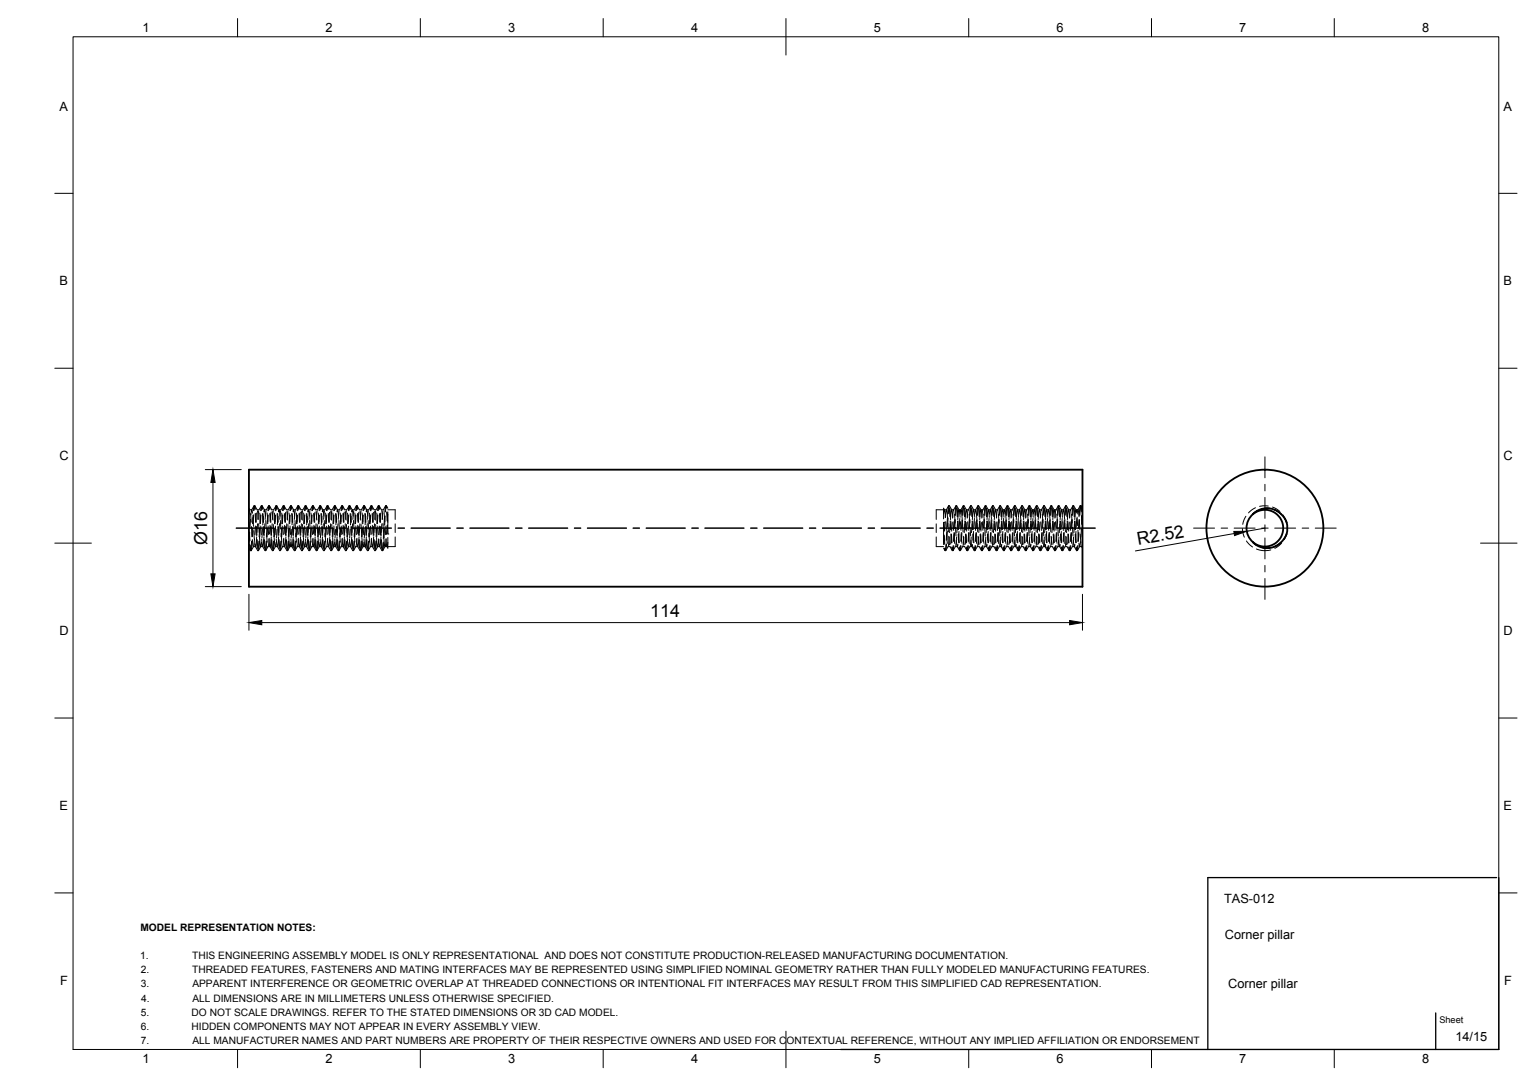
ISO-10303-21;
HEADER;
/* Generated by software containing ST-Developer
 * from STEP Tools, Inc. (www.steptools.com) 
 */

FILE_DESCRIPTION(
/* description */ (
'Independent welded steel electronics enclosure with removable sealed 
lid, internal mounting tray and two threaded cable entries. 300 x 220 
mm body. No ingress or electrical safety rating assigned.'),
/* implementation_level */ '2;1');

FILE_NAME(
/* name */ 'Corner pillar.step',
/* time_stamp */ '2026-11-14T09:13:27-08:00',
/* author */ (''),
/* organization */ (''),
/* preprocessor_version */ 'ST-DEVELOPER v20.2',
/* originating_system */ 'Autodesk Translation Framework v15.17.0.0',
/* authorisation */ '');

FILE_SCHEMA (('AUTOMOTIVE_DESIGN { 1 0 10303 214 3 1 1 }'));
ENDSEC;

DATA;
#10=MECHANICAL_DESIGN_GEOMETRIC_PRESENTATION_REPRESENTATION('',(#970),#94412);
#154=B_SPLINE_SURFACE_WITH_KNOTS('',3,3,((#38427,#38428,#38429,#38430,#38431,
#38432,#38433,#38434,#38435,#38436,#38437,#38438,#38439,#38440,#38441,#38442,
#38443,#38444,#38445,#38446,#38447,#38448,#38449,#38450,#38451,#38452,#38453,
#38454,#38455,#38456,#38457,#38458,#38459,#38460,#38461,#38462,#38463,#38464,
#38465,#38466,#38467,#38468,#38469,#38470,#38471,#38472,#38473,#38474,#38475,
#38476,#38477,#38478,#38479,#38480,#38481,#38482,#38483,#38484,#38485,#38486,
#38487,#38488,#38489,#38490,#38491,#38492,#38493,#38494,#38495,#38496,#38497,
#38498,#38499,#38500,#38501,#38502,#38503,#38504,#38505,#38506,#38507,#38508,
#38509,#38510,#38511,#38512,#38513,#38514,#38515,#38516,#38517,#38518,#38519,
#38520,#38521,#38522,#38523,#38524,#38525,#38526,#38527,#38528,#38529,#38530,
#38531,#38532,#38533,#38534,#38535,#38536,#38537,#38538,#38539,#38540,#38541,
#38542,#38543,#38544,#38545,#38546,#38547,#38548,#38549,#38550,#38551),
(#38552,#38553,#38554,#38555,#38556,#38557,#38558,#38559,#38560,#38561,
#38562,#38563,#38564,#38565,#38566,#38567,#38568,#38569,#38570,#38571,#38572,
#38573,#38574,#38575,#38576,#38577,#38578,#38579,#38580,#38581,#38582,#38583,
#38584,#38585,#38586,#38587,#38588,#38589,#38590,#38591,#38592,#38593,#38594,
#38595,#38596,#38597,#38598,#38599,#38600,#38601,#38602,#38603,#38604,#38605,
#38606,#38607,#38608,#38609,#38610,#38611,#38612,#38613,#38614,#38615,#38616,
#38617,#38618,#38619,#38620,#38621,#38622,#38623,#38624,#38625,#38626,#38627,
#38628,#38629,#38630,#38631,#38632,#38633,#38634,#38635,#38636,#38637,#38638,
#38639,#38640,#38641,#38642,#38643,#38644,#38645,#38646,#38647,#38648,#38649,
#38650,#38651,#38652,#38653,#38654,#38655,#38656,#38657,#38658,#38659,#38660,
#38661,#38662,#38663,#38664,#38665,#38666,#38667,#38668,#38669,#38670,#38671,
#38672,#38673,#38674,#38675,#38676),(#38677,#38678,#38679,#38680,#38681,
#38682,#38683,#38684,#38685,#38686,#38687,#38688,#38689,#38690,#38691,#38692,
#38693,#38694,#38695,#38696,#38697,#38698,#38699,#38700,#38701,#38702,#38703,
#38704,#38705,#38706,#38707,#38708,#38709,#38710,#38711,#38712,#38713,#38714,
#38715,#38716,#38717,#38718,#38719,#38720,#38721,#38722,#38723,#38724,#38725,
#38726,#38727,#38728,#38729,#38730,#38731,#38732,#38733,#38734,#38735,#38736,
#38737,#38738,#38739,#38740,#38741,#38742,#38743,#38744,#38745,#38746,#38747,
#38748,#38749,#38750,#38751,#38752,#38753,#38754,#38755,#38756,#38757,#38758,
#38759,#38760,#38761,#38762,#38763,#38764,#38765,#38766,#38767,#38768,#38769,
#38770,#38771,#38772,#38773,#38774,#38775,#38776,#38777,#38778,#38779,#38780,
#38781,#38782,#38783,#38784,#38785,#38786,#38787,#38788,#38789,#38790,#38791,
#38792,#38793,#38794,#38795,#38796,#38797,#38798,#38799,#38800,#38801),
(#38802,#38803,#38804,#38805,#38806,#38807,#38808,#38809,#38810,#38811,
#38812,#38813,#38814,#38815,#38816,#38817,#38818,#38819,#38820,#38821,#38822,
#38823,#38824,#38825,#38826,#38827,#38828,#38829,#38830,#38831,#38832,#38833,
#38834,#38835,#38836,#38837,#38838,#38839,#38840,#38841,#38842,#38843,#38844,
#38845,#38846,#38847,#38848,#38849,#38850,#38851,#38852,#38853,#38854,#38855,
#38856,#38857,#38858,#38859,#38860,#38861,#38862,#38863,#38864,#38865,#38866,
#38867,#38868,#38869,#38870,#38871,#38872,#38873,#38874,#38875,#38876,#38877,
#38878,#38879,#38880,#38881,#38882,#38883,#38884,#38885,#38886,#38887,#38888,
#38889,#38890,#38891,#38892,#38893,#38894,#38895,#38896,#38897,#38898,#38899,
#38900,#38901,#38902,#38903,#38904,#38905,#38906,#38907,#38908,#38909,#38910,
#38911,#38912,#38913,#38914,#38915,#38916,#38917,#38918,#38919,#38920,#38921,
#38922,#38923,#38924,#38925,#38926)),.UNSPECIFIED.,.F.,.F.,.F.,(4,4),(4,
1,1,1,1,1,1,1,1,1,1,1,1,1,1,1,1,1,1,1,1,1,1,1,1,1,1,1,1,1,1,1,1,1,1,1,1,
1,1,1,1,1,1,1,1,1,1,1,1,1,1,1,1,1,1,1,1,1,1,1,1,1,1,1,1,1,1,1,1,1,1,1,1,
1,1,1,1,1,1,1,1,1,1,1,1,1,1,1,1,1,1,1,1,1,1,1,1,1,1,1,1,1,1,1,1,1,1,1,1,
1,1,1,1,1,1,1,1,1,1,1,1,1,4),(-0.000512721802289974,0.0646569623865103),
(11.8584761405054,12.8540500568113,13.849111251315,14.8441724458186,15.8392336403222,
16.8342948348258,17.8293560293294,18.824417223833,19.8194784183366,20.8145396128402,
21.8096008073438,22.8046620018475,23.7997231963511,24.7947843908547,25.7898455853583,
26.7849067798619,27.7799679743655,28.7750291688691,29.7700903633727,30.7651515578764,
31.76021275238,32.7552739468836,33.7503351413872,34.7453963358908,35.7404575303944,
36.735518724898,37.7305799194016,38.7256411139052,39.7207023084089,40.7157635029125,
41.7108246974161,42.7058858919197,43.7009470864233,44.6960082809269,45.6910694754305,
46.6861306699341,47.6811918644377,48.6762530589414,49.671314253445,50.6663754479486,
51.6614366424522,52.6564978369558,53.6515590314594,54.646620225963,55.6416814204666,
56.6367426149702,57.6318038094739,58.6268650039775,59.6219261984811,60.6169873929847,
61.6120485874883,62.6071097819919,63.6021709764955,64.5972321709991,65.5922933655027,
66.5873545600064,67.58241575451,68.5774769490136,69.5725381435172,70.5675993380208,
71.5626605325244,72.557721727028,73.5527829215316,74.5478441160353,75.5429053105389,
76.5379665050425,77.5330276995461,78.5280888940497,79.5231500885533,80.5182112830569,
81.5132724775605,82.5083336720641,83.5033948665678,84.4984560610714,85.493517255575,
86.4885784500786,87.4836396445822,88.4787008390858,89.4737620335894,90.468823228093,
91.4638844225966,92.4589456171003,93.4540068116039,94.4490680061075,95.4441292006111,
96.4391903951147,97.4342515896183,98.4293127841219,99.4243739786255,100.419435173129,
101.414496367633,102.409557562136,103.40461875664,104.399679951144,105.394741145647,
106.389802340151,107.384863534654,108.379924729158,109.374985923662,110.370047118165,
111.365108312669,112.360169507172,113.355230701676,114.35029189618,115.345353090683,
116.340414285187,117.335475479691,118.330536674194,119.325597868698,120.320659063201,
121.315720257705,122.310781452209,123.305842646712,124.300903841216,125.295965035719,
126.291026230223,127.286087424727,128.28114861923,129.276209813734,130.271271008237,
131.266332202741,132.261393397245,133.256910204201),.UNSPECIFIED.);
#155=B_SPLINE_SURFACE_WITH_KNOTS('',3,3,((#39015,#39016,#39017,#39018,#39019,
#39020,#39021,#39022,#39023,#39024,#39025,#39026,#39027,#39028,#39029,#39030,
#39031,#39032,#39033,#39034,#39035,#39036,#39037,#39038,#39039,#39040,#39041,
#39042,#39043,#39044,#39045,#39046,#39047,#39048,#39049,#39050,#39051,#39052,
#39053,#39054,#39055,#39056,#39057,#39058,#39059,#39060,#39061,#39062,#39063,
#39064,#39065,#39066,#39067,#39068,#39069,#39070,#39071,#39072,#39073,#39074,
#39075,#39076,#39077,#39078,#39079,#39080,#39081,#39082,#39083,#39084,#39085,
#39086,#39087,#39088,#39089,#39090,#39091,#39092,#39093,#39094,#39095,#39096,
#39097,#39098,#39099,#39100,#39101,#39102,#39103,#39104,#39105,#39106,#39107,
#39108,#39109,#39110,#39111,#39112,#39113,#39114,#39115,#39116,#39117,#39118,
#39119,#39120,#39121,#39122,#39123,#39124,#39125,#39126,#39127,#39128,#39129,
#39130,#39131,#39132,#39133,#39134,#39135,#39136,#39137,#39138,#39139),
(#39140,#39141,#39142,#39143,#39144,#39145,#39146,#39147,#39148,#39149,
#39150,#39151,#39152,#39153,#39154,#39155,#39156,#39157,#39158,#39159,#39160,
#39161,#39162,#39163,#39164,#39165,#39166,#39167,#39168,#39169,#39170,#39171,
#39172,#39173,#39174,#39175,#39176,#39177,#39178,#39179,#39180,#39181,#39182,
#39183,#39184,#39185,#39186,#39187,#39188,#39189,#39190,#39191,#39192,#39193,
#39194,#39195,#39196,#39197,#39198,#39199,#39200,#39201,#39202,#39203,#39204,
#39205,#39206,#39207,#39208,#39209,#39210,#39211,#39212,#39213,#39214,#39215,
#39216,#39217,#39218,#39219,#39220,#39221,#39222,#39223,#39224,#39225,#39226,
#39227,#39228,#39229,#39230,#39231,#39232,#39233,#39234,#39235,#39236,#39237,
#39238,#39239,#39240,#39241,#39242,#39243,#39244,#39245,#39246,#39247,#39248,
#39249,#39250,#39251,#39252,#39253,#39254,#39255,#39256,#39257,#39258,#39259,
#39260,#39261,#39262,#39263,#39264),(#39265,#39266,#39267,#39268,#39269,
#39270,#39271,#39272,#39273,#39274,#39275,#39276,#39277,#39278,#39279,#39280,
#39281,#39282,#39283,#39284,#39285,#39286,#39287,#39288,#39289,#39290,#39291,
#39292,#39293,#39294,#39295,#39296,#39297,#39298,#39299,#39300,#39301,#39302,
#39303,#39304,#39305,#39306,#39307,#39308,#39309,#39310,#39311,#39312,#39313,
#39314,#39315,#39316,#39317,#39318,#39319,#39320,#39321,#39322,#39323,#39324,
#39325,#39326,#39327,#39328,#39329,#39330,#39331,#39332,#39333,#39334,#39335,
#39336,#39337,#39338,#39339,#39340,#39341,#39342,#39343,#39344,#39345,#39346,
#39347,#39348,#39349,#39350,#39351,#39352,#39353,#39354,#39355,#39356,#39357,
#39358,#39359,#39360,#39361,#39362,#39363,#39364,#39365,#39366,#39367,#39368,
#39369,#39370,#39371,#39372,#39373,#39374,#39375,#39376,#39377,#39378,#39379,
#39380,#39381,#39382,#39383,#39384,#39385,#39386,#39387,#39388,#39389),
(#39390,#39391,#39392,#39393,#39394,#39395,#39396,#39397,#39398,#39399,
#39400,#39401,#39402,#39403,#39404,#39405,#39406,#39407,#39408,#39409,#39410,
#39411,#39412,#39413,#39414,#39415,#39416,#39417,#39418,#39419,#39420,#39421,
#39422,#39423,#39424,#39425,#39426,#39427,#39428,#39429,#39430,#39431,#39432,
#39433,#39434,#39435,#39436,#39437,#39438,#39439,#39440,#39441,#39442,#39443,
#39444,#39445,#39446,#39447,#39448,#39449,#39450,#39451,#39452,#39453,#39454,
#39455,#39456,#39457,#39458,#39459,#39460,#39461,#39462,#39463,#39464,#39465,
#39466,#39467,#39468,#39469,#39470,#39471,#39472,#39473,#39474,#39475,#39476,
#39477,#39478,#39479,#39480,#39481,#39482,#39483,#39484,#39485,#39486,#39487,
#39488,#39489,#39490,#39491,#39492,#39493,#39494,#39495,#39496,#39497,#39498,
#39499,#39500,#39501,#39502,#39503,#39504,#39505,#39506,#39507,#39508,#39509,
#39510,#39511,#39512,#39513,#39514)),.UNSPECIFIED.,.F.,.F.,.F.,(4,4),(4,
1,1,1,1,1,1,1,1,1,1,1,1,1,1,1,1,1,1,1,1,1,1,1,1,1,1,1,1,1,1,1,1,1,1,1,1,
1,1,1,1,1,1,1,1,1,1,1,1,1,1,1,1,1,1,1,1,1,1,1,1,1,1,1,1,1,1,1,1,1,1,1,1,
1,1,1,1,1,1,1,1,1,1,1,1,1,1,1,1,1,1,1,1,1,1,1,1,1,1,1,1,1,1,1,1,1,1,1,1,
1,1,1,1,1,1,1,1,1,1,1,1,1,4),(-0.000455618124563469,0.0646112265793122),
(14.3984001269718,15.3934613214754,16.388522515979,17.3835837104826,18.3786449049862,
19.3737060994898,20.3687672939934,21.3638284884971,22.3588896830007,23.3539508775043,
24.3490120720079,25.3440732665115,26.3391344610151,27.3341956555187,28.3292568500223,
29.3243180445259,30.3193792390296,31.3144404335332,32.3095016280368,33.3045628225404,
34.299624017044,35.2946852115476,36.2897464060512,37.2848076005548,38.2798687950584,
39.2749299895621,40.2699911840657,41.2650523785693,42.2601135730729,43.2551747675765,
44.2502359620801,45.2452971565837,46.2403583510873,47.235419545591,48.2304807400946,
49.2255419345982,50.2206031291018,51.2156643236054,52.210725518109,53.2057867126126,
54.2008479071162,55.1959091016198,56.1909702961235,57.1860314906271,58.1810926851307,
59.1761538796343,60.1712150741379,61.1662762686415,62.1613374631451,63.1563986576487,
64.1514598521523,65.1465210466559,66.1415822411596,67.1366434356632,68.1317046301668,
69.1267658246704,70.121827019174,71.1168882136776,72.1119494081812,73.1070106026849,
74.1020717971885,75.0971329916921,76.0921941861957,77.0872553806993,78.0823165752029,
79.0773777697065,80.0724389642101,81.0675001587137,82.0625613532173,83.057622547721,
84.0526837422246,85.0477449367282,86.0428061312318,87.0378673257354,88.032928520239,
89.0279897147426,90.0230509092463,91.0181121037498,92.0131732982535,93.0082344927571,
94.0032956872607,94.9983568817643,95.9934180762679,96.9884792707715,97.9835404652751,
98.9786016597787,99.9736628542824,100.968724048786,101.96378524329,102.958846437793,
103.953907632297,104.9489688268,105.944030021304,106.939091215808,107.934152410311,
108.929213604815,109.924274799318,110.919335993822,111.914397188326,112.909458382829,
113.904519577333,114.899580771837,115.89464196634,116.889703160844,117.884764355347,
118.879825549851,119.874886744355,120.869947938858,121.865009133362,122.860070327865,
123.855131522369,124.850192716873,125.845253911376,126.84031510588,127.835376300383,
128.830437494887,129.825498689391,130.820559883894,131.815621078398,132.810682272902,
133.805743467405,134.800804661909,135.795865856412),.UNSPECIFIED.);
#156=B_SPLINE_SURFACE_WITH_KNOTS('',3,3,((#39790,#39791,#39792,#39793,#39794,
#39795,#39796,#39797,#39798,#39799,#39800,#39801,#39802,#39803,#39804,#39805,
#39806,#39807,#39808,#39809,#39810,#39811,#39812,#39813,#39814,#39815,#39816,
#39817,#39818,#39819,#39820,#39821,#39822,#39823,#39824,#39825,#39826,#39827,
#39828,#39829,#39830,#39831,#39832,#39833,#39834,#39835,#39836,#39837,#39838,
#39839,#39840,#39841,#39842,#39843,#39844,#39845,#39846,#39847,#39848,#39849,
#39850,#39851,#39852,#39853,#39854,#39855,#39856,#39857,#39858,#39859,#39860,
#39861,#39862,#39863,#39864,#39865,#39866,#39867,#39868,#39869,#39870,#39871,
#39872,#39873,#39874,#39875,#39876,#39877,#39878,#39879,#39880,#39881,#39882,
#39883,#39884,#39885,#39886,#39887,#39888,#39889,#39890,#39891,#39892,#39893,
#39894,#39895,#39896,#39897,#39898,#39899,#39900,#39901,#39902,#39903,#39904,
#39905,#39906,#39907,#39908,#39909,#39910,#39911,#39912,#39913,#39914),
(#39915,#39916,#39917,#39918,#39919,#39920,#39921,#39922,#39923,#39924,
#39925,#39926,#39927,#39928,#39929,#39930,#39931,#39932,#39933,#39934,#39935,
#39936,#39937,#39938,#39939,#39940,#39941,#39942,#39943,#39944,#39945,#39946,
#39947,#39948,#39949,#39950,#39951,#39952,#39953,#39954,#39955,#39956,#39957,
#39958,#39959,#39960,#39961,#39962,#39963,#39964,#39965,#39966,#39967,#39968,
#39969,#39970,#39971,#39972,#39973,#39974,#39975,#39976,#39977,#39978,#39979,
#39980,#39981,#39982,#39983,#39984,#39985,#39986,#39987,#39988,#39989,#39990,
#39991,#39992,#39993,#39994,#39995,#39996,#39997,#39998,#39999,#40000,#40001,
#40002,#40003,#40004,#40005,#40006,#40007,#40008,#40009,#40010,#40011,#40012,
#40013,#40014,#40015,#40016,#40017,#40018,#40019,#40020,#40021,#40022,#40023,
#40024,#40025,#40026,#40027,#40028,#40029,#40030,#40031,#40032,#40033,#40034,
#40035,#40036,#40037,#40038,#40039),(#40040,#40041,#40042,#40043,#40044,
#40045,#40046,#40047,#40048,#40049,#40050,#40051,#40052,#40053,#40054,#40055,
#40056,#40057,#40058,#40059,#40060,#40061,#40062,#40063,#40064,#40065,#40066,
#40067,#40068,#40069,#40070,#40071,#40072,#40073,#40074,#40075,#40076,#40077,
#40078,#40079,#40080,#40081,#40082,#40083,#40084,#40085,#40086,#40087,#40088,
#40089,#40090,#40091,#40092,#40093,#40094,#40095,#40096,#40097,#40098,#40099,
#40100,#40101,#40102,#40103,#40104,#40105,#40106,#40107,#40108,#40109,#40110,
#40111,#40112,#40113,#40114,#40115,#40116,#40117,#40118,#40119,#40120,#40121,
#40122,#40123,#40124,#40125,#40126,#40127,#40128,#40129,#40130,#40131,#40132,
#40133,#40134,#40135,#40136,#40137,#40138,#40139,#40140,#40141,#40142,#40143,
#40144,#40145,#40146,#40147,#40148,#40149,#40150,#40151,#40152,#40153,#40154,
#40155,#40156,#40157,#40158,#40159,#40160,#40161,#40162,#40163,#40164),
(#40165,#40166,#40167,#40168,#40169,#40170,#40171,#40172,#40173,#40174,
#40175,#40176,#40177,#40178,#40179,#40180,#40181,#40182,#40183,#40184,#40185,
#40186,#40187,#40188,#40189,#40190,#40191,#40192,#40193,#40194,#40195,#40196,
#40197,#40198,#40199,#40200,#40201,#40202,#40203,#40204,#40205,#40206,#40207,
#40208,#40209,#40210,#40211,#40212,#40213,#40214,#40215,#40216,#40217,#40218,
#40219,#40220,#40221,#40222,#40223,#40224,#40225,#40226,#40227,#40228,#40229,
#40230,#40231,#40232,#40233,#40234,#40235,#40236,#40237,#40238,#40239,#40240,
#40241,#40242,#40243,#40244,#40245,#40246,#40247,#40248,#40249,#40250,#40251,
#40252,#40253,#40254,#40255,#40256,#40257,#40258,#40259,#40260,#40261,#40262,
#40263,#40264,#40265,#40266,#40267,#40268,#40269,#40270,#40271,#40272,#40273,
#40274,#40275,#40276,#40277,#40278,#40279,#40280,#40281,#40282,#40283,#40284,
#40285,#40286,#40287,#40288,#40289)),.UNSPECIFIED.,.F.,.F.,.F.,(4,4),(4,
1,1,1,1,1,1,1,1,1,1,1,1,1,1,1,1,1,1,1,1,1,1,1,1,1,1,1,1,1,1,1,1,1,1,1,1,
1,1,1,1,1,1,1,1,1,1,1,1,1,1,1,1,1,1,1,1,1,1,1,1,1,1,1,1,1,1,1,1,1,1,1,1,
1,1,1,1,1,1,1,1,1,1,1,1,1,1,1,1,1,1,1,1,1,1,1,1,1,1,1,1,1,1,1,1,1,1,1,1,
1,1,1,1,1,1,1,1,1,1,1,1,1,4),(-0.000520200608884411,0.0646393933935523),
(11.8584686616988,12.8540500568113,13.8491112513149,14.8441724458185,15.8392336403222,
16.8342948348258,17.8293560293294,18.824417223833,19.8194784183366,20.8145396128402,
21.8096008073438,22.8046620018474,23.799723196351,24.7947843908547,25.7898455853583,
26.7849067798619,27.7799679743655,28.7750291688691,29.7700903633727,30.7651515578763,
31.7602127523799,32.7552739468835,33.7503351413872,34.7453963358908,35.7404575303944,
36.735518724898,37.7305799194016,38.7256411139052,39.7207023084088,40.7157635029124,
41.7108246974161,42.7058858919197,43.7009470864233,44.6960082809269,45.6910694754305,
46.6861306699341,47.6811918644377,48.6762530589413,49.6713142534449,50.6663754479486,
51.6614366424522,52.6564978369558,53.6515590314594,54.646620225963,55.6416814204666,
56.6367426149702,57.6318038094738,58.6268650039775,59.6219261984811,60.6169873929847,
61.6120485874883,62.6071097819919,63.6021709764955,64.5972321709991,65.5922933655027,
66.5873545600063,67.58241575451,68.5774769490136,69.5725381435172,70.5675993380208,
71.5626605325244,72.557721727028,73.5527829215316,74.5478441160352,75.5429053105389,
76.5379665050425,77.5330276995461,78.5280888940497,79.5231500885533,80.5182112830569,
81.5132724775605,82.5083336720641,83.5033948665677,84.4984560610714,85.493517255575,
86.4885784500786,87.4836396445822,88.4787008390858,89.4737620335894,90.468823228093,
91.4638844225966,92.4589456171003,93.4540068116039,94.4490680061075,95.4441292006111,
96.4391903951147,97.4342515896183,98.4293127841219,99.4243739786255,100.419435173129,
101.414496367633,102.409557562136,103.40461875664,104.399679951144,105.394741145647,
106.389802340151,107.384863534654,108.379924729158,109.374985923662,110.370047118165,
111.365108312669,112.360169507172,113.355230701676,114.35029189618,115.345353090683,
116.340414285187,117.335475479691,118.330536674194,119.325597868698,120.320659063201,
121.315720257705,122.310781452209,123.305842646712,124.300903841216,125.295965035719,
126.291026230223,127.286087424727,128.28114861923,129.276209813734,130.271271008237,
131.266332202741,132.261393397245,133.256454591748),.UNSPECIFIED.);
#157=B_SPLINE_SURFACE_WITH_KNOTS('',3,3,((#40378,#40379,#40380,#40381,#40382,
#40383,#40384,#40385,#40386,#40387,#40388,#40389,#40390,#40391,#40392,#40393,
#40394,#40395,#40396,#40397,#40398,#40399,#40400,#40401,#40402,#40403,#40404,
#40405,#40406,#40407,#40408,#40409,#40410,#40411,#40412,#40413,#40414,#40415,
#40416,#40417,#40418,#40419,#40420,#40421,#40422,#40423,#40424,#40425,#40426,
#40427,#40428,#40429,#40430,#40431,#40432,#40433,#40434,#40435,#40436,#40437,
#40438,#40439,#40440,#40441,#40442,#40443,#40444,#40445,#40446,#40447,#40448,
#40449,#40450,#40451,#40452,#40453,#40454,#40455,#40456,#40457,#40458,#40459,
#40460,#40461,#40462,#40463,#40464,#40465,#40466,#40467,#40468,#40469,#40470,
#40471,#40472,#40473,#40474,#40475,#40476,#40477,#40478,#40479,#40480,#40481,
#40482,#40483,#40484,#40485,#40486,#40487,#40488,#40489,#40490,#40491,#40492,
#40493,#40494,#40495,#40496,#40497,#40498,#40499,#40500,#40501,#40502),
(#40503,#40504,#40505,#40506,#40507,#40508,#40509,#40510,#40511,#40512,
#40513,#40514,#40515,#40516,#40517,#40518,#40519,#40520,#40521,#40522,#40523,
#40524,#40525,#40526,#40527,#40528,#40529,#40530,#40531,#40532,#40533,#40534,
#40535,#40536,#40537,#40538,#40539,#40540,#40541,#40542,#40543,#40544,#40545,
#40546,#40547,#40548,#40549,#40550,#40551,#40552,#40553,#40554,#40555,#40556,
#40557,#40558,#40559,#40560,#40561,#40562,#40563,#40564,#40565,#40566,#40567,
#40568,#40569,#40570,#40571,#40572,#40573,#40574,#40575,#40576,#40577,#40578,
#40579,#40580,#40581,#40582,#40583,#40584,#40585,#40586,#40587,#40588,#40589,
#40590,#40591,#40592,#40593,#40594,#40595,#40596,#40597,#40598,#40599,#40600,
#40601,#40602,#40603,#40604,#40605,#40606,#40607,#40608,#40609,#40610,#40611,
#40612,#40613,#40614,#40615,#40616,#40617,#40618,#40619,#40620,#40621,#40622,
#40623,#40624,#40625,#40626,#40627),(#40628,#40629,#40630,#40631,#40632,
#40633,#40634,#40635,#40636,#40637,#40638,#40639,#40640,#40641,#40642,#40643,
#40644,#40645,#40646,#40647,#40648,#40649,#40650,#40651,#40652,#40653,#40654,
#40655,#40656,#40657,#40658,#40659,#40660,#40661,#40662,#40663,#40664,#40665,
#40666,#40667,#40668,#40669,#40670,#40671,#40672,#40673,#40674,#40675,#40676,
#40677,#40678,#40679,#40680,#40681,#40682,#40683,#40684,#40685,#40686,#40687,
#40688,#40689,#40690,#40691,#40692,#40693,#40694,#40695,#40696,#40697,#40698,
#40699,#40700,#40701,#40702,#40703,#40704,#40705,#40706,#40707,#40708,#40709,
#40710,#40711,#40712,#40713,#40714,#40715,#40716,#40717,#40718,#40719,#40720,
#40721,#40722,#40723,#40724,#40725,#40726,#40727,#40728,#40729,#40730,#40731,
#40732,#40733,#40734,#40735,#40736,#40737,#40738,#40739,#40740,#40741,#40742,
#40743,#40744,#40745,#40746,#40747,#40748,#40749,#40750,#40751,#40752),
(#40753,#40754,#40755,#40756,#40757,#40758,#40759,#40760,#40761,#40762,
#40763,#40764,#40765,#40766,#40767,#40768,#40769,#40770,#40771,#40772,#40773,
#40774,#40775,#40776,#40777,#40778,#40779,#40780,#40781,#40782,#40783,#40784,
#40785,#40786,#40787,#40788,#40789,#40790,#40791,#40792,#40793,#40794,#40795,
#40796,#40797,#40798,#40799,#40800,#40801,#40802,#40803,#40804,#40805,#40806,
#40807,#40808,#40809,#40810,#40811,#40812,#40813,#40814,#40815,#40816,#40817,
#40818,#40819,#40820,#40821,#40822,#40823,#40824,#40825,#40826,#40827,#40828,
#40829,#40830,#40831,#40832,#40833,#40834,#40835,#40836,#40837,#40838,#40839,
#40840,#40841,#40842,#40843,#40844,#40845,#40846,#40847,#40848,#40849,#40850,
#40851,#40852,#40853,#40854,#40855,#40856,#40857,#40858,#40859,#40860,#40861,
#40862,#40863,#40864,#40865,#40866,#40867,#40868,#40869,#40870,#40871,#40872,
#40873,#40874,#40875,#40876,#40877)),.UNSPECIFIED.,.F.,.F.,.F.,(4,4),(4,
1,1,1,1,1,1,1,1,1,1,1,1,1,1,1,1,1,1,1,1,1,1,1,1,1,1,1,1,1,1,1,1,1,1,1,1,
1,1,1,1,1,1,1,1,1,1,1,1,1,1,1,1,1,1,1,1,1,1,1,1,1,1,1,1,1,1,1,1,1,1,1,1,
1,1,1,1,1,1,1,1,1,1,1,1,1,1,1,1,1,1,1,1,1,1,1,1,1,1,1,1,1,1,1,1,1,1,1,1,
1,1,1,1,1,1,1,1,1,1,1,1,1,4),(-0.000457317293645526,0.064610822672929),
(14.3984001269718,15.3934613214754,16.388522515979,17.3835837104827,18.3786449049863,
19.3737060994899,20.3687672939935,21.3638284884971,22.3588896830007,23.3539508775043,
24.3490120720079,25.3440732665115,26.3391344610152,27.3341956555188,28.3292568500224,
29.324318044526,30.3193792390296,31.3144404335332,32.3095016280368,33.3045628225404,
34.299624017044,35.2946852115477,36.2897464060513,37.2848076005549,38.2798687950585,
39.2749299895621,40.2699911840657,41.2650523785693,42.2601135730729,43.2551747675765,
44.2502359620802,45.2452971565838,46.2403583510874,47.235419545591,48.2304807400946,
49.2255419345982,50.2206031291018,51.2156643236054,52.2107255181091,53.2057867126127,
54.2008479071163,55.1959091016199,56.1909702961235,57.1860314906271,58.1810926851307,
59.1761538796343,60.1712150741379,61.1662762686416,62.1613374631452,63.1563986576488,
64.1514598521524,65.146521046656,66.1415822411596,67.1366434356632,68.1317046301668,
69.1267658246704,70.121827019174,71.1168882136777,72.1119494081813,73.1070106026849,
74.1020717971885,75.0971329916921,76.0921941861957,77.0872553806993,78.082316575203,
79.0773777697065,80.0724389642102,81.0675001587138,82.0625613532174,83.057622547721,
84.0526837422246,85.0477449367282,86.0428061312318,87.0378673257354,88.0329285202391,
89.0279897147427,90.0230509092463,91.0181121037499,92.0131732982535,93.0082344927571,
94.0032956872607,94.9983568817644,95.9934180762679,96.9884792707716,97.9835404652752,
98.9786016597788,99.9736628542824,100.968724048786,101.96378524329,102.958846437793,
103.953907632297,104.9489688268,105.944030021304,106.939091215808,107.934152410311,
108.929213604815,109.924274799319,110.919335993822,111.914397188326,112.909458382829,
113.904519577333,114.899580771837,115.89464196634,116.889703160844,117.884764355347,
118.879825549851,119.874886744355,120.869947938858,121.865009133362,122.860070327865,
123.855131522369,124.850192716873,125.845253911376,126.84031510588,127.835376300384,
128.830437494887,129.825498689391,130.820559883894,131.815621078398,132.810682272902,
133.805743467405,134.800804661909,135.795865856412),.UNSPECIFIED.);
#170=B_SPLINE_CURVE_WITH_KNOTS('',3,(#10608,#10609,#10610,#10611,#10612,
#10613,#10614,#10615,#10616,#10617,#10618,#10619,#10620,#10621,#10622,#10623,
#10624,#10625,#10626,#10627,#10628,#10629,#10630,#10631,#10632,#10633,#10634,
#10635,#10636,#10637,#10638,#10639,#10640,#10641,#10642,#10643,#10644,#10645,
#10646,#10647,#10648,#10649,#10650,#10651,#10652,#10653,#10654,#10655,#10656,
#10657,#10658,#10659,#10660,#10661,#10662,#10663,#10664,#10665,#10666,#10667,
#10668,#10669,#10670,#10671,#10672,#10673,#10674,#10675,#10676,#10677,#10678,
#10679,#10680,#10681,#10682,#10683),.UNSPECIFIED.,.F.,.F.,(4,3,3,3,3,3,
3,3,3,3,3,3,3,3,3,3,3,3,3,3,3,3,3,3,3,4),(131.030639485952,131.124862922685,
131.219235943061,131.266332202741,131.359553276607,131.452645853409,131.54563967122,
131.638570862278,131.731470852847,131.82436633402,131.917283987168,132.01031659896,
132.103410766158,132.196676516921,132.261393397245,132.358253800053,132.454968934237,
132.555154641426,132.651629546133,132.748037988853,132.844400764937,132.940738621606,
133.037097136043,133.133466654998,133.229897556966,133.256454591748),
 .UNSPECIFIED.);
#171=B_SPLINE_CURVE_WITH_KNOTS('',3,(#10686,#10687,#10688,#10689,#10690,
#10691,#10692,#10693,#10694,#10695,#10696,#10697,#10698,#10699,#10700,#10701,
#10702,#10703,#10704,#10705,#10706,#10707,#10708,#10709,#10710,#10711,#10712,
#10713,#10714,#10715,#10716,#10717,#10718,#10719,#10720,#10721,#10722,#10723,
#10724,#10725,#10726,#10727,#10728,#10729,#10730,#10731,#10732,#10733,#10734,
#10735,#10736,#10737,#10738,#10739,#10740,#10741,#10742,#10743,#10744,#10745,
#10746,#10747,#10748,#10749,#10750,#10751,#10752,#10753,#10754,#10755,#10756,
#10757,#10758,#10759,#10760,#10761,#10762,#10763,#10764,#10765,#10766,#10767,
#10768,#10769,#10770,#10771,#10772,#10773,#10774,#10775,#10776,#10777,#10778,
#10779),.UNSPECIFIED.,.F.,.F.,(4,3,3,3,3,3,3,3,3,3,3,3,3,3,3,3,3,3,3,3,
3,3,3,3,3,3,3,3,3,3,3,4),(131.031745185056,131.129729671724,131.223528237148,
131.317300342785,131.41107178814,131.504868364938,131.598771830413,131.692738307433,
131.78685139804,131.815621078398,131.910038792203,132.004328170091,132.098517526913,
132.192637791453,132.286722645945,132.380797529135,132.474887864195,132.569075924233,
132.663317785296,132.757707314553,132.810682272902,132.904609653633,132.998411531174,
133.095962894,133.189603092652,133.283213322859,133.376819590518,133.470447891049,
133.564178560621,133.657969940107,133.751903898015,133.778822433787),
 .UNSPECIFIED.);
#172=B_SPLINE_CURVE_WITH_KNOTS('',3,(#10785,#10786,#10787,#10788,#10789,
#10790,#10791,#10792,#10793,#10794,#10795,#10796,#10797,#10798,#10799,#10800,
#10801,#10802,#10803,#10804,#10805,#10806,#10807,#10808,#10809,#10810,#10811,
#10812,#10813,#10814,#10815,#10816,#10817,#10818,#10819,#10820,#10821,#10822,
#10823,#10824,#10825,#10826,#10827,#10828,#10829,#10830,#10831,#10832,#10833,
#10834,#10835,#10836,#10837,#10838,#10839,#10840,#10841,#10842,#10843,#10844,
#10845,#10846,#10847,#10848,#10849,#10850,#10851,#10852,#10853,#10854,#10855,
#10856,#10857,#10858,#10859,#10860,#10861,#10862,#10863,#10864,#10865,#10866,
#10867,#10868,#10869,#10870,#10871,#10872,#10873,#10874,#10875,#10876,#10877,
#10878,#10879,#10880,#10881,#10882,#10883,#10884,#10885,#10886,#10887,#10888,
#10889,#10890,#10891,#10892,#10893,#10894,#10895,#10896,#10897,#10898,#10899,
#10900,#10901,#10902,#10903,#10904,#10905,#10906,#10907,#10908,#10909,#10910,
#10911,#10912,#10913,#10914,#10915,#10916,#10917,#10918,#10919,#10920),
 .UNSPECIFIED.,.F.,.F.,(4,3,3,3,3,3,3,3,3,3,3,3,3,3,3,3,3,3,3,3,3,3,3,3,
3,3,3,3,3,3,3,3,3,3,3,3,3,3,3,3,3,3,3,3,3,4),(124.748128028511,124.842034576069,
124.935951918733,125.0299669327,125.124031831941,125.218255583323,125.295965035719,
125.390184105335,125.484275308534,125.578267220964,125.672191936185,125.766082489566,
125.859964553955,125.953863787903,126.047864515545,126.141920902379,126.236129692714,
126.291026230223,126.385285904234,126.479417652453,126.573449997981,126.667414816189,
126.761345254291,126.855266938143,126.949205479067,127.043244801221,127.137339437753,
127.231585558755,127.286087424727,127.380353085992,127.474491224045,127.568530347491,
127.662502487566,127.756440580176,127.850370239497,127.944317065442,128.038365089124,
128.132468674872,128.226724042984,128.28114861923,128.378996644742,128.476673059547,
128.574146032619,128.671497438999,128.768713686957,128.805298797182),
 .UNSPECIFIED.);
#173=B_SPLINE_CURVE_WITH_KNOTS('',3,(#10921,#10922,#10923,#10924,#10925,
#10926,#10927,#10928,#10929,#10930,#10931,#10932,#10933,#10934,#10935,#10936,
#10937,#10938,#10939,#10940,#10941,#10942,#10943,#10944,#10945,#10946,#10947,
#10948,#10949,#10950,#10951,#10952,#10953,#10954,#10955,#10956,#10957,#10958,
#10959,#10960,#10961,#10962,#10963,#10964,#10965,#10966,#10967,#10968,#10969,
#10970,#10971,#10972,#10973,#10974,#10975,#10976,#10977,#10978,#10979,#10980,
#10981,#10982,#10983,#10984,#10985,#10986,#10987,#10988,#10989,#10990,#10991,
#10992,#10993),.UNSPECIFIED.,.F.,.F.,(4,3,3,3,3,3,3,3,3,3,3,3,3,3,3,3,3,
3,3,3,3,3,3,3,4),(128.805298797455,128.904575923864,129.004169174393,129.103925506044,
129.203971261245,129.276209813734,129.370627582079,129.464917013993,129.559106424263,
129.653226741186,129.747311647382,129.84138658154,129.935476966773,130.029665075484,
130.123906984442,130.218296559918,130.271271008237,130.366192067951,130.460422790932,
130.554564192512,130.648641837038,130.744141249266,130.838189532557,130.934414509254,
131.030639485952),.UNSPECIFIED.);
#174=B_SPLINE_CURVE_WITH_KNOTS('',3,(#10995,#10996,#10997,#10998,#10999,
#11000,#11001,#11002,#11003,#11004,#11005,#11006,#11007,#11008,#11009,#11010,
#11011,#11012,#11013,#11014,#11015,#11016,#11017,#11018,#11019,#11020,#11021,
#11022,#11023,#11024,#11025,#11026,#11027,#11028,#11029,#11030,#11031,#11032,
#11033,#11034,#11035,#11036,#11037,#11038,#11039,#11040,#11041,#11042,#11043,
#11044,#11045,#11046,#11047,#11048,#11049,#11050,#11051,#11052,#11053,#11054,
#11055,#11056,#11057,#11058,#11059,#11060,#11061,#11062,#11063,#11064,#11065,
#11066,#11067,#11068,#11069,#11070,#11071,#11072,#11073),.UNSPECIFIED.,
 .F.,.F.,(4,3,3,3,3,3,3,3,3,3,3,3,3,3,3,3,3,3,3,3,3,3,3,3,3,3,4),(128.805298797182,
128.830437494887,128.924697154801,129.018828889054,129.112861220763,129.206826025422,
129.300756450148,129.394678120809,129.488616648745,129.582655958293,129.676750582416,
129.770996691439,129.825498689391,129.919764295011,130.01390237706,130.107941444223,
130.201913527833,130.295851563885,130.389781166627,130.483727936041,130.577775903607,
130.671879433392,130.766134746334,130.820559883894,130.914675364851,131.0086511327,
131.031745185056),.UNSPECIFIED.);
#175=B_SPLINE_CURVE_WITH_KNOTS('',3,(#11074,#11075,#11076,#11077,#11078,
#11079,#11080,#11081),.UNSPECIFIED.,.F.,.F.,(4,1,1,1,1,4),(124.74739205894,
124.850192716873,125.845253911376,126.84031510588,127.835376300383,128.805295331209),
 .UNSPECIFIED.);
#176=B_SPLINE_CURVE_WITH_KNOTS('',3,(#11087,#11088,#11089,#11090,#11091,
#11092,#11093,#11094,#11095,#11096,#11097,#11098,#11099,#11100,#11101,#11102,
#11103,#11104,#11105,#11106,#11107,#11108,#11109,#11110,#11111,#11112,#11113,
#11114,#11115,#11116,#11117,#11118,#11119,#11120,#11121,#11122,#11123,#11124,
#11125,#11126,#11127,#11128,#11129,#11130,#11131,#11132,#11133,#11134,#11135,
#11136,#11137,#11138,#11139,#11140,#11141,#11142,#11143,#11144,#11145,#11146,
#11147,#11148,#11149,#11150,#11151,#11152,#11153,#11154,#11155,#11156,#11157,
#11158,#11159,#11160,#11161,#11162,#11163,#11164,#11165,#11166,#11167,#11168,
#11169,#11170,#11171,#11172,#11173,#11174,#11175,#11176,#11177,#11178,#11179,
#11180,#11181,#11182,#11183,#11184,#11185,#11186,#11187,#11188,#11189,#11190,
#11191,#11192,#11193,#11194,#11195,#11196,#11197,#11198,#11199,#11200,#11201,
#11202,#11203,#11204,#11205,#11206,#11207,#11208,#11209,#11210,#11211,#11212,
#11213,#11214,#11215,#11216,#11217,#11218,#11219),.UNSPECIFIED.,.F.,.F.,
(4,3,3,3,3,3,3,3,3,3,3,3,3,3,3,3,3,3,3,3,3,3,3,3,3,3,3,3,3,3,3,3,3,3,3,
3,3,3,3,3,3,3,3,3,4),(118.465309189798,118.559373810011,118.655151817347,
118.749077565128,118.842980638927,118.936886679199,119.034064476574,119.128108308656,
119.226853088677,119.325597868698,119.419836017092,119.513946331371,119.607957361602,
119.701901126583,119.795810680877,119.889711674647,119.983629743695,120.077649048852,
120.171723895481,120.26595077801,120.320659063201,120.414897817102,120.509008734383,
120.603020364354,120.696964721818,120.790874863903,120.884776440091,120.978695085495,
121.072714954328,121.166790358315,121.261017782786,121.315720257705,121.409959739289,
121.504071392924,121.598083766821,121.69202887633,121.78593977519,121.879842111928,
121.973761520711,122.067782152519,122.16185832038,122.256086502537,122.310781452209,
122.4414864556,122.522113490002),.UNSPECIFIED.);
#177=B_SPLINE_CURVE_WITH_KNOTS('',3,(#11220,#11221,#11222,#11223,#11224,
#11225,#11226,#11227,#11228,#11229,#11230,#11231,#11232,#11233,#11234,#11235,
#11236,#11237,#11238,#11239,#11240,#11241,#11242,#11243,#11244,#11245,#11246,
#11247,#11248,#11249,#11250,#11251,#11252,#11253,#11254,#11255,#11256,#11257,
#11258,#11259,#11260,#11261,#11262,#11263,#11264,#11265,#11266,#11267,#11268,
#11269,#11270,#11271,#11272,#11273,#11274,#11275,#11276,#11277,#11278,#11279,
#11280,#11281,#11282,#11283,#11284,#11285,#11286,#11287,#11288,#11289,#11290,
#11291,#11292,#11293,#11294,#11295),.UNSPECIFIED.,.F.,.F.,(4,3,3,3,3,3,
3,3,3,3,3,3,3,3,3,3,3,3,3,3,3,3,3,3,3,4),(122.522113490206,122.614859586664,
122.707525591219,122.800150201744,122.892760399084,122.985383144327,123.078100878442,
123.170872581003,123.263789214971,123.305842646712,123.400083492223,123.494196487762,
123.588210180099,123.682156568083,123.776068720305,123.869972283944,123.96389289179,
124.057914673282,124.151991964677,124.246221218337,124.300903841216,124.395154214485,
124.489253372224,124.583264788189,124.677212213272,124.748128028511),
 .UNSPECIFIED.);
#178=B_SPLINE_CURVE_WITH_KNOTS('',3,(#11297,#11298,#11299,#11300,#11301,
#11302),.UNSPECIFIED.,.F.,.F.,(4,1,1,4),(122.522113490002,122.860070327865,
123.855131522369,124.74739205894),.UNSPECIFIED.);
#179=B_SPLINE_CURVE_WITH_KNOTS('',3,(#11303,#11304,#11305,#11306,#11307,
#11308,#11309,#11310),.UNSPECIFIED.,.F.,.F.,(4,1,1,1,1,4),(118.464366347269,
118.879825549851,119.874886744355,120.869947938858,121.865009133362,122.522113490002),
 .UNSPECIFIED.);
#180=B_SPLINE_CURVE_WITH_KNOTS('',3,(#11316,#11317,#11318,#11319,#11320,
#11321,#11322,#11323,#11324,#11325,#11326,#11327,#11328,#11329,#11330,#11331,
#11332,#11333,#11334,#11335,#11336,#11337,#11338,#11339,#11340,#11341,#11342,
#11343,#11344,#11345,#11346,#11347,#11348,#11349,#11350,#11351,#11352,#11353,
#11354,#11355,#11356,#11357,#11358,#11359,#11360,#11361,#11362,#11363,#11364,
#11365,#11366,#11367,#11368,#11369,#11370,#11371,#11372,#11373,#11374,#11375,
#11376,#11377,#11378,#11379,#11380,#11381,#11382,#11383,#11384,#11385,#11386,
#11387,#11388,#11389,#11390,#11391,#11392,#11393,#11394,#11395,#11396,#11397,
#11398,#11399,#11400,#11401,#11402,#11403,#11404,#11405,#11406,#11407,#11408,
#11409,#11410,#11411,#11412,#11413,#11414,#11415,#11416,#11417,#11418,#11419,
#11420,#11421,#11422,#11423,#11424,#11425,#11426,#11427,#11428,#11429,#11430,
#11431,#11432,#11433,#11434,#11435,#11436,#11437,#11438,#11439,#11440,#11441,
#11442,#11443,#11444,#11445,#11446,#11447,#11448,#11449,#11450,#11451),
 .UNSPECIFIED.,.F.,.F.,(4,3,3,3,3,3,3,3,3,3,3,3,3,3,3,3,3,3,3,3,3,3,3,3,
3,3,3,3,3,3,3,3,3,3,3,3,3,3,3,3,3,3,3,3,3,4),(112.181027744827,112.275243743586,
112.360169507172,112.454408044935,112.548518748739,112.642530168135,112.736474320159,
112.830384260048,112.924285637504,113.018204087869,113.112223768433,113.20629898769,
113.3005262348,113.355230701676,113.449469228602,113.543579921563,113.637591330125,
113.731535471375,113.825445400529,113.919346767303,114.013265207052,114.107284877163,
114.201360086044,114.295587323002,114.35029189618,114.444530429606,114.538641128994,
114.632652543903,114.726596691355,114.820506626619,114.914407999406,115.008326445062,
115.102346120886,115.196421335378,115.290648577732,115.345353090683,115.438408490029,
115.531337087903,115.624161186544,115.716928481106,115.809665873421,115.90240022995,
115.995209800998,116.088059601802,116.181043570387,116.238928182603),
 .UNSPECIFIED.);
#181=B_SPLINE_CURVE_WITH_KNOTS('',3,(#11452,#11453,#11454,#11455,#11456,
#11457,#11458,#11459,#11460,#11461,#11462,#11463,#11464,#11465,#11466,#11467,
#11468,#11469,#11470,#11471,#11472,#11473,#11474,#11475,#11476,#11477,#11478,
#11479,#11480,#11481,#11482,#11483,#11484,#11485,#11486,#11487,#11488,#11489,
#11490,#11491,#11492,#11493,#11494,#11495,#11496,#11497,#11498,#11499,#11500,
#11501,#11502,#11503,#11504,#11505,#11506,#11507,#11508,#11509,#11510,#11511,
#11512,#11513,#11514,#11515,#11516,#11517,#11518,#11519,#11520,#11521,#11522,
#11523,#11524,#11525,#11526,#11527),.UNSPECIFIED.,.F.,.F.,(4,3,3,3,3,3,
3,3,3,3,3,3,3,3,3,3,3,3,3,3,3,3,3,3,3,4),(116.238928182822,116.340414285187,
116.434652766824,116.528763414508,116.622774777863,116.716718874193,116.810628758621,
116.904530080917,116.998448476488,117.092468103145,117.186543268915,117.280770463729,
117.335475479691,117.429714028249,117.523824742414,117.617836171729,117.711780332983,
117.805690281671,117.899591667489,117.993510125772,118.087529813532,118.18160503959,
118.275832292814,118.330536674194,118.424770353341,118.465309189798),
 .UNSPECIFIED.);
#182=B_SPLINE_CURVE_WITH_KNOTS('',3,(#11529,#11530,#11531,#11532,#11533,
#11534),.UNSPECIFIED.,.F.,.F.,(4,1,1,4),(116.238928182822,116.889703160844,
117.884764355347,118.464366347269),.UNSPECIFIED.);
#183=B_SPLINE_CURVE_WITH_KNOTS('',3,(#11535,#11536,#11537,#11538,#11539,
#11540,#11541,#11542),.UNSPECIFIED.,.F.,.F.,(4,1,1,1,1,4),(112.182488223733,
112.909458382829,113.904519577333,114.899580771837,115.89464196634,116.238928182822),
 .UNSPECIFIED.);
#184=B_SPLINE_CURVE_WITH_KNOTS('',3,(#11548,#11549,#11550,#11551,#11552,
#11553,#11554,#11555,#11556,#11557,#11558,#11559,#11560,#11561,#11562,#11563,
#11564,#11565,#11566,#11567,#11568,#11569,#11570,#11571,#11572,#11573,#11574,
#11575,#11576,#11577,#11578,#11579,#11580,#11581,#11582,#11583,#11584,#11585,
#11586,#11587,#11588,#11589,#11590,#11591,#11592,#11593,#11594,#11595,#11596,
#11597,#11598,#11599,#11600,#11601,#11602,#11603,#11604,#11605,#11606,#11607,
#11608,#11609,#11610,#11611,#11612,#11613,#11614,#11615,#11616,#11617,#11618,
#11619,#11620,#11621,#11622,#11623,#11624,#11625,#11626,#11627,#11628,#11629,
#11630,#11631,#11632,#11633,#11634,#11635,#11636,#11637,#11638,#11639,#11640,
#11641,#11642,#11643,#11644,#11645,#11646,#11647,#11648,#11649,#11650,#11651,
#11652,#11653,#11654,#11655,#11656,#11657,#11658,#11659,#11660,#11661,#11662,
#11663,#11664,#11665,#11666,#11667,#11668,#11669,#11670,#11671,#11672,#11673,
#11674,#11675,#11676,#11677,#11678,#11679,#11680,#11681,#11682,#11683),
 .UNSPECIFIED.,.F.,.F.,(4,3,3,3,3,3,3,3,3,3,3,3,3,3,3,3,3,3,3,3,3,3,3,3,
3,3,3,3,3,3,3,3,3,3,3,3,3,3,3,3,3,3,3,3,3,4),(105.898399443487,105.992303958498,
106.08623467724,106.180271478522,106.274372028075,106.368615159332,106.389802340151,
106.484040874008,106.578151573893,106.672162989362,106.766107137465,106.860017073436,
106.953918446983,107.047836893455,107.141856570169,107.235931785597,107.330159028946,
107.384863534654,107.479102068317,107.573212768008,107.667224183284,107.761168331195,
107.855078266976,107.948979640334,108.042898086619,108.136917763148,108.230992978392,
108.325220221563,108.379924729158,108.474163262819,108.568273962506,108.662285377776,
108.756229525679,108.850139461449,108.944040834797,109.037959281067,109.131978957582,
109.226054172809,109.320281415961,109.374985923662,109.471046274508,109.566961713017,
109.664157003673,109.759830056109,109.857786465876,109.955742875643),
 .UNSPECIFIED.);
#185=B_SPLINE_CURVE_WITH_KNOTS('',3,(#11684,#11685,#11686,#11687,#11688,
#11689,#11690,#11691,#11692,#11693,#11694,#11695,#11696,#11697,#11698,#11699,
#11700,#11701,#11702,#11703,#11704,#11705,#11706,#11707,#11708,#11709,#11710,
#11711,#11712,#11713,#11714,#11715,#11716,#11717,#11718,#11719,#11720,#11721,
#11722,#11723,#11724,#11725,#11726,#11727,#11728,#11729,#11730,#11731,#11732,
#11733,#11734,#11735,#11736,#11737,#11738,#11739,#11740,#11741,#11742,#11743,
#11744,#11745,#11746,#11747,#11748,#11749,#11750,#11751,#11752,#11753,#11754,
#11755,#11756),.UNSPECIFIED.,.F.,.F.,(4,3,3,3,3,3,3,3,3,3,3,3,3,3,3,3,3,
3,3,3,3,3,3,3,4),(109.955742875829,110.059318936413,110.162337101908,110.266192110037,
110.370047118165,110.464285651067,110.558396349998,110.652407764516,110.746351911677,
110.840261846711,110.934163219329,111.028081664878,111.122101340687,111.216176555218,
111.310403797692,111.365108312669,111.459358827616,111.55345200354,111.647455302587,
111.741394476697,111.835295216048,111.929214837184,112.023142266139,112.117153308002,
112.181027744827),.UNSPECIFIED.);
#186=B_SPLINE_CURVE_WITH_KNOTS('',3,(#11758,#11759,#11760,#11761,#11762,
#11763),.UNSPECIFIED.,.F.,.F.,(4,1,1,4),(109.955742875643,110.919335993822,
111.914397188326,112.182488223733),.UNSPECIFIED.);
#187=B_SPLINE_CURVE_WITH_KNOTS('',3,(#11764,#11765,#11766,#11767,#11768,
#11769,#11770,#11771,#11772),.UNSPECIFIED.,.F.,.F.,(4,1,1,1,1,1,4),(105.898136542595,
105.944030021304,106.939091215808,107.934152410311,108.929213604815,109.924274799318,
109.955742875643),.UNSPECIFIED.);
#188=B_SPLINE_CURVE_WITH_KNOTS('',3,(#11778,#11779,#11780,#11781,#11782,
#11783,#11784,#11785,#11786,#11787,#11788,#11789,#11790,#11791,#11792,#11793,
#11794,#11795,#11796,#11797,#11798,#11799,#11800,#11801,#11802,#11803,#11804,
#11805,#11806,#11807,#11808,#11809,#11810,#11811,#11812,#11813,#11814,#11815,
#11816,#11817,#11818,#11819,#11820,#11821,#11822,#11823,#11824,#11825,#11826,
#11827,#11828,#11829,#11830,#11831,#11832,#11833,#11834,#11835,#11836,#11837,
#11838,#11839,#11840,#11841,#11842,#11843,#11844,#11845,#11846,#11847,#11848,
#11849,#11850,#11851,#11852,#11853,#11854,#11855,#11856,#11857,#11858,#11859,
#11860,#11861,#11862,#11863,#11864,#11865,#11866,#11867,#11868,#11869,#11870,
#11871,#11872,#11873,#11874,#11875,#11876,#11877,#11878,#11879,#11880,#11881,
#11882,#11883,#11884,#11885,#11886,#11887,#11888,#11889,#11890,#11891,#11892,
#11893,#11894,#11895,#11896,#11897,#11898,#11899,#11900,#11901,#11902,#11903,
#11904,#11905,#11906,#11907,#11908,#11909,#11910,#11911,#11912,#11913),
 .UNSPECIFIED.,.F.,.F.,(4,3,3,3,3,3,3,3,3,3,3,3,3,3,3,3,3,3,3,3,3,3,3,3,
3,3,3,3,3,3,3,3,3,3,3,3,3,3,3,3,3,3,3,3,3,4),(99.6158155142023,99.7098241487408,
99.8037667638163,99.8976760105222,99.9915775377616,100.085496980766,100.179518115865,
100.273595547336,100.36782410646,100.419435173129,100.513673706899,100.607784406696,
100.701795822077,100.795739970093,100.889649905977,100.983551279438,101.077469725824,
101.171489402453,101.265564617795,101.359791861062,101.414496367633,101.5087349014,
101.602845601194,101.696857016572,101.790801164585,101.884711100466,101.978612473925,
102.072530920308,102.166550596934,102.260625812274,102.354853055537,102.409557562136,
102.5037960959,102.597906795691,102.691918211066,102.785862359076,102.879772294954,
102.97367366841,103.067592114789,103.161611791412,103.255687006749,103.34991425001,
103.40461875664,103.524030082473,103.64134504394,103.672557568263),
 .UNSPECIFIED.);
#189=B_SPLINE_CURVE_WITH_KNOTS('',3,(#11914,#11915,#11916,#11917,#11918,
#11919,#11920,#11921,#11922,#11923,#11924,#11925,#11926,#11927,#11928,#11929,
#11930,#11931,#11932,#11933,#11934,#11935,#11936,#11937,#11938,#11939,#11940,
#11941,#11942,#11943,#11944,#11945,#11946,#11947,#11948,#11949,#11950,#11951,
#11952,#11953,#11954,#11955,#11956,#11957,#11958,#11959,#11960,#11961,#11962,
#11963,#11964,#11965,#11966,#11967,#11968,#11969,#11970,#11971,#11972,#11973,
#11974,#11975,#11976,#11977,#11978,#11979,#11980,#11981,#11982,#11983,#11984,
#11985,#11986,#11987,#11988,#11989),.UNSPECIFIED.,.F.,.F.,(4,3,3,3,3,3,
3,3,3,3,3,3,3,3,3,3,3,3,3,3,3,3,3,3,3,4),(103.672557568463,103.765628528253,
103.858652863662,103.951657206799,104.04466816524,104.137772858376,104.230925480976,
104.324235541602,104.399679951144,104.4939184849,104.588029184684,104.682040600052,
104.775984748054,104.869894683925,104.963796057374,105.057714503746,105.151734180363,
105.245809395693,105.340036638947,105.394741145647,105.488978918377,105.583093547084,
105.677096798483,105.771035902528,105.864939461167,105.898399443487),
 .UNSPECIFIED.);
#190=B_SPLINE_CURVE_WITH_KNOTS('',3,(#11991,#11992,#11993,#11994,#11995,
#11996),.UNSPECIFIED.,.F.,.F.,(4,1,1,4),(103.672557568463,103.953907632297,
104.9489688268,105.898136542595),.UNSPECIFIED.);
#191=B_SPLINE_CURVE_WITH_KNOTS('',3,(#11997,#11998,#11999,#12000,#12001,
#12002,#12003,#12004),.UNSPECIFIED.,.F.,.F.,(4,1,1,1,1,4),(99.6145705654374,
99.9736628542824,100.968724048786,101.96378524329,102.958846437793,103.672557568463),
 .UNSPECIFIED.);
#192=B_SPLINE_CURVE_WITH_KNOTS('',3,(#12010,#12011,#12012,#12013,#12014,
#12015,#12016,#12017,#12018,#12019,#12020,#12021,#12022,#12023,#12024,#12025,
#12026,#12027,#12028,#12029,#12030,#12031,#12032,#12033,#12034,#12035,#12036,
#12037,#12038,#12039,#12040,#12041,#12042,#12043,#12044,#12045,#12046,#12047,
#12048,#12049,#12050,#12051,#12052,#12053,#12054,#12055,#12056,#12057,#12058,
#12059,#12060,#12061,#12062,#12063,#12064,#12065,#12066,#12067,#12068,#12069,
#12070,#12071,#12072,#12073,#12074,#12075,#12076,#12077,#12078,#12079,#12080,
#12081,#12082,#12083,#12084,#12085,#12086,#12087,#12088,#12089,#12090,#12091,
#12092,#12093,#12094,#12095,#12096,#12097,#12098,#12099,#12100,#12101,#12102,
#12103,#12104,#12105,#12106,#12107,#12108,#12109,#12110,#12111,#12112,#12113,
#12114,#12115,#12116,#12117,#12118,#12119,#12120,#12121,#12122,#12123,#12124,
#12125,#12126,#12127,#12128,#12129,#12130,#12131,#12132,#12133,#12134,#12135,
#12136,#12137,#12138,#12139,#12140,#12141,#12142,#12143,#12144,#12145,#12146,
#12147,#12148),.UNSPECIFIED.,.F.,.F.,(4,3,3,3,3,3,3,3,3,3,3,3,3,3,3,3,3,
3,3,3,3,3,3,3,3,3,3,3,3,3,3,3,3,3,3,3,3,3,3,3,3,3,3,3,3,3,4),(93.3315517313818,
93.4257912333858,93.4540068116039,93.548245345372,93.6423560451674,93.7363674605468,
93.8303116085609,93.9242215444431,94.0181229179026,94.1120413642863,94.2060610409137,
94.3001362562545,94.394363499519,94.4490680061075,94.5433065398756,94.6374172396711,
94.7314286550505,94.8253728030646,94.9192827389468,95.0131841124064,95.1071025587901,
95.2011222354176,95.2951974507585,95.389424694023,95.4441292006111,95.5383677343792,
95.6324784341746,95.7264898495538,95.820433997568,95.9143439334501,96.0082453069096,
96.1021637532933,96.1961834299208,96.2902586452616,96.3844858885261,96.4391903951147,
96.5327727036347,96.6262277012863,96.7216207712496,96.8149119236731,96.9081721054003,
97.0014277028664,97.0984138423979,97.1917929587829,97.2852342917175,97.3788110498964,
97.3893722609925),.UNSPECIFIED.);
#193=B_SPLINE_CURVE_WITH_KNOTS('',3,(#12149,#12150,#12151,#12152,#12153,
#12154,#12155,#12156,#12157,#12158,#12159,#12160,#12161,#12162,#12163,#12164,
#12165,#12166,#12167,#12168,#12169,#12170,#12171,#12172,#12173,#12174,#12175,
#12176,#12177,#12178,#12179,#12180,#12181,#12182,#12183,#12184,#12185,#12186,
#12187,#12188,#12189,#12190,#12191,#12192,#12193,#12194,#12195,#12196,#12197,
#12198,#12199,#12200,#12201,#12202,#12203,#12204,#12205,#12206,#12207,#12208,
#12209,#12210,#12211,#12212,#12213,#12214,#12215,#12216,#12217,#12218,#12219,
#12220,#12221,#12222,#12223,#12224),.UNSPECIFIED.,.F.,.F.,(4,3,3,3,3,3,
3,3,3,3,3,3,3,3,3,3,3,3,3,3,3,3,3,3,3,4),(97.3893722612835,97.4342515896183,
97.5284901233866,97.6226008231821,97.7166122385618,97.8105563865762,97.9044663224586,
97.9983676959184,98.0922861423024,98.18630581893,98.280381034271,98.3746082775358,
98.4293127841219,98.5235513178899,98.6176620176852,98.7116734330645,98.8056175810786,
98.8995275169606,98.99342889042,99.0873473368037,99.181367013431,99.2754422287717,
99.3696694720362,99.4243739786255,99.5200947464139,99.6158155142023),
 .UNSPECIFIED.);
#194=B_SPLINE_CURVE_WITH_KNOTS('',3,(#12226,#12227,#12228,#12229,#12230,
#12231),.UNSPECIFIED.,.F.,.F.,(4,1,1,4),(97.3893722612835,97.9835404652751,
98.9786016597787,99.6145705654374),.UNSPECIFIED.);
#195=B_SPLINE_CURVE_WITH_KNOTS('',3,(#12232,#12233,#12234,#12235,#12236,
#12237,#12238,#12239),.UNSPECIFIED.,.F.,.F.,(4,1,1,1,1,4),(93.3328220857922,
94.0032956872607,94.9983568817643,95.9934180762679,96.9884792707715,97.3893722612835),
 .UNSPECIFIED.);
#196=B_SPLINE_CURVE_WITH_KNOTS('',3,(#12245,#12246,#12247,#12248,#12249,
#12250,#12251,#12252,#12253,#12254,#12255,#12256,#12257,#12258,#12259,#12260,
#12261,#12262,#12263,#12264,#12265,#12266,#12267,#12268,#12269,#12270,#12271,
#12272,#12273,#12274,#12275,#12276,#12277,#12278,#12279,#12280,#12281,#12282,
#12283,#12284,#12285,#12286,#12287,#12288,#12289,#12290,#12291,#12292,#12293,
#12294,#12295,#12296,#12297,#12298,#12299,#12300,#12301,#12302,#12303,#12304,
#12305,#12306,#12307,#12308,#12309,#12310,#12311,#12312,#12313,#12314,#12315,
#12316,#12317,#12318,#12319,#12320,#12321,#12322,#12323,#12324,#12325,#12326,
#12327,#12328,#12329,#12330,#12331,#12332,#12333,#12334,#12335,#12336,#12337,
#12338,#12339,#12340,#12341,#12342,#12343,#12344,#12345,#12346,#12347,#12348,
#12349,#12350,#12351,#12352,#12353,#12354,#12355,#12356,#12357,#12358,#12359,
#12360,#12361,#12362,#12363,#12364,#12365,#12366,#12367,#12368,#12369,#12370,
#12371,#12372,#12373,#12374,#12375,#12376,#12377,#12378,#12379,#12380),
 .UNSPECIFIED.,.F.,.F.,(4,3,3,3,3,3,3,3,3,3,3,3,3,3,3,3,3,3,3,3,3,3,3,3,
3,3,3,3,3,3,3,3,3,3,3,3,3,3,3,3,3,3,3,3,3,4),(87.0486737068653,87.1425908968732,
87.2366087113943,87.3306810779644,87.424906653528,87.4836396445822,87.5778781783503,
87.6719888781456,87.7660002935252,87.8599444415393,87.9538543774215,88.0477557508808,
88.1416741972643,88.2356938738917,88.3297690892326,88.4239963324971,88.4787008390858,
88.5729393728539,88.6670500726492,88.7610614880287,88.8550056360428,88.9489155719249,
89.0428169453844,89.1367353917684,89.2307550683958,89.3248302837367,89.4190575270012,
89.4737620335894,89.5680005673576,89.6621112671529,89.7561226825329,89.8500668305469,
89.9439767664291,90.0378781398886,90.1317965862726,90.2258162628999,90.3198914782409,
90.4141187215054,90.468823228093,90.5634949768986,90.6580371372986,90.7524748824258,
90.8468296227406,90.9411345169126,91.0354333352937,91.106186954104),
 .UNSPECIFIED.);
#197=B_SPLINE_CURVE_WITH_KNOTS('',3,(#12381,#12382,#12383,#12384,#12385,
#12386,#12387,#12388,#12389,#12390,#12391,#12392,#12393,#12394,#12395,#12396,
#12397,#12398,#12399,#12400,#12401,#12402,#12403,#12404,#12405,#12406,#12407,
#12408,#12409,#12410,#12411,#12412,#12413,#12414,#12415,#12416,#12417,#12418,
#12419,#12420,#12421,#12422,#12423,#12424,#12425,#12426,#12427,#12428,#12429,
#12430,#12431,#12432,#12433,#12434,#12435,#12436,#12437,#12438,#12439,#12440,
#12441,#12442,#12443,#12444,#12445,#12446,#12447,#12448,#12449,#12450,#12451,
#12452,#12453,#12454,#12455,#12456),.UNSPECIFIED.,.F.,.F.,(4,3,3,3,3,3,
3,3,3,3,3,3,3,3,3,3,3,3,3,3,3,3,3,3,3,4),(91.1061869543323,91.213064427723,
91.3204667481002,91.4284945161649,91.4638844225966,91.5581229563647,91.65223365616,
91.7462450715394,91.8401892195535,91.9340991554356,92.0280005288953,92.121918975279,
92.2159386519064,92.3100138672473,92.4042411105118,92.4589456171003,92.5531921674731,
92.6504871129617,92.7444873978673,92.8384257693604,92.9323279140037,93.0262194804531,
93.1201637235949,93.2141400856374,93.3082154234006,93.3315517313818),
 .UNSPECIFIED.);
#198=B_SPLINE_CURVE_WITH_KNOTS('',3,(#12458,#12459,#12460,#12461,#12462,
#12463),.UNSPECIFIED.,.F.,.F.,(4,1,1,4),(91.106186954104,92.0131732982535,
93.0082344927571,93.3328220857922),.UNSPECIFIED.);
#199=B_SPLINE_CURVE_WITH_KNOTS('',3,(#12464,#12465,#12466,#12467,#12468,
#12469,#12470,#12471),.UNSPECIFIED.,.F.,.F.,(4,1,1,1,1,4),(87.0489316649163,
88.032928520239,89.0279897147426,90.0230509092463,91.0181121037498,91.106186954104),
 .UNSPECIFIED.);
#200=B_SPLINE_CURVE_WITH_KNOTS('',3,(#12477,#12478,#12479,#12480,#12481,
#12482,#12483,#12484,#12485,#12486,#12487,#12488,#12489,#12490,#12491,#12492,
#12493,#12494,#12495,#12496,#12497,#12498,#12499,#12500,#12501,#12502,#12503,
#12504,#12505,#12506,#12507,#12508,#12509,#12510,#12511,#12512,#12513,#12514,
#12515,#12516,#12517,#12518,#12519,#12520,#12521,#12522,#12523,#12524,#12525,
#12526,#12527,#12528,#12529,#12530,#12531,#12532,#12533,#12534,#12535,#12536,
#12537,#12538,#12539,#12540,#12541,#12542,#12543,#12544,#12545,#12546,#12547,
#12548,#12549,#12550,#12551,#12552,#12553,#12554,#12555,#12556,#12557,#12558,
#12559,#12560,#12561,#12562,#12563,#12564,#12565,#12566,#12567,#12568,#12569,
#12570,#12571,#12572,#12573,#12574,#12575,#12576,#12577,#12578,#12579,#12580,
#12581,#12582,#12583,#12584,#12585,#12586,#12587,#12588,#12589,#12590,#12591,
#12592,#12593,#12594,#12595,#12596,#12597,#12598,#12599,#12600,#12601,#12602,
#12603,#12604,#12605,#12606,#12607,#12608,#12609),.UNSPECIFIED.,.F.,.F.,
(4,3,3,3,3,3,3,3,3,3,3,3,3,3,3,3,3,3,3,3,3,3,3,3,3,3,3,3,3,3,3,3,3,3,3,
3,3,3,3,3,3,3,3,3,4),(80.7662489266783,80.8602119699798,80.9541314258835,
81.0480329545828,81.1419421942353,81.2359473431976,81.3299996171077,81.4242143061157,
81.5132724775605,81.6075110113286,81.7016217111242,81.7956331265037,81.8895772745178,
81.9834872103999,82.0773885838594,82.1713070302434,82.2653267068708,82.3594019222119,
82.4536291654764,82.5083336720641,82.6025722058322,82.6966829056277,82.7906943210076,
82.8846384690218,82.9785484049039,83.0724497783636,83.1663682247472,83.2603879013746,
83.3544631167155,83.44869035998,83.5033948665678,83.5976334003359,83.6917441001315,
83.7857555155109,83.879699663525,83.9736095994071,84.0675109728665,84.1614294192497,
84.2554490958772,84.3495243112182,84.4437515544827,84.4984560610714,84.6098153997727,
84.7200586670623,84.8230016467187),.UNSPECIFIED.);
#201=B_SPLINE_CURVE_WITH_KNOTS('',3,(#12610,#12611,#12612,#12613,#12614,
#12615,#12616,#12617,#12618,#12619,#12620,#12621,#12622,#12623,#12624,#12625,
#12626,#12627,#12628,#12629,#12630,#12631,#12632,#12633,#12634,#12635,#12636,
#12637,#12638,#12639,#12640,#12641,#12642,#12643,#12644,#12645,#12646,#12647,
#12648,#12649,#12650,#12651,#12652,#12653,#12654,#12655,#12656,#12657,#12658,
#12659,#12660,#12661,#12662,#12663,#12664,#12665,#12666,#12667,#12668,#12669,
#12670,#12671,#12672,#12673,#12674,#12675,#12676,#12677,#12678,#12679,#12680,
#12681,#12682,#12683,#12684,#12685),.UNSPECIFIED.,.F.,.F.,(4,3,3,3,3,3,
3,3,3,3,3,3,3,3,3,3,3,3,3,3,3,3,3,3,3,4),(84.8230016469244,84.9167396222475,
85.0104582715235,85.1041833778222,85.2015168472604,85.2953896866708,85.3893326790534,
85.4834206132757,85.493517255575,85.5877557893431,85.6818664891383,85.7758779045175,
85.8698220525316,85.9637319884137,86.0576333618732,86.1515518082569,86.2455714848842,
86.3396467002252,86.4338739434898,86.4885784500786,86.5828095671125,86.6769188826881,
86.7709219388292,86.864861379201,86.9587807538247,87.0486737068653),
 .UNSPECIFIED.);
#202=B_SPLINE_CURVE_WITH_KNOTS('',3,(#12687,#12688,#12689,#12690,#12691,
#12692,#12693),.UNSPECIFIED.,.F.,.F.,(4,1,1,1,4),(84.8230016469244,85.0477449367282,
86.0428061312318,87.0378673257354,87.0489316649163),.UNSPECIFIED.);
#203=B_SPLINE_CURVE_WITH_KNOTS('',3,(#12694,#12695,#12696,#12697,#12698,
#12699,#12700,#12701),.UNSPECIFIED.,.F.,.F.,(4,1,1,1,1,4),(80.7648480623333,
81.0675001587137,82.0625613532173,83.057622547721,84.0526837422246,84.8230016469244),
 .UNSPECIFIED.);
#204=B_SPLINE_CURVE_WITH_KNOTS('',3,(#12707,#12708,#12709,#12710,#12711,
#12712,#12713,#12714,#12715),.UNSPECIFIED.,.F.,.F.,(4,1,1,1,1,1,4),(74.4820968515054,
74.5478441160353,75.5429053105389,76.5379665050425,77.5330276995461,78.5280888940497,
78.5398163397448),.UNSPECIFIED.);
#205=B_SPLINE_CURVE_WITH_KNOTS('',3,(#12716,#12717,#12718,#12719,#12720,
#12721,#12722,#12723,#12724,#12725,#12726,#12727,#12728,#12729,#12730,#12731,
#12732,#12733,#12734,#12735,#12736,#12737,#12738,#12739,#12740,#12741,#12742,
#12743,#12744,#12745,#12746,#12747,#12748,#12749,#12750,#12751,#12752,#12753,
#12754,#12755,#12756,#12757,#12758,#12759,#12760,#12761,#12762,#12763,#12764,
#12765,#12766,#12767,#12768,#12769,#12770,#12771,#12772,#12773,#12774,#12775,
#12776,#12777,#12778,#12779,#12780,#12781,#12782,#12783,#12784,#12785,#12786,
#12787,#12788,#12789,#12790,#12791),.UNSPECIFIED.,.F.,.F.,(4,3,3,3,3,3,
3,3,3,3,3,3,3,3,3,3,3,3,3,3,3,3,3,3,3,4),(78.5398163397448,78.6338611328131,
78.7277784183953,78.8215970084241,78.9153494264419,79.0090686503385,79.1027805638895,
79.1965110375713,79.290343065833,79.3842324145137,79.4782706042544,79.5231500885533,
79.6173886223214,79.7114993221167,79.8055107374961,79.8994548855102,79.9933648213923,
80.087266194852,80.1811846412356,80.275204317863,80.3692795332038,80.4635067764684,
80.5182112830569,80.6124499986686,80.7065483033557,80.7662489266783),
 .UNSPECIFIED.);
#206=B_SPLINE_CURVE_WITH_KNOTS('',3,(#12793,#12794,#12795,#12796,#12797,
#12798),.UNSPECIFIED.,.F.,.F.,(4,1,1,4),(78.5398163397448,79.0773777697065,
80.0724389642101,80.7648480623333),.UNSPECIFIED.);
#207=B_SPLINE_CURVE_WITH_KNOTS('',3,(#12799,#12800,#12801,#12802,#12803,
#12804,#12805,#12806),.UNSPECIFIED.,.F.,.F.,(4,1,1,1,1,4),(74.483068094227,
75.0971329916921,76.0921941861957,77.0872553806993,78.0823165752029,78.5398163397448),
 .UNSPECIFIED.);
#208=B_SPLINE_CURVE_WITH_KNOTS('',3,(#12812,#12813,#12814,#12815,#12816,
#12817,#12818,#12819),.UNSPECIFIED.,.F.,.F.,(4,1,1,1,1,4),(68.1987206882195,
68.5774769490136,69.5725381435172,70.5675993380208,71.5626605325244,72.2566310325652),
 .UNSPECIFIED.);
#209=B_SPLINE_CURVE_WITH_KNOTS('',3,(#12820,#12821,#12822,#12823,#12824,
#12825),.UNSPECIFIED.,.F.,.F.,(4,1,1,4),(72.2566310325652,72.557721727028,
73.5527829215316,74.4820968515054),.UNSPECIFIED.);
#210=B_SPLINE_CURVE_WITH_KNOTS('',3,(#12827,#12828,#12829,#12830,#12831,
#12832),.UNSPECIFIED.,.F.,.F.,(4,1,1,4),(72.2566310325652,73.1070106026849,
74.1020717971885,74.483068094227),.UNSPECIFIED.);
#211=B_SPLINE_CURVE_WITH_KNOTS('',3,(#12833,#12834,#12835,#12836,#12837,
#12838,#12839,#12840),.UNSPECIFIED.,.F.,.F.,(4,1,1,1,1,4),(68.1997135830677,
69.1267658246704,70.121827019174,71.1168882136776,72.1119494081812,72.2566310325652),
 .UNSPECIFIED.);
#212=B_SPLINE_CURVE_WITH_KNOTS('',3,(#12846,#12847,#12848,#12849,#12850,
#12851,#12852,#12853),.UNSPECIFIED.,.F.,.F.,(4,1,1,1,1,4),(61.9169450544327,
62.6071097819919,63.6021709764955,64.5972321709991,65.5922933655027,65.9734457253856),
 .UNSPECIFIED.);
#213=B_SPLINE_CURVE_WITH_KNOTS('',3,(#12854,#12855,#12856,#12857,#12858,
#12859),.UNSPECIFIED.,.F.,.F.,(4,1,1,4),(65.9734457253856,66.5873545600064,
67.58241575451,68.1987206882195),.UNSPECIFIED.);
#214=B_SPLINE_CURVE_WITH_KNOTS('',3,(#12861,#12862,#12863,#12864,#12865,
#12866,#12867),.UNSPECIFIED.,.F.,.F.,(4,1,1,1,4),(65.9734457253856,66.1415822411596,
67.1366434356632,68.1317046301668,68.1997135830677),.UNSPECIFIED.);
#215=B_SPLINE_CURVE_WITH_KNOTS('',3,(#12868,#12869,#12870,#12871,#12872,
#12873,#12874,#12875,#12876,#12877,#12878,#12879,#12880,#12881,#12882,#12883,
#12884,#12885,#12886,#12887,#12888,#12889,#12890,#12891,#12892,#12893,#12894,
#12895,#12896,#12897,#12898,#12899,#12900,#12901,#12902,#12903,#12904,#12905,
#12906,#12907,#12908,#12909,#12910,#12911,#12912,#12913,#12914,#12915,#12916,
#12917,#12918,#12919,#12920,#12921,#12922,#12923,#12924,#12925,#12926,#12927,
#12928,#12929,#12930,#12931,#12932,#12933,#12934,#12935,#12936,#12937,#12938,
#12939,#12940,#12941,#12942,#12943,#12944,#12945,#12946,#12947,#12948,#12949,
#12950,#12951,#12952,#12953,#12954,#12955,#12956,#12957,#12958,#12959,#12960,
#12961,#12962,#12963,#12964,#12965,#12966,#12967,#12968,#12969,#12970,#12971,
#12972,#12973,#12974,#12975,#12976,#12977,#12978,#12979,#12980,#12981,#12982,
#12983,#12984,#12985,#12986,#12987,#12988,#12989,#12990,#12991,#12992,#12993,
#12994,#12995,#12996,#12997,#12998,#12999,#13000,#13001,#13002,#13003),
 .UNSPECIFIED.,.F.,.F.,(4,3,3,3,3,3,3,3,3,3,3,3,3,3,3,3,3,3,3,3,3,3,3,3,
3,3,3,3,3,3,3,3,3,3,3,3,3,3,3,3,3,3,3,3,3,4),(61.9155474649507,62.0096207055437,
62.1038467898607,62.1613374631451,62.2555759969132,62.3496866967087,62.443698112088,
62.5376422601021,62.6315521959843,62.7254535694438,62.8193720158276,62.913391692455,
63.0074669077958,63.1016941510604,63.1563986576487,63.2506371914168,63.3447478912122,
63.4387593065916,63.5327034546057,63.6266133904879,63.7205147639474,63.8144332103311,
63.9084528869585,64.0025281022993,64.0967553455639,64.1514598521523,64.2456983859204,
64.3398090857158,64.4338205010951,64.5277646491093,64.6216745849914,64.715575958451,
64.8094944048347,64.903514081462,64.9975892968029,65.0918165400675,65.1465210466559,
65.2393639284444,65.3320574568455,65.4246665115195,65.5172182347161,65.6097397018219,
65.7023016612752,65.7948804375009,65.887574788458,65.9734457253856),
 .UNSPECIFIED.);
#216=B_SPLINE_CURVE_WITH_KNOTS('',3,(#13009,#13010,#13011,#13012,#13013,
#13014,#13015,#13016,#13017),.UNSPECIFIED.,.F.,.F.,(4,1,1,1,1,1,4),(55.63288052974,
55.6416814204666,56.6367426149702,57.6318038094739,58.6268650039775,59.6219261984811,
59.690260418206),.UNSPECIFIED.);
#217=B_SPLINE_CURVE_WITH_KNOTS('',3,(#13018,#13019,#13020,#13021,#13022,
#13023),.UNSPECIFIED.,.F.,.F.,(4,1,1,4),(59.690260418206,60.6169873929847,
61.6120485874883,61.9169450544327),.UNSPECIFIED.);
#218=B_SPLINE_CURVE_WITH_KNOTS('',3,(#13025,#13026,#13027,#13028,#13029,
#13030,#13031,#13032,#13033,#13034,#13035,#13036,#13037,#13038,#13039,#13040,
#13041,#13042,#13043,#13044,#13045,#13046,#13047,#13048,#13049,#13050,#13051,
#13052,#13053,#13054,#13055,#13056,#13057,#13058,#13059,#13060,#13061,#13062,
#13063,#13064,#13065,#13066,#13067,#13068,#13069,#13070,#13071,#13072,#13073,
#13074,#13075,#13076,#13077,#13078,#13079,#13080,#13081,#13082,#13083,#13084,
#13085,#13086,#13087,#13088,#13089,#13090,#13091,#13092,#13093,#13094,#13095,
#13096,#13097),.UNSPECIFIED.,.F.,.F.,(4,3,3,3,3,3,3,3,3,3,3,3,3,3,3,3,3,
3,3,3,3,3,3,3,4),(59.69026041838,59.7892918179424,59.8886169604212,59.9880911992762,
60.0878449487758,60.1712150741379,60.265453607906,60.3595643077015,60.453575723081,
60.5475198710951,60.6414298069773,60.7353311804368,60.8292496268206,60.9232693034479,
61.0173445187888,61.1115717620534,61.1662762686415,61.2604897277826,61.3545858806246,
61.4485905700231,61.5425295525125,61.636449941463,61.7303545167224,61.8243186129422,
61.9155474649507),.UNSPECIFIED.);
#219=B_SPLINE_CURVE_WITH_KNOTS('',3,(#13098,#13099,#13100,#13101,#13102,
#13103,#13104,#13105,#13106,#13107,#13108,#13109,#13110,#13111,#13112,#13113,
#13114,#13115,#13116,#13117,#13118,#13119,#13120,#13121,#13122,#13123,#13124,
#13125,#13126,#13127,#13128,#13129,#13130,#13131,#13132,#13133,#13134,#13135,
#13136,#13137,#13138,#13139,#13140,#13141,#13142,#13143,#13144,#13145,#13146,
#13147,#13148,#13149,#13150,#13151,#13152,#13153,#13154,#13155,#13156,#13157,
#13158,#13159,#13160,#13161,#13162,#13163,#13164,#13165,#13166,#13167,#13168,
#13169,#13170,#13171,#13172,#13173,#13174,#13175,#13176,#13177,#13178,#13179,
#13180,#13181,#13182,#13183,#13184,#13185,#13186,#13187,#13188,#13189,#13190,
#13191,#13192,#13193,#13194,#13195,#13196,#13197,#13198,#13199,#13200,#13201,
#13202,#13203,#13204,#13205,#13206,#13207,#13208,#13209,#13210,#13211,#13212,
#13213,#13214,#13215,#13216,#13217,#13218,#13219,#13220,#13221,#13222,#13223,
#13224,#13225,#13226,#13227,#13228,#13229,#13230,#13231,#13232,#13233),
 .UNSPECIFIED.,.F.,.F.,(4,3,3,3,3,3,3,3,3,3,3,3,3,3,3,3,3,3,3,3,3,3,3,3,
3,3,3,3,3,3,3,3,3,3,3,3,3,3,3,3,3,3,3,3,3,4),(55.6331177742522,55.7270192353002,
55.8209287590395,55.9149343983334,56.0089874786209,56.1032025709014,56.1909702961235,
56.2852088298917,56.3793195296874,56.4733309450668,56.5672750930809,56.661185028963,
56.7550864024225,56.8490048488062,56.9430245254336,57.0370997407745,57.1313269840391,
57.1860314906271,57.2802700243952,57.3743807241905,57.4683921395699,57.562336287584,
57.656246223466,57.7501475969256,57.8440660433095,57.9380857199369,58.0321609352777,
58.1263881785422,58.1810926851307,58.2753312188987,58.3694419186941,58.463453334074,
58.557397482088,58.6513074179702,58.7452087914297,58.8391272378137,58.933146914441,
59.0272221297817,59.1214493730463,59.1761538796343,59.274502750808,59.3726743921946,
59.4706312790708,59.568458264237,59.6661366206854,59.690260418206),
 .UNSPECIFIED.);
#220=B_SPLINE_CURVE_WITH_KNOTS('',3,(#13239,#13240,#13241,#13242,#13243,
#13244,#13245,#13246),.UNSPECIFIED.,.F.,.F.,(4,1,1,1,1,4),(49.3489697493475,
49.671314253445,50.6663754479486,51.6614366424522,52.6564978369558,53.4070751110264),
 .UNSPECIFIED.);
#221=B_SPLINE_CURVE_WITH_KNOTS('',3,(#13247,#13248,#13249,#13250,#13251,
#13252),.UNSPECIFIED.,.F.,.F.,(4,1,1,4),(53.4070751110264,53.6515590314594,
54.646620225963,55.63288052974),.UNSPECIFIED.);
#222=B_SPLINE_CURVE_WITH_KNOTS('',3,(#13254,#13255,#13256,#13257,#13258,
#13259,#13260,#13261,#13262,#13263,#13264,#13265,#13266,#13267,#13268,#13269,
#13270,#13271,#13272,#13273,#13274,#13275,#13276,#13277,#13278,#13279,#13280,
#13281,#13282,#13283,#13284,#13285,#13286,#13287,#13288,#13289,#13290,#13291,
#13292,#13293,#13294,#13295,#13296,#13297,#13298,#13299,#13300,#13301,#13302,
#13303,#13304,#13305,#13306,#13307,#13308,#13309,#13310,#13311,#13312,#13313,
#13314,#13315,#13316,#13317,#13318,#13319,#13320,#13321,#13322,#13323,#13324,
#13325,#13326,#13327,#13328,#13329),.UNSPECIFIED.,.F.,.F.,(4,3,3,3,3,3,
3,3,3,3,3,3,3,3,3,3,3,3,3,3,3,3,3,3,3,4),(53.4070751113289,53.4997993899176,
53.5924384457477,53.685032722364,53.777609233099,53.8701949680628,53.9628735164002,
54.0556031024292,54.1484802212983,54.2008479071162,54.2950864408842,54.3891971406796,
54.483208556059,54.5771527040731,54.6710626399553,54.7649640134149,54.8588824597985,
54.9529021364258,55.0469773517667,55.1412045950313,55.1959091016198,55.2901555279544,
55.3842501725594,55.4782569490822,55.5721977073362,55.6331177742522),
 .UNSPECIFIED.);
#223=B_SPLINE_CURVE_WITH_KNOTS('',3,(#13330,#13331,#13332,#13333,#13334,
#13335,#13336,#13337,#13338,#13339,#13340,#13341,#13342,#13343,#13344,#13345,
#13346,#13347,#13348,#13349,#13350,#13351,#13352,#13353,#13354,#13355,#13356,
#13357,#13358,#13359,#13360,#13361,#13362,#13363,#13364,#13365,#13366,#13367,
#13368,#13369,#13370,#13371,#13372,#13373,#13374,#13375,#13376,#13377,#13378,
#13379,#13380,#13381,#13382,#13383,#13384,#13385,#13386,#13387,#13388,#13389,
#13390,#13391,#13392,#13393,#13394,#13395,#13396,#13397,#13398,#13399,#13400,
#13401,#13402,#13403,#13404,#13405,#13406,#13407,#13408,#13409,#13410,#13411,
#13412,#13413,#13414,#13415,#13416,#13417,#13418,#13419,#13420,#13421,#13422,
#13423,#13424,#13425,#13426,#13427,#13428,#13429,#13430,#13431,#13432,#13433,
#13434,#13435,#13436,#13437,#13438,#13439,#13440,#13441,#13442,#13443,#13444,
#13445,#13446,#13447,#13448,#13449,#13450,#13451,#13452,#13453,#13454,#13455,
#13456,#13457,#13458,#13459,#13460,#13461,#13462,#13463,#13464,#13465),
 .UNSPECIFIED.,.F.,.F.,(4,3,3,3,3,3,3,3,3,3,3,3,3,3,3,3,3,3,3,3,3,3,3,3,
3,3,3,3,3,3,3,3,3,3,3,3,3,3,3,3,3,3,3,3,3,4),(49.3502511000592,49.4443265486276,
49.5413611211869,49.6352901440451,49.7291940914598,49.8230986056186,49.9170293218311,
50.0110661197233,50.1051666643787,50.1994097924107,50.2206031291018,50.3148416628698,
50.4089523626651,50.5029637780443,50.5969079260583,50.6908178619404,50.7847192353998,
50.8786376817835,50.9726573584107,51.0667325737515,51.1609598170159,51.2156643236054,
51.3099028573735,51.4040135571689,51.4980249725482,51.5919691205624,51.6858790564445,
51.779780429904,51.8736988762878,51.9677185529151,52.061793768256,52.1560210115205,
52.210725518109,52.3049640518771,52.3990747516726,52.493086167052,52.5870303150662,
52.6809402509483,52.7748416244079,52.8687600707917,52.9627797474192,53.05685496276,
53.1510822060246,53.2057867126126,53.3395856335401,53.4070751110264),
 .UNSPECIFIED.);
#224=B_SPLINE_CURVE_WITH_KNOTS('',3,(#13471,#13472,#13473,#13474,#13475,
#13476,#13477,#13478),.UNSPECIFIED.,.F.,.F.,(4,1,1,1,1,4),(43.0672191665734,
43.7009470864233,44.6960082809269,45.6910694754305,46.6861306699341,47.1238898038468),
 .UNSPECIFIED.);
#225=B_SPLINE_CURVE_WITH_KNOTS('',3,(#13479,#13480,#13481,#13482,#13483,
#13484),.UNSPECIFIED.,.F.,.F.,(4,1,1,4),(47.1238898038468,47.6811918644377,
48.6762530589414,49.3489697493475),.UNSPECIFIED.);
#226=B_SPLINE_CURVE_WITH_KNOTS('',3,(#13486,#13487,#13488,#13489,#13490,
#13491,#13492,#13493,#13494,#13495,#13496,#13497,#13498,#13499,#13500,#13501,
#13502,#13503,#13504,#13505,#13506,#13507,#13508,#13509,#13510,#13511,#13512,
#13513,#13514,#13515,#13516,#13517,#13518,#13519,#13520,#13521,#13522,#13523,
#13524,#13525,#13526,#13527,#13528,#13529,#13530,#13531,#13532,#13533,#13534,
#13535,#13536,#13537,#13538,#13539,#13540,#13541,#13542,#13543,#13544,#13545,
#13546,#13547,#13548,#13549,#13550,#13551,#13552,#13553,#13554,#13555,#13556,
#13557,#13558,#13559,#13560,#13561),.UNSPECIFIED.,.F.,.F.,(4,3,3,3,3,3,
3,3,3,3,3,3,3,3,3,3,3,3,3,3,3,3,3,3,3,4),(47.1238898038468,47.235419545591,
47.3296580793584,47.4237687791533,47.5177801945321,47.6117243425455,47.7056342784269,
47.7995356518858,47.8934540982688,47.9874737748954,48.0815489902356,48.1757762334995,
48.2304807400946,48.3247192738626,48.418829973658,48.5128413890372,48.6067855370512,
48.7006954729333,48.7945968463928,48.8885152927764,48.9825349694037,49.0766101847445,
49.1708374280089,49.2255419345982,49.3197803055326,49.3502511000592),
 .UNSPECIFIED.);
#227=B_SPLINE_CURVE_WITH_KNOTS('',3,(#13562,#13563,#13564,#13565,#13566,
#13567,#13568,#13569,#13570,#13571,#13572,#13573,#13574,#13575,#13576,#13577,
#13578,#13579,#13580,#13581,#13582,#13583,#13584,#13585,#13586,#13587,#13588,
#13589,#13590,#13591,#13592,#13593,#13594,#13595,#13596,#13597,#13598,#13599,
#13600,#13601,#13602,#13603,#13604,#13605,#13606,#13607,#13608,#13609,#13610,
#13611,#13612,#13613,#13614,#13615,#13616,#13617,#13618,#13619,#13620,#13621,
#13622,#13623,#13624,#13625,#13626,#13627,#13628,#13629,#13630,#13631,#13632,
#13633,#13634,#13635,#13636,#13637,#13638,#13639,#13640,#13641,#13642,#13643,
#13644,#13645,#13646,#13647,#13648,#13649,#13650,#13651,#13652,#13653,#13654,
#13655,#13656,#13657,#13658,#13659,#13660,#13661,#13662,#13663,#13664,#13665,
#13666,#13667,#13668,#13669,#13670,#13671,#13672,#13673,#13674,#13675,#13676,
#13677,#13678,#13679,#13680,#13681,#13682,#13683,#13684,#13685,#13686,#13687,
#13688,#13689,#13690,#13691,#13692,#13693,#13694,#13695,#13696,#13697),
 .UNSPECIFIED.,.F.,.F.,(4,3,3,3,3,3,3,3,3,3,3,3,3,3,3,3,3,3,3,3,3,3,3,3,
3,3,3,3,3,3,3,3,3,3,3,3,3,3,3,3,3,3,3,3,3,4),(43.0659835124591,43.1605791400178,
43.2551747675765,43.3494133013565,43.4435240011641,43.5375354165557,43.6314795645823,
43.725389500477,43.8192908739492,43.9132093203457,44.0072289969859,44.1013042123396,
44.1955314556169,44.2502359620801,44.3444744958442,44.4385851956356,44.5325966110109,
44.6265407590209,44.720450694899,44.8143520683544,44.908270514734,45.0022901913573,
45.0963654066941,45.1905926499546,45.2452971565837,45.3395356903508,45.4336463901451,
45.5276578055234,45.6216019535364,45.7155118894175,45.8094132628759,45.9033317092585,
45.9973513858848,46.0914266012245,46.1856538444878,46.2403583510873,46.333353832454,
46.4262225404454,46.5189866105434,46.6116939361539,46.7043714684796,46.7970461230593,
46.8897940511829,46.9825825279247,47.0754997300084,47.1238898036263),
 .UNSPECIFIED.);
#228=B_SPLINE_CURVE_WITH_KNOTS('',3,(#13703,#13704,#13705,#13706,#13707,
#13708,#13709,#13710),.UNSPECIFIED.,.F.,.F.,(4,1,1,1,1,4),(36.7836747455901,
37.7305799194016,38.7256411139052,39.7207023084089,40.7157635029125,40.8407044966672),
 .UNSPECIFIED.);
#229=B_SPLINE_CURVE_WITH_KNOTS('',3,(#13711,#13712,#13713,#13714,#13715,
#13716),.UNSPECIFIED.,.F.,.F.,(4,1,1,4),(40.8407044966672,41.7108246974161,
42.7058858919197,43.0672191665734),.UNSPECIFIED.);
#230=B_SPLINE_CURVE_WITH_KNOTS('',3,(#13718,#13719,#13720,#13721,#13722,
#13723,#13724,#13725,#13726,#13727,#13728,#13729,#13730,#13731,#13732,#13733,
#13734,#13735,#13736,#13737,#13738,#13739,#13740,#13741,#13742,#13743,#13744,
#13745,#13746,#13747,#13748,#13749,#13750,#13751,#13752,#13753,#13754,#13755,
#13756,#13757,#13758,#13759,#13760,#13761,#13762,#13763,#13764,#13765,#13766,
#13767,#13768,#13769,#13770,#13771,#13772,#13773,#13774,#13775,#13776,#13777,
#13778,#13779,#13780,#13781,#13782,#13783,#13784,#13785,#13786,#13787,#13788,
#13789,#13790),.UNSPECIFIED.,.F.,.F.,(4,3,3,3,3,3,3,3,3,3,3,3,3,3,3,3,3,
3,3,3,3,3,3,3,4),(40.8407044968377,40.9467914672706,41.0491746663428,41.1571135224561,
41.2650523785693,41.3592909123152,41.4534016120883,41.5474130274451,41.6413571754367,
41.7352671112963,41.8291684847333,41.9230869310945,42.0171066076995,42.111181823018,
42.2054090662605,42.2601135730729,42.3543648080943,42.4484583692329,42.5424618160507,
42.6364009011465,42.7303013150761,42.8242184397312,42.9181432776328,43.0121464883181,
43.0659835124591),.UNSPECIFIED.);
#231=B_SPLINE_CURVE_WITH_KNOTS('',3,(#13791,#13792,#13793,#13794,#13795,
#13796,#13797,#13798,#13799,#13800,#13801,#13802,#13803,#13804,#13805,#13806,
#13807,#13808,#13809,#13810,#13811,#13812,#13813,#13814,#13815,#13816,#13817,
#13818,#13819,#13820,#13821,#13822,#13823,#13824,#13825,#13826,#13827,#13828,
#13829,#13830,#13831,#13832,#13833,#13834,#13835,#13836,#13837,#13838,#13839,
#13840,#13841,#13842,#13843,#13844,#13845,#13846,#13847,#13848,#13849,#13850,
#13851,#13852,#13853,#13854,#13855,#13856,#13857,#13858,#13859,#13860,#13861,
#13862,#13863,#13864,#13865,#13866,#13867,#13868,#13869,#13870,#13871,#13872,
#13873,#13874,#13875,#13876,#13877,#13878,#13879,#13880,#13881,#13882,#13883,
#13884,#13885,#13886,#13887,#13888,#13889,#13890,#13891,#13892,#13893,#13894,
#13895,#13896,#13897,#13898,#13899,#13900,#13901,#13902,#13903,#13904,#13905,
#13906,#13907,#13908,#13909,#13910,#13911,#13912,#13913,#13914,#13915,#13916,
#13917,#13918,#13919,#13920,#13921,#13922,#13923,#13924,#13925,#13926),
 .UNSPECIFIED.,.F.,.F.,(4,3,3,3,3,3,3,3,3,3,3,3,3,3,3,3,3,3,3,3,3,3,3,3,
3,3,3,3,3,3,3,3,3,3,3,3,3,3,3,3,3,3,3,3,3,4),(36.7833917266701,36.8772949592417,
36.971221661623,37.0652530285966,37.1593456853982,37.2535836813732,37.2848076005548,
37.3790461348947,37.4731568352694,37.5671682512346,37.6611123998426,37.755022336323,
37.8489237103847,37.9428421573735,38.036861834607,38.1309370505553,38.2251642944236,
38.2798687950584,38.3741073287149,38.4682180283984,38.5622294436654,38.6561735915675,
38.750083527338,38.843984900686,38.9379033469586,39.0319230234764,39.1259982387085,
39.2202254818661,39.2749299895621,39.3691685232372,39.4632792229378,39.5572906382204,
39.6512347861354,39.7451447219173,39.8390460952754,39.932964541557,40.0269842180808,
40.1210594333172,40.2152866764772,40.2699911840657,40.3663474040655,40.4625550535571,
40.5586031869615,40.6545575386078,40.7504306626063,40.8407044966672),
 .UNSPECIFIED.);
#232=B_SPLINE_CURVE_WITH_KNOTS('',3,(#13932,#13933,#13934,#13935,#13936,
#13937,#13938,#13939),.UNSPECIFIED.,.F.,.F.,(4,1,1,1,1,4),(30.4993075292779,
30.7651515578764,31.76021275238,32.7552739468836,33.7503351413872,34.5575191894876),
 .UNSPECIFIED.);
#233=B_SPLINE_CURVE_WITH_KNOTS('',3,(#13940,#13941,#13942,#13943,#13944,
#13945,#13946),.UNSPECIFIED.,.F.,.F.,(4,1,1,1,4),(34.5575191894876,34.7453963358908,
35.7404575303944,36.735518724898,36.7836747455901),.UNSPECIFIED.);
#234=B_SPLINE_CURVE_WITH_KNOTS('',3,(#13948,#13949,#13950,#13951,#13952,
#13953,#13954,#13955,#13956,#13957,#13958,#13959,#13960,#13961,#13962,#13963,
#13964,#13965,#13966,#13967,#13968,#13969,#13970,#13971,#13972,#13973,#13974,
#13975,#13976,#13977,#13978,#13979,#13980,#13981,#13982,#13983,#13984,#13985,
#13986,#13987,#13988,#13989,#13990,#13991,#13992,#13993,#13994,#13995,#13996,
#13997,#13998,#13999,#14000,#14001,#14002,#14003,#14004,#14005,#14006,#14007,
#14008,#14009,#14010,#14011,#14012,#14013,#14014,#14015,#14016,#14017,#14018,
#14019,#14020,#14021,#14022,#14023),.UNSPECIFIED.,.F.,.F.,(4,3,3,3,3,3,
3,3,3,3,3,3,3,3,3,3,3,3,3,3,3,3,3,3,3,4),(34.5575191894876,34.650507384765,
34.7434447378057,34.8363579762665,34.9292737992236,35.0222802874223,35.1153312645007,
35.208542165953,35.2946852115476,35.3889237448561,35.4830344441946,35.5770458591202,
35.6709900066873,35.7648999421268,35.8588013151486,35.9527197611,36.0467394373063,
36.1408146522315,36.2350418950937,36.2897464060512,36.3839854254529,36.4781010625499,
36.572104614555,36.6660439246588,36.7599457437182,36.7833917266701),
 .UNSPECIFIED.);
#235=B_SPLINE_CURVE_WITH_KNOTS('',3,(#14024,#14025,#14026,#14027,#14028,
#14029,#14030,#14031,#14032,#14033,#14034,#14035,#14036,#14037,#14038,#14039,
#14040,#14041,#14042,#14043,#14044,#14045,#14046,#14047,#14048,#14049,#14050,
#14051,#14052,#14053,#14054,#14055,#14056,#14057,#14058,#14059,#14060,#14061,
#14062,#14063,#14064,#14065,#14066,#14067,#14068,#14069,#14070,#14071,#14072,
#14073,#14074,#14075,#14076,#14077,#14078,#14079,#14080,#14081,#14082,#14083,
#14084,#14085,#14086,#14087,#14088,#14089,#14090,#14091,#14092,#14093,#14094,
#14095,#14096,#14097,#14098,#14099,#14100,#14101,#14102,#14103,#14104,#14105,
#14106,#14107,#14108,#14109,#14110,#14111,#14112,#14113,#14114,#14115,#14116,
#14117,#14118,#14119,#14120,#14121,#14122,#14123,#14124,#14125,#14126,#14127,
#14128,#14129,#14130,#14131,#14132,#14133,#14134,#14135,#14136,#14137,#14138,
#14139,#14140,#14141,#14142,#14143,#14144,#14145,#14146,#14147,#14148,#14149,
#14150,#14151,#14152,#14153,#14154,#14155,#14156,#14157,#14158,#14159),
 .UNSPECIFIED.,.F.,.F.,(4,3,3,3,3,3,3,3,3,3,3,3,3,3,3,3,3,3,3,3,3,3,3,3,
3,3,3,3,3,3,3,3,3,3,3,3,3,3,3,3,3,3,3,3,3,4),(30.5007718328711,30.5947895666449,
30.6887372141556,30.7826487508107,30.8765498282776,30.9704660823069,31.0644825169794,
31.1585527858859,31.2527771290475,31.3144404335332,31.408678991978,31.5027897167387,
31.5968011573355,31.6907453308385,31.7846552923679,31.8785566916019,31.9724751638558,
32.0664948663422,32.1605701075741,32.2547973765244,32.3095016280368,32.4037401608989,
32.4978508598401,32.591862274418,32.6858064217136,32.7797163569288,32.8736177297741,
32.9675361755972,33.0615558517501,33.1556310666643,33.2498583095829,33.3045628225404,
33.3988013500615,33.4929120435014,33.5869234524259,33.6808675938635,33.7747775230965,
33.868678889842,33.9625973294547,34.0566169992651,34.1506922077529,34.2449194441747,
34.299624017044,34.4208944647328,34.5397648462028,34.5575191891919),
 .UNSPECIFIED.);
#236=B_SPLINE_CURVE_WITH_KNOTS('',3,(#14165,#14166,#14167,#14168,#14169,
#14170,#14171,#14172),.UNSPECIFIED.,.F.,.F.,(4,1,1,1,1,4),(24.2174208605652,
24.7947843908547,25.7898455853583,26.7849067798619,27.7799679743655,28.274333882308),
 .UNSPECIFIED.);
#237=B_SPLINE_CURVE_WITH_KNOTS('',3,(#14173,#14174,#14175,#14176,#14177,
#14178),.UNSPECIFIED.,.F.,.F.,(4,1,1,4),(28.274333882308,28.7750291688691,
29.7700903633727,30.4993075292779),.UNSPECIFIED.);
#238=B_SPLINE_CURVE_WITH_KNOTS('',3,(#14180,#14181,#14182,#14183,#14184,
#14185,#14186,#14187,#14188,#14189,#14190,#14191,#14192,#14193,#14194,#14195,
#14196,#14197,#14198,#14199,#14200,#14201,#14202,#14203,#14204,#14205,#14206,
#14207,#14208,#14209,#14210,#14211,#14212,#14213,#14214,#14215,#14216,#14217,
#14218,#14219,#14220,#14221,#14222,#14223,#14224,#14225,#14226,#14227,#14228,
#14229,#14230,#14231,#14232,#14233,#14234,#14235,#14236,#14237,#14238,#14239,
#14240,#14241,#14242,#14243,#14244,#14245,#14246,#14247,#14248,#14249,#14250,
#14251,#14252,#14253,#14254,#14255),.UNSPECIFIED.,.F.,.F.,(4,3,3,3,3,3,
3,3,3,3,3,3,3,3,3,3,3,3,3,3,3,3,3,3,3,4),(28.274333882308,28.3292568500223,
28.4234955385194,28.5176063946983,28.6116179678894,28.7055622751876,28.7994723712053,
28.8933739054553,28.9872925130887,29.0813123506841,29.1753877270723,29.2696151299171,
29.3243180445259,29.4185565881387,29.5126672983678,29.6066787247526,29.7006228845845,
29.7945328327832,29.8884342190449,29.9823526787031,30.0763723692509,30.1704475988978,
30.2646748569405,30.3193792390296,30.4135944693525,30.5007718328711),
 .UNSPECIFIED.);
#239=B_SPLINE_CURVE_WITH_KNOTS('',3,(#14256,#14257,#14258,#14259,#14260,
#14261,#14262,#14263,#14264,#14265,#14266,#14267,#14268,#14269,#14270,#14271,
#14272,#14273,#14274,#14275,#14276,#14277,#14278,#14279,#14280,#14281,#14282,
#14283,#14284,#14285,#14286,#14287,#14288,#14289,#14290,#14291,#14292,#14293,
#14294,#14295,#14296,#14297,#14298,#14299,#14300,#14301,#14302,#14303,#14304,
#14305,#14306,#14307,#14308,#14309,#14310,#14311,#14312,#14313,#14314,#14315,
#14316,#14317,#14318,#14319,#14320,#14321,#14322,#14323,#14324,#14325,#14326,
#14327,#14328,#14329,#14330,#14331,#14332,#14333,#14334,#14335,#14336,#14337,
#14338,#14339,#14340,#14341,#14342,#14343,#14344,#14345,#14346,#14347,#14348,
#14349,#14350,#14351,#14352,#14353,#14354,#14355,#14356,#14357,#14358,#14359,
#14360,#14361,#14362,#14363,#14364,#14365,#14366,#14367,#14368,#14369,#14370,
#14371,#14372,#14373,#14374,#14375,#14376,#14377,#14378,#14379,#14380,#14381,
#14382,#14383,#14384,#14385,#14386,#14387,#14388,#14389,#14390,#14391),
 .UNSPECIFIED.,.F.,.F.,(4,3,3,3,3,3,3,3,3,3,3,3,3,3,3,3,3,3,3,3,3,3,3,3,
3,3,3,3,3,3,3,3,3,3,3,3,3,3,3,3,3,3,3,3,3,4),(24.2164936820193,24.3107305689308,
24.3490120720079,24.4432480127433,24.53735608089,24.6313648298541,24.7253062705863,
24.8192134748993,24.9131120958114,25.0070277719615,25.1010446681085,25.1951170930602,
25.2893415577707,25.3440732665115,25.4383127320977,25.5324243724796,25.6264367358588,
25.720381838964,25.8142927339653,25.908195069392,26.0021144794129,26.0961351163385,
26.1902112915144,26.2844394843798,26.3391344610151,26.4333731743329,26.5274840592679,
26.6214956650936,26.7154400107166,26.8093501485702,26.903251728129,26.9971703845084,
27.0911902758432,27.185265708871,27.2794931724116,27.3341956555187,27.4276602318839,
27.5209976121009,27.6151646458553,27.7083392261065,27.8014829430723,27.8946222986052,
27.9895501944879,28.0828111807321,28.1785725314341,28.2743338821362),
 .UNSPECIFIED.);
#240=B_SPLINE_CURVE_WITH_KNOTS('',3,(#14397,#14398,#14399,#14400,#14401,
#14402,#14403,#14404,#14405,#14406,#14407,#14408,#14409,#14410,#14411,#14412,
#14413,#14414,#14415,#14416,#14417,#14418,#14419,#14420,#14421,#14422,#14423,
#14424,#14425,#14426,#14427,#14428,#14429,#14430,#14431,#14432,#14433,#14434,
#14435,#14436,#14437,#14438,#14439,#14440,#14441,#14442,#14443,#14444,#14445,
#14446,#14447,#14448,#14449,#14450,#14451,#14452,#14453,#14454,#14455,#14456,
#14457,#14458,#14459,#14460,#14461,#14462,#14463,#14464,#14465,#14466,#14467,
#14468,#14469,#14470,#14471,#14472),.UNSPECIFIED.,.F.,.F.,(4,3,3,3,3,3,
3,3,3,3,3,3,3,3,3,3,3,3,3,3,3,3,3,3,3,4),(15.7079632679489,15.8007859309492,
15.8935795723414,15.9863709089602,16.0791866498076,16.1721111225518,16.2650994944724,
16.3582389121077,16.388522515979,16.4829033285741,16.5771564891806,16.6713103389117,
16.7653962546427,16.8594474840588,16.9534894914163,17.0475477260245,17.141705019005,
17.2359168213297,17.3302776617067,17.3835837104826,17.4779774291156,17.5722520765761,
17.6664233060793,17.7605330002792,17.854621932,17.9336209525117),
 .UNSPECIFIED.);
#241=B_SPLINE_CURVE_WITH_KNOTS('',3,(#14474,#14475,#14476,#14477,#14478),
 .UNSPECIFIED.,.F.,.F.,(4,1,4),(14.3984001269718,15.3934613214754,15.7079548348344),
 .UNSPECIFIED.);
#242=B_SPLINE_CURVE_WITH_KNOTS('',3,(#14482,#14483,#14484,#14485,#14486,
#14487,#14488,#14489,#14490,#14491,#14492,#14493,#14494,#14495,#14496,#14497,
#14498,#14499,#14500,#14501,#14502,#14503,#14504,#14505,#14506,#14507,#14508,
#14509,#14510,#14511,#14512,#14513,#14514,#14515,#14516,#14517,#14518,#14519,
#14520,#14521,#14522,#14523,#14524,#14525,#14526,#14527,#14528,#14529,#14530,
#14531,#14532,#14533,#14534,#14535,#14536,#14537,#14538,#14539,#14540,#14541,
#14542,#14543,#14544,#14545),.UNSPECIFIED.,.F.,.F.,(4,3,3,3,3,3,3,3,3,3,
3,3,3,3,3,3,3,3,3,3,3,4),(13.8759338288966,13.9698681094706,14.063675502176,
14.1612376201314,14.2548798577636,14.3484908494825,14.4420966018558,14.5357231098688,
14.6294501266586,14.7232367530041,14.8171644342521,14.8441724458186,14.9372022831589,
15.0335474062577,15.1263493200002,15.2190977781909,15.3118197005127,15.4045419742366,
15.4973366037527,15.590174778641,15.6831317332385,15.7079632679489),
 .UNSPECIFIED.);
#243=B_SPLINE_CURVE_WITH_KNOTS('',3,(#14546,#14547,#14548,#14549,#14550,
#14551,#14552),.UNSPECIFIED.,.F.,.F.,(4,1,1,1,4),(15.7079632679489,15.8392336403222,
16.8342948348258,17.8293560293294,17.9344061060102),.UNSPECIFIED.);
#244=B_SPLINE_CURVE_WITH_KNOTS('',3,(#14558,#14559,#14560,#14561,#14562,
#14563,#14564,#14565,#14566,#14567,#14568,#14569),.UNSPECIFIED.,.F.,.F.,
(4,2,2,2,2,4),(-0.0891720069757108,-0.0494869050463887,-0.0101787320937009,
-0.00433426661833915,-0.00195064461630957,0.),.UNSPECIFIED.);
#245=B_SPLINE_CURVE_WITH_KNOTS('',3,(#14577,#14578,#14579,#14580,#14581,
#14582,#14583,#14584,#14585,#14586,#14587,#14588,#14589,#14590,#14591,#14592,
#14593,#14594,#14595,#14596,#14597,#14598,#14599,#14600,#14601,#14602,#14603,
#14604,#14605,#14606,#14607,#14608,#14609,#14610,#14611,#14612,#14613,#14614,
#14615,#14616,#14617,#14618,#14619,#14620,#14621,#14622,#14623,#14624,#14625,
#14626,#14627,#14628,#14629,#14630,#14631,#14632,#14633,#14634,#14635,#14636,
#14637,#14638,#14639,#14640,#14641,#14642,#14643),.UNSPECIFIED.,.F.,.F.,
(4,3,3,3,3,3,3,3,3,3,3,3,3,3,3,3,3,3,3,3,3,3,4),(-119.380510462334,-119.281771177695,
-119.183171276094,-119.084683219952,-118.98625595986,-118.88785925611,-118.789462906781,
-118.690971819416,-118.592433148612,-118.493725456286,-118.41228214593,
-118.313053489152,-118.213961788152,-118.114369183561,-118.015446937852,
-117.916554860053,-117.817663412407,-117.717552797162,-117.618516407178,
-117.517868679302,-117.417220951426,-117.311998815212,-117.299669606592),
 .UNSPECIFIED.);
#246=B_SPLINE_CURVE_WITH_KNOTS('',3,(#14649,#14650,#14651,#14652,#14653,
#14654,#14655,#14656,#14657,#14658,#14659,#14660,#14661,#14662,#14663,#14664,
#14665,#14666,#14667,#14668,#14669,#14670,#14671,#14672,#14673,#14674,#14675,
#14676,#14677,#14678,#14679,#14680,#14681,#14682,#14683,#14684,#14685,#14686,
#14687,#14688,#14689,#14690,#14691,#14692,#14693,#14694,#14695,#14696,#14697,
#14698,#14699,#14700,#14701,#14702,#14703,#14704,#14705,#14706,#14707,#14708,
#14709,#14710,#14711,#14712,#14713,#14714,#14715,#14716,#14717,#14718,#14719,
#14720,#14721,#14722,#14723,#14724,#14725,#14726,#14727,#14728,#14729,#14730,
#14731,#14732,#14733,#14734,#14735,#14736,#14737,#14738,#14739,#14740,#14741,
#14742,#14743,#14744,#14745,#14746,#14747,#14748,#14749,#14750,#14751,#14752,
#14753,#14754,#14755,#14756,#14757,#14758,#14759,#14760,#14761,#14762,#14763,
#14764,#14765,#14766,#14767,#14768,#14769,#14770,#14771,#14772,#14773,#14774,
#14775,#14776,#14777,#14778,#14779,#14780,#14781,#14782,#14783,#14784,#14785,
#14786,#14787,#14788,#14789,#14790,#14791,#14792,#14793,#14794,#14795,#14796,
#14797,#14798,#14799,#14800,#14801,#14802,#14803,#14804,#14805,#14806,#14807,
#14808,#14809,#14810,#14811,#14812,#14813,#14814,#14815,#14816,#14817,#14818,
#14819,#14820,#14821,#14822,#14823,#14824,#14825,#14826,#14827,#14828,#14829,
#14830,#14831,#14832),.UNSPECIFIED.,.F.,.F.,(4,3,3,3,3,3,3,3,3,3,3,3,3,
3,3,3,3,3,3,3,3,3,3,3,3,3,3,3,3,3,3,3,3,3,3,3,3,3,3,3,3,3,3,3,3,3,3,3,3,
3,3,3,3,3,3,3,3,3,3,3,3,4),(114.761330096248,114.860080090372,114.958806946108,
115.057540414678,115.156375577384,115.255263663134,115.354321468029,115.427098562419,
115.526186136662,115.625133609413,115.724761877852,115.823533291856,115.922272394729,
116.021008931117,116.121296637569,116.220174922379,116.321167339651,116.422159756923,
116.521079048506,116.619857573038,116.719527995337,116.818130058757,116.916700027885,
117.015267869772,117.115756140185,117.214468515351,117.315844733388,117.417220951426,
117.516468414644,117.615574873252,117.715163282337,117.814090335468,117.91298347636,
118.011872245612,118.111974720691,118.210999270349,118.311640708139,118.41228214593,
118.51148086908,118.610541479571,118.710141712178,118.809030190265,118.907887549976,
119.006743360195,119.106893355254,119.205892130244,119.306617735339,119.407343340433,
119.505333524646,119.60318256861,119.703085314401,119.800762950198,119.89841208206,
119.996063705263,120.097648912682,120.195465284113,120.293361575936,120.391426373293,
120.402404534937,120.534601350672,120.663480247902,120.690073491388),
 .UNSPECIFIED.);
#247=B_SPLINE_CURVE_WITH_KNOTS('',3,(#14833,#14834,#14835,#14836,#14837,
#14838,#14839,#14840,#14841,#14842,#14843,#14844,#14845,#14846,#14847,#14848,
#14849,#14850,#14851,#14852),.UNSPECIFIED.,.F.,.F.,(4,2,2,2,2,2,2,2,2,4),
(-0.178823947996459,-0.142362827283928,-0.126740729259348,-0.12110726670276,
-0.117062474690017,-0.113022490578283,-0.109070108678785,-0.103377303050124,
-0.0894510093045505,-0.0891720069757108),.UNSPECIFIED.);
#248=B_SPLINE_CURVE_WITH_KNOTS('',3,(#14854,#14855,#14856,#14857,#14858,
#14859,#14860,#14861,#14862,#14863,#14864,#14865,#14866),.UNSPECIFIED.,
 .F.,.F.,(4,3,3,3,4),(-117.299669606592,-117.194805922057,-117.090145972068,
-116.985755035457,-116.946309935109),.UNSPECIFIED.);
#249=B_SPLINE_CURVE_WITH_KNOTS('',3,(#14867,#14868,#14869,#14870,#14871,
#14872,#14873,#14874,#14875,#14876,#14877,#14878,#14879,#14880,#14881,#14882,
#14883,#14884,#14885,#14886,#14887,#14888,#14889,#14890,#14891,#14892,#14893,
#14894,#14895,#14896,#14897,#14898,#14899,#14900,#14901,#14902,#14903,#14904,
#14905,#14906,#14907,#14908,#14909,#14910,#14911,#14912,#14913,#14914,#14915,
#14916,#14917,#14918,#14919,#14920,#14921,#14922,#14923,#14924,#14925,#14926,
#14927,#14928,#14929,#14930,#14931,#14932,#14933,#14934,#14935,#14936,#14937,
#14938,#14939,#14940,#14941,#14942,#14943,#14944,#14945,#14946,#14947,#14948,
#14949,#14950,#14951,#14952,#14953,#14954,#14955,#14956,#14957,#14958,#14959,
#14960,#14961,#14962,#14963,#14964,#14965,#14966,#14967,#14968,#14969,#14970,
#14971,#14972,#14973,#14974,#14975,#14976,#14977,#14978,#14979,#14980,#14981,
#14982,#14983,#14984,#14985,#14986,#14987,#14988,#14989,#14990,#14991,#14992,
#14993,#14994,#14995,#14996,#14997,#14998,#14999,#15000,#15001,#15002,#15003,
#15004,#15005,#15006,#15007,#15008,#15009,#15010,#15011,#15012,#15013,#15014,
#15015,#15016,#15017,#15018,#15019,#15020,#15021,#15022,#15023,#15024,#15025,
#15026,#15027,#15028,#15029,#15030,#15031,#15032,#15033,#15034,#15035,#15036,
#15037,#15038,#15039,#15040,#15041,#15042,#15043,#15044,#15045,#15046,#15047,
#15048,#15049,#15050,#15051,#15052,#15053,#15054,#15055,#15056,#15057,#15058,
#15059,#15060,#15061,#15062,#15063,#15064,#15065,#15066),.UNSPECIFIED.,
 .F.,.F.,(4,2,2,2,2,2,2,2,2,2,2,2,2,2,2,2,2,2,2,2,2,2,2,2,2,2,2,2,2,2,2,
2,2,2,2,2,2,2,2,2,2,2,2,2,2,2,2,2,2,2,2,2,2,2,2,2,2,2,2,2,2,2,2,2,2,2,2,
2,2,2,2,2,2,2,2,2,2,2,2,2,2,2,2,2,2,2,2,2,2,2,2,2,2,2,2,2,2,2,2,4),(-3.17306480281887,
-3.17031484000139,-3.16702949099971,-3.16357845900456,-3.15898974631456,
-3.14908917358974,-3.13871904583365,-3.09338330631132,-3.0497559080526,
-3.04427467983949,-3.04173163639629,-3.03977609528626,-3.03749715605209,
-3.03349583520392,-3.01607623423926,-2.97206449120236,-2.92764725149413,
-2.92031574423137,-2.91629008485033,-2.91286552807971,-2.90879756401509,
-2.9015209743123,-2.85317700352524,-2.81612752193056,-2.80290955054846,
-2.79449102094127,-2.79145426303676,-2.78940447377351,-2.78756203924621,
-2.78502055221003,-2.77854920780034,-2.73999230460291,-2.69688096552749,
-2.67476879138662,-2.66859810618169,-2.66476788008122,-2.6612413129484,
-2.6566883864451,-2.64673342784875,-2.59498225700094,-2.56534414342733,
-2.55179741996168,-2.54323388281634,-2.54018590528232,-2.53814045860138,
-2.53630787075916,-2.53330764179099,-2.52568548954152,-2.47396426601489,
-2.42723505989897,-2.41889428352826,-2.41460669782412,-2.41112133712132,
-2.4070986672778,-2.40021003083625,-2.37040805697371,-2.31979073887641,
-2.30251506025713,-2.29567342382265,-2.29054405344137,-2.28805763546822,
-2.28628746235987,-2.28403114102655,-2.28012678810709,-2.26409276851681,
-2.19920558313719,-2.18168302415323,-2.16947559351126,-2.16448973953458,
-2.16090520542717,-2.15763752132235,-2.15324369428735,-2.14465257285608,
-2.08549010643853,-2.04487905252895,-2.03946046521272,-2.0369158830879,
-2.03495208127562,-2.03265822773036,-2.02858893341875,-2.01006858852172,
-1.95649051486607,-1.9223662483841,-1.91540697721669,-1.91140662811411,
-1.90791571821389,-1.90358913525673,-1.89690266429737,-1.84827039965294,
-1.81100662114177,-1.79781730636118,-1.78941752718114,-1.78639195533164,
-1.78435109299796,-1.78251336957195,-1.77998086993912,-1.77354403440157,
-1.73236136865648,-1.69256242796197,-1.67593543967424),.UNSPECIFIED.);
#250=B_SPLINE_CURVE_WITH_KNOTS('',3,(#15072,#15073,#15074,#15075,#15076,
#15077,#15078,#15079,#15080,#15081,#15082,#15083,#15084,#15085,#15086,#15087,
#15088,#15089,#15090,#15091,#15092,#15093,#15094,#15095,#15096,#15097,#15098,
#15099,#15100,#15101,#15102,#15103,#15104,#15105,#15106,#15107,#15108,#15109,
#15110,#15111,#15112,#15113,#15114,#15115,#15116,#15117,#15118,#15119,#15120,
#15121,#15122,#15123,#15124,#15125,#15126,#15127,#15128,#15129,#15130,#15131,
#15132,#15133,#15134,#15135,#15136,#15137,#15138,#15139,#15140,#15141,#15142,
#15143,#15144,#15145,#15146,#15147,#15148,#15149,#15150,#15151,#15152,#15153,
#15154,#15155,#15156,#15157,#15158,#15159,#15160,#15161,#15162,#15163,#15164,
#15165,#15166,#15167,#15168,#15169,#15170,#15171,#15172,#15173,#15174,#15175,
#15176,#15177,#15178,#15179,#15180,#15181,#15182,#15183,#15184,#15185,#15186,
#15187,#15188,#15189,#15190,#15191,#15192,#15193,#15194,#15195,#15196,#15197,
#15198,#15199,#15200,#15201,#15202,#15203,#15204,#15205,#15206,#15207,#15208,
#15209,#15210,#15211,#15212,#15213,#15214,#15215,#15216,#15217,#15218,#15219,
#15220,#15221,#15222,#15223,#15224,#15225,#15226,#15227,#15228,#15229,#15230,
#15231,#15232,#15233,#15234,#15235,#15236,#15237,#15238,#15239,#15240,#15241,
#15242,#15243,#15244,#15245,#15246,#15247,#15248,#15249,#15250,#15251,#15252),
 .UNSPECIFIED.,.F.,.F.,(4,3,3,3,3,3,3,3,3,3,3,3,3,3,3,3,3,3,3,3,3,3,3,3,
3,3,3,3,3,3,3,3,3,3,3,3,3,3,3,3,3,3,3,3,3,3,3,3,3,3,3,3,3,3,3,3,3,3,3,3,
4),(108.477780689588,108.5768149494,108.675714162024,108.774507135944,108.873242407719,
108.971949794152,109.070659077164,109.169467502809,109.268324650162,109.367357262576,
109.456731395397,109.555791506682,109.654711181245,109.754346357327,109.853089367671,
109.951799904424,110.050507752022,110.150828961492,110.249678553296,110.350735571598,
110.451792589901,110.550848797479,110.649764558671,110.749400711888,110.848139813769,
110.946846452491,111.045550417668,111.145876259352,111.244722046462,111.345787915433,
111.446853784404,111.545915329689,111.644836413925,111.744471234548,111.84321558588,
111.941927435112,112.040636565101,112.140956168553,112.239806956383,112.340860967646,
112.441914978908,112.540979666107,112.639903958053,112.739537984973,112.838285679204,
112.937000914266,113.035713468157,113.136029144471,113.234883413822,113.335929793617,
113.436976173412,113.535600535162,113.634084744862,113.732456535692,113.830767187538,
113.929047085794,114.027326577713,114.125701961597,114.224125092387,114.322720068555,
114.406898669989),.UNSPECIFIED.);
#251=B_SPLINE_CURVE_WITH_KNOTS('',3,(#15253,#15254,#15255,#15256,#15257,
#15258,#15259,#15260,#15261,#15262,#15263,#15264,#15265,#15266,#15267,#15268),
 .UNSPECIFIED.,.F.,.F.,(4,3,3,3,3,4),(114.40689867021,114.432037367915,
114.531100262932,114.630039899472,114.728867567748,114.761330096248),
 .UNSPECIFIED.);
#252=B_SPLINE_CURVE_WITH_KNOTS('',3,(#15269,#15270,#15271,#15272,#15273,
#15274,#15275,#15276,#15277,#15278,#15279,#15280,#15281,#15282,#15283,#15284,
#15285,#15286,#15287,#15288,#15289,#15290,#15291,#15292,#15293,#15294,#15295,
#15296,#15297,#15298,#15299,#15300,#15301,#15302,#15303,#15304,#15305,#15306,
#15307,#15308,#15309,#15310,#15311,#15312,#15313,#15314,#15315,#15316,#15317,
#15318,#15319,#15320,#15321,#15322,#15323,#15324,#15325,#15326,#15327,#15328,
#15329,#15330,#15331,#15332,#15333,#15334,#15335,#15336,#15337,#15338,#15339,
#15340,#15341,#15342,#15343,#15344,#15345,#15346,#15347,#15348,#15349,#15350,
#15351,#15352,#15353,#15354,#15355,#15356,#15357,#15358,#15359,#15360,#15361,
#15362,#15363,#15364,#15365,#15366,#15367,#15368,#15369,#15370,#15371,#15372,
#15373,#15374,#15375,#15376,#15377,#15378,#15379,#15380,#15381,#15382,#15383,
#15384,#15385,#15386,#15387,#15388,#15389,#15390,#15391,#15392,#15393,#15394,
#15395,#15396,#15397,#15398,#15399,#15400,#15401,#15402,#15403,#15404,#15405,
#15406,#15407,#15408,#15409,#15410,#15411,#15412,#15413,#15414,#15415,#15416,
#15417,#15418,#15419,#15420,#15421,#15422,#15423,#15424,#15425,#15426,#15427,
#15428,#15429,#15430,#15431,#15432,#15433,#15434,#15435,#15436,#15437,#15438,
#15439,#15440,#15441,#15442,#15443,#15444,#15445,#15446,#15447,#15448,#15449,
#15450,#15451,#15452,#15453,#15454,#15455,#15456,#15457,#15458,#15459,#15460,
#15461,#15462,#15463,#15464,#15465,#15466,#15467,#15468,#15469,#15470,#15471,
#15472,#15473,#15474,#15475,#15476,#15477,#15478,#15479,#15480,#15481,#15482,
#15483,#15484,#15485,#15486,#15487,#15488,#15489,#15490,#15491,#15492,#15493,
#15494,#15495,#15496,#15497,#15498,#15499,#15500,#15501,#15502,#15503,#15504,
#15505,#15506,#15507,#15508,#15509,#15510,#15511,#15512,#15513,#15514,#15515,
#15516,#15517,#15518,#15519,#15520,#15521,#15522,#15523,#15524,#15525,#15526,
#15527,#15528,#15529,#15530,#15531,#15532,#15533,#15534),.UNSPECIFIED.,
 .F.,.F.,(4,2,2,2,2,2,2,2,2,2,2,2,2,2,2,2,2,2,2,2,2,2,2,2,2,2,2,2,2,2,2,
2,2,2,2,2,2,2,2,2,2,2,2,2,2,2,2,2,2,2,2,2,2,2,2,2,2,2,2,2,2,2,2,2,2,2,2,
2,2,2,2,2,2,2,2,2,2,2,2,2,2,2,2,2,2,2,2,2,2,2,2,2,2,2,2,2,2,2,2,2,2,2,2,
2,2,2,2,2,2,2,2,2,2,2,2,2,2,2,2,2,2,2,2,2,2,2,2,2,2,2,2,2,4),(-1.67593543967424,
-1.66977071673315,-1.66354338195487,-1.65970269687102,-1.6561828918038,
-1.65166153531714,-1.64186898951177,-1.58634824894007,-1.54408962606901,
-1.53768435112349,-1.53515704690784,-1.53332059773318,-1.53127792378963,
-1.52824448468582,-1.51978946372215,-1.5064782730895,-1.46932156034882,
-1.42074022860206,-1.4140535538658,-1.40972678469582,-1.40623565313944,
-1.40223496659467,-1.39527486134847,-1.36113297586233,-1.33008289262082,
-1.311897933727,-1.28951619754529,-1.28561070249212,-1.28314763875336,-1.28119020106764,
-1.27883569814171,-1.274365456639,-1.24122551170778,-1.18894101047551,-1.16756528212953,
-1.16123706487441,-1.15737414235223,-1.15385999665028,-1.14930622145439,
-1.13960488170706,-1.10006900335747,-1.05784774183277,-1.03808274275315,
-1.03394194019783,-1.03163233178748,-1.02986816179068,-1.02745127240965,
-1.02267768203832,-0.980115772537609,-0.921927856483065,-0.912301497716021,
-0.907810551833117,-0.904294918827611,-0.900438921298833,-0.894141611983562,
-0.870516464371559,-0.828011912858863,-0.810533582686724,-0.803829989198249,
-0.786620077210319,-0.782634748517623,-0.780360453081858,-0.778592386597329,
-0.776130388602689,-0.771131501835579,-0.730658552018725,-0.670477574292303,
-0.661027362715015,-0.656520968644825,-0.653013057915604,-0.649126210953403,
-0.642687022142984,-0.617248156183727,-0.587319819794684,-0.538998674496578,
-0.532837592146501,-0.530351753654805,-0.528344334310793,-0.526245201980107,
-0.522947702781798,-0.512354900195278,-0.493979030775597,-0.437748537043523,
-0.414389473105762,-0.407868567874907,-0.403964070590822,-0.400460178951072,
-0.395986550410335,-0.386707768108472,-0.350631073872998,-0.322597152601837,
-0.285219816526485,-0.281097498216689,-0.278570049382816,-0.27660911752628,
-0.276597237604701,-0.276585878671202,-0.276575017380847,-0.276562679594506,
-0.276550465228692,-0.276538372722027,-0.276526400552761,-0.276514547213202,
-0.276502811223774,-0.276491191118132,-0.27647968545302,-0.276468292803317,
-0.276457011765121,-0.276445840955162,-0.276434779009765,-0.276423824572702,
-0.276412976324931,-0.276402232954849,-0.276391593166715,-0.276381055688099,
-0.276370619265946,-0.276360282659443,-0.276350044652056,-0.276339904043702,
-0.276329859643788,-0.276319910288696,-0.276310054812429,-0.273939459509603,
-0.269266499659848,-0.263130102235049,-0.200228930266931,-0.164576114030874,
-0.157409452806997,-0.153322721388574,-0.149872398915665,-0.145672531750551,
-0.137766863027111,-0.0898945060156978),.UNSPECIFIED.);
#253=B_SPLINE_CURVE_WITH_KNOTS('',3,(#15540,#15541,#15542,#15543,#15544,
#15545,#15546,#15547,#15548,#15549,#15550,#15551,#15552,#15553,#15554,#15555,
#15556,#15557,#15558,#15559,#15560,#15561,#15562,#15563,#15564,#15565,#15566,
#15567,#15568,#15569,#15570,#15571,#15572,#15573,#15574,#15575,#15576,#15577,
#15578,#15579,#15580,#15581,#15582,#15583,#15584,#15585,#15586,#15587,#15588,
#15589,#15590,#15591,#15592,#15593,#15594,#15595,#15596,#15597,#15598,#15599,
#15600,#15601,#15602,#15603,#15604,#15605,#15606,#15607,#15608,#15609,#15610,
#15611,#15612,#15613,#15614,#15615,#15616,#15617,#15618,#15619,#15620,#15621,
#15622,#15623,#15624,#15625,#15626,#15627,#15628,#15629,#15630,#15631,#15632,
#15633,#15634,#15635,#15636,#15637,#15638,#15639,#15640,#15641,#15642,#15643,
#15644,#15645,#15646,#15647,#15648,#15649,#15650,#15651,#15652,#15653,#15654,
#15655,#15656,#15657,#15658,#15659,#15660,#15661,#15662,#15663,#15664,#15665,
#15666,#15667,#15668,#15669,#15670,#15671,#15672,#15673,#15674,#15675,#15676,
#15677,#15678,#15679,#15680,#15681,#15682,#15683,#15684,#15685,#15686,#15687,
#15688,#15689,#15690,#15691,#15692,#15693,#15694,#15695,#15696,#15697,#15698,
#15699,#15700,#15701,#15702,#15703,#15704,#15705,#15706,#15707,#15708,#15709,
#15710,#15711,#15712,#15713,#15714,#15715,#15716,#15717,#15718,#15719,#15720),
 .UNSPECIFIED.,.F.,.F.,(4,3,3,3,3,3,3,3,3,3,3,3,3,3,3,3,3,3,3,3,3,3,3,3,
3,3,3,3,3,3,3,3,3,3,3,3,3,3,3,3,3,3,3,3,3,3,3,3,3,3,3,3,3,3,3,3,3,3,3,3,
4),(102.194035073172,102.293066856479,102.392288804316,102.491303033872,
102.590362151105,102.689280824941,102.788916250371,102.88765825113,102.986367777226,
103.085074614465,103.185397017943,103.28424561045,103.385304919413,103.486364228376,
103.585423372849,103.68434207411,103.783977492706,103.88271952114,103.981429074944,
104.080135939883,104.180458310632,104.279306930543,104.380366176711,104.481425422879,
104.580484485822,104.679403105462,104.779038544452,104.877780491632,104.976489964496,
105.075196748918,105.175519216035,105.274367757282,105.375427187332,105.476486617383,
105.575545750516,105.67446443986,105.774099861363,105.872841876573,105.971551416695,
106.070258267518,106.17058065361,106.26942925849,106.370488535188,106.471547811886,
106.570607096495,106.669525938662,106.769161322128,106.867903492302,106.966613187844,
107.06532019433,107.165642397345,107.264491156885,107.365550081638,107.46660900639,
107.565720969537,107.664694591166,107.763559737028,107.862348777346,107.96109209191,
108.059845284113,108.12371336303),.UNSPECIFIED.);
#254=B_SPLINE_CURVE_WITH_KNOTS('',3,(#15721,#15722,#15723,#15724,#15725,
#15726,#15727,#15728,#15729,#15730,#15731,#15732,#15733),.UNSPECIFIED.,
 .F.,.F.,(4,3,3,3,4),(108.123713363395,108.237935126024,108.353261782782,
108.461670200894,108.477780689588),.UNSPECIFIED.);
#255=B_SPLINE_CURVE_WITH_KNOTS('',3,(#15735,#15736,#15737,#15738,#15739,
#15740,#15741,#15742,#15743,#15744,#15745,#15746,#15747,#15748,#15749,#15750,
#15751,#15752,#15753,#15754,#15755,#15756,#15757,#15758),.UNSPECIFIED.,
 .F.,.F.,(4,2,2,2,2,2,2,2,2,2,2,4),(-0.0898945060156978,-0.0877788736441257,
-0.0584159942359854,-0.0420681203200915,-0.0318936166568689,-0.0285276046855637,
-0.0264136235710413,-0.0245613831015139,-0.02256053581784,-0.0198266182957172,
-0.0129848053672012,-0.00073538908808835),.UNSPECIFIED.);
#256=B_SPLINE_CURVE_WITH_KNOTS('',3,(#15759,#15760,#15761,#15762,#15763,
#15764,#15765,#15766,#15767,#15768,#15769,#15770,#15771,#15772,#15773,#15774,
#15775,#15776,#15777,#15778,#15779,#15780,#15781,#15782,#15783,#15784,#15785,
#15786,#15787,#15788,#15789,#15790,#15791,#15792,#15793,#15794,#15795,#15796,
#15797,#15798,#15799,#15800,#15801,#15802,#15803,#15804,#15805,#15806,#15807,
#15808,#15809,#15810,#15811,#15812,#15813,#15814,#15815,#15816,#15817,#15818,
#15819,#15820,#15821,#15822,#15823,#15824,#15825,#15826,#15827,#15828,#15829,
#15830,#15831,#15832,#15833,#15834,#15835,#15836,#15837,#15838,#15839,#15840,
#15841,#15842,#15843,#15844,#15845,#15846,#15847,#15848,#15849,#15850,#15851,
#15852,#15853,#15854,#15855,#15856,#15857,#15858,#15859,#15860,#15861,#15862,
#15863,#15864,#15865,#15866,#15867,#15868,#15869,#15870,#15871,#15872,#15873,
#15874,#15875,#15876,#15877,#15878,#15879,#15880,#15881,#15882,#15883,#15884,
#15885,#15886,#15887,#15888,#15889,#15890,#15891,#15892,#15893,#15894,#15895,
#15896,#15897,#15898,#15899,#15900,#15901,#15902,#15903,#15904,#15905,#15906,
#15907,#15908,#15909,#15910,#15911,#15912,#15913,#15914,#15915,#15916,#15917,
#15918,#15919,#15920,#15921,#15922,#15923,#15924,#15925,#15926,#15927,#15928,
#15929,#15930,#15931,#15932,#15933,#15934,#15935,#15936,#15937,#15938,#15939,
#15940,#15941,#15942,#15943,#15944,#15945,#15946,#15947,#15948,#15949,#15950,
#15951,#15952,#15953,#15954),.UNSPECIFIED.,.F.,.F.,(4,2,2,2,2,2,2,2,2,2,
2,2,2,2,2,2,2,2,2,2,2,2,2,2,2,2,2,2,2,2,2,2,2,2,2,2,2,2,2,2,2,2,2,2,2,2,
2,2,2,2,2,2,2,2,2,2,2,2,2,2,2,2,2,2,2,2,2,2,2,2,2,2,2,2,2,2,2,2,2,2,2,2,
2,2,2,2,2,2,2,2,2,2,2,2,2,2,2,4),(-3.17299869679545,-3.11930868620718,-3.08516340173328,
-3.0782033673962,-3.07420299319222,-3.07071230450638,-3.06638630930797,
-3.05970133226788,-3.01057690666402,-2.97143166652684,-2.95971840779162,
-2.95446075643838,-2.95144690533868,-2.94885196127524,-2.94691465319532,
-2.94475488930145,-2.94118378964679,-2.92926687777781,-2.8733577666771,
-2.83772729522022,-2.82850472930221,-2.82404147000846,-2.82053831344959,
-2.8166269896721,-2.8100763476369,-2.78639181069776,-2.7362217952012,-2.70523489407633,
-2.69984428601455,-2.69730626778358,-2.69534415057137,-2.69304812126027,
-2.68896725915922,-2.67026600134761,-2.61687386102311,-2.58276964344561,
-2.57581212225449,-2.57181256763865,-2.56832222822974,-2.56399619202329,
-2.55731024136613,-2.51013164139134,-2.47613848394035,-2.45215196593302,
-2.44794263153176,-2.44564353797843,-2.44368189528988,-2.44114847131218,
-2.43700648764584,-2.40258751709594,-2.33574739643697,-2.32625748155609,
-2.32174374069557,-2.31823510386827,-2.31435253101593,-2.3079323237752,
-2.28557987932447,-2.22837541068936,-2.20112534521756,-2.19680174369964,
-2.19447838274541,-2.1925193399347,-2.19001909025172,-2.18598847928527,
-2.16008795613757,-2.11364937095877,-2.08032853919854,-2.07340879037839,
-2.06941753445167,-2.06592654366318,-2.06158943649462,-2.05486657409817,
-2.00789996740124,-1.97417154799861,-1.95772113977322,-1.95109781991293,
-1.94609540520812,-1.94363284327397,-1.94186483412151,-1.93959127415406,
-1.93560872631805,-1.91843957669912,-1.87431182369492,-1.8314436777169,
-1.82321565830487,-1.81894926166893,-1.81546293016809,-1.81141865724694,
-1.80444174463076,-1.77305818201536,-1.72333265178782,-1.69868871668601,
-1.69445431188591,-1.69214996679527,-1.69018910419601,-1.68766348217317,
-1.68354749361738,-1.67617331063835),.UNSPECIFIED.);
#257=B_SPLINE_CURVE_WITH_KNOTS('',3,(#15960,#15961,#15962,#15963,#15964,
#15965,#15966,#15967,#15968,#15969,#15970,#15971,#15972,#15973,#15974,#15975,
#15976,#15977,#15978,#15979,#15980,#15981,#15982,#15983,#15984,#15985,#15986,
#15987,#15988,#15989,#15990,#15991,#15992,#15993,#15994,#15995,#15996,#15997,
#15998,#15999,#16000,#16001,#16002,#16003,#16004,#16005,#16006,#16007,#16008,
#16009,#16010,#16011,#16012,#16013,#16014,#16015,#16016,#16017,#16018,#16019,
#16020,#16021,#16022,#16023,#16024,#16025,#16026,#16027,#16028,#16029,#16030,
#16031,#16032,#16033,#16034,#16035,#16036,#16037,#16038,#16039,#16040,#16041,
#16042,#16043,#16044,#16045,#16046,#16047,#16048,#16049,#16050,#16051,#16052,
#16053,#16054,#16055,#16056,#16057,#16058,#16059,#16060,#16061,#16062,#16063,
#16064,#16065,#16066,#16067,#16068,#16069,#16070,#16071,#16072,#16073,#16074,
#16075,#16076,#16077,#16078,#16079,#16080,#16081,#16082,#16083,#16084,#16085,
#16086,#16087,#16088,#16089,#16090,#16091,#16092,#16093,#16094,#16095,#16096,
#16097,#16098,#16099,#16100,#16101,#16102,#16103,#16104,#16105,#16106,#16107,
#16108,#16109,#16110,#16111,#16112,#16113,#16114,#16115,#16116,#16117,#16118,
#16119,#16120,#16121,#16122,#16123,#16124,#16125,#16126,#16127,#16128,#16129,
#16130,#16131,#16132,#16133,#16134,#16135,#16136,#16137,#16138,#16139,#16140),
 .UNSPECIFIED.,.F.,.F.,(4,3,3,3,3,3,3,3,3,3,3,3,3,3,3,3,3,3,3,3,3,3,3,3,
3,3,3,3,3,3,3,3,3,3,3,3,3,3,3,3,3,3,3,3,3,3,3,3,3,3,3,3,3,3,3,3,3,3,3,3,
4),(95.9117879380488,96.0100034795647,96.1082084022929,96.2113902684322,
96.3097261601217,96.4081294765302,96.5066850939811,96.5209358668503,96.6199949843232,
96.7189136584695,96.81854908383,96.9172910850647,97.0160006116976,97.1147074495317,
97.2150298524872,97.3138784457295,97.4149377535417,97.5159970613539,97.6150561795708,
97.7139748544642,97.8136102796383,97.9123522816226,98.0110618090045,98.1097686475857,
98.2100910496536,98.3089396436311,98.4099989497443,98.5110582558575,98.6101173725349,
98.7090360458894,98.8086714714483,98.9074134719061,99.006122997769,99.1048298348414,
99.2051522387213,99.3040008312296,99.4050601407953,99.5061194503611,99.6051785675261,
99.7040972413552,99.8037326667939,99.9024746676917,100.001184193981,100.099891031466,
100.200213434816,100.299062027698,100.400121336281,100.501180644865,100.600239766633,
100.69915844509,100.798793869374,100.897535874927,100.99624540587,101.094952248002,
101.195274645844,101.294123243309,101.395182541339,101.496241839368,101.611067070977,
101.725797563226,101.840528055476),.UNSPECIFIED.);
#258=B_SPLINE_CURVE_WITH_KNOTS('',3,(#16141,#16142,#16143,#16144,#16145,
#16146,#16147,#16148,#16149,#16150,#16151,#16152,#16153),.UNSPECIFIED.,
 .F.,.F.,(4,3,3,3,4),(101.84052805585,101.939398954914,102.038252712471,
102.13715687785,102.194035073172),.UNSPECIFIED.);
#259=B_SPLINE_CURVE_WITH_KNOTS('',3,(#16154,#16155,#16156,#16157,#16158,
#16159,#16160,#16161,#16162,#16163,#16164,#16165,#16166,#16167,#16168,#16169,
#16170,#16171,#16172,#16173,#16174,#16175,#16176,#16177,#16178,#16179,#16180,
#16181,#16182,#16183,#16184,#16185,#16186,#16187,#16188,#16189,#16190,#16191,
#16192,#16193,#16194,#16195,#16196,#16197,#16198,#16199,#16200,#16201,#16202,
#16203,#16204,#16205,#16206,#16207,#16208,#16209,#16210,#16211,#16212,#16213,
#16214,#16215,#16216,#16217,#16218,#16219,#16220,#16221,#16222,#16223,#16224,
#16225,#16226,#16227,#16228,#16229,#16230,#16231,#16232,#16233,#16234,#16235,
#16236,#16237,#16238,#16239,#16240,#16241,#16242,#16243,#16244,#16245,#16246,
#16247,#16248,#16249,#16250,#16251,#16252,#16253,#16254,#16255,#16256,#16257,
#16258,#16259,#16260,#16261,#16262,#16263,#16264,#16265,#16266,#16267,#16268,
#16269,#16270,#16271,#16272,#16273,#16274,#16275,#16276,#16277,#16278,#16279,
#16280,#16281,#16282,#16283,#16284,#16285,#16286,#16287,#16288,#16289,#16290,
#16291,#16292,#16293,#16294,#16295,#16296,#16297,#16298,#16299,#16300,#16301,
#16302,#16303,#16304,#16305,#16306,#16307,#16308,#16309,#16310,#16311,#16312,
#16313,#16314,#16315,#16316,#16317,#16318,#16319,#16320,#16321,#16322,#16323,
#16324,#16325,#16326,#16327,#16328,#16329,#16330,#16331,#16332,#16333,#16334,
#16335,#16336,#16337,#16338,#16339,#16340,#16341,#16342,#16343,#16344,#16345,
#16346,#16347,#16348,#16349,#16350,#16351,#16352,#16353,#16354,#16355),
 .UNSPECIFIED.,.F.,.F.,(4,2,2,2,2,2,2,2,2,2,2,2,2,2,2,2,2,2,2,2,2,2,2,2,
2,2,2,2,2,2,2,2,2,2,2,2,2,2,2,2,2,2,2,2,2,2,2,2,2,2,2,2,2,2,2,2,2,2,2,2,
2,2,2,2,2,2,2,2,2,2,2,2,2,2,2,2,2,2,2,2,2,2,2,2,2,2,2,2,2,2,2,2,2,2,2,2,
2,2,2,2,4),(-1.67617331063835,-1.65240527865461,-1.58687592034162,-1.57442556265288,
-1.56926424535368,-1.56601000523216,-1.56241757877178,-1.55737807047799,
-1.54481344327795,-1.4793696505965,-1.44802118236873,-1.44390266605422,
-1.44137630223774,-1.43941540291114,-1.43711166835483,-1.43287998920887,
-1.40831238849089,-1.37469787011544,-1.3277573326033,-1.32105082638772,
-1.31671879965861,-1.31322833391444,-1.3092337844796,-1.30229826622656,
-1.26864079726897,-1.21935167748512,-1.19652066960891,-1.19259819116766,
-1.19013042844333,-1.18817331943532,-1.18582407860207,-1.181377308325,-1.14936068376642,
-1.14561538752557,-1.08666483299086,-1.07265258302901,-1.06724130086439,
-1.06394192907254,-1.06038726053178,-1.05555970995575,-1.04430782832272,
-1.00383906640406,-0.955902843636391,-0.943964555576926,-0.940391730966087,
-0.938231909977202,-0.936235182236847,-0.933439536542829,-0.926578127566507,
-0.916560121925209,-0.884645511785449,-0.829239768756867,-0.819441950638088,
-0.814920026342847,-0.811400557812437,-0.807561016390277,-0.801337251876116,
-0.778577818170857,-0.738872834052586,-0.697644244322333,-0.691211055000536,
-0.688679419105671,-0.68684210805264,-0.684801515971349,-0.681775846915014,
-0.673372644654906,-0.660172853642147,-0.622915133599126,-0.57429251824916,
-0.567608153363514,-0.563282978348824,-0.559793201584947,-0.555794147350037,
-0.54883710564091,-0.51471845981321,-0.461086219597697,-0.442677525577018,
-0.438616544874642,-0.436325255813899,-0.434362943197346,-0.431819124933974,
-0.426396509729469,-0.381917409217466,-0.327018231694746,-0.317305841914941,
-0.31273167827336,-0.309204618487064,-0.305389709784263,-0.29963636586302,
-0.280325453086069,-0.246025036075861,-0.194715530598949,-0.18918085810934,
-0.186259915204884,-0.1842603314317,-0.182150006312332,-0.178800731731504,
-0.167954900504291,-0.136827243060613,-0.104566733046293,-0.0902712750032826),
 .UNSPECIFIED.);
#260=B_SPLINE_CURVE_WITH_KNOTS('',3,(#16361,#16362,#16363,#16364,#16365,
#16366,#16367,#16368,#16369,#16370,#16371,#16372,#16373,#16374,#16375,#16376,
#16377,#16378,#16379,#16380,#16381,#16382,#16383,#16384,#16385,#16386,#16387,
#16388,#16389,#16390,#16391,#16392,#16393,#16394,#16395,#16396,#16397,#16398,
#16399,#16400,#16401,#16402,#16403,#16404,#16405,#16406,#16407,#16408,#16409,
#16410,#16411,#16412,#16413,#16414,#16415,#16416,#16417,#16418,#16419,#16420,
#16421,#16422,#16423,#16424,#16425,#16426,#16427,#16428,#16429,#16430,#16431,
#16432,#16433,#16434,#16435,#16436,#16437,#16438,#16439,#16440,#16441,#16442,
#16443,#16444,#16445,#16446,#16447,#16448,#16449,#16450,#16451,#16452,#16453,
#16454,#16455,#16456,#16457,#16458,#16459,#16460,#16461,#16462,#16463,#16464,
#16465,#16466,#16467,#16468,#16469,#16470,#16471,#16472,#16473,#16474,#16475,
#16476,#16477,#16478,#16479,#16480,#16481,#16482,#16483,#16484,#16485,#16486,
#16487,#16488,#16489,#16490,#16491,#16492,#16493,#16494,#16495,#16496,#16497,
#16498,#16499,#16500,#16501,#16502,#16503,#16504,#16505,#16506,#16507,#16508,
#16509,#16510,#16511,#16512,#16513,#16514,#16515,#16516,#16517,#16518,#16519,
#16520,#16521,#16522,#16523,#16524,#16525,#16526,#16527,#16528,#16529,#16530,
#16531,#16532,#16533,#16534,#16535,#16536,#16537,#16538,#16539,#16540,#16541,
#16542,#16543,#16544),.UNSPECIFIED.,.F.,.F.,(4,3,3,3,3,3,3,3,3,3,3,3,3,
3,3,3,3,3,3,3,3,3,3,3,3,3,3,3,3,3,3,3,3,3,3,3,3,3,3,3,3,3,3,3,3,3,3,3,3,
3,3,3,3,3,3,3,3,3,3,3,3,4),(89.6284844345084,89.7274368855644,89.8303283623474,
89.929082090238,90.02779646593,90.1265012818364,90.2252263120905,90.3240613148707,
90.4229615017662,90.5220189447325,90.5505686998286,90.6496278174091,90.7485464916642,
90.8481819169977,90.9469239183443,91.04563344509,91.1443402830374,91.2446626858612,
91.3435112792174,91.4445705867748,91.5456298943323,91.6446890119303,91.7436076862031,
91.8432431115322,91.9419851128963,92.0406946396595,92.1394014776244,92.2397238804273,
92.3385724738006,92.4396317813182,92.5406910888358,92.6397502064081,92.7386688806553,
92.8383043059908,92.9370463073297,93.0357558340677,93.1344626720077,93.2347850748407,
93.3336336681899,93.4346929757647,93.5357522833395,93.6348114009011,93.7337300751373,
93.8333655004755,93.9321075018028,94.030817028529,94.129523866457,94.2298462693035,
94.3286948626404,94.4297541702417,94.5308134778431,94.6298725955208,94.7287912698735,
94.8284266951827,94.9271686966265,95.0258782234692,95.1245850615132,95.2249074642216,
95.3237560576724,95.4248153650096,95.5258746723467,95.5573427486709),
 .UNSPECIFIED.);
#261=B_SPLINE_CURVE_WITH_KNOTS('',3,(#16545,#16546,#16547,#16548,#16549,
#16550,#16551,#16552,#16553,#16554,#16555,#16556,#16557),.UNSPECIFIED.,
 .F.,.F.,(4,3,3,3,4),(95.5573427489394,95.6558631085308,95.7542623752097,
95.8525566826487,95.9117879380488),.UNSPECIFIED.);
#262=B_SPLINE_CURVE_WITH_KNOTS('',3,(#16559,#16560,#16561,#16562,#16563,
#16564,#16565,#16566,#16567,#16568,#16569,#16570,#16571,#16572,#16573,#16574,
#16575,#16576),.UNSPECIFIED.,.F.,.F.,(4,2,2,2,2,2,2,2,4),(-0.0902712750032826,
-0.0715222222732456,-0.0644702729272379,-0.0604092697845244,-0.0569242638253706,
-0.0535880866901934,-0.0494330478813112,-0.0431186936204873,-0.000735300760668054),
 .UNSPECIFIED.);
#263=B_SPLINE_CURVE_WITH_KNOTS('',3,(#16577,#16578,#16579,#16580,#16581,
#16582,#16583,#16584,#16585,#16586,#16587,#16588,#16589,#16590,#16591,#16592,
#16593,#16594,#16595,#16596,#16597,#16598,#16599,#16600,#16601,#16602,#16603,
#16604,#16605,#16606,#16607,#16608,#16609,#16610,#16611,#16612,#16613,#16614,
#16615,#16616,#16617,#16618,#16619,#16620,#16621,#16622,#16623,#16624,#16625,
#16626,#16627,#16628,#16629,#16630,#16631,#16632,#16633,#16634,#16635,#16636,
#16637,#16638,#16639,#16640,#16641,#16642,#16643,#16644,#16645,#16646,#16647,
#16648,#16649,#16650,#16651,#16652,#16653,#16654,#16655,#16656,#16657,#16658,
#16659,#16660,#16661,#16662,#16663,#16664,#16665,#16666,#16667,#16668,#16669,
#16670,#16671,#16672,#16673,#16674,#16675,#16676,#16677,#16678,#16679,#16680,
#16681,#16682,#16683,#16684,#16685,#16686,#16687,#16688,#16689,#16690,#16691,
#16692,#16693,#16694,#16695,#16696,#16697,#16698,#16699,#16700,#16701,#16702,
#16703,#16704,#16705,#16706,#16707,#16708,#16709,#16710,#16711,#16712,#16713,
#16714,#16715,#16716,#16717,#16718,#16719,#16720,#16721,#16722,#16723,#16724,
#16725,#16726,#16727,#16728,#16729,#16730,#16731,#16732,#16733,#16734,#16735,
#16736,#16737,#16738,#16739,#16740,#16741,#16742,#16743,#16744,#16745,#16746,
#16747,#16748,#16749,#16750,#16751,#16752,#16753,#16754,#16755,#16756,#16757,
#16758,#16759,#16760,#16761,#16762,#16763,#16764,#16765,#16766,#16767,#16768,
#16769,#16770,#16771,#16772),.UNSPECIFIED.,.F.,.F.,(4,2,2,2,2,2,2,2,2,2,
2,2,2,2,2,2,2,2,2,2,2,2,2,2,2,2,2,2,2,2,2,2,2,2,2,2,2,2,2,2,2,2,2,2,2,2,
2,2,2,2,2,2,2,2,2,2,2,2,2,2,2,2,2,2,2,2,2,2,2,2,2,2,2,2,2,2,2,2,2,2,2,2,
2,2,2,2,2,2,2,2,2,2,2,2,2,2,2,4),(-3.17301486575304,-3.1206283445989,-3.11407337427932,
-3.11056394982659,-3.10753018932838,-3.10548730126036,-3.10365040474306,
-3.10112245888732,-3.0947153741012,-3.05241203064243,-3.01284825003375,
-2.99079619169157,-2.98488514110301,-2.98099007817135,-2.97748268291822,
-2.97298798518856,-2.96360368478635,-2.90144618614788,-2.86327364670942,
-2.85800863157681,-2.85549422419458,-2.85353353619308,-2.85121937078231,
-2.84705977303144,-2.82696252670283,-2.7602873464793,-2.74632465560078,
-2.7360404617071,-2.73137994349378,-2.7278506959479,-2.724036688092,-2.71793424587706,
-2.69861344667929,-2.63812877933858,-2.61935040144618,-2.61212096353624,
-2.60676698599902,-2.60423563489,-2.60227373439065,-2.59997218175929,-2.59586810912478,
-2.57677422610921,-2.51485685331853,-2.48879305540503,-2.48230695477302,
-2.47840940274739,-2.47490297859551,-2.47041398216779,-2.46105822842412,
-2.39996331632049,-2.3609309519789,-2.35551534083815,-2.35297233482591,
-2.35100949683694,-2.34871627676867,-2.34464880324007,-2.3261520343103,
-2.27254313667151,-2.23841063472823,-2.23145093024342,-2.22745050336487,
-2.22395962693813,-2.21963321554159,-2.21294724305685,-2.16432918558983,
-2.12707837980584,-2.11388481409811,-2.10548300889584,-2.10245696381255,
-2.10041584346821,-2.0985778517584,-2.09604499381951,-2.0896072678779,-2.04840130561755,
-2.00862123847753,-1.98583514559368,-1.97960772459686,-1.97576665709208,
-1.97224627618495,-1.96772385759357,-1.95792764197776,-1.90247498967226,
-1.88839175429163,-1.85846943078831,-1.85307884475064,-1.850540663228,-1.8485783394236,
-1.84628197463637,-1.84220029875838,-1.82349073063694,-1.77009891745668,
-1.73599163242005,-1.72903337740783,-1.7250333892754,-1.72154266468868,
-1.71721614218406,-1.7105294228205,-1.67610690530384),.UNSPECIFIED.);
#264=B_SPLINE_CURVE_WITH_KNOTS('',3,(#16778,#16779,#16780,#16781,#16782,
#16783,#16784,#16785,#16786,#16787,#16788,#16789,#16790,#16791,#16792,#16793,
#16794,#16795,#16796,#16797,#16798,#16799,#16800,#16801,#16802,#16803,#16804,
#16805,#16806,#16807,#16808,#16809,#16810,#16811,#16812,#16813,#16814,#16815,
#16816,#16817,#16818,#16819,#16820,#16821,#16822,#16823,#16824,#16825,#16826,
#16827,#16828,#16829,#16830,#16831,#16832,#16833,#16834,#16835,#16836,#16837,
#16838,#16839,#16840,#16841,#16842,#16843,#16844,#16845,#16846,#16847,#16848,
#16849,#16850,#16851,#16852,#16853,#16854,#16855,#16856,#16857,#16858,#16859,
#16860,#16861,#16862,#16863,#16864,#16865,#16866,#16867,#16868,#16869,#16870,
#16871,#16872,#16873,#16874,#16875,#16876,#16877,#16878,#16879,#16880,#16881,
#16882,#16883,#16884,#16885,#16886,#16887,#16888,#16889,#16890,#16891,#16892,
#16893,#16894,#16895,#16896,#16897,#16898,#16899,#16900,#16901,#16902,#16903,
#16904,#16905,#16906,#16907,#16908,#16909,#16910,#16911,#16912,#16913,#16914,
#16915,#16916,#16917,#16918,#16919,#16920,#16921,#16922,#16923,#16924,#16925,
#16926,#16927,#16928,#16929,#16930,#16931,#16932,#16933,#16934,#16935,#16936,
#16937,#16938,#16939,#16940,#16941,#16942,#16943,#16944,#16945,#16946,#16947,
#16948,#16949,#16950,#16951,#16952,#16953,#16954,#16955,#16956,#16957,#16958,
#16959,#16960,#16961),.UNSPECIFIED.,.F.,.F.,(4,3,3,3,3,3,3,3,3,3,3,3,3,
3,3,3,3,3,3,3,3,3,3,3,3,3,3,3,3,3,3,3,3,3,3,3,3,3,3,3,3,3,3,3,3,3,3,3,3,
3,3,3,3,3,3,3,3,3,3,3,3,4),(83.3443379263979,83.4447395826579,83.5453289227515,
83.5851403383034,83.684199455888,83.7831181301475,83.8827535554799,83.9814955568308,
84.0802050835807,84.1789119215326,84.2792343243512,84.3780829177116,84.4791422252593,
84.580201532807,84.6792606503917,84.7781793246507,84.8778147499832,84.9765567513339,
85.0752662780837,85.1739731160353,85.2742955188541,85.3731441122144,85.4742034197625,
85.5752627273106,85.6743218448955,85.7732405191552,85.8728759444876,85.9716179458387,
86.0703274725889,86.1690343105409,86.2693567133593,86.3682053067201,86.4692646142671,
86.5703239218142,86.6693830393988,86.7683017136583,86.8679371389907,86.9666791403415,
87.0653886670914,87.1640955050432,87.2644179078619,87.3632665012222,87.46432580877,
87.5653851163178,87.6644442339017,87.7633629081602,87.8629983334929,87.9617403348428,
88.060449861592,88.159156699543,88.2594791023626,88.3583276957222,88.4593870032718,
88.5604463108214,88.6586782050391,88.7567801508798,88.8547831364389,88.9527180356713,
89.0506354266417,89.1485438993684,89.2465050935619,89.2741574414913),
 .UNSPECIFIED.);
#265=B_SPLINE_CURVE_WITH_KNOTS('',3,(#16962,#16963,#16964,#16965,#16966,
#16967,#16968,#16969,#16970,#16971,#16972,#16973,#16974),.UNSPECIFIED.,
 .F.,.F.,(4,3,3,3,4),(89.2741574417129,89.3952590898568,89.5183032212418,
89.555507505325,89.6284844345084),.UNSPECIFIED.);
#266=B_SPLINE_CURVE_WITH_KNOTS('',3,(#16975,#16976,#16977,#16978,#16979,
#16980,#16981,#16982,#16983,#16984,#16985,#16986,#16987,#16988,#16989,#16990,
#16991,#16992,#16993,#16994,#16995,#16996,#16997,#16998,#16999,#17000,#17001,
#17002,#17003,#17004,#17005,#17006,#17007,#17008,#17009,#17010,#17011,#17012,
#17013,#17014,#17015,#17016,#17017,#17018,#17019,#17020,#17021,#17022,#17023,
#17024,#17025,#17026,#17027,#17028,#17029,#17030,#17031,#17032,#17033,#17034,
#17035,#17036,#17037,#17038,#17039,#17040,#17041,#17042,#17043,#17044,#17045,
#17046,#17047,#17048,#17049,#17050,#17051,#17052,#17053,#17054,#17055,#17056,
#17057,#17058,#17059,#17060,#17061,#17062,#17063,#17064,#17065,#17066,#17067,
#17068,#17069,#17070,#17071,#17072,#17073,#17074,#17075,#17076,#17077,#17078,
#17079,#17080,#17081,#17082,#17083,#17084,#17085,#17086,#17087,#17088,#17089,
#17090,#17091,#17092,#17093,#17094,#17095,#17096,#17097,#17098,#17099,#17100,
#17101,#17102,#17103,#17104,#17105,#17106,#17107,#17108,#17109,#17110,#17111,
#17112,#17113,#17114,#17115,#17116,#17117,#17118,#17119,#17120,#17121,#17122,
#17123,#17124,#17125,#17126,#17127,#17128,#17129,#17130,#17131,#17132,#17133,
#17134,#17135,#17136,#17137,#17138,#17139,#17140,#17141,#17142,#17143,#17144,
#17145,#17146,#17147,#17148,#17149,#17150,#17151,#17152,#17153,#17154,#17155,
#17156,#17157,#17158,#17159,#17160,#17161,#17162,#17163,#17164,#17165,#17166,
#17167,#17168,#17169,#17170,#17171,#17172,#17173,#17174,#17175,#17176,#17177,
#17178,#17179,#17180,#17181,#17182,#17183,#17184,#17185,#17186,#17187,#17188,
#17189,#17190,#17191,#17192,#17193,#17194,#17195,#17196,#17197,#17198,#17199,
#17200,#17201,#17202,#17203,#17204),.UNSPECIFIED.,.F.,.F.,(4,2,2,2,2,2,
2,2,2,2,2,2,2,2,2,2,2,2,2,2,2,2,2,2,2,2,2,2,2,2,2,2,2,2,2,2,2,2,2,2,2,2,
2,2,2,2,2,2,2,2,2,2,2,2,2,2,2,2,2,2,2,2,2,2,2,2,2,2,2,2,2,2,2,2,2,2,2,2,
2,2,2,2,2,2,2,2,2,2,2,2,2,2,2,2,2,2,2,2,2,2,2,2,2,2,2,2,2,2,2,2,2,2,2,2,
4),(-1.67610690530384,-1.6616369887965,-1.62333502436374,-1.61096724728315,
-1.60294978026278,-1.59997780896286,-1.59794773242811,-1.5960994502116,
-1.59352637505502,-1.58683233751666,-1.5768486480398,-1.54513187295802,
-1.48942278688358,-1.47963748100296,-1.47511721859763,-1.47159733351867,
-1.46775561050102,-1.461524424053,-1.43868987089723,-1.39875742273635,-1.3578246093106,
-1.35138663769448,-1.34885387598515,-1.34701600803389,-1.34497511122133,
-1.34194952498888,-1.33355000241599,-1.3203593926047,-1.28308031174571,
-1.23444010741391,-1.22775420407525,-1.22342804097365,-1.21993747175966,
-1.21593751468033,-1.2089789159288,-1.1748529936249,-1.12121280191642,-1.10279567750514,
-1.0987335162647,-1.09644164856244,-1.09447889831456,-1.09193458805955,
-1.08651119289879,-1.04129543346864,-0.987136726983808,-0.978257759967374,
-0.973793857064194,-0.970510122579206,-0.966942804391354,-0.962044746684032,
-0.950371840794784,-0.912877498172957,-0.869045980907529,-0.851501911813965,
-0.847494624944847,-0.845215276346162,-0.843269559894183,-0.840717627740071,
-0.835253506745143,-0.796548696827613,-0.735116849406508,-0.725795186697969,
-0.721313136481602,-0.717808029656794,-0.713907718925966,-0.707406984130386,
-0.681125986141361,-0.617641911449229,-0.600240180318242,-0.59624212837838,
-0.593964878170609,-0.592018837985877,-0.589463724190013,-0.583982715851276,
-0.543041178005608,-0.484272344219113,-0.474814472468086,-0.470289464739249,
-0.466769131731241,-0.462930195873847,-0.456710891376531,-0.434010493816948,
-0.394493357917899,-0.352996728369668,-0.346559228090515,-0.344026660515154,
-0.342188936429314,-0.34014820298669,-0.337122865100116,-0.32872407166341,
-0.315534646011128,-0.259359438239033,-0.22887831113395,-0.221951293100366,
-0.217918225180366,-0.214436322317702,-0.214354968226818,-0.214282117819541,
-0.214216647499058,-0.214157620443795,-0.214104249088067,-0.21405586634476,
-0.214011903269021,-0.213971871545232,-0.213935349618804,-0.21385359452961,
-0.209447266042847,-0.200158986039909,-0.187794132821037,-0.155762060016917,
-0.105580955608446,-0.0963519117470314,-0.0931109279364058,-0.0912314720885978,
-0.0899840747648518),.UNSPECIFIED.);
#267=B_SPLINE_CURVE_WITH_KNOTS('',3,(#17210,#17211,#17212,#17213,#17214,
#17215,#17216,#17217,#17218,#17219,#17220,#17221,#17222,#17223,#17224,#17225,
#17226,#17227,#17228,#17229,#17230,#17231,#17232,#17233,#17234,#17235,#17236,
#17237,#17238,#17239,#17240,#17241,#17242,#17243,#17244,#17245,#17246,#17247,
#17248,#17249,#17250,#17251,#17252,#17253,#17254,#17255,#17256,#17257,#17258,
#17259,#17260,#17261,#17262,#17263,#17264,#17265,#17266,#17267,#17268,#17269,
#17270,#17271,#17272,#17273,#17274,#17275,#17276,#17277,#17278,#17279,#17280,
#17281,#17282,#17283,#17284,#17285,#17286,#17287,#17288,#17289,#17290,#17291,
#17292,#17293,#17294,#17295,#17296,#17297,#17298,#17299,#17300,#17301,#17302,
#17303,#17304,#17305,#17306,#17307,#17308,#17309,#17310,#17311,#17312,#17313,
#17314,#17315,#17316,#17317,#17318,#17319,#17320,#17321,#17322,#17323,#17324,
#17325,#17326,#17327,#17328,#17329,#17330,#17331,#17332,#17333,#17334,#17335,
#17336,#17337,#17338,#17339,#17340,#17341,#17342,#17343,#17344,#17345,#17346,
#17347,#17348,#17349,#17350,#17351,#17352,#17353,#17354,#17355,#17356,#17357,
#17358,#17359,#17360,#17361,#17362,#17363,#17364,#17365,#17366,#17367,#17368,
#17369,#17370,#17371,#17372,#17373,#17374,#17375,#17376,#17377,#17378,#17379,
#17380,#17381,#17382,#17383,#17384,#17385,#17386,#17387,#17388,#17389,#17390),
 .UNSPECIFIED.,.F.,.F.,(4,3,3,3,3,3,3,3,3,3,3,3,3,3,3,3,3,3,3,3,3,3,3,3,
3,3,3,3,3,3,3,3,3,3,3,3,3,3,3,3,3,3,3,3,3,3,3,3,3,3,3,3,3,3,3,3,3,3,3,3,
4),(77.0622289400388,77.1598104900222,77.2573935220109,77.3550721489496,
77.4528016237076,77.5506953978965,77.6147731712817,77.7138322888664,77.8127509631259,
77.9123863884583,78.0111283898092,78.1098379165591,78.2085447545109,78.3088671573295,
78.4077157506899,78.5087750582376,78.6098343657853,78.7088934833699,78.8078121576294,
78.9074475829619,79.0061895843128,79.1048991110627,79.2036059490145,79.3039283518331,
79.4027769451936,79.5038362527413,79.6048955602889,79.7039546778735,79.802873352133,
79.9025087774654,80.0012507788162,80.0999603055661,80.1986671435179,80.2989895463366,
80.397838139697,80.4988974472448,80.5999567547925,80.6990158723771,80.7979345466367,
80.8975699719691,80.99631197332,81.0950215000699,81.1937283380216,81.2940507408402,
81.3928993342007,81.4939586417484,81.5950179492961,81.6940770668806,81.7929957411399,
81.8926311664724,81.9913731678233,82.0900826945732,82.1887895325249,82.2891119353436,
82.3879605287041,82.4890198362519,82.5900791437997,82.699827112012,82.8092455102988,
82.9180995588103,82.990972133969),.UNSPECIFIED.);
#268=B_SPLINE_CURVE_WITH_KNOTS('',3,(#17391,#17392,#17393,#17394,#17395,
#17396,#17397,#17398,#17399,#17400,#17401,#17402,#17403),.UNSPECIFIED.,
 .F.,.F.,(4,3,3,3,4),(82.9909721343117,83.0910899879919,83.1912299242207,
83.2914717628289,83.3443379263979),.UNSPECIFIED.);
#269=B_SPLINE_CURVE_WITH_KNOTS('',3,(#17405,#17406,#17407,#17408,#17409,
#17410,#17411,#17412,#17413,#17414,#17415,#17416),.UNSPECIFIED.,.F.,.F.,
(4,2,2,2,2,4),(-0.0899840747648518,-0.0892272765238516,-0.086389960181531,
-0.0792681453191874,-0.0687374840803309,-0.000736241093440834),
 .UNSPECIFIED.);
#270=B_SPLINE_CURVE_WITH_KNOTS('',3,(#17417,#17418,#17419,#17420,#17421,
#17422,#17423,#17424,#17425,#17426,#17427,#17428,#17429,#17430,#17431,#17432,
#17433,#17434,#17435,#17436,#17437,#17438,#17439,#17440,#17441,#17442,#17443,
#17444,#17445,#17446,#17447,#17448,#17449,#17450,#17451,#17452,#17453,#17454,
#17455,#17456,#17457,#17458,#17459,#17460,#17461,#17462,#17463,#17464,#17465,
#17466,#17467,#17468,#17469,#17470,#17471,#17472,#17473,#17474,#17475,#17476,
#17477,#17478,#17479,#17480,#17481,#17482,#17483,#17484,#17485,#17486,#17487,
#17488,#17489,#17490,#17491,#17492,#17493,#17494,#17495,#17496,#17497,#17498,
#17499,#17500,#17501,#17502,#17503,#17504,#17505,#17506,#17507,#17508,#17509,
#17510,#17511,#17512,#17513,#17514,#17515,#17516,#17517,#17518,#17519,#17520,
#17521,#17522,#17523,#17524,#17525,#17526,#17527,#17528,#17529,#17530,#17531,
#17532,#17533,#17534,#17535,#17536,#17537,#17538,#17539,#17540,#17541,#17542,
#17543,#17544,#17545,#17546,#17547,#17548,#17549,#17550,#17551,#17552,#17553,
#17554,#17555,#17556,#17557,#17558,#17559,#17560,#17561,#17562,#17563,#17564,
#17565,#17566,#17567,#17568,#17569,#17570,#17571,#17572,#17573,#17574,#17575,
#17576,#17577,#17578,#17579,#17580,#17581,#17582,#17583,#17584,#17585,#17586,
#17587,#17588,#17589,#17590,#17591,#17592,#17593,#17594,#17595,#17596,#17597,
#17598,#17599,#17600,#17601,#17602,#17603,#17604,#17605,#17606,#17607,#17608,
#17609,#17610,#17611,#17612,#17613,#17614,#17615,#17616,#17617,#17618,#17619,
#17620,#17621,#17622,#17623,#17624,#17625,#17626,#17627,#17628,#17629,#17630,
#17631,#17632,#17633,#17634,#17635,#17636,#17637,#17638,#17639,#17640,#17641,
#17642,#17643,#17644,#17645,#17646,#17647,#17648,#17649,#17650,#17651,#17652,
#17653,#17654,#17655,#17656),.UNSPECIFIED.,.F.,.F.,(4,2,2,2,2,2,2,2,2,2,
2,2,2,2,2,2,2,2,2,2,2,2,2,2,2,2,2,2,2,2,2,2,2,2,2,2,2,2,2,2,2,2,2,2,2,2,
2,2,2,2,2,2,2,2,2,2,2,2,2,2,2,2,2,2,2,2,2,2,2,2,2,2,2,2,2,2,2,2,2,2,2,2,
2,2,2,2,2,2,2,2,2,2,2,2,2,2,2,2,2,2,2,2,2,2,2,2,2,2,2,2,2,2,2,2,2,2,2,2,
2,4),(-3.17255739968768,-3.1576069634066,-3.14810732836851,-3.1434954008955,
-3.14001384955691,-3.1366931493451,-3.13341536905306,-3.12897456274974,
-3.11789721165226,-3.09383691093029,-3.05431535560038,-3.02234715151782,
-3.01585248463183,-3.0131172296154,-3.0111303830683,-3.00894508086758,-3.00525735952246,
-2.99217804282792,-2.93735433907239,-2.91155966332515,-2.90077694145438,
-2.89242416032427,-2.888175408801,-2.88813682609947,-2.88809592484398,-2.88805255764975,
-2.88800656701802,-2.88795778460018,-2.88790603041391,-2.88785111200833,
-2.8877928235698,-2.88773094498928,-2.88766524088317,-2.88759545956919,
-2.88752133201663,-2.88744257077892,-2.8873916312179,-2.88732376443447,
-2.88383385795497,-2.87950808817963,-2.87282203001381,-2.82425470811119,
-2.78707875500556,-2.77382862793589,-2.76540157604663,-2.76237260180553,
-2.76033129012896,-2.75849452277717,-2.75596512238182,-2.7495456510586,
-2.70805249457556,-2.66848411540881,-2.65343162211825,-2.64254216049128,
-2.63777630490657,-2.63423179872332,-2.6304619102664,-2.62455886316772,
-2.60692581809593,-2.54452914118,-2.52565285485955,-2.51839967740849,-2.51303255352772,
-2.51049922246228,-2.50853776331244,-2.50623903802823,-2.50214536434144,
-2.48321505155067,-2.41545795016458,-2.40141088354109,-2.39108020280365,
-2.38641256868019,-2.38288347968782,-2.37954029889709,-2.37389537766366,
-2.35826974519288,-2.29366213650761,-2.27455594012858,-2.26368070816965,
-2.26035230955456,-2.25824652364475,-2.25624393067389,-2.25377574107253,
-2.24771576250172,-2.19730867504513,-2.15167721387559,-2.14035302513635,
-2.13551344101775,-2.13195685753111,-2.12866062188454,-2.12326571199652,
-2.10935786499212,-2.05034045231045,-2.01466594914582,-2.01015434745451,
-2.00779164049775,-2.00583529778113,-2.00338352628568,-1.99951373709683,
-1.97798602112789,-1.92961929266239,-1.90580901282673,-1.89557754644634,
-1.88750095468426,-1.88326570157758,-1.88011904533669,-1.87617276256836,
-1.86945916271794,-1.84363199615531,-1.78972878497356,-1.77173815772437,
-1.7647101512041,-1.75947235049566,-1.75696389032812,-1.7551908631053,-1.75294907964165,
-1.74910487000024,-1.73376493847121,-1.68831539067684,-1.67587718660285),
 .UNSPECIFIED.);
#271=B_SPLINE_CURVE_WITH_KNOTS('',3,(#17662,#17663,#17664,#17665,#17666,
#17667,#17668,#17669,#17670,#17671,#17672,#17673,#17674,#17675,#17676,#17677,
#17678,#17679,#17680,#17681,#17682,#17683,#17684,#17685,#17686,#17687,#17688,
#17689,#17690,#17691,#17692,#17693,#17694,#17695,#17696,#17697,#17698,#17699,
#17700,#17701,#17702,#17703,#17704,#17705,#17706,#17707,#17708,#17709,#17710,
#17711,#17712,#17713,#17714,#17715,#17716,#17717,#17718,#17719,#17720,#17721,
#17722,#17723,#17724,#17725,#17726,#17727,#17728,#17729,#17730,#17731,#17732,
#17733,#17734,#17735,#17736,#17737,#17738,#17739,#17740,#17741,#17742,#17743,
#17744,#17745,#17746,#17747,#17748,#17749,#17750,#17751,#17752,#17753,#17754,
#17755,#17756,#17757,#17758,#17759,#17760,#17761,#17762,#17763,#17764,#17765,
#17766,#17767,#17768,#17769,#17770,#17771,#17772,#17773,#17774,#17775,#17776,
#17777,#17778,#17779,#17780,#17781,#17782,#17783,#17784,#17785,#17786,#17787,
#17788,#17789,#17790,#17791,#17792,#17793,#17794,#17795,#17796,#17797,#17798,
#17799,#17800,#17801,#17802,#17803,#17804,#17805,#17806,#17807,#17808,#17809,
#17810,#17811,#17812,#17813,#17814,#17815,#17816,#17817,#17818,#17819,#17820,
#17821,#17822,#17823,#17824,#17825,#17826,#17827,#17828,#17829,#17830,#17831,
#17832,#17833,#17834,#17835,#17836,#17837,#17838,#17839,#17840,#17841,#17842),
 .UNSPECIFIED.,.F.,.F.,(4,3,3,3,3,3,3,3,3,3,3,3,3,3,3,3,3,3,3,3,3,3,3,3,
3,3,3,3,3,3,3,3,3,3,3,3,3,3,3,3,3,3,3,3,3,3,3,3,3,3,3,3,3,3,3,3,3,3,3,3,
4),(70.7790859150367,70.8779677866101,70.976750148986,71.0754792147284,
71.1741847940566,71.272896666296,71.3717103894916,71.4705767843822,71.5696140703515,
71.64440600426,71.7434651218447,71.8423837961042,71.9420192214366,72.0407612227875,
72.1394707495375,72.2381775874893,72.3384999903079,72.4373485836684,72.5384078912161,
72.6394671987637,72.7385263163483,72.8374449906077,72.9370804159401,73.0358224172909,
73.1345319440408,73.2332387819926,73.3335611848112,73.4324097781717,73.5334690857194,
73.6345283932672,73.7335875108519,73.8325061851113,73.9321416104438,74.0308836117947,
74.1295931385446,74.2282999764964,74.328622379315,74.4274709726755,74.5285302802232,
74.6295895877709,74.7286487053556,74.827567379615,74.9272028049475,75.0259448062983,
75.1246543330483,75.223361171,75.3236835738186,75.4225321671791,75.5235914747268,
75.6246507822745,75.7237098998592,75.8226285741186,75.9222639994511,76.0210060008019,
76.1197155275518,76.2184223655036,76.3187447683222,76.4175933616826,76.5186526692304,
76.6197119767781,76.7077868271321),.UNSPECIFIED.);
#272=B_SPLINE_CURVE_WITH_KNOTS('',3,(#17843,#17844,#17845,#17846,#17847,
#17848,#17849,#17850,#17851,#17852,#17853,#17854,#17855),.UNSPECIFIED.,
 .F.,.F.,(4,3,3,3,4),(76.7077868273919,76.80563266964,76.9033659598873,
77.0010095015004,77.0622289400388),.UNSPECIFIED.);
#273=B_SPLINE_CURVE_WITH_KNOTS('',3,(#17856,#17857,#17858,#17859,#17860,
#17861,#17862,#17863,#17864,#17865,#17866,#17867,#17868,#17869,#17870,#17871,
#17872,#17873,#17874,#17875,#17876,#17877,#17878,#17879,#17880,#17881,#17882,
#17883,#17884,#17885,#17886,#17887,#17888,#17889,#17890,#17891,#17892,#17893,
#17894,#17895,#17896,#17897,#17898,#17899,#17900,#17901,#17902,#17903,#17904,
#17905,#17906,#17907,#17908,#17909,#17910,#17911,#17912,#17913,#17914,#17915,
#17916,#17917,#17918,#17919,#17920,#17921,#17922,#17923,#17924,#17925,#17926,
#17927,#17928,#17929,#17930,#17931,#17932,#17933,#17934,#17935,#17936,#17937,
#17938,#17939,#17940,#17941,#17942,#17943,#17944,#17945,#17946,#17947,#17948,
#17949,#17950,#17951,#17952,#17953,#17954,#17955,#17956,#17957,#17958,#17959,
#17960,#17961,#17962,#17963,#17964,#17965,#17966,#17967,#17968,#17969,#17970,
#17971,#17972,#17973,#17974,#17975,#17976,#17977,#17978,#17979,#17980,#17981,
#17982,#17983,#17984,#17985,#17986,#17987,#17988,#17989,#17990,#17991,#17992,
#17993,#17994,#17995,#17996,#17997,#17998,#17999,#18000,#18001,#18002,#18003,
#18004,#18005,#18006,#18007,#18008,#18009,#18010,#18011,#18012,#18013,#18014,
#18015,#18016,#18017,#18018,#18019,#18020,#18021,#18022,#18023,#18024,#18025,
#18026,#18027,#18028,#18029,#18030,#18031,#18032,#18033,#18034,#18035,#18036,
#18037,#18038,#18039,#18040,#18041,#18042,#18043,#18044,#18045,#18046,#18047,
#18048,#18049,#18050,#18051,#18052,#18053,#18054,#18055,#18056,#18057,#18058,
#18059,#18060,#18061,#18062,#18063,#18064,#18065,#18066,#18067,#18068,#18069,
#18070,#18071,#18072,#18073,#18074,#18075,#18076,#18077,#18078,#18079,#18080,
#18081,#18082,#18083,#18084,#18085,#18086,#18087,#18088,#18089,#18090,#18091,
#18092,#18093,#18094,#18095,#18096,#18097,#18098,#18099,#18100,#18101,#18102,
#18103,#18104,#18105,#18106,#18107,#18108,#18109,#18110,#18111,#18112,#18113,
#18114,#18115,#18116,#18117,#18118,#18119),.UNSPECIFIED.,.F.,.F.,(4,2,2,
2,2,2,2,2,2,2,2,2,2,2,2,2,2,2,2,2,2,2,2,2,2,2,2,2,2,2,2,2,2,2,2,2,2,2,2,
2,2,2,2,2,2,2,2,2,2,2,2,2,2,2,2,2,2,2,2,2,2,2,2,2,2,2,2,2,2,2,2,2,2,2,2,
2,2,2,2,2,2,2,2,2,2,2,2,2,2,2,2,2,2,2,2,2,2,2,2,2,2,2,2,2,2,2,2,2,2,2,2,
2,2,2,2,2,2,2,2,2,2,2,2,2,2,2,2,2,2,2,2,4),(-1.67587718660285,-1.64470114731754,
-1.63647046963179,-1.63220378597921,-1.62871775902039,-1.62467444600192,
-1.6177007090087,-1.58636809487528,-1.55382222748207,-1.51560561651707,
-1.50915676664446,-1.50662260068978,-1.50478470099826,-1.50274495878806,
-1.4997231097777,-1.49134699995697,-1.47820598339102,-1.44088827611686,
-1.39223653872546,-1.38555236722436,-1.38122735493086,-1.37773773384927,
-1.37373888475572,-1.36678226923295,-1.33266754457923,-1.27905923984327,
-1.26062970521329,-1.25656758957397,-1.25427610557754,-1.25231392102026,
-1.24977065231729,-1.24435057700418,-1.20064947555576,-1.14488351546687,
-1.1351050407246,-1.13058685891227,-1.1270681467531,-1.12322725200407,-1.11699639170761,
-1.09415043676683,-1.05417258885683,-1.01333443966294,-1.0068962700886,
-1.00436392221548,-1.00252652364608,-1.00048635198209,-0.997462188138732,
-0.989068854014529,-0.975890169613667,-0.938614078903735,-0.889984451129513,
-0.883300572107022,-0.878975723789251,-0.875486218612126,-0.871487484358028,
-0.864531022016475,-0.830415817385973,-0.776794804848949,-0.758380451001099,
-0.754319355211467,-0.752028147121937,-0.75006600050795,-0.747522523119937,
-0.742101083048869,-0.697144193570694,-0.64273914651985,-0.633021504888423,
-0.628446534665607,-0.624919573066694,-0.621105483888715,-0.614997317620162,
-0.593529695061223,-0.523171917700296,-0.506923580403083,-0.50300514422664,
-0.500746351216423,-0.498976348647329,-0.496493494002344,-0.491387295857933,
-0.484585700126944,-0.467463706225077,-0.416972038713945,-0.386891587004229,
-0.379985316746016,-0.375957271575916,-0.372470138009076,-0.368183977833826,
-0.359857332809512,-0.308097725810674,-0.259426865680415,-0.253290154277052,
-0.250589983140797,-0.248631522338408,-0.248546394839057,-0.248480095286316,
-0.248434302691515,-0.248401216776203,-0.248356785540407,-0.248314849649355,
-0.248275051527834,-0.24823709904409,-0.248200750116737,-0.248165801610515,
-0.24813208113155,-0.248099440884787,-0.248067752982383,-0.2480369058037,
-0.248006801144657,-0.247977351956688,-0.247948480520079,-0.247920116975015,
-0.247892198115205,-0.247864666392897,-0.247837469092272,-0.247810557626377,
-0.247783886950667,-0.247757415076964,-0.247731102636315,-0.247704912507719,
-0.247678809502094,-0.247652760086345,-0.245124567611522,-0.239610186869502,
-0.194140884841972,-0.140430070911066,-0.131537338139361,-0.127070658394206,
-0.123786806840283,-0.120221209184394,-0.115328872331299,-0.103686018322656,
-0.0900938466068125),.UNSPECIFIED.);
#274=B_SPLINE_CURVE_WITH_KNOTS('',3,(#18125,#18126,#18127,#18128,#18129,
#18130,#18131,#18132,#18133,#18134,#18135,#18136,#18137,#18138,#18139,#18140,
#18141,#18142,#18143,#18144,#18145,#18146,#18147,#18148,#18149,#18150,#18151,
#18152,#18153,#18154,#18155,#18156,#18157,#18158,#18159,#18160,#18161,#18162,
#18163,#18164,#18165,#18166,#18167,#18168,#18169,#18170,#18171,#18172,#18173,
#18174,#18175,#18176,#18177,#18178,#18179,#18180,#18181,#18182,#18183,#18184,
#18185,#18186,#18187,#18188,#18189,#18190,#18191,#18192,#18193,#18194,#18195,
#18196,#18197,#18198,#18199,#18200,#18201,#18202,#18203,#18204,#18205,#18206,
#18207,#18208,#18209,#18210,#18211,#18212,#18213,#18214,#18215,#18216,#18217,
#18218,#18219,#18220,#18221,#18222,#18223,#18224,#18225,#18226,#18227,#18228,
#18229,#18230,#18231,#18232,#18233,#18234,#18235,#18236,#18237,#18238,#18239,
#18240,#18241,#18242,#18243,#18244,#18245,#18246,#18247,#18248,#18249,#18250,
#18251,#18252,#18253,#18254,#18255,#18256,#18257,#18258,#18259,#18260,#18261,
#18262,#18263,#18264,#18265,#18266,#18267,#18268,#18269,#18270,#18271,#18272,
#18273,#18274,#18275,#18276,#18277,#18278,#18279,#18280,#18281,#18282,#18283,
#18284,#18285,#18286,#18287,#18288,#18289,#18290,#18291,#18292,#18293,#18294,
#18295,#18296,#18297,#18298,#18299,#18300,#18301,#18302,#18303,#18304,#18305),
 .UNSPECIFIED.,.F.,.F.,(4,3,3,3,3,3,3,3,3,3,3,3,3,3,3,3,3,3,3,3,3,3,3,3,
3,3,3,3,3,3,3,3,3,3,3,3,3,3,3,3,3,3,3,3,3,3,3,3,3,3,3,3,3,3,3,3,3,3,3,3,
4),(64.494741390819,64.5971431881403,64.6789776427348,64.7780367603194,
64.8769554345788,64.9765908599113,65.0753328612621,65.1740423880121,65.2727492259639,
65.3730716287825,65.471920222143,65.5729795296907,65.6740388372384,65.7730979548231,
65.8720166290825,65.9716520544149,66.0703940557658,66.1691035825159,66.2678104204676,
66.3681328232862,66.4669814166466,66.5680407241943,66.669100031742,66.7681591493267,
66.8670778235862,66.9667132489186,67.0654552502695,67.1641647770195,67.2628716149714,
67.36319401779,67.4620426111503,67.563101918698,67.6641612262456,67.7632203438303,
67.8621390180899,67.9617744434223,68.0605164447731,68.1592259715231,68.257932809475,
68.3582552122935,68.457103805654,68.5581631132016,68.6592224207492,68.7582815383338,
68.8572002125931,68.9568356379256,69.0555776392764,69.1542871660265,69.252994003978,
69.3533164067967,69.4521650001572,69.553224307705,69.6542836152528,69.7520048359883,
69.8496009043765,69.9471033152915,70.0445434457333,70.1419872142467,70.239427096225,
70.3369604616554,70.4246015196188),.UNSPECIFIED.);
#275=B_SPLINE_CURVE_WITH_KNOTS('',3,(#18306,#18307,#18308,#18309,#18310,
#18311,#18312,#18313,#18314,#18315,#18316,#18317,#18318),.UNSPECIFIED.,
 .F.,.F.,(4,3,3,3,4),(70.4246015199525,70.558216925384,70.6493448097564,
70.7484011637564,70.7790859150367),.UNSPECIFIED.);
#276=B_SPLINE_CURVE_WITH_KNOTS('',3,(#18320,#18321,#18322,#18323,#18324,
#18325,#18326,#18327,#18328,#18329,#18330,#18331),.UNSPECIFIED.,.F.,.F.,
(4,2,2,2,2,4),(-0.0900938466068125,-0.0674452343315531,-0.0150635790955834,
-0.00474487467251724,-0.00202527891974473,-0.000735711368292737),
 .UNSPECIFIED.);
#277=B_SPLINE_CURVE_WITH_KNOTS('',3,(#18332,#18333,#18334,#18335,#18336,
#18337,#18338,#18339,#18340,#18341,#18342,#18343,#18344,#18345,#18346,#18347,
#18348,#18349,#18350,#18351,#18352,#18353,#18354,#18355,#18356,#18357,#18358,
#18359,#18360,#18361,#18362,#18363,#18364,#18365,#18366,#18367,#18368,#18369,
#18370,#18371,#18372,#18373,#18374,#18375,#18376,#18377,#18378,#18379,#18380,
#18381,#18382,#18383,#18384,#18385,#18386,#18387,#18388,#18389,#18390,#18391,
#18392,#18393,#18394,#18395,#18396,#18397,#18398,#18399,#18400,#18401,#18402,
#18403,#18404,#18405,#18406,#18407,#18408,#18409,#18410,#18411,#18412,#18413,
#18414,#18415,#18416,#18417,#18418,#18419,#18420,#18421,#18422,#18423,#18424,
#18425,#18426,#18427,#18428,#18429,#18430,#18431,#18432,#18433,#18434,#18435,
#18436,#18437,#18438,#18439,#18440,#18441,#18442,#18443,#18444,#18445,#18446,
#18447,#18448,#18449,#18450,#18451,#18452,#18453,#18454,#18455,#18456,#18457,
#18458,#18459,#18460,#18461,#18462,#18463,#18464,#18465,#18466,#18467,#18468,
#18469,#18470,#18471,#18472,#18473,#18474,#18475,#18476,#18477,#18478,#18479,
#18480,#18481,#18482,#18483,#18484,#18485,#18486,#18487,#18488,#18489,#18490,
#18491,#18492,#18493,#18494,#18495,#18496,#18497,#18498,#18499,#18500,#18501,
#18502,#18503,#18504,#18505,#18506,#18507,#18508,#18509,#18510,#18511,#18512,
#18513,#18514,#18515,#18516,#18517,#18518,#18519,#18520,#18521,#18522,#18523,
#18524,#18525,#18526,#18527,#18528,#18529),.UNSPECIFIED.,.F.,.F.,(4,2,2,
2,2,2,2,2,2,2,2,2,2,2,2,2,2,2,2,2,2,2,2,2,2,2,2,2,2,2,2,2,2,2,2,2,2,2,2,
2,2,2,2,2,2,2,2,2,2,2,2,2,2,2,2,2,2,2,2,2,2,2,2,2,2,2,2,2,2,2,2,2,2,2,2,
2,2,2,2,2,2,2,2,2,2,2,2,2,2,2,2,2,2,2,2,2,2,2,4),(-3.17281145082706,-3.17188027035177,
-3.17011455900862,-3.16814177566368,-3.16536628592734,-3.15874480285747,
-3.15220734656136,-3.10107551468508,-3.06396462670712,-3.05229874038881,
-3.04740198696655,-3.04383505388989,-3.04055129370548,-3.03608676995585,
-3.02720478086407,-2.97321112537944,-2.9403159161049,-2.92508434746351,
-2.9223517896374,-2.91989294767224,-2.91796885123375,-2.91567095303065,
-2.91165945767271,-2.89355018091552,-2.82498478813721,-2.8108738051289,
-2.80050696065795,-2.79583260004176,-2.7923022345682,-2.78849601899172,
-2.78242566322933,-2.76338309446505,-2.69540674641322,-2.68133621198321,
-2.67253820728772,-2.66945904008345,-2.66740713480705,-2.66557876538935,
-2.66308337399262,-2.65686647058534,-2.60936117063643,-2.57254067602311,
-2.55910703345573,-2.54912373534732,-2.54451843205932,-2.54099786332001,
-2.53716081099802,-2.53094935906433,-2.5106642423816,-2.45128072817204,
-2.43258150088448,-2.42186218796596,-2.41855062813285,-2.41644837588608,
-2.41444303680745,-2.41196504279072,-2.40584956329628,-2.35672826458412,
-2.30473691496518,-2.29676401322865,-2.29254987678195,-2.28940496931344,
-2.28544258395633,-2.27865582592454,-2.2517194580498,-2.19877863104351,
-2.18097230430283,-2.17399163084602,-2.16878106314646,-2.16627774498469,
-2.16450522136393,-2.16225978498189,-2.15840015819994,-2.1429358618492,
-2.0975776506416,-2.05401530361326,-2.04578419546068,-2.04151720767012,
-2.03803089221701,-2.03398719957246,-2.02701269506793,-1.99567387081475,
-1.94591795336698,-1.92125799155268,-1.91702303195283,-1.91471858844261,
-1.91275776866927,-1.91023236524179,-1.90611705058611,-1.87501721898451,
-1.82536639610872,-1.79974373585842,-1.79329110579242,-1.78940152535256,
-1.78589457133846,-1.78139417962398,-1.7719744872921,-1.71154169179078,
-1.67612525783103),.UNSPECIFIED.);
#278=B_SPLINE_CURVE_WITH_KNOTS('',3,(#18535,#18536,#18537,#18538,#18539,
#18540,#18541,#18542,#18543,#18544,#18545,#18546,#18547,#18548,#18549,#18550,
#18551,#18552,#18553,#18554,#18555,#18556,#18557,#18558,#18559,#18560,#18561,
#18562,#18563,#18564,#18565,#18566,#18567,#18568,#18569,#18570,#18571,#18572,
#18573,#18574,#18575,#18576,#18577,#18578,#18579,#18580,#18581,#18582,#18583,
#18584,#18585,#18586,#18587,#18588,#18589,#18590,#18591,#18592,#18593,#18594,
#18595,#18596,#18597,#18598,#18599,#18600,#18601,#18602,#18603,#18604,#18605,
#18606,#18607,#18608,#18609,#18610,#18611,#18612,#18613,#18614,#18615,#18616,
#18617,#18618,#18619,#18620,#18621,#18622,#18623,#18624,#18625,#18626,#18627,
#18628,#18629,#18630,#18631,#18632,#18633,#18634,#18635,#18636,#18637,#18638,
#18639,#18640,#18641,#18642,#18643,#18644,#18645,#18646,#18647,#18648,#18649,
#18650,#18651,#18652,#18653,#18654,#18655,#18656,#18657,#18658,#18659,#18660,
#18661,#18662,#18663,#18664,#18665,#18666,#18667,#18668,#18669,#18670,#18671,
#18672,#18673,#18674,#18675,#18676,#18677,#18678,#18679,#18680,#18681,#18682,
#18683,#18684,#18685,#18686,#18687,#18688,#18689,#18690,#18691,#18692,#18693,
#18694,#18695,#18696,#18697,#18698,#18699,#18700,#18701,#18702,#18703,#18704,
#18705,#18706,#18707,#18708,#18709,#18710,#18711,#18712,#18713,#18714,#18715),
 .UNSPECIFIED.,.F.,.F.,(4,3,3,3,3,3,3,3,3,3,3,3,3,3,3,3,3,3,3,3,3,3,3,3,
3,3,3,3,3,3,3,3,3,3,3,3,3,3,3,3,3,3,3,3,3,3,3,3,3,3,3,3,3,3,3,3,3,3,3,3,
4),(58.2125415401659,58.3098255944961,58.4095218148003,58.506928276048,
58.6077693758806,58.7086104757131,58.8076695932977,58.9065882675571,59.0062236928895,
59.1049656942404,59.2036752209903,59.302382058942,59.4027044617607,59.5015530551212,
59.602612362669,59.7036716702167,59.8027307878014,59.901649462061,60.0012848873934,
60.1000268887443,60.1987364154943,60.297443253446,60.3977656562646,60.4966142496251,
60.5976735571727,60.6987328647203,60.7977919823049,60.8967106565642,60.9963460818967,
61.0950880832477,61.1937976099976,61.2925044479492,61.3928268507679,61.4916754441283,
61.5927347516761,61.6937940592239,61.7928531768085,61.891771851068,61.9914072764005,
62.0901492777514,62.1888588045013,62.287565642453,62.3878880452717,62.4867366386322,
62.5877959461799,62.6888552537275,62.787914371312,62.886833045571,62.9864684709035,
63.0852104722542,63.1839199990042,63.2826268369558,63.3829492397746,63.4817978331351,
63.5828571406831,63.6839164482311,63.790091202586,63.8959105065078,64.0015055025796,
64.1067929756919,64.1414162124289),.UNSPECIFIED.);
#279=B_SPLINE_CURVE_WITH_KNOTS('',3,(#18716,#18717,#18718,#18719,#18720,
#18721,#18722,#18723,#18724,#18725,#18726,#18727,#18728),.UNSPECIFIED.,
 .F.,.F.,(4,3,3,3,4),(64.1414162127729,64.2432632342092,64.3451869563365,
64.4472800563271,64.494741390819),.UNSPECIFIED.);
#280=B_SPLINE_CURVE_WITH_KNOTS('',3,(#18729,#18730,#18731,#18732,#18733,
#18734,#18735,#18736,#18737,#18738,#18739,#18740,#18741,#18742,#18743,#18744,
#18745,#18746,#18747,#18748,#18749,#18750,#18751,#18752,#18753,#18754,#18755,
#18756,#18757,#18758,#18759,#18760,#18761,#18762,#18763,#18764,#18765,#18766,
#18767,#18768,#18769,#18770,#18771,#18772,#18773,#18774,#18775,#18776,#18777,
#18778,#18779,#18780,#18781,#18782,#18783,#18784,#18785,#18786,#18787,#18788,
#18789,#18790,#18791,#18792,#18793,#18794,#18795,#18796,#18797,#18798,#18799,
#18800,#18801,#18802,#18803,#18804,#18805,#18806,#18807,#18808,#18809,#18810,
#18811,#18812,#18813,#18814,#18815,#18816,#18817,#18818,#18819,#18820,#18821,
#18822,#18823,#18824,#18825,#18826,#18827,#18828,#18829,#18830,#18831,#18832,
#18833,#18834,#18835,#18836,#18837,#18838,#18839,#18840,#18841,#18842,#18843,
#18844,#18845,#18846,#18847,#18848,#18849,#18850,#18851,#18852,#18853,#18854,
#18855,#18856,#18857,#18858,#18859,#18860,#18861,#18862,#18863,#18864,#18865,
#18866,#18867,#18868,#18869,#18870,#18871,#18872,#18873,#18874,#18875,#18876,
#18877,#18878,#18879,#18880,#18881,#18882,#18883,#18884,#18885,#18886,#18887,
#18888,#18889,#18890,#18891,#18892,#18893,#18894,#18895,#18896,#18897,#18898,
#18899,#18900,#18901,#18902,#18903,#18904,#18905,#18906,#18907,#18908,#18909,
#18910,#18911,#18912,#18913,#18914,#18915,#18916,#18917,#18918,#18919,#18920,
#18921,#18922,#18923,#18924,#18925,#18926,#18927,#18928,#18929,#18930,#18931,
#18932,#18933,#18934,#18935,#18936,#18937,#18938,#18939,#18940,#18941,#18942,
#18943,#18944,#18945,#18946,#18947,#18948,#18949,#18950,#18951,#18952,#18953,
#18954,#18955,#18956,#18957,#18958,#18959,#18960,#18961,#18962),
 .UNSPECIFIED.,.F.,.F.,(4,2,2,2,2,2,2,2,2,2,2,2,2,2,2,2,2,2,2,2,2,2,2,2,
2,2,2,2,2,2,2,2,2,2,2,2,2,2,2,2,2,2,2,2,2,2,2,2,2,2,2,2,2,2,2,2,2,2,2,2,
2,2,2,2,2,2,2,2,2,2,2,2,2,2,2,2,2,2,2,2,2,2,2,2,2,2,2,2,2,2,2,2,2,2,2,2,
2,2,2,2,2,2,2,2,2,2,2,2,2,2,2,2,2,2,2,2,4),(-1.67612525783103,-1.67174155907941,
-1.66648156089626,-1.66396868833182,-1.66200878639615,-1.65969506490472,
-1.65553511836417,-1.63540930721214,-1.62791510237671,-1.58699491302144,
-1.55012914773024,-1.54355213901721,-1.53925941060774,-1.53577151944839,
-1.53174770444095,-1.52467686017826,-1.4879475655404,-1.43011326387354,
-1.41778899611528,-1.41417614708776,-1.41200731945494,-1.41001406766565,
-1.4072399095018,-1.40051159009237,-1.39075243572799,-1.36026795863329,
-1.30278664947792,-1.29310955289729,-1.28860944621497,-1.28509274360082,
-1.28124178547242,-1.27496683694818,-1.25160834000514,-1.20998964578862,
-1.17140470168752,-1.16494154608508,-1.16240479488504,-1.1605660603719,
-1.15852664402118,-1.15550740738203,-1.14715219810917,-1.13405737329597,
-1.09653663451939,-1.04799751253387,-1.04131266115002,-1.03698710189031,
-1.03349697003164,-1.02949745947286,-1.02253949583949,-0.988412944134841,
-0.934735496039016,-0.916364898014789,-0.91230593754306,-0.910014964838313,
-0.908052377271597,-0.905507492527266,-0.900080067987926,-0.892720579479789,
-0.873418276659511,-0.808250294851859,-0.793223255264992,-0.787662671944456,
-0.784335242298483,-0.780797485085342,-0.776074978341524,-0.765435754157361,
-0.750838630810988,-0.708071731289013,-0.669041224697704,-0.662597791203747,
-0.660064384195309,-0.658226564648076,-0.65618634450042,-0.653162822247264,
-0.644775864418675,-0.631611716705835,-0.594313695712995,-0.545669150698194,
-0.538984390849457,-0.534658983050692,-0.531169033245429,-0.527169796921197,
-0.520212480438021,-0.486093596738575,-0.432471748943184,-0.41404901850279,
-0.409987038857585,-0.407695456099797,-0.405733070753092,-0.403189390685247,
-0.397767899600971,-0.353325302359996,-0.298385286632885,-0.288670657109038,
-0.284095927751782,-0.280568643134865,-0.280263529789934,-0.280127193369226,
-0.280024732261122,-0.279947873131842,-0.279890296579403,-0.27981037236961,
-0.279735201254423,-0.275740057189021,-0.27146445934223,-0.264857510107381,
-0.252288982215485,-0.219383292098332,-0.165732596392655,-0.15990316160231,
-0.157505808860149,-0.155521027524159,-0.153383949837367,-0.149913837214301,
-0.137656752234916,-0.114724389595725,-0.0901916154543634),
 .UNSPECIFIED.);
#281=B_SPLINE_CURVE_WITH_KNOTS('',3,(#18968,#18969,#18970,#18971,#18972,
#18973,#18974,#18975,#18976,#18977,#18978,#18979,#18980,#18981,#18982,#18983,
#18984,#18985,#18986,#18987,#18988,#18989,#18990,#18991,#18992,#18993,#18994,
#18995,#18996,#18997,#18998,#18999,#19000,#19001,#19002,#19003,#19004,#19005,
#19006,#19007,#19008,#19009,#19010,#19011,#19012,#19013,#19014,#19015,#19016,
#19017,#19018,#19019,#19020,#19021,#19022,#19023,#19024,#19025,#19026,#19027,
#19028,#19029,#19030,#19031,#19032,#19033,#19034,#19035,#19036,#19037,#19038,
#19039,#19040,#19041,#19042,#19043,#19044,#19045,#19046,#19047,#19048,#19049,
#19050,#19051,#19052,#19053,#19054,#19055,#19056,#19057,#19058,#19059,#19060,
#19061,#19062,#19063,#19064,#19065,#19066,#19067,#19068,#19069,#19070,#19071,
#19072,#19073,#19074,#19075,#19076,#19077,#19078,#19079,#19080,#19081,#19082,
#19083,#19084,#19085,#19086,#19087,#19088,#19089,#19090,#19091,#19092,#19093,
#19094,#19095,#19096,#19097,#19098,#19099,#19100,#19101,#19102,#19103,#19104,
#19105,#19106,#19107,#19108,#19109,#19110,#19111,#19112,#19113,#19114,#19115,
#19116,#19117,#19118,#19119,#19120,#19121,#19122,#19123,#19124,#19125,#19126,
#19127,#19128,#19129,#19130,#19131,#19132,#19133,#19134,#19135,#19136,#19137,
#19138,#19139,#19140,#19141,#19142,#19143,#19144,#19145,#19146,#19147,#19148),
 .UNSPECIFIED.,.F.,.F.,(4,3,3,3,3,3,3,3,3,3,3,3,3,3,3,3,3,3,3,3,3,3,3,3,
3,3,3,3,3,3,3,3,3,3,3,3,3,3,3,3,3,3,3,3,3,3,3,3,3,3,3,3,3,3,3,3,3,3,3,3,
4),(51.9295993767367,52.030679868231,52.1294268781299,52.2281383612316,
52.3268441060956,52.4296939067445,52.5285380981942,52.6274520266398,52.7265185872557,
52.7382433086914,52.8373024262761,52.9362211005355,53.0358565258679,53.1345985272188,
53.2333080539687,53.3320148919204,53.4323372947391,53.5311858880996,53.6322451956473,
53.733304503195,53.8323636207796,53.9312822950391,54.0309177203715,54.1296597217224,
54.2283692484723,54.327076086424,54.4273984892427,54.5262470826031,54.6273063901509,
54.7283656976986,54.8274248152833,54.9263434895427,55.0259789148752,55.1247209162261,
55.223430442976,55.3221372809278,55.4224596837464,55.5213082771069,55.6223675846546,
55.7234268922023,55.822486009787,55.9214046840465,56.0210401093789,56.1197821107298,
56.2184916374798,56.3171984754316,56.4175208782501,56.5163694716106,56.6174287791582,
56.7184880867059,56.8175472042906,56.9164658785501,57.0161013038825,57.1148433052334,
57.2135528319833,57.3122596699351,57.4125820727537,57.5114306661142,57.6124899736618,
57.7135492812095,57.8582309055933),.UNSPECIFIED.);
#282=B_SPLINE_CURVE_WITH_KNOTS('',3,(#19149,#19150,#19151,#19152,#19153,
#19154,#19155,#19156,#19157,#19158,#19159,#19160,#19161),.UNSPECIFIED.,
 .F.,.F.,(4,3,3,3,4),(57.8582309058197,57.9557212700061,58.0531125158964,
58.1504356450135,58.2125415401659),.UNSPECIFIED.);
#283=B_SPLINE_CURVE_WITH_KNOTS('',3,(#19163,#19164,#19165,#19166,#19167,
#19168,#19169,#19170,#19171,#19172,#19173,#19174,#19175,#19176,#19177,#19178,
#19179,#19180,#19181,#19182),.UNSPECIFIED.,.F.,.F.,(4,2,2,2,2,2,2,2,2,4),
(-0.0901916154543634,-0.0674014413990488,-0.0431045913887549,-0.0359174086979867,
-0.031825889082996,-0.0286630733899206,-0.0253644269643822,-0.0213655915020832,
-0.0130902425129321,-0.000734942023342333),.UNSPECIFIED.);
#284=B_SPLINE_CURVE_WITH_KNOTS('',3,(#19183,#19184,#19185,#19186,#19187,
#19188,#19189,#19190,#19191,#19192,#19193,#19194,#19195,#19196,#19197,#19198,
#19199,#19200,#19201,#19202,#19203,#19204,#19205,#19206,#19207,#19208,#19209,
#19210,#19211,#19212,#19213,#19214,#19215,#19216,#19217,#19218,#19219,#19220,
#19221,#19222,#19223,#19224,#19225,#19226,#19227,#19228,#19229,#19230,#19231,
#19232,#19233,#19234,#19235,#19236,#19237,#19238,#19239,#19240,#19241,#19242,
#19243,#19244,#19245,#19246,#19247,#19248,#19249,#19250,#19251,#19252,#19253,
#19254,#19255,#19256,#19257,#19258,#19259,#19260,#19261,#19262,#19263,#19264,
#19265,#19266,#19267,#19268,#19269,#19270,#19271,#19272,#19273,#19274,#19275,
#19276,#19277,#19278,#19279,#19280,#19281,#19282,#19283,#19284,#19285,#19286,
#19287,#19288,#19289,#19290,#19291,#19292,#19293,#19294,#19295,#19296,#19297,
#19298,#19299,#19300,#19301,#19302,#19303,#19304,#19305,#19306,#19307,#19308,
#19309,#19310,#19311,#19312,#19313,#19314,#19315,#19316,#19317,#19318,#19319,
#19320,#19321,#19322,#19323,#19324,#19325,#19326,#19327,#19328,#19329,#19330,
#19331,#19332,#19333,#19334,#19335,#19336,#19337,#19338,#19339,#19340,#19341,
#19342,#19343,#19344,#19345,#19346,#19347,#19348,#19349,#19350,#19351,#19352,
#19353,#19354,#19355,#19356,#19357,#19358,#19359,#19360,#19361,#19362,#19363,
#19364,#19365,#19366,#19367,#19368,#19369,#19370,#19371,#19372,#19373,#19374,
#19375,#19376,#19377,#19378,#19379,#19380,#19381,#19382,#19383,#19384,#19385,
#19386,#19387,#19388),.UNSPECIFIED.,.F.,.F.,(4,2,2,2,2,2,2,2,2,2,2,2,2,
2,2,2,2,2,2,2,2,2,2,2,2,2,2,2,2,2,2,2,2,2,2,2,2,2,2,2,2,2,2,2,2,2,2,2,2,
2,2,2,2,2,2,2,2,2,2,2,2,2,2,2,2,2,2,2,2,2,2,2,2,2,2,2,2,2,2,2,2,2,2,2,2,
2,2,2,2,2,2,2,2,2,2,2,2,2,2,2,2,2,4),(-3.17197906884703,-3.10233466004078,
-3.089202820326,-3.08083016006895,-3.0778087659958,-3.07576908159546,-3.07393104859413,
-3.07139643924237,-3.06494515748726,-3.0250064008028,-2.98434155349365,
-2.969062282852,-2.96149583078054,-2.95522557350808,-2.95145121181416,-2.94795203707633,
-2.94351945030074,-2.93445282117953,-2.87091017572828,-2.83390571702822,
-2.82849433722826,-2.82595265796583,-2.8239905392314,-2.82169780433466,
-2.81763037603098,-2.79911749706469,-2.74554947518647,-2.71143124425603,
-2.70447406319494,-2.70047504552521,-2.69698537465109,-2.69266042605793,
-2.68597665402958,-2.63734724162226,-2.60005378034847,-2.58691715724735,
-2.5785423167163,-2.57552063662163,-2.5734809049158,-2.57164294363849,-2.56910857842963,
-2.56265869954775,-2.52377639203534,-2.48087102576355,-2.45881671916317,
-2.45265493229194,-2.44882903076144,-2.44530566693922,-2.4407557949069,
-2.43080303020682,-2.37959668304745,-2.34968991379883,-2.33608719051898,
-2.32749975612256,-2.32444905958529,-2.32240334456791,-2.32057057596628,
-2.3180567157288,-2.31172952406076,-2.26675882142933,-2.22823420224264,
-2.21444975133346,-2.20426730008706,-2.19962628629593,-2.19610111206187,
-2.19228113815883,-2.18614633315895,-2.16651063085258,-2.10641258449006,
-2.0876653494613,-2.07692801989668,-2.07361479158612,-2.07151237925171,
-2.06950765985588,-2.06703124301668,-2.06092364659599,-2.01164170773385,
-1.98226238920811,-1.95708012101653,-1.95066083152453,-1.94677874952197,
-1.94327051996894,-1.93875725086566,-1.92926807521707,-1.86956606516565,
-1.84058779339195,-1.83111315372105,-1.82453252462884,-1.8217830304196,
-1.81979405219135,-1.81761531280894,-1.81395671970291,-1.8011863593112,
-1.78980566277747,-1.77194431229076,-1.72787970199721,-1.70550815978039,
-1.69931810463794,-1.69548595781237,-1.69196437054264,-1.68742732020908,
-1.67754594539564,-1.67566955000462),.UNSPECIFIED.);
#285=B_SPLINE_CURVE_WITH_KNOTS('',3,(#19394,#19395,#19396,#19397,#19398,
#19399,#19400,#19401,#19402,#19403,#19404,#19405,#19406,#19407,#19408,#19409,
#19410,#19411,#19412,#19413,#19414,#19415,#19416,#19417,#19418,#19419,#19420,
#19421,#19422,#19423,#19424,#19425,#19426,#19427,#19428,#19429,#19430,#19431,
#19432,#19433,#19434,#19435,#19436,#19437,#19438,#19439,#19440,#19441,#19442,
#19443,#19444,#19445,#19446,#19447,#19448,#19449,#19450,#19451,#19452,#19453,
#19454,#19455,#19456,#19457,#19458,#19459,#19460,#19461,#19462,#19463,#19464,
#19465,#19466,#19467,#19468,#19469,#19470,#19471,#19472,#19473,#19474,#19475,
#19476,#19477,#19478,#19479,#19480,#19481,#19482,#19483,#19484,#19485,#19486,
#19487,#19488,#19489,#19490,#19491,#19492,#19493,#19494,#19495,#19496,#19497,
#19498,#19499,#19500,#19501,#19502,#19503,#19504,#19505,#19506,#19507,#19508,
#19509,#19510,#19511,#19512,#19513,#19514,#19515,#19516,#19517,#19518,#19519,
#19520,#19521,#19522,#19523,#19524,#19525,#19526,#19527,#19528,#19529,#19530,
#19531,#19532,#19533,#19534,#19535,#19536,#19537,#19538,#19539,#19540,#19541,
#19542,#19543,#19544,#19545,#19546,#19547,#19548,#19549,#19550,#19551,#19552,
#19553,#19554,#19555,#19556,#19557,#19558,#19559,#19560,#19561,#19562,#19563,
#19564,#19565,#19566,#19567,#19568,#19569,#19570,#19571,#19572,#19573,#19574,
#19575,#19576,#19577),.UNSPECIFIED.,.F.,.F.,(4,3,3,3,3,3,3,3,3,3,3,3,3,
3,3,3,3,3,3,3,3,3,3,3,3,3,3,3,3,3,3,3,3,3,3,3,3,3,3,3,3,3,3,3,3,3,3,3,3,
3,3,3,3,3,3,3,3,3,3,3,3,4),(45.6452617210371,45.7501727111588,45.7728149471661,
45.8718740647507,45.9707927390101,46.0704281643426,46.1691701656934,46.2678796924433,
46.3665865303951,46.4669089332138,46.5657575265742,46.666816834122,46.7678761416697,
46.8669352592544,46.9658539335139,47.0654893588463,47.1642313601972,47.2629408869472,
47.361647724899,47.4619701277176,47.5608187210781,47.6618780286258,47.7629373361734,
47.8619964537581,47.9609151280175,48.0605505533499,48.1592925547008,48.2580020814507,
48.3567089194025,48.4570313222211,48.5558799155816,48.6569392231293,48.757998530677,
48.8570576482616,48.955976322521,49.0556117478535,49.1543537492043,49.2530632759542,
49.351770113906,49.4520925167247,49.5509411100851,49.6520004176329,49.7530597251806,
49.8521188427653,49.9510375170247,50.0506729423571,50.149414943708,50.2481244704579,
50.3468313084097,50.4471537112284,50.5460023045888,50.6470616121365,50.7481209196842,
50.8457129935021,50.9431428324126,51.0404816382021,51.1377609277277,51.2350121400979,
51.3323110164863,51.4296360130142,51.5270774501447,51.5750455980568),
 .UNSPECIFIED.);
#286=B_SPLINE_CURVE_WITH_KNOTS('',3,(#19578,#19579,#19580,#19581,#19582,
#19583,#19584,#19585,#19586,#19587,#19588,#19589,#19590),.UNSPECIFIED.,
 .F.,.F.,(4,3,3,3,4),(51.5750455984137,51.7300295918744,51.7431821141878,
51.842215157546,51.9295993767367),.UNSPECIFIED.);
#287=B_SPLINE_CURVE_WITH_KNOTS('',3,(#19591,#19592,#19593,#19594,#19595,
#19596,#19597,#19598,#19599,#19600,#19601,#19602,#19603,#19604,#19605,#19606,
#19607,#19608,#19609,#19610,#19611,#19612,#19613,#19614,#19615,#19616,#19617,
#19618,#19619,#19620,#19621,#19622,#19623,#19624,#19625,#19626,#19627,#19628,
#19629,#19630,#19631,#19632,#19633,#19634,#19635,#19636,#19637,#19638,#19639,
#19640,#19641,#19642,#19643,#19644,#19645,#19646,#19647,#19648,#19649,#19650,
#19651,#19652,#19653,#19654,#19655,#19656,#19657,#19658,#19659,#19660,#19661,
#19662,#19663,#19664,#19665,#19666,#19667,#19668,#19669,#19670,#19671,#19672,
#19673,#19674,#19675,#19676,#19677,#19678,#19679,#19680,#19681,#19682,#19683,
#19684,#19685,#19686,#19687,#19688,#19689,#19690,#19691,#19692,#19693,#19694,
#19695,#19696,#19697,#19698,#19699,#19700,#19701,#19702,#19703,#19704,#19705,
#19706,#19707,#19708,#19709,#19710,#19711,#19712,#19713,#19714,#19715,#19716,
#19717,#19718,#19719,#19720,#19721,#19722,#19723,#19724,#19725,#19726,#19727,
#19728,#19729,#19730,#19731,#19732,#19733,#19734,#19735,#19736,#19737,#19738,
#19739,#19740,#19741,#19742,#19743,#19744,#19745,#19746,#19747,#19748,#19749,
#19750,#19751,#19752,#19753,#19754,#19755,#19756,#19757,#19758,#19759,#19760,
#19761,#19762,#19763,#19764,#19765,#19766,#19767,#19768,#19769,#19770,#19771,
#19772,#19773,#19774,#19775,#19776,#19777,#19778,#19779,#19780,#19781,#19782,
#19783,#19784,#19785,#19786,#19787,#19788,#19789,#19790,#19791,#19792,#19793,
#19794,#19795,#19796,#19797,#19798,#19799,#19800),.UNSPECIFIED.,.F.,.F.,
(4,2,2,2,2,2,2,2,2,2,2,2,2,2,2,2,2,2,2,2,2,2,2,2,2,2,2,2,2,2,2,2,2,2,2,
2,2,2,2,2,2,2,2,2,2,2,2,2,2,2,2,2,2,2,2,2,2,2,2,2,2,2,2,2,2,2,2,2,2,2,2,
2,2,2,2,2,2,2,2,2,2,2,2,2,2,2,2,2,2,2,2,2,2,2,2,2,2,2,2,2,2,2,2,2,4),(-1.67566955000462,
-1.62411491162083,-1.60674415883351,-1.58623055946249,-1.57503720608005,
-1.57154768364484,-1.56940633036676,-1.56740097292286,-1.56455629235962,
-1.55738628313311,-1.54675921648381,-1.5112589881279,-1.46074593018652,
-1.4507750026778,-1.44622171730574,-1.44269772364112,-1.43887314646134,
-1.43271793382074,-1.41073790447629,-1.3681008033436,-1.3288992828815,-1.32245896173317,
-1.31992615367768,-1.31808855393356,-1.3160483189293,-1.3130243337789,-1.30463325217463,
-1.29145983491177,-1.25417454372432,-1.20553814664101,-1.19885378435457,
-1.19452862728413,-1.19103887555055,-1.18703986156701,-1.18008291986628,
-1.14596555666727,-1.09234301715617,-1.07392508799704,-1.0698635670663,
-1.06757216588501,-1.06560988488886,-1.06306627358454,-1.05764469179629,
-1.01288069432577,-0.958261093183116,-0.948551928914253,-0.943978409472746,
-0.9404514681725,-0.936636312780529,-0.930524050795131,-0.909015149970924,
-0.838288406454097,-0.822399702657275,-0.818507573102457,-0.816254703494791,
-0.814483558449131,-0.811991575260142,-0.806839205561288,-0.79995834299321,
-0.782534985482966,-0.73147080004639,-0.702309511062795,-0.695455624195293,
-0.691439289955971,-0.687950927486531,-0.683648711071536,-0.675243445917033,
-0.62915881384798,-0.578652117622415,-0.569791322604171,-0.566602315316714,
-0.564733098986074,-0.562721715518813,-0.559844891891954,-0.55246797125806,
-0.541425267082822,-0.503271993686869,-0.456142650631887,-0.446146552816527,
-0.441588513029076,-0.438063587498571,-0.43424073841388,-0.428094367904544,
-0.4062162620152,-0.363944647654126,-0.324250480498227,-0.317808583247715,
-0.315275397716622,-0.31343760739642,-0.311397261223514,-0.30837328233016,
-0.299983319833441,-0.286812744540177,-0.230838151453552,-0.21565229953022,
-0.19802124651622,-0.192118292723605,-0.188348355919944,-0.184803732176448,
-0.181320715284496,-0.17349963142948,-0.140472726878903,-0.10990709668926,
-0.0921187839005196,-0.0898458279024645),.UNSPECIFIED.);
#288=B_SPLINE_CURVE_WITH_KNOTS('',3,(#19806,#19807,#19808,#19809,#19810,
#19811,#19812,#19813,#19814,#19815,#19816,#19817,#19818,#19819,#19820,#19821,
#19822,#19823,#19824,#19825,#19826,#19827,#19828,#19829,#19830,#19831,#19832,
#19833,#19834,#19835,#19836,#19837,#19838,#19839,#19840,#19841,#19842,#19843,
#19844,#19845,#19846,#19847,#19848,#19849,#19850,#19851,#19852,#19853,#19854,
#19855,#19856,#19857,#19858,#19859,#19860,#19861,#19862,#19863,#19864,#19865,
#19866,#19867,#19868,#19869,#19870,#19871,#19872,#19873,#19874,#19875,#19876,
#19877,#19878,#19879,#19880,#19881,#19882,#19883,#19884,#19885,#19886,#19887,
#19888,#19889,#19890,#19891,#19892,#19893,#19894,#19895,#19896,#19897,#19898,
#19899,#19900,#19901,#19902,#19903,#19904,#19905,#19906,#19907,#19908,#19909,
#19910,#19911,#19912,#19913,#19914,#19915,#19916,#19917,#19918,#19919,#19920,
#19921,#19922,#19923,#19924,#19925,#19926,#19927,#19928,#19929,#19930,#19931,
#19932,#19933,#19934,#19935,#19936,#19937,#19938,#19939,#19940,#19941,#19942,
#19943,#19944,#19945,#19946,#19947,#19948,#19949,#19950,#19951,#19952,#19953,
#19954,#19955,#19956,#19957,#19958,#19959,#19960,#19961,#19962,#19963,#19964,
#19965,#19966,#19967,#19968,#19969,#19970,#19971,#19972,#19973,#19974,#19975,
#19976,#19977,#19978,#19979,#19980,#19981,#19982,#19983,#19984,#19985,#19986),
 .UNSPECIFIED.,.F.,.F.,(4,3,3,3,3,3,3,3,3,3,3,3,3,3,3,3,3,3,3,3,3,3,3,3,
3,3,3,3,3,3,3,3,3,3,3,3,3,3,3,3,3,3,3,3,3,3,3,3,3,3,3,3,3,3,3,3,3,3,3,3,
4),(39.3627720041259,39.4600899844457,39.5575043562114,39.6549724183856,
39.752599552229,39.8024477801445,39.9015068977291,40.0004255719885,40.1000609973209,
40.1988029986718,40.2975125254217,40.3962193633734,40.4965417661921,40.5953903595525,
40.6964496671003,40.7975089746481,40.8965680922327,40.995486766492,41.0951221918245,
41.1938641931753,41.2925737199253,41.3912805578772,41.4916029606958,41.5904515540563,
41.691510861604,41.7925701691517,41.8916292867364,41.990547960996,42.0901833863284,
42.1889253876793,42.2876349144293,42.3863417523808,42.4866641551994,42.58551274856,
42.6865720561076,42.7876313636553,42.8866904812401,42.9856091554995,43.0852445808319,
43.1839865821829,43.2826961089329,43.3814029468845,43.4817253497031,43.5805739430635,
43.6816332506112,43.7826925581589,43.8817516757435,43.9806703500029,44.0803057753354,
44.1790477766862,44.2777573034362,44.376464141388,44.4767865442066,44.5756351375672,
44.6766944451148,44.7777537526625,44.8811334637464,44.9842446946408,45.0871977961317,
45.1899571772782,45.2918602912341),.UNSPECIFIED.);
#289=B_SPLINE_CURVE_WITH_KNOTS('',3,(#19987,#19988,#19989,#19990,#19991,
#19992,#19993,#19994,#19995,#19996,#19997,#19998,#19999),.UNSPECIFIED.,
 .F.,.F.,(4,3,3,3,4),(45.2918602914992,45.3960300356268,45.5003580442835,
45.6049490187659,45.6452617210371),.UNSPECIFIED.);
#290=B_SPLINE_CURVE_WITH_KNOTS('',3,(#20001,#20002,#20003,#20004,#20005,
#20006,#20007,#20008,#20009,#20010,#20011,#20012,#20013,#20014,#20015,#20016,
#20017,#20018,#20019,#20020),.UNSPECIFIED.,.F.,.F.,(4,2,2,2,2,2,2,2,2,4),
(-0.0898458279024645,-0.0696861600915073,-0.0657796954558397,-0.0633168309216045,
-0.0613600445003724,-0.0590069121563804,-0.0564756214434564,-0.0524233687460561,
-0.044365270485274,-0.000735688467659968),.UNSPECIFIED.);
#291=B_SPLINE_CURVE_WITH_KNOTS('',3,(#20021,#20022,#20023,#20024,#20025,
#20026,#20027,#20028,#20029,#20030,#20031,#20032,#20033,#20034,#20035,#20036,
#20037,#20038,#20039,#20040,#20041,#20042,#20043,#20044,#20045,#20046,#20047,
#20048,#20049,#20050,#20051,#20052,#20053,#20054,#20055,#20056,#20057,#20058,
#20059,#20060,#20061,#20062,#20063,#20064,#20065,#20066,#20067,#20068,#20069,
#20070,#20071,#20072,#20073,#20074,#20075,#20076,#20077,#20078,#20079,#20080,
#20081,#20082,#20083,#20084,#20085,#20086,#20087,#20088,#20089,#20090,#20091,
#20092,#20093,#20094,#20095,#20096,#20097,#20098,#20099,#20100,#20101,#20102,
#20103,#20104,#20105,#20106,#20107,#20108,#20109,#20110,#20111,#20112,#20113,
#20114,#20115,#20116,#20117,#20118,#20119,#20120,#20121,#20122,#20123,#20124,
#20125,#20126,#20127,#20128,#20129,#20130,#20131,#20132,#20133,#20134,#20135,
#20136,#20137,#20138,#20139,#20140,#20141,#20142,#20143,#20144,#20145,#20146,
#20147,#20148,#20149,#20150,#20151,#20152,#20153,#20154,#20155,#20156,#20157,
#20158,#20159,#20160,#20161,#20162,#20163,#20164,#20165,#20166,#20167,#20168,
#20169,#20170,#20171,#20172,#20173,#20174,#20175,#20176,#20177,#20178,#20179,
#20180,#20181,#20182,#20183,#20184,#20185,#20186,#20187,#20188,#20189,#20190,
#20191,#20192,#20193,#20194,#20195,#20196,#20197,#20198,#20199,#20200,#20201,
#20202,#20203,#20204,#20205,#20206,#20207,#20208,#20209,#20210,#20211,#20212,
#20213,#20214,#20215,#20216,#20217,#20218,#20219,#20220,#20221,#20222,#20223,
#20224,#20225,#20226,#20227,#20228,#20229,#20230),.UNSPECIFIED.,.F.,.F.,
(4,2,2,2,2,2,2,2,2,2,2,2,2,2,2,2,2,2,2,2,2,2,2,2,2,2,2,2,2,2,2,2,2,2,2,
2,2,2,2,2,2,2,2,2,2,2,2,2,2,2,2,2,2,2,2,2,2,2,2,2,2,2,2,2,2,2,2,2,2,2,2,
2,2,2,2,2,2,2,2,2,2,2,2,2,2,2,2,2,2,2,2,2,2,2,2,2,2,2,2,2,2,2,2,2,4),(-3.17259999392289,
-3.12496881097331,-3.11836850531031,-3.11409579174395,-3.11002953984388,
-3.10689426367969,-3.10280406102069,-3.09562214452332,-3.05960615618452,
-3.02877649122314,-3.00059430551812,-2.98882473813139,-2.98538225075395,
-2.98325139063015,-2.98126368167241,-2.97885376594607,-2.97270862514894,
-2.92190725684228,-2.88722496237993,-2.87425465035336,-2.86453796234612,
-2.85998224423964,-2.85646882497619,-2.85260892897295,-2.84629076818517,
-2.82498876061778,-2.75953341354037,-2.74562383800142,-2.73689813799119,
-2.73382884353142,-2.73177921139855,-2.7299495445617,-2.72744822390498,
-2.7211251809285,-2.67558398587311,-2.65399673618474,-2.6305432910418,-2.62041360092054,
-2.61240032196748,-2.608178148527,-2.60503280917959,-2.60107718417831,-2.59432029185784,
-2.56783148277945,-2.51451017236128,-2.49663007165224,-2.48963060511916,
-2.48440930915592,-2.48190407937595,-2.47994493067311,-2.47762594694345,
-2.47344187708961,-2.45284748328633,-2.38668621375722,-2.3727707006047,
-2.36251429884992,-2.35786014461553,-2.35433322507059,-2.35051932673315,
-2.34441178492399,-2.32502587302667,-2.26465423624521,-2.24589026394476,
-2.23514667285458,-2.23183287369807,-2.22973041292791,-2.2277259167726,
-2.22525005872627,-2.2191452309043,-2.16980389027994,-2.13419142953018,
-2.12101714495601,-2.11118291204162,-2.1066054820195,-2.10308924688258,
-2.09924010951645,-2.09297109912761,-2.07210282520022,-2.01943346272415,
-1.98615278737952,-1.98168173241009,-1.97932761105158,-1.97737106295488,
-1.97490982246655,-1.97100831342367,-1.94869780021006,-1.93049401466996,
-1.89957831685155,-1.86523602564397,-1.8582685817792,-1.85426741581928,
-1.85077806427195,-1.84645635066849,-1.83978302805478,-1.79122605800795,
-1.75368854772611,-1.74064835924039,-1.73231798451588,-1.72930250868749,
-1.72726408851753,-1.72542504877492,-1.72288632131961,-1.71641036265964,
-1.67799079970043,-1.67605418873215),.UNSPECIFIED.);
#292=B_SPLINE_CURVE_WITH_KNOTS('',3,(#20236,#20237,#20238,#20239,#20240,
#20241,#20242,#20243,#20244,#20245,#20246,#20247,#20248,#20249,#20250,#20251,
#20252,#20253,#20254,#20255,#20256,#20257,#20258,#20259,#20260,#20261,#20262,
#20263,#20264,#20265,#20266,#20267,#20268,#20269,#20270,#20271,#20272,#20273,
#20274,#20275,#20276,#20277,#20278,#20279,#20280,#20281,#20282,#20283,#20284,
#20285,#20286,#20287,#20288,#20289,#20290,#20291,#20292,#20293,#20294,#20295,
#20296,#20297,#20298,#20299,#20300,#20301,#20302,#20303,#20304,#20305,#20306,
#20307,#20308,#20309,#20310,#20311,#20312,#20313,#20314,#20315,#20316,#20317,
#20318,#20319,#20320,#20321,#20322,#20323,#20324,#20325,#20326,#20327,#20328,
#20329,#20330,#20331,#20332,#20333,#20334,#20335,#20336,#20337,#20338,#20339,
#20340,#20341,#20342,#20343,#20344,#20345,#20346,#20347,#20348,#20349,#20350,
#20351,#20352,#20353,#20354,#20355,#20356,#20357,#20358,#20359,#20360,#20361,
#20362,#20363,#20364,#20365,#20366,#20367,#20368,#20369,#20370,#20371,#20372,
#20373,#20374,#20375,#20376,#20377,#20378,#20379,#20380,#20381,#20382,#20383,
#20384,#20385,#20386,#20387,#20388,#20389,#20390,#20391,#20392,#20393,#20394,
#20395,#20396,#20397,#20398,#20399,#20400,#20401,#20402,#20403,#20404,#20405,
#20406,#20407,#20408,#20409,#20410,#20411,#20412,#20413,#20414,#20415,#20416),
 .UNSPECIFIED.,.F.,.F.,(4,3,3,3,3,3,3,3,3,3,3,3,3,3,3,3,3,3,3,3,3,3,3,3,
3,3,3,3,3,3,3,3,3,3,3,3,3,3,3,3,3,3,3,3,3,3,3,3,3,3,3,3,3,3,3,3,3,3,3,3,
4),(33.0800387021028,33.1788114424491,33.2775352322483,33.3762398755367,
33.4749551493895,33.5737748761942,33.672651172472,33.7716939664021,33.8320806131228,
33.9311397307074,34.0300584049669,34.1296938302993,34.2284358316502,34.3271453584,
34.4258521963517,34.5261745991704,34.6250231925307,34.7260825000786,34.8271418076264,
34.9262009252113,35.025119599471,35.1247550248034,35.2234970261545,35.3222065529047,
35.4209133908568,35.5212357936751,35.6200843870359,35.7211436945829,35.82220300213,
35.9212621197145,36.0201807939738,36.1198162193063,36.218558220657,36.3172677474068,
36.4159745853584,36.5162969881772,36.6151455815376,36.7162048890856,36.8172641966336,
36.9163233142183,37.0152419884777,37.1148774138102,37.213619415161,37.312328941911,
37.4110357798628,37.5113581826814,37.6102067760418,37.7112660835895,37.8123253911372,
37.9113845087219,38.0103031829812,38.1099386083137,38.2086806096646,38.3073901364146,
38.4060969743664,38.506419377185,38.6052679705455,38.7063272780932,38.8073865856408,
38.9480297229087,39.0086749840545),.UNSPECIFIED.);
#293=B_SPLINE_CURVE_WITH_KNOTS('',3,(#20417,#20418,#20419,#20420,#20421,
#20422,#20423,#20424,#20425,#20426,#20427,#20428,#20429),.UNSPECIFIED.,
 .F.,.F.,(4,3,3,3,4),(39.0086749844145,39.1061283325211,39.2034999693848,
39.3008301805805,39.3627720041259),.UNSPECIFIED.);
#294=B_SPLINE_CURVE_WITH_KNOTS('',3,(#20430,#20431,#20432,#20433,#20434,
#20435,#20436,#20437,#20438,#20439,#20440,#20441,#20442,#20443,#20444,#20445,
#20446,#20447,#20448,#20449,#20450,#20451,#20452,#20453,#20454,#20455,#20456,
#20457,#20458,#20459,#20460,#20461,#20462,#20463,#20464,#20465,#20466,#20467,
#20468,#20469,#20470,#20471,#20472,#20473,#20474,#20475,#20476,#20477,#20478,
#20479,#20480,#20481,#20482,#20483,#20484,#20485,#20486,#20487,#20488,#20489,
#20490,#20491,#20492,#20493,#20494,#20495,#20496,#20497,#20498,#20499,#20500,
#20501,#20502,#20503,#20504,#20505,#20506,#20507,#20508,#20509,#20510,#20511,
#20512,#20513,#20514,#20515,#20516,#20517,#20518,#20519,#20520,#20521,#20522,
#20523,#20524,#20525,#20526,#20527,#20528,#20529,#20530,#20531,#20532,#20533,
#20534,#20535,#20536,#20537,#20538,#20539,#20540,#20541,#20542,#20543,#20544,
#20545,#20546,#20547,#20548,#20549,#20550,#20551,#20552,#20553,#20554,#20555,
#20556,#20557,#20558,#20559,#20560,#20561,#20562,#20563,#20564,#20565,#20566,
#20567,#20568,#20569,#20570,#20571,#20572,#20573,#20574,#20575,#20576,#20577,
#20578,#20579,#20580,#20581,#20582,#20583,#20584,#20585,#20586,#20587,#20588,
#20589,#20590,#20591,#20592,#20593,#20594,#20595,#20596,#20597,#20598,#20599,
#20600,#20601,#20602,#20603,#20604,#20605,#20606,#20607,#20608,#20609,#20610,
#20611,#20612,#20613,#20614,#20615,#20616,#20617,#20618,#20619,#20620,#20621,
#20622,#20623,#20624,#20625,#20626,#20627,#20628,#20629,#20630,#20631,#20632,
#20633,#20634,#20635,#20636,#20637,#20638,#20639,#20640,#20641,#20642,#20643,
#20644,#20645,#20646,#20647,#20648,#20649,#20650,#20651,#20652,#20653,#20654,
#20655,#20656,#20657,#20658,#20659,#20660,#20661,#20662,#20663,#20664,#20665,
#20666,#20667,#20668,#20669,#20670,#20671,#20672,#20673,#20674,#20675,#20676,
#20677,#20678,#20679,#20680,#20681,#20682,#20683,#20684,#20685,#20686,#20687,
#20688,#20689,#20690,#20691,#20692,#20693,#20694,#20695,#20696,#20697,#20698,
#20699,#20700,#20701,#20702,#20703,#20704,#20705,#20706,#20707,#20708,#20709,
#20710,#20711),.UNSPECIFIED.,.F.,.F.,(4,2,2,2,2,2,2,2,2,2,2,2,2,2,2,2,2,
2,2,2,2,2,2,2,2,2,2,2,2,2,2,2,2,2,2,2,2,2,2,2,2,2,2,2,2,2,2,2,2,2,2,2,2,
2,2,2,2,2,2,2,2,2,2,2,2,2,2,2,2,2,2,2,2,2,2,2,2,2,2,2,2,2,2,2,2,2,2,2,2,
2,2,2,2,2,2,2,2,2,2,2,2,2,2,2,2,2,2,2,2,2,2,2,2,2,2,2,2,2,2,2,2,2,2,2,2,
2,2,2,2,2,2,2,2,2,2,2,2,2,2,2,4),(-1.67605418873215,-1.64446552570341,-1.61379541775656,
-1.60701601277305,-1.60305556305347,-1.59956146742909,-1.59518083036428,
-1.5866652416678,-1.55554836586235,-1.5033602837115,-1.48349741059974,-1.47935214976674,
-1.47704191306747,-1.47508196051158,-1.47256513654394,-1.46728355612929,
-1.46017877962238,-1.44188723341273,-1.38622875021952,-1.36227578346616,
-1.35570970119145,-1.35179569110038,-1.34829420571763,-1.34383866044754,
-1.3346523968148,-1.29929990316282,-1.24450322155425,-1.23144841080082,
-1.22776336141326,-1.22557881180475,-1.22359203767492,-1.22085601540368,
-1.21435562866304,-1.18232067991372,-1.12494103461589,-1.10929772679816,
-1.10365023977041,-1.10030660719022,-1.0967778391588,-1.09211195806968,
-1.0817906749433,-1.06776180082129,-1.00019830630836,-0.981109862488433,
-0.977007476205776,-0.974706853092972,-0.972745751438243,-0.970215414628244,
-0.964863569053112,-0.95763633031546,-0.938861914522575,-0.878450212878529,
-0.85905961949471,-0.8529511941131,-0.849136922517839,-0.845609782394701,
-0.840955519171999,-0.83069956500679,-0.816786713232761,-0.750636562863323,
-0.730066131986696,-0.725883341835163,-0.723564581856462,-0.721605327615493,
-0.719099565054224,-0.713875843771598,-0.706871626704422,-0.688972709089678,
-0.635575059923181,-0.609127613602163,-0.602373012061714,-0.59841781204071,
-0.595272308838384,-0.591049287001067,-0.583032205895378,-0.572897405359785,
-0.549427761675534,-0.502070482124086,-0.4908011501141,-0.477937518753328,
-0.474270282965583,-0.472089614076389,-0.470101324319369,-0.467356181427008,
-0.460801770271742,-0.451376249849108,-0.422654098414317,-0.362494730231977,
-0.35304486090271,-0.348538984343869,-0.345031630484092,-0.341145558191662,
-0.334708025063276,-0.309281319965056,-0.251283129256886,-0.228028623128943,
-0.224087392688026,-0.221614070539676,-0.219656813946372,-0.219638336092407,
-0.219620301519892,-0.219602694229522,-0.219585498971227,-0.219568701210277,
-0.219552287083677,-0.219536243368154,-0.219520557435778,-0.219505217218149,
-0.219490211197498,-0.219475528353639,-0.219461158145889,-0.219447090482153,
-0.219433315699463,-0.219419824552559,-0.219406608180464,-0.219393658073746,
-0.21938096608702,-0.219368524395416,-0.219356325492313,-0.219344362172756,
-0.219332627505137,-0.219321114832145,-0.219309817756675,-0.21929873012358,
-0.21928784600388,-0.219277159697579,-0.219266665729188,-0.219256358809398,
-0.21924623383803,-0.219236285913427,-0.219226510299542,-0.216726955493797,
-0.211587091030562,-0.20456762403992,-0.186609213777033,-0.132898376147193,
-0.10681202752676,-0.100081213120034,-0.0961312667424419,-0.0929852106039781,
-0.0902181295836139),.UNSPECIFIED.);
#295=B_SPLINE_CURVE_WITH_KNOTS('',3,(#20717,#20718,#20719,#20720,#20721,
#20722,#20723,#20724,#20725,#20726,#20727,#20728,#20729,#20730,#20731,#20732,
#20733,#20734,#20735,#20736,#20737,#20738,#20739,#20740,#20741,#20742,#20743,
#20744,#20745,#20746,#20747,#20748,#20749,#20750,#20751,#20752,#20753,#20754,
#20755,#20756,#20757,#20758,#20759,#20760,#20761,#20762,#20763,#20764,#20765,
#20766,#20767,#20768,#20769,#20770,#20771,#20772,#20773,#20774,#20775,#20776,
#20777,#20778,#20779,#20780,#20781,#20782,#20783,#20784,#20785,#20786,#20787,
#20788,#20789,#20790,#20791,#20792,#20793,#20794,#20795,#20796,#20797,#20798,
#20799,#20800,#20801,#20802,#20803,#20804,#20805,#20806,#20807,#20808,#20809,
#20810,#20811,#20812,#20813,#20814,#20815,#20816,#20817,#20818,#20819,#20820,
#20821,#20822,#20823,#20824,#20825,#20826,#20827,#20828,#20829,#20830,#20831,
#20832,#20833,#20834,#20835,#20836,#20837,#20838,#20839,#20840,#20841,#20842,
#20843,#20844,#20845,#20846,#20847,#20848,#20849,#20850,#20851,#20852,#20853,
#20854,#20855,#20856,#20857,#20858,#20859,#20860,#20861,#20862,#20863,#20864,
#20865,#20866,#20867,#20868,#20869,#20870,#20871,#20872,#20873,#20874,#20875,
#20876,#20877,#20878,#20879,#20880,#20881,#20882,#20883,#20884,#20885,#20886,
#20887,#20888,#20889,#20890,#20891,#20892,#20893,#20894,#20895,#20896,#20897),
 .UNSPECIFIED.,.F.,.F.,(4,3,3,3,3,3,3,3,3,3,3,3,3,3,3,3,3,3,3,3,3,3,3,3,
3,3,3,3,3,3,3,3,3,3,3,3,3,3,3,3,3,3,3,3,3,3,3,3,3,3,3,3,3,3,3,3,3,3,3,3,
4),(26.7958998905728,26.8666522515975,26.9657113691588,27.0646300433946,
27.1642654687329,27.2630074700601,27.3617169967863,27.4604238347143,27.560746237561,
27.6595948308979,27.7606541384995,27.8617134461011,27.9607725636749,28.0596912379233,
28.1593266632585,28.2580686645977,28.3567781913358,28.4554850292756,28.5558074321079,
28.654656025456,28.7557153330304,28.8567746406047,28.9558337582019,29.0547524324741,
29.1543878578034,29.2531298591674,29.3518393859305,29.4505462238956,29.5508686266988,
29.6497172200727,29.7507765275905,29.8518358351083,29.9508949526888,30.049813626944,
30.1494490522775,30.2481910536241,30.3469005803698,30.4456074183172,30.5459298211409,
30.6447784144971,30.7458377220545,30.846897029612,30.9459561471956,31.044874821454,
31.1445102467867,31.2432522481365,31.3419617748852,31.4406686128358,31.5409910156558,
31.639839609015,31.7408989165653,31.8419582241156,31.9397107034381,32.037933075085,
32.1354344299592,32.2328770951257,32.3302923655568,32.429091693321,32.5265951482302,
32.6260424124219,32.7254896766136),.UNSPECIFIED.);
#296=B_SPLINE_CURVE_WITH_KNOTS('',3,(#20898,#20899,#20900,#20901,#20902,
#20903,#20904,#20905,#20906,#20907,#20908,#20909,#20910),.UNSPECIFIED.,
 .F.,.F.,(4,3,3,3,4),(32.7254896768749,32.8370194186192,32.936080057733,
33.0349883528382,33.0800387021028),.UNSPECIFIED.);
#297=B_SPLINE_CURVE_WITH_KNOTS('',3,(#20912,#20913,#20914,#20915,#20916,
#20917,#20918,#20919,#20920,#20921,#20922,#20923),.UNSPECIFIED.,.F.,.F.,
(4,2,2,2,2,4),(-0.0902181295836139,-0.0887553371504392,-0.0807045076511089,
-0.0705153572373448,-0.0468548506221579,-0.000736301001977398),
 .UNSPECIFIED.);
#298=B_SPLINE_CURVE_WITH_KNOTS('',3,(#20924,#20925,#20926,#20927,#20928,
#20929,#20930,#20931,#20932,#20933,#20934,#20935,#20936,#20937,#20938,#20939,
#20940,#20941,#20942,#20943,#20944,#20945,#20946,#20947,#20948,#20949,#20950,
#20951,#20952,#20953,#20954,#20955,#20956,#20957,#20958,#20959,#20960,#20961,
#20962,#20963,#20964,#20965,#20966,#20967,#20968,#20969,#20970,#20971,#20972,
#20973,#20974,#20975,#20976,#20977,#20978,#20979,#20980,#20981,#20982,#20983,
#20984,#20985,#20986,#20987,#20988,#20989,#20990,#20991,#20992,#20993,#20994,
#20995,#20996,#20997,#20998,#20999,#21000,#21001,#21002,#21003,#21004,#21005,
#21006,#21007,#21008,#21009,#21010,#21011,#21012,#21013,#21014,#21015,#21016,
#21017,#21018,#21019,#21020,#21021,#21022,#21023,#21024,#21025,#21026,#21027,
#21028,#21029,#21030,#21031,#21032,#21033,#21034,#21035,#21036,#21037,#21038,
#21039,#21040,#21041,#21042,#21043,#21044,#21045,#21046,#21047,#21048,#21049,
#21050,#21051,#21052,#21053,#21054,#21055,#21056,#21057,#21058,#21059,#21060,
#21061,#21062,#21063,#21064,#21065,#21066,#21067,#21068,#21069,#21070,#21071,
#21072,#21073,#21074,#21075,#21076,#21077,#21078,#21079,#21080,#21081,#21082,
#21083,#21084,#21085,#21086,#21087,#21088,#21089,#21090,#21091,#21092,#21093,
#21094,#21095,#21096,#21097,#21098,#21099,#21100,#21101,#21102,#21103,#21104,
#21105,#21106,#21107,#21108,#21109,#21110,#21111,#21112,#21113,#21114,#21115,
#21116,#21117,#21118,#21119,#21120,#21121,#21122,#21123,#21124,#21125),
 .UNSPECIFIED.,.F.,.F.,(4,2,2,2,2,2,2,2,2,2,2,2,2,2,2,2,2,2,2,2,2,2,2,2,
2,2,2,2,2,2,2,2,2,2,2,2,2,2,2,2,2,2,2,2,2,2,2,2,2,2,2,2,2,2,2,2,2,2,2,2,
2,2,2,2,2,2,2,2,2,2,2,2,2,2,2,2,2,2,2,2,2,2,2,2,2,2,2,2,2,2,2,2,2,2,2,2,
2,2,2,2,4),(-3.17338897415504,-3.15145317667747,-3.14756194944923,-3.14509576002276,
-3.14318825463869,-3.14141535638956,-3.13916544226158,-3.13528952983564,
-3.11963491996032,-3.10145196086512,-3.04897341387108,-3.0344935147722,
-3.02391898825236,-3.01920624991346,-3.01566846281435,-3.01187475928096,
-3.00586853141856,-2.98739721949976,-2.93257978086865,-2.90911608726844,
-2.90077838506334,-2.89484499951574,-2.89223441317387,-2.89028827015876,
-2.88809411425886,-2.88436962501802,-2.87091237686426,-2.81629739892998,
-2.78108350996001,-2.77191243662363,-2.76745810105447,-2.76395483749657,
-2.76003600221971,-2.7534549666887,-2.72934498263058,-2.67938776270491,
-2.64990438696998,-2.64365174469296,-2.64095697210415,-2.63897553599654,
-2.63676972479563,-2.63299197959258,-2.61895275076301,-2.55203199647492,
-2.52530058844043,-2.51876657121876,-2.51485828579963,-2.51135354158148,
-2.50688233168194,-2.49762149406868,-2.43563900632499,-2.39733040241475,
-2.39191501264215,-2.38937187009492,-2.38740881571431,-2.3851152135072,
-2.381046765334,-2.3625396277497,-2.30893254648497,-2.27479692368528,-2.26783644213133,
-2.26383555357514,-2.26034426548011,-2.25601733248866,-2.24933053204391,
-2.2006961827,-2.16342015612807,-2.15024469047998,-2.14185091834582,-2.13882576047495,
-2.13678465577309,-2.13494622137547,-2.13241217364397,-2.1259683135347,
-2.08665031358038,-2.04402966533529,-2.02205008673329,-2.01589305528209,
-2.01206703761017,-2.00854151307228,-2.00398596608263,-1.99400882575514,
-1.94371019187171,-1.90805558163563,-1.89740222508034,-1.89021768609199,
-1.88737003247275,-1.88536351595007,-1.88322192583434,-1.879733861959,-1.86856123299659,
-1.81098941514518,-1.78546219930833,-1.77475114567881,-1.76637809000447,
-1.7620815756749,-1.75859260958355,-1.75456977841347,-1.74769053193514,
-1.71811416048442,-1.67634727028989),.UNSPECIFIED.);
#299=B_SPLINE_CURVE_WITH_KNOTS('',3,(#21131,#21132,#21133,#21134,#21135,
#21136,#21137,#21138,#21139,#21140,#21141,#21142,#21143,#21144,#21145,#21146,
#21147,#21148,#21149,#21150,#21151,#21152,#21153,#21154,#21155,#21156,#21157,
#21158,#21159,#21160,#21161,#21162,#21163,#21164,#21165,#21166,#21167,#21168,
#21169,#21170,#21171,#21172,#21173,#21174,#21175,#21176,#21177,#21178,#21179,
#21180,#21181,#21182,#21183,#21184,#21185,#21186,#21187,#21188,#21189,#21190,
#21191,#21192,#21193,#21194,#21195,#21196,#21197,#21198,#21199,#21200,#21201,
#21202,#21203,#21204,#21205,#21206,#21207,#21208,#21209,#21210,#21211,#21212,
#21213,#21214,#21215,#21216,#21217,#21218,#21219,#21220,#21221,#21222,#21223,
#21224,#21225,#21226,#21227,#21228,#21229,#21230,#21231,#21232,#21233,#21234,
#21235,#21236,#21237,#21238,#21239,#21240,#21241,#21242,#21243,#21244,#21245,
#21246,#21247,#21248,#21249,#21250,#21251,#21252,#21253,#21254,#21255,#21256,
#21257,#21258,#21259,#21260,#21261,#21262,#21263,#21264,#21265,#21266,#21267,
#21268,#21269,#21270,#21271,#21272,#21273,#21274,#21275,#21276,#21277,#21278,
#21279,#21280,#21281,#21282,#21283,#21284,#21285,#21286,#21287,#21288,#21289,
#21290,#21291,#21292,#21293,#21294,#21295,#21296,#21297,#21298,#21299,#21300,
#21301,#21302,#21303,#21304,#21305,#21306,#21307,#21308,#21309,#21310,#21311),
 .UNSPECIFIED.,.F.,.F.,(4,3,3,3,3,3,3,3,3,3,3,3,3,3,3,3,3,3,3,3,3,3,3,3,
3,3,3,3,3,3,3,3,3,3,3,3,3,3,3,3,3,3,3,3,3,3,3,3,3,3,3,3,3,3,3,3,3,3,3,3,
4),(20.5129680002155,20.6107259391232,20.7085286089183,20.8065050140131,
20.8962850845758,20.9953442016773,21.0942628754568,21.1938983009096,21.292640301791,
21.3913498280767,21.4900566655699,21.5903790689473,21.6892276618682,21.7902869704738,
21.8913462790794,21.9904053958419,22.0893240692632,22.1889594948032,22.2877014952828,
22.386411021151,22.4851178582115,22.5854402620544,22.6842888545097,22.7853481640464,
22.8864074735831,22.9854665917689,23.0843852666377,23.1840206918188,23.282762693795,
23.3814722211749,23.4801790597604,23.580501461842,23.6793500558389,23.7804093619628,
23.8814686680867,23.9805277855541,24.0794464596959,24.1790818850577,24.2778238862909,
24.3765334129235,24.4752402507583,24.5755626537163,24.6744112469619,24.7754705547761,
24.8765298625903,24.975588980077,25.0745076542362,25.1741430795934,25.27288508084,
25.3715946074844,25.4703014453291,25.5706238482703,25.6694724415217,25.7705317493078,
25.8715910570939,25.9728761869164,26.0739977696392,26.1749480073185,26.2757973957606,
26.3765610499166,26.4423043696953),.UNSPECIFIED.);
#300=B_SPLINE_CURVE_WITH_KNOTS('',3,(#21312,#21313,#21314,#21315,#21316,
#21317,#21318,#21319,#21320,#21321,#21322,#21323,#21324),.UNSPECIFIED.,
 .F.,.F.,(4,3,3,3,4),(26.4423043699728,26.5495705796222,26.6571264780996,
26.765082346119,26.7958998905728),.UNSPECIFIED.);
#301=B_SPLINE_CURVE_WITH_KNOTS('',3,(#21325,#21326,#21327,#21328,#21329,
#21330,#21331,#21332,#21333,#21334,#21335,#21336,#21337,#21338,#21339,#21340,
#21341,#21342,#21343,#21344,#21345,#21346,#21347,#21348,#21349,#21350,#21351,
#21352,#21353,#21354,#21355,#21356,#21357,#21358,#21359,#21360,#21361,#21362,
#21363,#21364,#21365,#21366,#21367,#21368,#21369,#21370,#21371,#21372,#21373,
#21374,#21375,#21376,#21377,#21378,#21379,#21380,#21381,#21382,#21383,#21384,
#21385,#21386,#21387,#21388,#21389,#21390,#21391,#21392,#21393,#21394,#21395,
#21396,#21397,#21398,#21399,#21400,#21401,#21402,#21403,#21404,#21405,#21406,
#21407,#21408,#21409,#21410,#21411,#21412,#21413,#21414,#21415,#21416,#21417,
#21418,#21419,#21420,#21421,#21422,#21423,#21424,#21425,#21426,#21427,#21428,
#21429,#21430,#21431,#21432,#21433,#21434,#21435,#21436,#21437,#21438,#21439,
#21440,#21441,#21442,#21443,#21444,#21445,#21446,#21447,#21448,#21449,#21450,
#21451,#21452,#21453,#21454,#21455,#21456,#21457,#21458,#21459,#21460,#21461,
#21462,#21463,#21464,#21465,#21466,#21467,#21468,#21469,#21470,#21471,#21472,
#21473,#21474,#21475,#21476,#21477,#21478,#21479,#21480,#21481,#21482,#21483,
#21484,#21485,#21486,#21487,#21488,#21489,#21490,#21491,#21492,#21493,#21494,
#21495,#21496,#21497,#21498,#21499,#21500,#21501,#21502,#21503,#21504,#21505,
#21506,#21507,#21508,#21509,#21510,#21511,#21512,#21513,#21514,#21515,#21516,
#21517,#21518,#21519,#21520,#21521,#21522,#21523,#21524,#21525,#21526,#21527,
#21528,#21529,#21530,#21531,#21532,#21533,#21534,#21535,#21536,#21537,#21538,
#21539,#21540,#21541,#21542,#21543,#21544,#21545,#21546,#21547,#21548,#21549,
#21550,#21551,#21552,#21553,#21554,#21555,#21556),.UNSPECIFIED.,.F.,.F.,
(4,2,2,2,2,2,2,2,2,2,2,2,2,2,2,2,2,2,2,2,2,2,2,2,2,2,2,2,2,2,2,2,2,2,2,
2,2,2,2,2,2,2,2,2,2,2,2,2,2,2,2,2,2,2,2,2,2,2,2,2,2,2,2,2,2,2,2,2,2,2,2,
2,2,2,2,2,2,2,2,2,2,2,2,2,2,2,2,2,2,2,2,2,2,2,2,2,2,2,2,2,2,2,2,2,2,2,2,
2,2,2,2,2,2,2,2,4),(-1.67634727028989,-1.66741515781725,-1.65007009753052,
-1.64320884805284,-1.63806717820834,-1.63557685571605,-1.63380546311439,
-1.63155034778241,-1.62765009107774,-1.61166443286676,-1.60273261522532,
-1.58721972708483,-1.52486415310859,-1.51564296736236,-1.51117969066712,
-1.50767621711202,-1.50376422498485,-1.49721170849928,-1.47020172013932,
-1.40068169303466,-1.38914158875836,-1.38561174988993,-1.3834609372194,
-1.38145901503103,-1.3786367864817,-1.37161344401501,-1.36127887301356,
-1.32755292182266,-1.27462480242134,-1.26471717194173,-1.26017426015671,
-1.25665068583042,-1.2528189443509,-1.24663525729233,-1.22435372328808,
-1.18063693076381,-1.16673827571981,-1.15823326743009,-1.13908221184482,
-1.1349751377007,-1.13267294041826,-1.13071118576053,-1.12818089747551,
-1.12283227601954,-1.1156114729253,-1.09686633357667,-1.03698458136081,
-1.01708923153163,-1.01092464452101,-1.00709720834416,-1.00357256756493,
-0.998943121216566,-0.98883068662824,-0.975172844065648,-0.937279909720506,
-0.891402723743196,-0.885089300562871,-0.882588766966048,-0.880758870749702,
-0.878708017677102,-0.875635203490524,-0.866888202350397,-0.852931320846599,
-0.786872125674087,-0.766053683765324,-0.759788706660085,-0.755939624042054,
-0.752421854319723,-0.747840148259659,-0.737987620695772,-0.724784247100402,
-0.68904544589373,-0.639916004034322,-0.633801977568994,-0.631324110062701,
-0.629318670685728,-0.627216094946634,-0.623903612812235,-0.613178048028686,
-0.594461268734392,-0.534944580871909,-0.514733791760564,-0.508533247839354,
-0.504698380367309,-0.501176798729665,-0.496565786413771,-0.486552301820809,
-0.473067577684551,-0.436005111597049,-0.432337303794875,-0.389149229170169,
-0.382756589481615,-0.380231480904177,-0.378395641265319,-0.376352730259696,
-0.37331687277746,-0.364841502733728,-0.35148476677032,-0.322641606957777,
-0.269891760856808,-0.260149903565411,-0.255567057890482,-0.25217184455642,
-0.248905096645079,-0.243525283894319,-0.228601392735488,-0.205469003111721,
-0.174869595024417,-0.157070991986575,-0.134640831473529,-0.130734154595829,
-0.128271092978842,-0.126314108723162,-0.123960689724939,-0.119494270154341,
-0.0901440899991799),.UNSPECIFIED.);
#302=B_SPLINE_CURVE_WITH_KNOTS('',3,(#21562,#21563,#21564,#21565,#21566,
#21567,#21568,#21569,#21570,#21571,#21572,#21573,#21574,#21575,#21576,#21577,
#21578,#21579,#21580,#21581,#21582,#21583,#21584,#21585,#21586,#21587,#21588,
#21589,#21590,#21591,#21592,#21593,#21594,#21595,#21596,#21597,#21598,#21599,
#21600,#21601,#21602,#21603,#21604,#21605,#21606,#21607,#21608,#21609,#21610,
#21611,#21612,#21613,#21614,#21615,#21616,#21617,#21618,#21619,#21620,#21621,
#21622,#21623,#21624,#21625,#21626,#21627,#21628,#21629,#21630,#21631,#21632,
#21633,#21634,#21635,#21636,#21637,#21638,#21639,#21640,#21641,#21642,#21643,
#21644,#21645,#21646,#21647,#21648,#21649,#21650,#21651,#21652,#21653,#21654,
#21655,#21656,#21657,#21658,#21659,#21660,#21661,#21662,#21663,#21664,#21665,
#21666,#21667,#21668,#21669,#21670,#21671,#21672,#21673,#21674,#21675,#21676,
#21677,#21678,#21679,#21680,#21681,#21682,#21683,#21684,#21685,#21686,#21687,
#21688,#21689,#21690,#21691,#21692,#21693,#21694,#21695,#21696,#21697,#21698,
#21699,#21700,#21701,#21702,#21703,#21704,#21705,#21706,#21707,#21708,#21709,
#21710,#21711,#21712,#21713,#21714,#21715,#21716,#21717,#21718,#21719,#21720,
#21721,#21722,#21723,#21724,#21725,#21726,#21727,#21728,#21729,#21730,#21731,
#21732,#21733,#21734,#21735,#21736,#21737,#21738,#21739),.UNSPECIFIED.,
 .F.,.F.,(4,3,3,3,3,3,3,3,3,3,3,3,3,3,3,3,3,3,3,3,3,3,3,3,3,3,3,3,3,3,3,
3,3,3,3,3,3,3,3,3,3,3,3,3,3,3,3,3,3,3,3,3,3,3,3,3,3,3,3,4),(14.2304175189723,
14.3291587597253,14.4278681142516,14.5265753676279,14.6264110051095,14.7252606329009,
14.8255892752276,14.9259179175542,15.0249770454872,15.1238957307452,15.2235311534093,
15.3222731672754,15.4209827070846,15.5196895586242,15.6200119469826,15.7188605551067,
15.8199198335823,15.9209791120578,16.0200381791658,16.1189568020786,16.218592240139,
16.3173341883945,16.4160436615095,16.5147504453582,16.615072910659,16.7139214493074,
16.8149808779344,16.9160403065614,17.0150994500851,17.1140181506013,17.2136535694092,
17.3123955975981,17.4111051513445,17.5098120164147,17.6101343875773,17.7089830080811,
17.8100422545731,17.911101501065,18.0101606176973,18.1090792910617,18.2087147166251,
18.3074567172289,18.4061662432893,18.5048730806102,18.6051954843498,18.7040440772322,
18.8051033864004,18.9061626955686,19.0052218065867,19.1041404741599,19.2037759011489,
19.3025178955699,19.4012274153137,19.4999342461923,19.6002566571623,19.6991052433558,
19.800164566714,19.9012238900722,20.0301714761699,20.1591190622677),
 .UNSPECIFIED.);
#303=B_SPLINE_CURVE_WITH_KNOTS('',3,(#21740,#21741,#21742,#21743,#21744,
#21745,#21746,#21747,#21748,#21749,#21750,#21751,#21752),.UNSPECIFIED.,
 .F.,.F.,(4,3,3,3,4),(20.1591190625158,20.2568630563804,20.3545467790412,
20.4522206776011,20.5129680002155),.UNSPECIFIED.);
#304=B_SPLINE_CURVE_WITH_KNOTS('',3,(#21754,#21755,#21756,#21757,#21758,
#21759,#21760,#21761,#21762,#21763,#21764,#21765,#21766,#21767),
 .UNSPECIFIED.,.F.,.F.,(4,2,2,2,2,2,4),(-0.0901440899991799,-0.0865142020355592,
-0.0179497024792971,-0.00869120363488619,-0.00427521847958375,-0.00207284054739809,
-0.000735550131679377),.UNSPECIFIED.);
#305=B_SPLINE_CURVE_WITH_KNOTS('',3,(#21768,#21769,#21770,#21771,#21772,
#21773,#21774,#21775,#21776,#21777,#21778,#21779,#21780,#21781,#21782,#21783,
#21784,#21785,#21786,#21787,#21788,#21789,#21790,#21791,#21792,#21793,#21794,
#21795,#21796,#21797,#21798,#21799,#21800,#21801,#21802,#21803,#21804,#21805,
#21806,#21807,#21808,#21809,#21810,#21811,#21812,#21813,#21814,#21815,#21816,
#21817,#21818,#21819,#21820,#21821,#21822,#21823,#21824,#21825,#21826,#21827,
#21828,#21829,#21830,#21831,#21832,#21833,#21834,#21835,#21836,#21837,#21838,
#21839,#21840,#21841,#21842,#21843,#21844,#21845,#21846,#21847,#21848,#21849,
#21850,#21851,#21852,#21853,#21854,#21855,#21856,#21857,#21858,#21859,#21860,
#21861,#21862,#21863,#21864,#21865,#21866,#21867,#21868,#21869,#21870,#21871,
#21872,#21873,#21874,#21875,#21876,#21877,#21878,#21879,#21880,#21881,#21882,
#21883,#21884,#21885,#21886,#21887,#21888,#21889,#21890,#21891,#21892,#21893,
#21894,#21895,#21896,#21897,#21898,#21899,#21900,#21901,#21902,#21903,#21904,
#21905,#21906,#21907,#21908,#21909,#21910,#21911,#21912,#21913,#21914,#21915,
#21916,#21917,#21918,#21919,#21920,#21921,#21922,#21923,#21924,#21925,#21926,
#21927,#21928,#21929,#21930,#21931,#21932,#21933,#21934,#21935,#21936,#21937,
#21938,#21939,#21940,#21941,#21942,#21943,#21944,#21945,#21946,#21947,#21948,
#21949,#21950,#21951,#21952,#21953,#21954,#21955,#21956,#21957,#21958,#21959,
#21960,#21961,#21962,#21963,#21964,#21965,#21966,#21967,#21968,#21969,#21970,
#21971),.UNSPECIFIED.,.F.,.F.,(4,2,2,2,2,2,2,2,2,2,2,2,2,2,2,2,2,2,2,2,
2,2,2,2,2,2,2,2,2,2,2,2,2,2,2,2,2,2,2,2,2,2,2,2,2,2,2,2,2,2,2,2,2,2,2,2,
2,2,2,2,2,2,2,2,2,2,2,2,2,2,2,2,2,2,2,2,2,2,2,2,2,2,2,2,2,2,2,2,2,2,2,2,
2,2,2,2,2,2,2,2,2,4),(-3.1722509398096,-3.17060364178562,-3.16756475987777,
-3.16076857491728,-3.13202985013187,-3.08130818076906,-3.06339374770734,
-3.05638483235411,-3.05115778742784,-3.04865107524353,-3.04687793928561,
-3.04463418047412,-3.0407826670575,-3.02542533057891,-3.01857113997389,
-2.95893977948005,-2.9332330746546,-2.92677375012245,-2.92346955050727,
-2.9203213030464,-2.91636991923783,-2.90957452080238,-2.88068670174827,
-2.83632851963011,-2.80674846121586,-2.80048740143094,-2.79779183442152,
-2.79581092189301,-2.79360690004671,-2.78983481507202,-2.77584730469061,
-2.76578292607347,-2.74800166937713,-2.70395026721197,-2.68158065245759,
-2.67539006103701,-2.67155737864756,-2.66803516305312,-2.66349711221027,
-2.65361276970661,-2.600208147281,-2.58280452884286,-2.55529296747341,-2.54924577813284,
-2.54658754310513,-2.54461192544506,-2.54238909799065,-2.538531275098,-2.52355856240514,
-2.5145469624538,-2.46830336670483,-2.43430116973454,-2.42592508108142,
-2.42162858020279,-2.41814038861373,-2.41411929948595,-2.40724512539072,
-2.37773552562209,-2.32699665401711,-2.3096447536604,-2.3027822612045,-2.29764014561524,
-2.29515009680769,-2.29337909812818,-2.29112476577515,-2.28722647397197,
-2.27125846537618,-2.20056490119876,-2.17905603290402,-2.17294358245344,
-2.16912833361109,-2.16560132708545,-2.16102775594893,-2.15131857266118,
-2.09676063498915,-2.05199131310598,-2.04656643728882,-2.04402217086125,
-2.0420597212145,-2.03976847212473,-2.03570822808801,-2.0173176594134,-1.96363422800829,
-1.92950574779454,-1.92254781741689,-1.91854846217572,-1.91505854555955,
-1.91073335040183,-1.90404929937544,-1.85543194457712,-1.81816313581032,
-1.80500257106894,-1.79661667137624,-1.79359340868247,-1.791553324392,-1.78971587244261,
-1.7871829365979,-1.78074074700496,-1.74158616324513,-1.70684684234202,
-1.67788094058519,-1.67566337115906),.UNSPECIFIED.);
#306=B_SPLINE_CURVE_WITH_KNOTS('',3,(#21977,#21978,#21979,#21980,#21981,
#21982,#21983,#21984,#21985,#21986,#21987,#21988,#21989,#21990,#21991,#21992,
#21993,#21994,#21995,#21996,#21997,#21998),.UNSPECIFIED.,.F.,.F.,(4,2,2,
2,2,2,2,2,2,2,4),(-0.0899054331255484,-0.076554022126443,-0.0575923344739192,
-0.0404520211695611,-0.0364869914952116,-0.0342258185213306,-0.0324608490723674,
-0.0305641377237055,-0.0281332474336483,-0.0243291396135012,-0.00076704490792084),
 .UNSPECIFIED.);
#307=B_SPLINE_CURVE_WITH_KNOTS('',3,(#22000,#22001,#22002,#22003,#22004,
#22005,#22006,#22007,#22008,#22009,#22010,#22011,#22012,#22013,#22014,#22015,
#22016,#22017,#22018,#22019,#22020,#22021,#22022,#22023,#22024,#22025,#22026,
#22027,#22028,#22029,#22030,#22031,#22032,#22033,#22034,#22035,#22036,#22037,
#22038,#22039,#22040,#22041,#22042,#22043,#22044,#22045,#22046,#22047,#22048,
#22049,#22050,#22051,#22052,#22053,#22054,#22055,#22056,#22057,#22058,#22059,
#22060,#22061,#22062,#22063,#22064,#22065,#22066,#22067,#22068,#22069,#22070,
#22071,#22072,#22073,#22074,#22075,#22076,#22077,#22078,#22079,#22080,#22081,
#22082,#22083,#22084,#22085,#22086,#22087,#22088,#22089,#22090,#22091,#22092,
#22093,#22094,#22095,#22096,#22097,#22098,#22099,#22100,#22101,#22102,#22103,
#22104,#22105,#22106,#22107,#22108,#22109,#22110,#22111,#22112,#22113,#22114,
#22115,#22116,#22117,#22118,#22119,#22120),.UNSPECIFIED.,.F.,.F.,(4,3,3,
3,3,3,3,3,3,3,3,3,3,3,3,3,3,3,3,3,3,3,3,3,3,3,3,3,3,3,3,3,3,3,3,3,3,3,3,
3,4),(-3.84897440539517,-3.75125824246988,-3.65367165958683,-3.55615640926645,
-3.45868120095872,-3.36121479544941,-3.26366285251732,-3.16606894445241,
-3.06831010828305,-2.98518358351084,-2.88598456951401,-2.78692366642958,
-2.68732350675178,-2.58843473405244,-2.48957707964969,-2.39072097507435,
-2.29057132855757,-2.19157226309705,-2.09084732605214,-1.99012238900722,
-1.89213277745176,-1.7942843081741,-1.69438141896529,-1.59670435988929,
-1.49905580466275,-1.40140475752039,-1.29981886676619,-1.20200306502378,
-1.10410734082398,-1.00604310459973,-0.995061194503613,-0.893246091409371,
-0.791590847240874,-0.690095795641479,-0.588695144143975,-0.487364670179868,
-0.386080230764985,-0.284788586297225,-0.183499496794958,-0.0821381948532282,
-1.10844070079203E-14),.UNSPECIFIED.);
#308=B_SPLINE_CURVE_WITH_KNOTS('',3,(#22124,#22125,#22126,#22127,#22128,
#22129,#22130,#22131,#22132,#22133,#22134,#22135,#22136,#22137,#22138,#22139,
#22140,#22141,#22142,#22143,#22144,#22145,#22146,#22147,#22148,#22149,#22150,
#22151,#22152,#22153,#22154,#22155,#22156,#22157,#22158,#22159,#22160,#22161,
#22162,#22163,#22164,#22165,#22166,#22167,#22168,#22169,#22170,#22171,#22172,
#22173,#22174,#22175,#22176,#22177,#22178,#22179,#22180,#22181,#22182,#22183,
#22184,#22185,#22186,#22187,#22188,#22189,#22190,#22191,#22192,#22193,#22194,
#22195,#22196,#22197,#22198,#22199,#22200,#22201,#22202,#22203,#22204,#22205,
#22206,#22207,#22208,#22209,#22210,#22211,#22212,#22213,#22214,#22215,#22216,
#22217,#22218,#22219,#22220,#22221,#22222,#22223,#22224,#22225,#22226,#22227,
#22228,#22229,#22230,#22231,#22232,#22233,#22234,#22235,#22236,#22237,#22238,
#22239,#22240,#22241,#22242,#22243,#22244,#22245,#22246,#22247,#22248,#22249,
#22250,#22251,#22252,#22253,#22254,#22255,#22256,#22257,#22258,#22259,#22260,
#22261,#22262,#22263,#22264,#22265,#22266,#22267,#22268,#22269,#22270,#22271,
#22272,#22273,#22274,#22275,#22276,#22277,#22278,#22279,#22280,#22281,#22282,
#22283,#22284,#22285,#22286,#22287,#22288,#22289,#22290,#22291,#22292,#22293,
#22294,#22295),.UNSPECIFIED.,.F.,.F.,(4,3,3,3,3,3,3,3,3,3,3,3,3,3,3,3,3,
3,3,3,3,3,3,3,3,3,3,3,3,3,3,3,3,3,3,3,3,3,3,3,3,3,3,3,3,3,3,3,3,3,3,3,3,
3,3,3,3,4),(2.01695526861829,2.11569428289456,2.21429391180832,2.31278169291955,
2.41120867663817,2.50960510300603,2.60800117427649,2.70649198428098,2.80503037766619,
2.90373779545109,2.98518358351083,3.08441219206656,3.18350384345799,3.28309646027754,
3.38201865334366,3.4809106774714,3.57980207048774,3.67991274736941,3.77894908090012,
3.87959692945728,3.98024477801444,4.07917123083895,4.17795538394911,4.27762420752023,
4.37622812463871,4.4747985304458,4.57336539305711,4.67385053792235,4.77255845171639,
4.87393221211723,4.97530597251806,5.0743944712415,5.17334267030362,5.27297073239337,
5.37174238517647,5.47048154357541,5.56921795237523,5.66950525603684,5.76838296393618,
5.86937506547893,5.97036716702167,6.06944598088698,6.16838478747198,6.26801523422864,
6.3667782867615,6.46550916360479,6.56423762247439,6.66453530723711,6.76340597267392,
6.8644171670996,6.96542836152528,7.06514551960968,7.1647175303196,7.2641732783273,
7.36353573611598,7.46284448248297,7.5621384291416,7.59274844815658),
 .UNSPECIFIED.);
#309=B_SPLINE_CURVE_WITH_KNOTS('',3,(#22296,#22297,#22298,#22299,#22300,
#22301,#22302,#22303,#22304,#22305,#22306,#22307,#22308),.UNSPECIFIED.,
 .F.,.F.,(4,3,3,3,4),(7.59274844853383,7.7041721787488,7.81611578899353,
7.92866788548955,7.94663621176237),.UNSPECIFIED.);
#310=B_SPLINE_CURVE_WITH_KNOTS('',3,(#22314,#22315,#22316,#22317,#22318,
#22319),.UNSPECIFIED.,.F.,.F.,(4,1,1,4),(131.030246900353,131.266332202741,
132.261393397245,133.256454591748),.UNSPECIFIED.);
#311=B_SPLINE_CURVE_WITH_KNOTS('',3,(#22322,#22323,#22324,#22325,#22326,
#22327,#22328,#22329,#22330,#22331,#22332,#22333,#22334,#22335,#22336,#22337,
#22338,#22339,#22340,#22341,#22342,#22343,#22344,#22345,#22346,#22347,#22348,
#22349,#22350,#22351,#22352,#22353,#22354,#22355,#22356,#22357,#22358,#22359,
#22360,#22361,#22362,#22363,#22364,#22365,#22366,#22367,#22368,#22369,#22370,
#22371,#22372,#22373,#22374,#22375,#22376,#22377,#22378,#22379,#22380,#22381,
#22382,#22383,#22384,#22385,#22386,#22387,#22388,#22389,#22390,#22391,#22392,
#22393,#22394,#22395,#22396,#22397,#22398,#22399,#22400,#22401,#22402,#22403,
#22404,#22405,#22406,#22407,#22408,#22409,#22410,#22411,#22412,#22413,#22414,
#22415),.UNSPECIFIED.,.F.,.F.,(4,3,3,3,3,3,3,3,3,3,3,3,3,3,3,3,3,3,3,3,
3,3,3,3,3,3,3,3,3,3,3,4),(131.031732990453,131.129719001446,131.223540756003,
131.317335965402,131.411130403081,131.504949834588,131.598875844033,131.69286470379,
131.786999793311,131.815621078398,131.910029099741,132.004308879585,132.098488743851,
132.192599708902,132.286675386837,132.38074122658,132.474822661588,132.569002090768,
132.663235460962,132.757616799081,132.810682272902,132.90455843657,132.998308854135,
133.095869530573,133.189457985588,133.283016460457,133.376571017001,133.470147706645,
133.563827171698,133.657567522566,133.751451095249,133.778794265637),
 .UNSPECIFIED.);
#312=B_SPLINE_CURVE_WITH_KNOTS('',3,(#22421,#22422,#22423,#22424,#22425,
#22426,#22427,#22428,#22429,#22430,#22431,#22432,#22433,#22434,#22435,#22436,
#22437,#22438,#22439,#22440,#22441,#22442,#22443,#22444,#22445,#22446,#22447,
#22448,#22449,#22450,#22451,#22452,#22453,#22454,#22455,#22456,#22457,#22458,
#22459,#22460,#22461,#22462,#22463,#22464,#22465,#22466,#22467,#22468,#22469,
#22470,#22471,#22472,#22473,#22474,#22475,#22476,#22477,#22478,#22479,#22480,
#22481,#22482,#22483,#22484,#22485,#22486,#22487,#22488,#22489,#22490,#22491,
#22492,#22493,#22494,#22495,#22496,#22497,#22498,#22499,#22500,#22501,#22502,
#22503,#22504,#22505,#22506,#22507,#22508,#22509,#22510,#22511,#22512,#22513,
#22514,#22515,#22516,#22517,#22518,#22519,#22520,#22521,#22522,#22523,#22524,
#22525,#22526,#22527,#22528,#22529,#22530,#22531,#22532,#22533,#22534,#22535,
#22536,#22537,#22538,#22539,#22540,#22541,#22542,#22543,#22544,#22545,#22546,
#22547,#22548,#22549,#22550,#22551,#22552,#22553,#22554,#22555,#22556),
 .UNSPECIFIED.,.F.,.F.,(4,3,3,3,3,3,3,3,3,3,3,3,3,3,3,3,3,3,3,3,3,3,3,3,
3,3,3,3,3,3,3,3,3,3,3,3,3,3,3,3,3,3,3,3,3,4),(124.748116942751,124.842021477706,
124.935936809012,125.029949826741,125.124012734743,125.21823452561,125.295965035719,
125.390188901834,125.484284908524,125.578281625117,125.672211126157,125.766106452365,
125.859993270984,125.953897234944,126.047902627316,126.14196364901,126.236176981576,
126.291026230223,126.385283355284,126.479412577247,126.573442422118,126.667404787361,
126.761332802783,126.8552520969,126.949188283725,127.043225319743,127.13731770511,
127.231561651695,127.286087424727,127.380343323035,127.474471636526,127.568500887675,
127.662463125408,127.756391300844,127.85031104033,127.944247955951,128.038286144246,
128.132379922439,128.226625623753,128.28114861923,128.379025264194,128.47673030057,
128.574231689995,128.671611327341,128.768855381404,128.805298797182),
 .UNSPECIFIED.);
#313=B_SPLINE_CURVE_WITH_KNOTS('',3,(#22557,#22558,#22559,#22560,#22561,
#22562),.UNSPECIFIED.,.F.,.F.,(4,1,1,4),(128.80530075582,129.276209813734,
130.271271008237,131.030246900353),.UNSPECIFIED.);
#314=B_SPLINE_CURVE_WITH_KNOTS('',3,(#22564,#22565,#22566,#22567,#22568,
#22569,#22570,#22571,#22572,#22573,#22574,#22575,#22576,#22577,#22578,#22579,
#22580,#22581,#22582,#22583,#22584,#22585,#22586,#22587,#22588,#22589,#22590,
#22591,#22592,#22593,#22594,#22595,#22596,#22597,#22598,#22599,#22600,#22601,
#22602,#22603,#22604,#22605,#22606,#22607,#22608,#22609,#22610,#22611,#22612,
#22613,#22614,#22615,#22616,#22617,#22618,#22619,#22620,#22621,#22622,#22623,
#22624,#22625,#22626,#22627,#22628,#22629,#22630,#22631,#22632,#22633,#22634,
#22635,#22636,#22637,#22638,#22639,#22640,#22641,#22642),.UNSPECIFIED.,
 .F.,.F.,(4,3,3,3,3,3,3,3,3,3,3,3,3,3,3,3,3,3,3,3,3,3,3,3,3,3,4),(128.805298797182,
128.830437494887,128.924694627589,129.018823857126,129.1128537095,129.206816082106,
129.300744104803,129.394663406099,129.488599599999,129.582636642893,129.676729035032,
129.770972988163,129.825498689391,129.919754615869,130.013882957705,130.107912237332,
130.201874503625,130.29580270766,130.389722475749,130.483659419942,130.577697636588,
130.671791443048,130.766037172219,130.820559883894,130.914698557345,131.008697567804,
131.031732990453),.UNSPECIFIED.);
#315=B_SPLINE_CURVE_WITH_KNOTS('',3,(#22643,#22644,#22645,#22646,#22647,
#22648,#22649,#22650),.UNSPECIFIED.,.F.,.F.,(4,1,1,1,1,4),(124.747381147578,
124.850192716873,125.845253911376,126.84031510588,127.835376300384,128.805295307034),
 .UNSPECIFIED.);
#316=B_SPLINE_CURVE_WITH_KNOTS('',3,(#22656,#22657,#22658,#22659,#22660,
#22661,#22662,#22663,#22664,#22665,#22666,#22667,#22668,#22669,#22670,#22671,
#22672,#22673,#22674,#22675,#22676,#22677,#22678,#22679,#22680,#22681,#22682,
#22683,#22684,#22685,#22686,#22687,#22688,#22689,#22690,#22691,#22692,#22693,
#22694,#22695,#22696,#22697,#22698,#22699,#22700,#22701,#22702,#22703,#22704,
#22705,#22706,#22707,#22708,#22709,#22710,#22711,#22712,#22713,#22714,#22715,
#22716,#22717,#22718,#22719,#22720,#22721,#22722,#22723,#22724,#22725,#22726,
#22727,#22728,#22729,#22730,#22731,#22732,#22733,#22734,#22735,#22736,#22737,
#22738,#22739,#22740,#22741,#22742,#22743,#22744,#22745,#22746,#22747,#22748,
#22749,#22750,#22751,#22752,#22753,#22754,#22755,#22756,#22757,#22758,#22759,
#22760,#22761,#22762,#22763,#22764,#22765,#22766,#22767,#22768,#22769,#22770,
#22771,#22772,#22773,#22774,#22775,#22776,#22777,#22778,#22779,#22780,#22781,
#22782,#22783,#22784,#22785,#22786,#22787,#22788),.UNSPECIFIED.,.F.,.F.,
(4,3,3,3,3,3,3,3,3,3,3,3,3,3,3,3,3,3,3,3,3,3,3,3,3,3,3,3,3,3,3,3,3,3,3,
3,3,3,3,3,3,3,3,3,4),(118.465298607546,118.559363166675,118.655142504428,
118.749068183104,118.842971185363,118.936877151751,119.034057330988,119.12810108778,
119.226849478239,119.325597868698,119.419836160087,119.513946617396,119.607957790504,
119.701901697558,119.795811393377,119.889712527958,119.983630736934,120.077650179834,
120.171725163178,120.265952179458,120.320659063201,120.414897776923,120.50900865503,
120.603020246869,120.696964567888,120.790874674582,120.884776216466,120.978694828691,
121.072714666242,121.166790039971,121.261017436083,121.315720257705,121.40995935154,
121.504070615355,121.598082597901,121.692027315394,121.785937821971,121.879839766635,
121.97375878403,122.067779027872,122.161854809123,122.256082610628,122.310781452209,
122.44149000973,122.522113490002),.UNSPECIFIED.);
#317=B_SPLINE_CURVE_WITH_KNOTS('',3,(#22789,#22790,#22791,#22792,#22793,
#22794,#22795,#22796,#22797,#22798,#22799,#22800,#22801,#22802,#22803,#22804,
#22805,#22806,#22807,#22808,#22809,#22810,#22811,#22812,#22813,#22814,#22815,
#22816,#22817,#22818,#22819,#22820,#22821,#22822,#22823,#22824,#22825,#22826,
#22827,#22828,#22829,#22830,#22831,#22832,#22833,#22834,#22835,#22836,#22837,
#22838,#22839,#22840,#22841,#22842,#22843,#22844,#22845,#22846,#22847,#22848,
#22849,#22850,#22851,#22852,#22853,#22854,#22855,#22856,#22857,#22858,#22859,
#22860,#22861,#22862,#22863,#22864),.UNSPECIFIED.,.F.,.F.,(4,3,3,3,3,3,
3,3,3,3,3,3,3,3,3,3,3,3,3,3,3,3,3,3,3,4),(122.522113490219,122.614860375032,
122.707527160722,122.800152547904,122.892763516874,122.98538702816,123.078105516595,
123.170877967855,123.26379533639,123.305842646712,123.400083101606,123.494195711582,
123.58820902383,123.682155041317,123.776066829089,123.869970034715,123.963890291383,
124.057911734141,124.15198869332,124.246217628225,124.300903841216,124.395152233769,
124.489249395523,124.583258807334,124.677204221474,124.748116942751),
 .UNSPECIFIED.);
#318=B_SPLINE_CURVE_WITH_KNOTS('',3,(#22866,#22867,#22868,#22869,#22870,
#22871),.UNSPECIFIED.,.F.,.F.,(4,1,1,4),(122.522120559769,122.860070327865,
123.855131522369,124.747381147578),.UNSPECIFIED.);
#319=B_SPLINE_CURVE_WITH_KNOTS('',3,(#22872,#22873,#22874,#22875,#22876,
#22877,#22878,#22879,#22880,#22881,#22882,#22883,#22884,#22885,#22886,#22887,
#22888,#22889,#22890,#22891,#22892,#22893,#22894,#22895,#22896,#22897,#22898,
#22899,#22900,#22901,#22902,#22903,#22904,#22905,#22906,#22907,#22908,#22909,
#22910,#22911,#22912,#22913,#22914,#22915,#22916,#22917,#22918,#22919,#22920,
#22921,#22922,#22923,#22924,#22925,#22926,#22927,#22928,#22929,#22930,#22931,
#22932,#22933,#22934,#22935,#22936,#22937,#22938,#22939,#22940,#22941,#22942,
#22943,#22944,#22945,#22946,#22947,#22948,#22949,#22950,#22951,#22952,#22953,
#22954,#22955,#22956,#22957,#22958,#22959,#22960,#22961,#22962,#22963,#22964,
#22965,#22966,#22967,#22968,#22969,#22970,#22971,#22972,#22973,#22974,#22975,
#22976,#22977,#22978,#22979,#22980,#22981,#22982,#22983,#22984,#22985,#22986,
#22987,#22988,#22989,#22990,#22991,#22992,#22993,#22994,#22995,#22996,#22997,
#22998,#22999,#23000,#23001,#23002,#23003,#23004,#23005,#23006,#23007),
 .UNSPECIFIED.,.F.,.F.,(4,3,3,3,3,3,3,3,3,3,3,3,3,3,3,3,3,3,3,3,3,3,3,3,
3,3,3,3,3,3,3,3,3,3,3,3,3,3,3,3,3,3,3,3,3,4),(118.464533283335,118.558457081294,
118.652484421599,118.74657114206,118.840805385433,118.879825549851,118.974064053571,
119.068174723327,119.162186108714,119.256130226928,119.35004013314,119.443941477094,
119.537859894174,119.631879541979,119.725954728729,119.820181944045,119.874886744355,
119.969125291968,120.063236005371,120.157247434107,120.251191595053,120.3451015436,
120.439002929444,120.532921387917,120.626941076116,120.721016302753,120.81524355677,
120.869947938858,120.964186560255,121.05829734816,121.152308852005,121.246253088645,
121.340163113221,121.434064575333,121.527983110218,121.622002874577,121.716078177344,
121.810305506689,121.865009133362,121.959298109332,122.053461225864,122.147524199852,
122.24151443669,122.335459191593,122.429414396328,122.522113490002),
 .UNSPECIFIED.);
#320=B_SPLINE_CURVE_WITH_KNOTS('',3,(#23013,#23014,#23015,#23016,#23017,
#23018,#23019,#23020,#23021,#23022,#23023,#23024,#23025,#23026,#23027,#23028,
#23029,#23030,#23031,#23032,#23033,#23034,#23035,#23036,#23037,#23038,#23039,
#23040,#23041,#23042,#23043,#23044,#23045,#23046,#23047,#23048,#23049,#23050,
#23051,#23052,#23053,#23054,#23055,#23056,#23057,#23058,#23059,#23060,#23061,
#23062,#23063,#23064,#23065,#23066,#23067,#23068,#23069,#23070,#23071,#23072,
#23073,#23074,#23075,#23076,#23077,#23078,#23079,#23080,#23081,#23082,#23083,
#23084,#23085,#23086,#23087,#23088,#23089,#23090,#23091,#23092,#23093,#23094,
#23095,#23096,#23097,#23098,#23099,#23100,#23101,#23102,#23103,#23104,#23105,
#23106,#23107,#23108,#23109,#23110,#23111,#23112,#23113,#23114,#23115,#23116,
#23117,#23118,#23119,#23120,#23121,#23122,#23123,#23124,#23125,#23126,#23127,
#23128,#23129,#23130,#23131,#23132,#23133,#23134,#23135,#23136,#23137,#23138,
#23139,#23140,#23141,#23142,#23143,#23144,#23145,#23146,#23147,#23148),
 .UNSPECIFIED.,.F.,.F.,(4,3,3,3,3,3,3,3,3,3,3,3,3,3,3,3,3,3,3,3,3,3,3,3,
3,3,3,3,3,3,3,3,3,3,3,3,3,3,3,3,3,3,3,3,3,4),(112.181017173795,112.275233169463,
112.360169507172,112.454408042794,112.548518744449,112.642530161692,112.736474311568,
112.83038424931,112.924285624625,113.018204072858,113.112223751313,113.206298968473,
113.300526213524,113.355230701676,113.449469231835,113.543579928025,113.637591339807,
113.731535484251,113.825445416582,113.919346786512,114.013265229393,114.107284902579,
114.201360114508,114.295587354442,114.35029189618,114.444530430473,114.53864113076,
114.632652546598,114.72659669502,114.820506631279,114.914408005084,115.008326451781,
115.102346128671,115.196421344247,115.290648587701,115.345353090683,115.438408479076,
115.531337065953,115.624161153566,115.71692843708,115.809665818337,115.902400163806,
115.995209723843,116.088059513646,116.181043471339,116.238928182601),
 .UNSPECIFIED.);
#321=B_SPLINE_CURVE_WITH_KNOTS('',3,(#23149,#23150,#23151,#23152,#23153,
#23154,#23155,#23156,#23157,#23158,#23159,#23160,#23161,#23162,#23163,#23164,
#23165,#23166,#23167,#23168,#23169,#23170,#23171,#23172,#23173,#23174,#23175,
#23176,#23177,#23178,#23179,#23180,#23181,#23182,#23183,#23184,#23185,#23186,
#23187,#23188,#23189,#23190,#23191,#23192,#23193,#23194,#23195,#23196,#23197,
#23198,#23199,#23200,#23201,#23202,#23203,#23204,#23205,#23206,#23207,#23208,
#23209,#23210,#23211,#23212,#23213,#23214,#23215,#23216,#23217,#23218,#23219,
#23220,#23221,#23222,#23223,#23224),.UNSPECIFIED.,.F.,.F.,(4,3,3,3,3,3,
3,3,3,3,3,3,3,3,3,3,3,3,3,3,3,3,3,3,3,4),(116.238928182822,116.340414285187,
116.434652788961,116.528763458769,116.622774844209,116.716718962476,116.810628868741,
116.904530212748,116.998448629879,117.092468277736,117.186543464536,117.280770679902,
117.335475479691,117.429714027298,117.523824740696,117.617836169426,117.711780330368,
117.80569027891,117.899591664751,117.993510123221,118.087529811417,118.181605038051,
118.275832292067,118.330536674194,118.424770286337,118.465298607546),
 .UNSPECIFIED.);
#322=B_SPLINE_CURVE_WITH_KNOTS('',3,(#23226,#23227,#23228,#23229,#23230,
#23231,#23232,#23233,#23234,#23235,#23236,#23237,#23238,#23239,#23240,#23241,
#23242,#23243,#23244,#23245,#23246,#23247,#23248,#23249,#23250,#23251,#23252,
#23253,#23254,#23255,#23256,#23257,#23258,#23259,#23260,#23261,#23262,#23263,
#23264,#23265,#23266,#23267,#23268,#23269,#23270,#23271,#23272,#23273,#23274,
#23275,#23276,#23277,#23278,#23279,#23280,#23281,#23282,#23283,#23284,#23285,
#23286,#23287,#23288,#23289,#23290,#23291,#23292,#23293,#23294,#23295,#23296,
#23297,#23298,#23299,#23300,#23301),.UNSPECIFIED.,.F.,.F.,(4,3,3,3,3,3,
3,3,3,3,3,3,3,3,3,3,3,3,3,3,3,3,3,3,3,4),(116.238928182822,116.332983170984,
116.427030095315,116.521094265264,116.615267370442,116.709495278438,116.803894854092,
116.889703160844,116.983941695136,117.078052395421,117.172063811258,117.266007959679,
117.359917895936,117.453819269739,117.547737716434,117.641757393322,117.735832608897,
117.830059852349,117.884764355347,117.978993315107,118.073100941312,118.170959026818,
118.264897087566,118.358795692125,118.452689035773,118.464533283335),
 .UNSPECIFIED.);
#323=B_SPLINE_CURVE_WITH_KNOTS('',3,(#23302,#23303,#23304,#23305,#23306,
#23307,#23308,#23309,#23310,#23311,#23312,#23313,#23314,#23315,#23316,#23317,
#23318,#23319,#23320,#23321,#23322,#23323,#23324,#23325,#23326,#23327,#23328,
#23329,#23330,#23331,#23332,#23333,#23334,#23335,#23336,#23337,#23338,#23339,
#23340,#23341,#23342,#23343,#23344,#23345,#23346,#23347,#23348,#23349,#23350,
#23351,#23352,#23353,#23354,#23355,#23356,#23357,#23358,#23359,#23360,#23361,
#23362,#23363,#23364,#23365,#23366,#23367,#23368,#23369,#23370,#23371,#23372,
#23373,#23374,#23375,#23376,#23377,#23378,#23379,#23380,#23381,#23382,#23383,
#23384,#23385,#23386,#23387,#23388,#23389,#23390,#23391,#23392,#23393,#23394,
#23395,#23396,#23397,#23398,#23399,#23400,#23401,#23402,#23403,#23404,#23405,
#23406,#23407,#23408,#23409,#23410,#23411,#23412,#23413,#23414,#23415,#23416,
#23417,#23418,#23419,#23420,#23421,#23422,#23423,#23424,#23425,#23426,#23427,
#23428,#23429,#23430,#23431,#23432,#23433,#23434,#23435,#23436,#23437),
 .UNSPECIFIED.,.F.,.F.,(4,3,3,3,3,3,3,3,3,3,3,3,3,3,3,3,3,3,3,3,3,3,3,3,
3,3,3,3,3,3,3,3,3,3,3,3,3,3,3,3,3,3,3,3,3,4),(112.182146568534,112.276098342198,
112.370011913038,112.463912934884,112.557827043936,112.651840160733,112.745905233754,
112.840126670004,112.909458382829,113.003696916176,113.09780761555,113.19181903051,
113.285763178109,113.379673113578,113.473574486628,113.567492932605,113.661512608834,
113.755587823779,113.849815066659,113.904519577333,113.998758111003,114.092868810696,
114.186880225968,114.28082437387,114.374734309636,114.468635682976,114.562554129237,
114.656573805737,114.750649020949,114.844876264081,114.899580771837,114.993819307463,
115.087930009123,115.181941426371,115.275885576251,115.369795513998,115.463696889318,
115.557615337555,115.651635016015,115.745710233179,115.839937478235,115.89464196634,
116.00387938609,116.112620366374,116.220504130663,116.238928182603),
 .UNSPECIFIED.);
#324=B_SPLINE_CURVE_WITH_KNOTS('',3,(#23443,#23444,#23445,#23446,#23447,
#23448,#23449,#23450,#23451,#23452,#23453,#23454,#23455,#23456,#23457,#23458,
#23459,#23460,#23461,#23462,#23463,#23464,#23465,#23466,#23467,#23468,#23469,
#23470,#23471,#23472,#23473,#23474,#23475,#23476,#23477,#23478,#23479,#23480,
#23481,#23482,#23483,#23484,#23485,#23486,#23487,#23488,#23489,#23490,#23491,
#23492,#23493,#23494,#23495,#23496,#23497,#23498,#23499,#23500,#23501,#23502,
#23503,#23504,#23505,#23506,#23507,#23508,#23509,#23510,#23511,#23512,#23513,
#23514,#23515,#23516,#23517,#23518,#23519,#23520,#23521,#23522,#23523,#23524,
#23525,#23526,#23527,#23528,#23529,#23530,#23531,#23532,#23533,#23534,#23535,
#23536,#23537,#23538,#23539,#23540,#23541,#23542,#23543,#23544,#23545,#23546,
#23547,#23548,#23549,#23550,#23551,#23552,#23553,#23554,#23555,#23556,#23557,
#23558,#23559,#23560,#23561,#23562,#23563,#23564,#23565,#23566,#23567,#23568,
#23569,#23570,#23571,#23572,#23573,#23574,#23575,#23576,#23577,#23578),
 .UNSPECIFIED.,.F.,.F.,(4,3,3,3,3,3,3,3,3,3,3,3,3,3,3,3,3,3,3,3,3,3,3,3,
3,3,3,3,3,3,3,3,3,3,3,3,3,3,3,3,3,3,3,3,3,4),(105.898388911918,105.992293425444,
106.086224139824,106.180260935269,106.274361476398,106.368604602101,106.389802340151,
106.484040873954,106.578151573784,106.672162989198,106.766107137247,106.860017073163,
106.953918446657,107.047836893075,107.141856569736,107.235931785111,107.330159028408,
107.384863534654,107.479102068375,107.573212768123,107.667224183456,107.761168331424,
107.85507826726,107.948979640674,108.042898087013,108.136917763597,108.230992978894,
108.325220222116,108.379924729158,108.474163262893,108.568273962654,108.662285377998,
108.756229525977,108.850139461823,108.944040835246,109.037959281593,109.131978958184,
109.226054173488,109.320281416716,109.374985923662,109.471046274231,109.566961712461,
109.664157003256,109.759830055412,109.857786465528,109.955742875643),
 .UNSPECIFIED.);
#325=B_SPLINE_CURVE_WITH_KNOTS('',3,(#23579,#23580,#23581,#23582,#23583,
#23584,#23585,#23586,#23587,#23588,#23589,#23590,#23591,#23592,#23593,#23594,
#23595,#23596,#23597,#23598,#23599,#23600,#23601,#23602,#23603,#23604,#23605,
#23606,#23607,#23608,#23609,#23610,#23611,#23612,#23613,#23614,#23615,#23616,
#23617,#23618,#23619,#23620,#23621,#23622,#23623,#23624,#23625,#23626,#23627,
#23628,#23629,#23630,#23631,#23632,#23633,#23634,#23635,#23636,#23637,#23638,
#23639,#23640,#23641,#23642,#23643,#23644,#23645,#23646,#23647,#23648,#23649,
#23650,#23651),.UNSPECIFIED.,.F.,.F.,(4,3,3,3,3,3,3,3,3,3,3,3,3,3,3,3,3,
3,3,3,3,3,3,3,4),(109.955742875827,110.059318936412,110.162337101285,110.266192109725,
110.370047118165,110.464285651513,110.558396350888,110.652407765849,110.746351913449,
110.840261848919,110.934163221969,111.028081667947,111.122101344177,111.216176559123,
111.310403802003,111.365108312669,111.459358828674,111.553452005303,111.64745530481,
111.741394479135,111.835295218455,111.929214837249,112.023142263765,112.11715329755,
112.181017173795),.UNSPECIFIED.);
#326=B_SPLINE_CURVE_WITH_KNOTS('',3,(#23653,#23654,#23655,#23656,#23657,
#23658,#23659,#23660,#23661,#23662,#23663,#23664,#23665,#23666,#23667,#23668,
#23669,#23670,#23671,#23672,#23673,#23674,#23675,#23676,#23677,#23678,#23679,
#23680,#23681,#23682,#23683,#23684,#23685,#23686,#23687,#23688,#23689,#23690,
#23691,#23692,#23693,#23694,#23695,#23696,#23697,#23698,#23699,#23700,#23701,
#23702,#23703,#23704,#23705,#23706,#23707,#23708,#23709,#23710,#23711,#23712,
#23713,#23714,#23715,#23716,#23717,#23718,#23719,#23720,#23721,#23722,#23723,
#23724,#23725,#23726,#23727,#23728),.UNSPECIFIED.,.F.,.F.,(4,3,3,3,3,3,
3,3,3,3,3,3,3,3,3,3,3,3,3,3,3,3,3,3,3,4),(109.955742875862,110.04949173415,
110.143114524302,110.240142207992,110.333603103301,110.427034076366,110.520461333779,
110.613911072019,110.707463740762,110.801077867967,110.894834565712,110.919335993822,
111.013574527556,111.107685227317,111.201696642662,111.29564079064,111.389550726486,
111.483452099909,111.577370546256,111.671390222847,111.765465438151,111.859692681378,
111.914397188326,112.008631127952,112.102725431347,112.182146568534),
 .UNSPECIFIED.);
#327=B_SPLINE_CURVE_WITH_KNOTS('',3,(#23729,#23730,#23731,#23732,#23733,
#23734,#23735,#23736,#23737,#23738,#23739,#23740,#23741,#23742,#23743,#23744,
#23745,#23746,#23747,#23748,#23749,#23750,#23751,#23752,#23753,#23754,#23755,
#23756,#23757,#23758,#23759,#23760,#23761,#23762,#23763,#23764,#23765,#23766,
#23767,#23768,#23769,#23770,#23771,#23772,#23773,#23774,#23775,#23776,#23777,
#23778,#23779,#23780,#23781,#23782,#23783,#23784,#23785,#23786,#23787,#23788,
#23789,#23790,#23791,#23792,#23793,#23794,#23795,#23796,#23797,#23798,#23799,
#23800,#23801,#23802,#23803,#23804,#23805,#23806,#23807,#23808,#23809,#23810,
#23811,#23812,#23813,#23814,#23815,#23816,#23817,#23818,#23819,#23820,#23821,
#23822,#23823,#23824,#23825,#23826,#23827,#23828,#23829,#23830,#23831,#23832,
#23833,#23834,#23835,#23836,#23837,#23838,#23839,#23840,#23841,#23842,#23843,
#23844,#23845,#23846,#23847,#23848,#23849,#23850,#23851,#23852,#23853,#23854,
#23855,#23856,#23857,#23858,#23859,#23860,#23861,#23862,#23863,#23864,#23865,
#23866,#23867),.UNSPECIFIED.,.F.,.F.,(4,3,3,3,3,3,3,3,3,3,3,3,3,3,3,3,3,
3,3,3,3,3,3,3,3,3,3,3,3,3,3,3,3,3,3,3,3,3,3,3,3,3,3,3,3,3,4),(105.898164363444,
105.944030021304,106.038268555077,106.132379254877,106.226390670261,106.320334818279,
106.414244754166,106.50814612763,106.602064574018,106.69608425065,106.790159465995,
106.884386709264,106.939091215808,107.033329749571,107.127440449361,107.221451864736,
107.315396012745,107.409305948622,107.503207322077,107.597125768456,107.691145445079,
107.785220660415,107.879447903675,107.934152410311,108.028390944072,108.12250164386,
108.216513059233,108.31045720724,108.404367143114,108.498268516567,108.592186962943,
108.686206639563,108.780281854897,108.874509098154,108.929213604815,109.023452138618,
109.117562838448,109.211574253862,109.305518401911,109.399428337828,109.493329711322,
109.58724815774,109.681267834401,109.775343049776,109.869570293073,109.924274799319,
109.955742875643),.UNSPECIFIED.);
#328=B_SPLINE_CURVE_WITH_KNOTS('',3,(#23873,#23874,#23875,#23876,#23877,
#23878,#23879,#23880,#23881,#23882,#23883,#23884,#23885,#23886,#23887,#23888,
#23889,#23890,#23891,#23892,#23893,#23894,#23895,#23896,#23897,#23898,#23899,
#23900,#23901,#23902,#23903,#23904,#23905,#23906,#23907,#23908,#23909,#23910,
#23911,#23912,#23913,#23914,#23915,#23916,#23917,#23918,#23919,#23920,#23921,
#23922,#23923,#23924,#23925,#23926,#23927,#23928,#23929,#23930,#23931,#23932,
#23933,#23934,#23935,#23936,#23937,#23938,#23939,#23940,#23941,#23942,#23943,
#23944,#23945,#23946,#23947,#23948,#23949,#23950,#23951,#23952,#23953,#23954,
#23955,#23956,#23957,#23958,#23959,#23960,#23961,#23962,#23963,#23964,#23965,
#23966,#23967,#23968,#23969,#23970,#23971,#23972,#23973,#23974,#23975,#23976,
#23977,#23978,#23979,#23980,#23981,#23982,#23983,#23984,#23985,#23986,#23987,
#23988,#23989,#23990,#23991,#23992,#23993,#23994,#23995,#23996,#23997,#23998,
#23999,#24000,#24001,#24002,#24003,#24004,#24005,#24006,#24007,#24008),
 .UNSPECIFIED.,.F.,.F.,(4,3,3,3,3,3,3,3,3,3,3,3,3,3,3,3,3,3,3,3,3,3,3,3,
3,3,3,3,3,3,3,3,3,3,3,3,3,3,3,3,3,3,3,3,3,4),(99.6158049460037,99.7098135899942,
99.803756210262,99.8976654592765,99.9915669859436,100.085486425495,100.179507555568,
100.273584979423,100.367813533998,100.419435173129,100.513673706898,100.607784406694,
100.701795822074,100.795739970088,100.889649905971,100.983551279431,101.077469725815,
101.171489402443,101.265564617785,101.35979186105,101.414496367633,101.508734901401,
101.602845601196,101.696857016574,101.790801164588,101.88471110047,101.978612473929,
102.072530920312,102.166550596939,102.260625812279,102.354853055544,102.409557562136,
102.503796095903,102.597906795697,102.691918211075,102.785862359088,102.879772294969,
102.973673668427,103.067592114809,103.161611791436,103.255687006775,103.349914250038,
103.40461875664,103.524030082458,103.641345043911,103.67255756827),
 .UNSPECIFIED.);
#329=B_SPLINE_CURVE_WITH_KNOTS('',3,(#24009,#24010,#24011,#24012,#24013,
#24014,#24015,#24016,#24017,#24018,#24019,#24020,#24021,#24022,#24023,#24024,
#24025,#24026,#24027,#24028,#24029,#24030,#24031,#24032,#24033,#24034,#24035,
#24036,#24037,#24038,#24039,#24040,#24041,#24042,#24043,#24044,#24045,#24046,
#24047,#24048,#24049,#24050,#24051,#24052,#24053,#24054,#24055,#24056,#24057,
#24058,#24059,#24060,#24061,#24062,#24063,#24064,#24065,#24066,#24067,#24068,
#24069,#24070,#24071,#24072,#24073,#24074,#24075,#24076,#24077,#24078,#24079,
#24080,#24081,#24082,#24083,#24084),.UNSPECIFIED.,.F.,.F.,(4,3,3,3,3,3,
3,3,3,3,3,3,3,3,3,3,3,3,3,3,3,3,3,3,3,4),(103.672557568463,103.765628528244,
103.858652863645,103.951657206775,104.044668165207,104.137772858336,104.230925480928,
104.324235541546,104.399679951144,104.493918484907,104.588029184698,104.682040600072,
104.775984748081,104.869894683959,104.963796057413,105.057714503792,105.151734180415,
105.245809395752,105.340036639012,105.394741145647,105.488978919694,105.583093549466,
105.677096801156,105.771035905391,105.864939462047,105.898388911918),
 .UNSPECIFIED.);
#330=B_SPLINE_CURVE_WITH_KNOTS('',3,(#24086,#24087,#24088,#24089,#24090,
#24091,#24092,#24093,#24094,#24095,#24096,#24097,#24098,#24099,#24100,#24101,
#24102,#24103,#24104,#24105,#24106,#24107,#24108,#24109,#24110,#24111,#24112,
#24113,#24114,#24115,#24116,#24117,#24118,#24119,#24120,#24121,#24122,#24123,
#24124,#24125,#24126,#24127,#24128,#24129,#24130,#24131,#24132,#24133,#24134,
#24135,#24136,#24137,#24138,#24139,#24140,#24141,#24142,#24143,#24144,#24145,
#24146,#24147,#24148,#24149,#24150,#24151,#24152,#24153,#24154,#24155,#24156,
#24157,#24158),.UNSPECIFIED.,.F.,.F.,(4,3,3,3,3,3,3,3,3,3,3,3,3,3,3,3,3,
3,3,3,3,3,3,3,4),(103.67255756872,103.787765961805,103.90478701078,103.953907632297,
104.048146166065,104.14225686586,104.236268281238,104.330212429252,104.424122365134,
104.518023738593,104.611942184976,104.705961861603,104.800037076944,104.894264320208,
104.9489688268,105.043210275337,105.137323127687,105.232428282157,105.326369980879,
105.420276687691,105.514174051776,105.610171629693,105.704174610095,105.801169486769,
105.898164363444),.UNSPECIFIED.);
#331=B_SPLINE_CURVE_WITH_KNOTS('',3,(#24159,#24160,#24161,#24162,#24163,
#24164,#24165,#24166,#24167,#24168,#24169,#24170,#24171,#24172,#24173,#24174,
#24175,#24176,#24177,#24178,#24179,#24180,#24181,#24182,#24183,#24184,#24185,
#24186,#24187,#24188,#24189,#24190,#24191,#24192,#24193,#24194,#24195,#24196,
#24197,#24198,#24199,#24200,#24201,#24202,#24203,#24204,#24205,#24206,#24207,
#24208,#24209,#24210,#24211,#24212,#24213,#24214,#24215,#24216,#24217,#24218,
#24219,#24220,#24221,#24222,#24223,#24224,#24225,#24226,#24227,#24228,#24229,
#24230,#24231,#24232,#24233,#24234,#24235,#24236,#24237,#24238,#24239,#24240,
#24241,#24242,#24243,#24244,#24245,#24246,#24247,#24248,#24249,#24250,#24251,
#24252,#24253,#24254,#24255,#24256,#24257,#24258,#24259,#24260,#24261,#24262,
#24263,#24264,#24265,#24266,#24267,#24268,#24269,#24270,#24271,#24272,#24273,
#24274,#24275,#24276,#24277,#24278,#24279,#24280,#24281,#24282,#24283,#24284,
#24285,#24286,#24287,#24288,#24289,#24290,#24291,#24292,#24293,#24294),
 .UNSPECIFIED.,.F.,.F.,(4,3,3,3,3,3,3,3,3,3,3,3,3,3,3,3,3,3,3,3,3,3,3,3,
3,3,3,3,3,3,3,3,3,3,3,3,3,3,3,3,3,3,3,3,3,4),(99.614830573868,99.7088406605666,
99.802900937315,99.8971197623276,99.9736628542824,100.067901388051,100.162012087846,
100.256023503225,100.34996765124,100.443877587122,100.537778960582,100.631697406966,
100.725717083593,100.819792298935,100.914019542199,100.968724048786,101.062962582554,
101.157073282349,101.251084697729,101.345028845743,101.438938781625,101.532840155084,
101.626758601468,101.720778278096,101.814853493436,101.909080736701,101.96378524329,
102.058023777058,102.152134476853,102.246145892232,102.340090040246,102.433999976128,
102.527901349588,102.621819795971,102.715839472598,102.809914687939,102.904141931203,
102.958846437793,103.052298003948,103.145631281771,103.238872954843,103.332049611754,
103.425206679406,103.51835021553,103.611545131343,103.672557568463),
 .UNSPECIFIED.);
#332=B_SPLINE_CURVE_WITH_KNOTS('',3,(#24300,#24301,#24302,#24303,#24304,
#24305,#24306,#24307,#24308,#24309,#24310,#24311,#24312,#24313,#24314,#24315,
#24316,#24317,#24318,#24319,#24320,#24321,#24322,#24323,#24324,#24325,#24326,
#24327,#24328,#24329,#24330,#24331,#24332,#24333,#24334,#24335,#24336,#24337,
#24338,#24339,#24340,#24341,#24342,#24343,#24344,#24345,#24346,#24347,#24348,
#24349,#24350,#24351,#24352,#24353,#24354,#24355,#24356,#24357,#24358,#24359,
#24360,#24361,#24362,#24363,#24364,#24365,#24366,#24367,#24368,#24369,#24370,
#24371,#24372,#24373,#24374,#24375,#24376,#24377,#24378,#24379,#24380,#24381,
#24382,#24383,#24384,#24385,#24386,#24387,#24388,#24389,#24390,#24391,#24392,
#24393,#24394,#24395,#24396,#24397,#24398,#24399,#24400,#24401,#24402,#24403,
#24404,#24405,#24406,#24407,#24408,#24409,#24410,#24411,#24412,#24413,#24414,
#24415,#24416,#24417,#24418,#24419,#24420,#24421,#24422,#24423,#24424,#24425,
#24426,#24427,#24428,#24429,#24430,#24431,#24432,#24433,#24434,#24435,#24436,
#24437,#24438),.UNSPECIFIED.,.F.,.F.,(4,3,3,3,3,3,3,3,3,3,3,3,3,3,3,3,3,
3,3,3,3,3,3,3,3,3,3,3,3,3,3,3,3,3,3,3,3,3,3,3,3,3,3,3,3,3,4),(93.3315411447136,
93.4257806413673,93.4540068116039,93.548245345372,93.6423560451674,93.7363674605467,
93.8303116085608,93.924221544443,94.0181229179025,94.1120413642862,94.2060610409136,
94.3001362562545,94.394363499519,94.4490680061075,94.5433065398756,94.637417239671,
94.7314286550504,94.8253728030645,94.9192827389467,95.0131841124063,95.10710255879,
95.2011222354174,95.2951974507582,95.3894246940228,95.4441292006111,95.5383677343792,
95.6324784341746,95.726489849554,95.8204339975681,95.9143439334503,96.0082453069098,
96.1021637532934,96.1961834299208,96.2902586452616,96.3844858885262,96.4391903951147,
96.5327727036348,96.6262277012867,96.7216207712496,96.8149119236732,96.9081721054004,
97.0014277028667,97.0984138423976,97.1917929587827,97.2852342917173,97.3788110498964,
97.3893722609902),.UNSPECIFIED.);
#333=B_SPLINE_CURVE_WITH_KNOTS('',3,(#24439,#24440,#24441,#24442,#24443,
#24444,#24445,#24446,#24447,#24448,#24449,#24450,#24451,#24452,#24453,#24454,
#24455,#24456,#24457,#24458,#24459,#24460,#24461,#24462,#24463,#24464,#24465,
#24466,#24467,#24468,#24469,#24470,#24471,#24472,#24473,#24474,#24475,#24476,
#24477,#24478,#24479,#24480,#24481,#24482,#24483,#24484,#24485,#24486,#24487,
#24488,#24489,#24490,#24491,#24492,#24493,#24494,#24495,#24496,#24497,#24498,
#24499,#24500,#24501,#24502,#24503,#24504,#24505,#24506,#24507,#24508,#24509,
#24510,#24511,#24512,#24513,#24514),.UNSPECIFIED.,.F.,.F.,(4,3,3,3,3,3,
3,3,3,3,3,3,3,3,3,3,3,3,3,3,3,3,3,3,3,4),(97.3893722612835,97.4342515896183,
97.5284901233865,97.6226008231819,97.7166122385613,97.8105563865755,97.9044663224577,
97.9983676959173,98.0922861423011,98.1863058189285,98.2803810342694,98.3746082775341,
98.4293127841219,98.5235513178899,98.6176620176852,98.7116734330645,98.8056175810786,
98.8995275169606,98.9934288904202,99.0873473368038,99.1813670134312,99.275442228772,
99.3696694720365,99.4243739786255,99.5200894623146,99.6158049460037),
 .UNSPECIFIED.);
#334=B_SPLINE_CURVE_WITH_KNOTS('',3,(#24516,#24517,#24518,#24519,#24520,
#24521,#24522,#24523,#24524,#24525,#24526,#24527,#24528,#24529,#24530,#24531,
#24532,#24533,#24534,#24535,#24536,#24537,#24538,#24539,#24540,#24541,#24542,
#24543,#24544,#24545,#24546,#24547,#24548,#24549,#24550,#24551,#24552,#24553,
#24554,#24555,#24556,#24557,#24558,#24559,#24560,#24561,#24562,#24563,#24564,
#24565,#24566,#24567,#24568,#24569,#24570,#24571,#24572,#24573,#24574,#24575,
#24576,#24577,#24578,#24579,#24580,#24581,#24582,#24583,#24584,#24585,#24586,
#24587,#24588,#24589,#24590,#24591),.UNSPECIFIED.,.F.,.F.,(4,3,3,3,3,3,
3,3,3,3,3,3,3,3,3,3,3,3,3,3,3,3,3,3,3,4),(97.3893722612835,97.4846035291451,
97.5798662932485,97.6751835878792,97.7706423523568,97.8661846756541,97.961893063649,
97.9835404652752,98.0777789990433,98.1718896988386,98.2659011142179,98.359845262232,
98.4537551981142,98.5476565715738,98.6415750179575,98.7355946945849,98.8296699099256,
98.9238971531902,98.9786016597788,99.0728248085171,99.1669279658269,99.2609369867913,
99.3548809239173,99.4487849917754,99.5427012429723,99.614830573868),
 .UNSPECIFIED.);
#335=B_SPLINE_CURVE_WITH_KNOTS('',3,(#24592,#24593,#24594,#24595,#24596,
#24597,#24598,#24599,#24600,#24601,#24602,#24603,#24604,#24605,#24606,#24607,
#24608,#24609,#24610,#24611,#24612,#24613,#24614,#24615,#24616,#24617,#24618,
#24619,#24620,#24621,#24622,#24623,#24624,#24625,#24626,#24627,#24628,#24629,
#24630,#24631,#24632,#24633,#24634,#24635,#24636,#24637,#24638,#24639,#24640,
#24641,#24642,#24643,#24644,#24645,#24646,#24647,#24648,#24649,#24650,#24651,
#24652,#24653,#24654,#24655,#24656,#24657,#24658,#24659,#24660,#24661,#24662,
#24663,#24664,#24665,#24666,#24667,#24668,#24669,#24670,#24671,#24672,#24673,
#24674,#24675,#24676,#24677,#24678,#24679,#24680,#24681,#24682,#24683,#24684,
#24685,#24686,#24687,#24688,#24689,#24690,#24691,#24692,#24693,#24694,#24695,
#24696,#24697,#24698,#24699,#24700,#24701,#24702,#24703,#24704,#24705,#24706,
#24707,#24708,#24709,#24710,#24711,#24712,#24713,#24714,#24715,#24716,#24717,
#24718,#24719,#24720,#24721,#24722,#24723,#24724),.UNSPECIFIED.,.F.,.F.,
(4,3,3,3,3,3,3,3,3,3,3,3,3,3,3,3,3,3,3,3,3,3,3,3,3,3,3,3,3,3,3,3,3,3,3,
3,3,3,3,3,3,3,3,3,4),(93.3325033045339,93.4264290221299,93.520331971357,
93.6142377929244,93.7115022665084,93.8055457879678,93.9044207376143,94.0032956872607,
94.0975342210288,94.191644920824,94.2856563362031,94.3796004842171,94.4735104200992,
94.5674117935589,94.6613302399424,94.7553499165697,94.8494251319105,94.9436523751751,
94.9983568817644,95.0925954155325,95.1867061153279,95.280717530707,95.374661678721,
95.4685716146033,95.5624729880632,95.6563914344467,95.750411111074,95.8444863264147,
95.9387135696792,95.9934180762679,96.0876566100358,96.1817673098313,96.2757787252102,
96.3697228732243,96.4636328091064,96.5575341825662,96.6514526289502,96.7454723055776,
96.8395475209183,96.9337747641829,96.9884792707716,97.0928864960786,97.1969961549413,
97.3005780262804,97.3893722610814),.UNSPECIFIED.);
#336=B_SPLINE_CURVE_WITH_KNOTS('',3,(#24730,#24731,#24732,#24733,#24734,
#24735,#24736,#24737,#24738,#24739,#24740,#24741,#24742,#24743,#24744,#24745,
#24746,#24747,#24748,#24749,#24750,#24751,#24752,#24753,#24754,#24755,#24756,
#24757,#24758,#24759,#24760,#24761,#24762,#24763,#24764,#24765,#24766,#24767,
#24768,#24769,#24770,#24771,#24772,#24773,#24774,#24775,#24776,#24777,#24778,
#24779,#24780,#24781,#24782,#24783,#24784,#24785,#24786,#24787,#24788,#24789,
#24790,#24791,#24792,#24793,#24794,#24795,#24796,#24797,#24798,#24799,#24800,
#24801,#24802,#24803,#24804,#24805,#24806,#24807,#24808,#24809,#24810,#24811,
#24812,#24813,#24814,#24815,#24816,#24817,#24818,#24819,#24820,#24821,#24822,
#24823,#24824,#24825,#24826,#24827,#24828,#24829,#24830,#24831,#24832,#24833,
#24834,#24835,#24836,#24837,#24838,#24839,#24840,#24841,#24842,#24843,#24844,
#24845,#24846,#24847,#24848,#24849,#24850,#24851,#24852,#24853,#24854,#24855,
#24856,#24857,#24858,#24859,#24860,#24861,#24862,#24863,#24864,#24865),
 .UNSPECIFIED.,.F.,.F.,(4,3,3,3,3,3,3,3,3,3,3,3,3,3,3,3,3,3,3,3,3,3,3,3,
3,3,3,3,3,3,3,3,3,3,3,3,3,3,3,3,3,3,3,3,3,4),(87.0486631737809,87.1425803605593,
87.2365981702577,87.3306705294207,87.424896100684,87.4836396445822,87.5778781783503,
87.6719888781456,87.7660002935253,87.8599444415394,87.9538543774217,88.0477557508812,
88.1416741972647,88.2356938738921,88.3297690892331,88.4239963324976,88.4787008390858,
88.5729393728539,88.6670500726492,88.7610614880286,88.8550056360427,88.9489155719248,
89.0428169453843,89.1367353917682,89.2307550683955,89.3248302837365,89.4190575270009,
89.4737620335894,89.5680005673576,89.6621112671533,89.7561226825328,89.8500668305468,
89.9439767664289,90.0378781398886,90.1317965862717,90.2258162628992,90.3198914782399,
90.4141187215044,90.468823228093,90.5634949768987,90.6580371372988,90.7524748824259,
90.8468296227406,90.9411345169124,91.0354333352935,91.106186954104),
 .UNSPECIFIED.);
#337=B_SPLINE_CURVE_WITH_KNOTS('',3,(#24866,#24867,#24868,#24869,#24870,
#24871,#24872,#24873,#24874,#24875,#24876,#24877,#24878,#24879,#24880,#24881,
#24882,#24883,#24884,#24885,#24886,#24887,#24888,#24889,#24890,#24891,#24892,
#24893,#24894,#24895,#24896,#24897,#24898,#24899,#24900,#24901,#24902,#24903,
#24904,#24905,#24906,#24907,#24908,#24909,#24910,#24911,#24912,#24913,#24914,
#24915,#24916,#24917,#24918,#24919,#24920,#24921,#24922,#24923,#24924,#24925,
#24926,#24927,#24928,#24929,#24930,#24931,#24932,#24933,#24934,#24935,#24936,
#24937,#24938,#24939,#24940,#24941),.UNSPECIFIED.,.F.,.F.,(4,3,3,3,3,3,
3,3,3,3,3,3,3,3,3,3,3,3,3,3,3,3,3,3,3,4),(91.1061869543297,91.2130644277206,
91.3204667480979,91.4284945161628,91.4638844225966,91.5581229563647,91.6522336561603,
91.7462450715397,91.8401892195538,91.9340991554359,92.0280005288955,92.1219189752793,
92.2159386519067,92.3100138672475,92.404241110512,92.4589456171003,92.5531921681985,
92.6504857902629,92.744486076237,92.8384244481871,92.9323265926773,93.0262181583636,
93.1201623979588,93.21413875603,93.3082140844942,93.3315411447136),
 .UNSPECIFIED.);
#338=B_SPLINE_CURVE_WITH_KNOTS('',3,(#24943,#24944,#24945,#24946,#24947,
#24948,#24949,#24950,#24951,#24952,#24953,#24954,#24955,#24956,#24957,#24958,
#24959,#24960,#24961,#24962,#24963,#24964,#24965,#24966,#24967,#24968,#24969,
#24970,#24971,#24972,#24973,#24974,#24975,#24976,#24977,#24978,#24979,#24980,
#24981,#24982,#24983,#24984,#24985,#24986,#24987,#24988,#24989,#24990,#24991,
#24992,#24993,#24994,#24995,#24996,#24997,#24998,#24999,#25000,#25001,#25002,
#25003,#25004,#25005,#25006,#25007,#25008,#25009,#25010,#25011,#25012,#25013,
#25014,#25015,#25016,#25017,#25018),.UNSPECIFIED.,.F.,.F.,(4,3,3,3,3,3,
3,3,3,3,3,3,3,3,3,3,3,3,3,3,3,3,3,3,3,4),(91.10618695432,91.1992936832594,
91.29228331494,91.3851832836713,91.4780353414083,91.5708662949906,91.6637029252771,
91.7566310763317,91.8496066804956,91.9427360265074,92.0131732982535,92.1074118320216,
92.2015225318168,92.2955339471963,92.3894780952104,92.4833880310926,92.5772894045521,
92.6712078509361,92.7652275275635,92.8593027429045,92.9535299861691,93.0082344927571,
93.102456462241,93.1965663039992,93.2905714705558,93.3325033045339),
 .UNSPECIFIED.);
#339=B_SPLINE_CURVE_WITH_KNOTS('',3,(#25019,#25020,#25021,#25022,#25023,
#25024,#25025,#25026,#25027,#25028,#25029,#25030,#25031,#25032,#25033,#25034,
#25035,#25036,#25037,#25038,#25039,#25040,#25041,#25042,#25043,#25044,#25045,
#25046,#25047,#25048,#25049,#25050,#25051,#25052,#25053,#25054,#25055,#25056,
#25057,#25058,#25059,#25060,#25061,#25062,#25063,#25064,#25065,#25066,#25067,
#25068,#25069,#25070,#25071,#25072,#25073,#25074,#25075,#25076,#25077,#25078,
#25079,#25080,#25081,#25082,#25083,#25084,#25085,#25086,#25087,#25088,#25089,
#25090,#25091,#25092,#25093,#25094,#25095,#25096,#25097,#25098,#25099,#25100,
#25101,#25102,#25103,#25104,#25105,#25106,#25107,#25108,#25109,#25110,#25111,
#25112,#25113,#25114,#25115,#25116,#25117,#25118,#25119,#25120,#25121,#25122,
#25123,#25124,#25125,#25126,#25127,#25128,#25129,#25130,#25131,#25132,#25133,
#25134,#25135,#25136,#25137,#25138,#25139,#25140,#25141,#25142,#25143,#25144,
#25145,#25146,#25147,#25148,#25149,#25150,#25151,#25152,#25153,#25154),
 .UNSPECIFIED.,.F.,.F.,(4,3,3,3,3,3,3,3,3,3,3,3,3,3,3,3,3,3,3,3,3,3,3,3,
3,3,3,3,3,3,3,3,3,3,3,3,3,3,3,3,3,3,3,3,3,4),(87.0489171655824,87.1431392396,
87.2372368316046,87.3312384766754,87.425177288261,87.5190848946421,87.6129869427592,
87.7069090676515,87.8009340558435,87.8950172831459,87.9892493561579,88.0329285202391,
88.1271670540072,88.2212777538026,88.315289169182,88.4092333171961,88.5031432530783,
88.5970446265378,88.6909630729216,88.784982749549,88.8790579648898,88.9732852081544,
89.0279897147427,89.1222282485108,89.2163389483061,89.3103503636855,89.4042945116996,
89.4982044475817,89.5921058210413,89.6860242674251,89.7800439440525,89.8741191593933,
89.9683464026579,90.0230509092463,90.1172894430144,90.2114001428099,90.3054115581892,
90.3993557062033,90.4932656420854,90.587167015545,90.6810854619286,90.775105138556,
90.8691803538968,90.9634075971614,91.0181121037499,91.106186954104),
 .UNSPECIFIED.);
#340=B_SPLINE_CURVE_WITH_KNOTS('',3,(#25160,#25161,#25162,#25163,#25164,
#25165,#25166,#25167,#25168,#25169,#25170,#25171,#25172,#25173,#25174,#25175,
#25176,#25177,#25178,#25179,#25180,#25181,#25182,#25183,#25184,#25185,#25186,
#25187,#25188,#25189,#25190,#25191,#25192,#25193,#25194,#25195,#25196,#25197,
#25198,#25199,#25200,#25201,#25202,#25203,#25204,#25205,#25206,#25207,#25208,
#25209,#25210,#25211,#25212,#25213,#25214,#25215,#25216,#25217,#25218,#25219,
#25220,#25221,#25222,#25223,#25224,#25225,#25226,#25227,#25228,#25229,#25230,
#25231,#25232,#25233,#25234,#25235,#25236,#25237,#25238,#25239,#25240,#25241,
#25242,#25243,#25244,#25245,#25246,#25247,#25248,#25249,#25250,#25251,#25252,
#25253,#25254,#25255,#25256,#25257,#25258,#25259,#25260,#25261,#25262,#25263,
#25264,#25265,#25266,#25267,#25268,#25269,#25270,#25271,#25272,#25273,#25274,
#25275,#25276,#25277,#25278,#25279,#25280,#25281,#25282,#25283,#25284,#25285,
#25286,#25287,#25288,#25289,#25290,#25291,#25292),.UNSPECIFIED.,.F.,.F.,
(4,3,3,3,3,3,3,3,3,3,3,3,3,3,3,3,3,3,3,3,3,3,3,3,3,3,3,3,3,3,3,3,3,3,3,
3,3,3,3,3,3,3,3,3,4),(80.7662383708046,80.8602014204436,80.954120879801,
81.0480224090736,81.1419316464207,81.2359367913877,81.329989058716,81.4242037444454,
81.5132724775605,81.6075110113286,81.701621711124,81.795633126503,81.8895772745172,
81.9834872103992,82.0773885838586,82.1713070302423,82.2653267068696,82.3594019222105,
82.4536291654751,82.5083336720641,82.6025722058321,82.6966829056277,82.7906943210076,
82.8846384690217,82.9785484049038,83.0724497783633,83.1663682247469,83.2603879013744,
83.3544631167152,83.4486903599797,83.5033948665677,83.5976334003357,83.6917441001312,
83.7857555155109,83.879699663525,83.9736095994071,84.0675109728667,84.1614294192501,
84.2554490958774,84.3495243112181,84.4437515544826,84.4984560610714,84.6098153997746,
84.7200586670639,84.8230016467217),.UNSPECIFIED.);
#341=B_SPLINE_CURVE_WITH_KNOTS('',3,(#25293,#25294,#25295,#25296,#25297,
#25298,#25299,#25300,#25301,#25302,#25303,#25304,#25305,#25306,#25307,#25308,
#25309,#25310,#25311,#25312,#25313,#25314,#25315,#25316,#25317,#25318,#25319,
#25320,#25321,#25322,#25323,#25324,#25325,#25326,#25327,#25328,#25329,#25330,
#25331,#25332,#25333,#25334,#25335,#25336,#25337,#25338,#25339,#25340,#25341,
#25342,#25343,#25344,#25345,#25346,#25347,#25348,#25349,#25350,#25351,#25352,
#25353,#25354,#25355,#25356,#25357,#25358,#25359,#25360,#25361,#25362,#25363,
#25364,#25365,#25366,#25367,#25368),.UNSPECIFIED.,.F.,.F.,(4,3,3,3,3,3,
3,3,3,3,3,3,3,3,3,3,3,3,3,3,3,3,3,3,3,4),(84.8230016469244,84.9167396222475,
85.0104582715234,85.1041833778223,85.2015168472605,85.2953896866708,85.3893326790537,
85.4834206132759,85.493517255575,85.5877557893431,85.6818664891387,85.775877904518,
85.8698220525321,85.9637319884143,86.0576333618738,86.1515518082575,86.2455714848849,
86.3396467002259,86.4338739434905,86.4885784500786,86.5828095682953,86.6769188848032,
86.7709219407424,86.8648613808132,86.9587807515315,87.0486631737809),
 .UNSPECIFIED.);
#342=B_SPLINE_CURVE_WITH_KNOTS('',3,(#25370,#25371,#25372,#25373,#25374,
#25375,#25376,#25377,#25378,#25379,#25380,#25381,#25382,#25383,#25384,#25385,
#25386,#25387,#25388,#25389,#25390,#25391,#25392,#25393,#25394,#25395,#25396,
#25397,#25398,#25399,#25400,#25401,#25402,#25403,#25404,#25405,#25406,#25407,
#25408,#25409,#25410,#25411,#25412,#25413,#25414,#25415,#25416,#25417,#25418,
#25419,#25420,#25421,#25422,#25423,#25424,#25425,#25426,#25427,#25428,#25429,
#25430,#25431,#25432,#25433,#25434,#25435,#25436,#25437,#25438,#25439,#25440,
#25441,#25442,#25443,#25444,#25445),.UNSPECIFIED.,.F.,.F.,(4,3,3,3,3,3,
3,3,3,3,3,3,3,3,3,3,3,3,3,3,3,3,3,3,3,4),(84.8230016469244,84.9501148314948,
85.0477449367282,85.1419834704963,85.2360941702917,85.330105585671,85.4240497336852,
85.5179596695673,85.6118610430269,85.7057794894107,85.7997991660381,85.893874381379,
85.9881016246435,86.0428061312318,86.1370446649999,86.2311553647953,86.3251667801747,
86.4191109281888,86.5130208640709,86.6069222375305,86.7008406839142,86.7948603605416,
86.8889355758824,86.983162819147,87.0378673257354,87.0489171655824),
 .UNSPECIFIED.);
#343=B_SPLINE_CURVE_WITH_KNOTS('',3,(#25446,#25447,#25448,#25449,#25450,
#25451,#25452,#25453,#25454,#25455,#25456,#25457,#25458,#25459,#25460,#25461,
#25462,#25463,#25464,#25465,#25466,#25467,#25468,#25469,#25470,#25471,#25472,
#25473,#25474,#25475,#25476,#25477,#25478,#25479,#25480,#25481,#25482,#25483,
#25484,#25485,#25486,#25487,#25488,#25489,#25490,#25491,#25492,#25493,#25494,
#25495,#25496,#25497,#25498,#25499,#25500,#25501,#25502,#25503,#25504,#25505,
#25506,#25507,#25508,#25509,#25510,#25511,#25512,#25513,#25514,#25515,#25516,
#25517,#25518,#25519,#25520,#25521,#25522,#25523,#25524,#25525,#25526,#25527,
#25528,#25529,#25530,#25531,#25532,#25533,#25534,#25535,#25536,#25537,#25538,
#25539,#25540,#25541,#25542,#25543,#25544,#25545,#25546,#25547,#25548,#25549,
#25550,#25551,#25552,#25553,#25554,#25555,#25556,#25557,#25558,#25559,#25560,
#25561,#25562,#25563,#25564,#25565,#25566,#25567,#25568,#25569,#25570,#25571,
#25572,#25573,#25574,#25575,#25576,#25577,#25578,#25579,#25580,#25581,#25582,
#25583,#25584),.UNSPECIFIED.,.F.,.F.,(4,3,3,3,3,3,3,3,3,3,3,3,3,3,3,3,3,
3,3,3,3,3,3,3,3,3,3,3,3,3,3,3,3,3,3,3,3,3,3,3,3,3,3,3,3,3,4),(80.7651606363239,
80.8591981217149,80.9532996567776,81.047543439675,81.0675001587138,81.161738692482,
81.2558493922774,81.3498608076566,81.4438049556707,81.5377148915528,81.6316162650124,
81.7255347113963,81.8195543880237,81.9136296033645,82.007856846629,82.0625613532174,
82.1567998869855,82.2509105867808,82.34492200216,82.4388661501741,82.5327760860562,
82.6266774595158,82.7205959058996,82.8146155825271,82.908690797868,83.0029180411326,
83.057622547721,83.151861081489,83.2459717812843,83.3399831966636,83.4339273446778,
83.52783728056,83.6217386540197,83.7156571004035,83.8096767770308,83.9037519923715,
83.997979235636,84.0526837422246,84.1489734802914,84.241821690845,84.3345840307345,
84.4272875189037,84.5199591070544,84.6126557703783,84.7053683378321,84.7981603124173,
84.8230016467593),.UNSPECIFIED.);
#344=B_SPLINE_CURVE_WITH_KNOTS('',3,(#25590,#25591,#25592,#25593,#25594,
#25595,#25596,#25597,#25598,#25599,#25600,#25601,#25602,#25603,#25604,#25605,
#25606,#25607,#25608,#25609,#25610,#25611,#25612,#25613,#25614,#25615,#25616,
#25617,#25618,#25619,#25620,#25621,#25622,#25623,#25624,#25625,#25626,#25627,
#25628,#25629,#25630,#25631,#25632,#25633,#25634,#25635,#25636,#25637,#25638,
#25639,#25640,#25641,#25642,#25643,#25644,#25645,#25646,#25647,#25648,#25649,
#25650,#25651,#25652,#25653,#25654,#25655,#25656,#25657,#25658,#25659,#25660,
#25661,#25662,#25663,#25664,#25665,#25666,#25667,#25668,#25669,#25670,#25671,
#25672,#25673,#25674,#25675,#25676,#25677,#25678,#25679,#25680,#25681,#25682,
#25683,#25684,#25685,#25686,#25687,#25688,#25689,#25690,#25691,#25692,#25693,
#25694,#25695,#25696,#25697,#25698,#25699,#25700,#25701,#25702,#25703,#25704,
#25705,#25706,#25707,#25708,#25709,#25710,#25711,#25712,#25713,#25714,#25715,
#25716,#25717,#25718,#25719,#25720,#25721,#25722,#25723,#25724,#25725,#25726,
#25727,#25728),.UNSPECIFIED.,.F.,.F.,(4,3,3,3,3,3,3,3,3,3,3,3,3,3,3,3,3,
3,3,3,3,3,3,3,3,3,3,3,3,3,3,3,3,3,3,3,3,3,3,3,3,3,3,3,3,3,4),(74.4821549297256,
74.5478441160352,74.6420826498033,74.7361933495987,74.8302047649781,74.9241489129923,
75.0180588488744,75.111960222334,75.2058786687177,75.2998983453451,75.393973560686,
75.4882008039505,75.5429053105389,75.637143844307,75.7312545441024,75.8252659594818,
75.9192101074959,76.0131200433781,76.1070214168377,76.2009398632214,76.2949595398488,
76.3890347551896,76.4832619984542,76.5379665050425,76.6322050388106,76.726315738606,
76.8203271539855,76.9142713019996,77.0081812378817,77.1020826113412,77.1960010577249,
77.2900207343523,77.3840959496932,77.4783231929578,77.5330276995461,77.6272662333142,
77.7213769331097,77.815388348489,77.9093324965031,78.0032424323852,78.0971438058448,
78.1910622522284,78.2850819288558,78.3791571441966,78.4733843874612,78.5280888940497,
78.5398163397448),.UNSPECIFIED.);
#345=B_SPLINE_CURVE_WITH_KNOTS('',3,(#25729,#25730,#25731,#25732,#25733,
#25734,#25735,#25736,#25737,#25738,#25739,#25740,#25741,#25742,#25743,#25744,
#25745,#25746,#25747,#25748,#25749,#25750,#25751,#25752,#25753,#25754,#25755,
#25756,#25757,#25758,#25759,#25760,#25761,#25762,#25763,#25764,#25765,#25766,
#25767,#25768,#25769,#25770,#25771,#25772,#25773,#25774,#25775,#25776,#25777,
#25778,#25779,#25780,#25781,#25782,#25783,#25784,#25785,#25786,#25787,#25788,
#25789,#25790,#25791,#25792,#25793,#25794,#25795,#25796,#25797,#25798,#25799,
#25800,#25801,#25802,#25803,#25804),.UNSPECIFIED.,.F.,.F.,(4,3,3,3,3,3,
3,3,3,3,3,3,3,3,3,3,3,3,3,3,3,3,3,3,3,4),(78.5398163399313,78.6338611329994,
78.7277784185812,78.8215970086099,78.9153494266275,79.0090686505241,79.1027805640751,
79.1965110377571,79.2903430660188,79.3842324146997,79.4782706044405,79.5231500885533,
79.6173886223214,79.7114993221168,79.8055107374961,79.8994548855102,79.9933648213924,
80.0872661948518,80.1811846412358,80.2752043178631,80.3692795332041,80.4635067764686,
80.5182112830569,80.6124500013097,80.7065483084735,80.7662383708046),
 .UNSPECIFIED.);
#346=B_SPLINE_CURVE_WITH_KNOTS('',3,(#25806,#25807,#25808,#25809,#25810,
#25811,#25812,#25813,#25814,#25815,#25816,#25817,#25818,#25819,#25820,#25821,
#25822,#25823,#25824,#25825,#25826,#25827,#25828,#25829,#25830,#25831,#25832,
#25833,#25834,#25835,#25836,#25837,#25838,#25839,#25840,#25841,#25842,#25843,
#25844,#25845,#25846,#25847,#25848,#25849,#25850,#25851,#25852,#25853,#25854,
#25855,#25856,#25857,#25858,#25859,#25860,#25861,#25862,#25863,#25864,#25865,
#25866,#25867,#25868,#25869,#25870,#25871,#25872,#25873,#25874,#25875,#25876,
#25877,#25878,#25879,#25880,#25881),.UNSPECIFIED.,.F.,.F.,(4,3,3,3,3,3,
3,3,3,3,3,3,3,3,3,3,3,3,3,3,3,3,3,3,3,4),(78.5398163397448,78.6366735783784,
78.7336184927698,78.8307516518218,78.9279875108045,79.0254289346791,79.0773777697065,
79.1716163034746,79.26572700327,79.3597384186493,79.4536825666634,79.5475925025456,
79.6414938760053,79.7354123223889,79.8294319990163,79.9235072143572,80.0177344576217,
80.0724389642102,80.1666569505644,80.2607562877407,80.3547628245391,80.4487023217272,
80.5426132656405,80.6365078669387,80.7304367289939,80.7651606363239),
 .UNSPECIFIED.);
#347=B_SPLINE_CURVE_WITH_KNOTS('',3,(#25882,#25883,#25884,#25885,#25886,
#25887,#25888,#25889,#25890,#25891,#25892,#25893,#25894,#25895,#25896,#25897,
#25898,#25899,#25900,#25901,#25902,#25903,#25904,#25905,#25906,#25907,#25908,
#25909,#25910,#25911,#25912,#25913,#25914,#25915,#25916,#25917,#25918,#25919,
#25920,#25921,#25922,#25923,#25924,#25925,#25926,#25927,#25928,#25929,#25930,
#25931,#25932,#25933,#25934,#25935,#25936,#25937,#25938,#25939,#25940,#25941,
#25942,#25943,#25944,#25945,#25946,#25947,#25948,#25949,#25950,#25951,#25952,
#25953,#25954,#25955,#25956,#25957,#25958,#25959,#25960,#25961,#25962,#25963,
#25964,#25965,#25966,#25967,#25968,#25969,#25970,#25971,#25972,#25973,#25974,
#25975,#25976,#25977,#25978,#25979,#25980,#25981,#25982,#25983,#25984,#25985,
#25986,#25987,#25988,#25989,#25990,#25991,#25992,#25993,#25994,#25995,#25996,
#25997,#25998,#25999,#26000,#26001,#26002,#26003,#26004,#26005,#26006,#26007,
#26008,#26009,#26010,#26011,#26012,#26013,#26014,#26015,#26016,#26017),
 .UNSPECIFIED.,.F.,.F.,(4,3,3,3,3,3,3,3,3,3,3,3,3,3,3,3,3,3,3,3,3,3,3,3,
3,3,3,3,3,3,3,3,3,3,3,3,3,3,3,3,3,3,3,3,3,4),(74.4828190591072,74.5767280122671,
74.6706296157027,74.7645495046023,74.8585712872853,74.952649698683,75.0468788446621,
75.0971329916921,75.1913715254602,75.2854822252557,75.3794936406352,75.4734377886494,
75.5673477245314,75.6612490979911,75.755167544375,75.8491872210025,75.9432624363433,
76.0374896796078,76.0921941861957,76.1864327199638,76.2805434197591,76.3745548351389,
76.468498983153,76.5624089190352,76.6563102924947,76.7502287388782,76.8442484155056,
76.9383236308464,77.0325508741109,77.0872553806993,77.1814939144675,77.2756046142628,
77.3696160296426,77.4635601776567,77.5574701135388,77.6513714869983,77.7452899333823,
77.8393096100098,77.9333848253505,78.0276120686152,78.082316575203,78.1833244724824,
78.2840046924094,78.3844817302127,78.4846682932388,78.5398163395429),
 .UNSPECIFIED.);
#348=B_SPLINE_CURVE_WITH_KNOTS('',3,(#26023,#26024,#26025,#26026,#26027,
#26028,#26029,#26030,#26031,#26032,#26033,#26034,#26035,#26036,#26037,#26038,
#26039,#26040,#26041,#26042,#26043,#26044,#26045,#26046,#26047,#26048,#26049,
#26050,#26051,#26052,#26053,#26054,#26055,#26056,#26057,#26058,#26059,#26060,
#26061,#26062,#26063,#26064,#26065,#26066,#26067,#26068,#26069,#26070,#26071,
#26072,#26073,#26074,#26075,#26076,#26077,#26078,#26079,#26080,#26081,#26082,
#26083,#26084,#26085,#26086,#26087,#26088,#26089,#26090,#26091,#26092,#26093,
#26094,#26095,#26096,#26097,#26098,#26099,#26100,#26101,#26102,#26103,#26104,
#26105,#26106,#26107,#26108,#26109,#26110,#26111,#26112,#26113,#26114,#26115,
#26116,#26117,#26118,#26119,#26120,#26121,#26122,#26123,#26124,#26125,#26126,
#26127,#26128,#26129,#26130,#26131,#26132,#26133,#26134,#26135,#26136,#26137,
#26138,#26139,#26140,#26141,#26142,#26143,#26144,#26145,#26146,#26147,#26148,
#26149,#26150,#26151,#26152,#26153,#26154,#26155,#26156,#26157,#26158),
 .UNSPECIFIED.,.F.,.F.,(4,3,3,3,3,3,3,3,3,3,3,3,3,3,3,3,3,3,3,3,3,3,3,3,
3,3,3,3,3,3,3,3,3,3,3,3,3,3,3,3,3,3,3,3,3,4),(68.1989521886483,68.2935833787396,
68.3876316115364,68.482554280275,68.5774769490136,68.6717154827817,68.7658261825771,
68.8598375979564,68.9537817459705,69.0476916818527,69.1415930553122,69.2355115016959,
69.3295311783233,69.4236063936641,69.5178336369287,69.5725381435172,69.6667766772854,
69.7608873770811,69.8548987924605,69.9488429404746,70.0427528763567,70.136654249816,
70.2305726961998,70.3245923728273,70.418667588168,70.5128948314325,70.5675993380208,
70.6618378717889,70.7559485715847,70.849959986964,70.943904134978,71.0378140708604,
71.1317154443199,71.2256338907041,71.3196535673314,71.4137287826723,71.5079560259368,
71.5626605325244,71.6563624008107,71.7499437866432,71.8434311143557,71.9368507142558,
72.0302428754377,72.1236189950162,72.2170329468858,72.2566310325651),
 .UNSPECIFIED.);
#349=B_SPLINE_CURVE_WITH_KNOTS('',3,(#26159,#26160,#26161,#26162,#26163,
#26164,#26165,#26166,#26167,#26168,#26169,#26170,#26171,#26172,#26173,#26174,
#26175,#26176,#26177,#26178,#26179,#26180,#26181,#26182,#26183,#26184,#26185,
#26186,#26187,#26188,#26189,#26190,#26191,#26192,#26193,#26194,#26195,#26196,
#26197,#26198,#26199,#26200,#26201,#26202,#26203,#26204,#26205,#26206,#26207,
#26208,#26209,#26210,#26211,#26212,#26213,#26214,#26215,#26216,#26217,#26218,
#26219,#26220,#26221,#26222,#26223,#26224,#26225,#26226,#26227,#26228,#26229,
#26230,#26231),.UNSPECIFIED.,.F.,.F.,(4,3,3,3,3,3,3,3,3,3,3,3,3,3,3,3,3,
3,3,3,3,3,3,3,4),(72.2566310327337,72.3692721053914,72.4833775848208,72.557721727028,
72.6519602607961,72.7460709605916,72.8400823759709,72.934026523985,73.0279364598672,
73.1218378333268,73.2157562797105,73.3097759563379,73.4038511716787,73.4980784149432,
73.5527829215316,73.6470256624285,73.7411394776692,73.8351424981322,73.9290840728993,
74.022989888567,74.1168855945947,74.2108478893634,74.3048420661471,74.3989695987264,
74.4821549297256),.UNSPECIFIED.);
#350=B_SPLINE_CURVE_WITH_KNOTS('',3,(#26233,#26234,#26235,#26236,#26237,
#26238,#26239,#26240,#26241,#26242,#26243,#26244,#26245,#26246,#26247,#26248,
#26249,#26250,#26251,#26252,#26253,#26254,#26255,#26256,#26257,#26258,#26259,
#26260,#26261,#26262,#26263,#26264,#26265,#26266,#26267,#26268,#26269,#26270,
#26271,#26272,#26273,#26274,#26275,#26276,#26277,#26278,#26279,#26280,#26281,
#26282,#26283,#26284,#26285,#26286,#26287,#26288,#26289,#26290,#26291,#26292,
#26293,#26294,#26295,#26296,#26297,#26298,#26299,#26300,#26301,#26302,#26303,
#26304,#26305,#26306,#26307,#26308),.UNSPECIFIED.,.F.,.F.,(4,3,3,3,3,3,
3,3,3,3,3,3,3,3,3,3,3,3,3,3,3,3,3,3,3,4),(72.2566310327574,72.3493964521512,
72.4440982209679,72.5366897572247,72.6292473245243,72.7217979449971,72.8181011094191,
72.9107727200092,73.0035061356872,73.0963757548764,73.1070106026849,73.2012491364529,
73.2953598362483,73.3893712516278,73.4833153996419,73.577225335524,73.6711267089834,
73.7650451553672,73.8590648319946,73.9531400473355,74.0473672906001,74.1020717971885,
74.1972586126682,74.2913585663729,74.3870888127401,74.4828190591072),
 .UNSPECIFIED.);
#351=B_SPLINE_CURVE_WITH_KNOTS('',3,(#26309,#26310,#26311,#26312,#26313,
#26314,#26315,#26316,#26317,#26318,#26319,#26320,#26321,#26322,#26323,#26324,
#26325,#26326,#26327,#26328,#26329,#26330,#26331,#26332,#26333,#26334,#26335,
#26336,#26337,#26338,#26339,#26340,#26341,#26342,#26343,#26344,#26345,#26346,
#26347,#26348,#26349,#26350,#26351,#26352,#26353,#26354,#26355,#26356,#26357,
#26358,#26359,#26360,#26361,#26362,#26363,#26364,#26365,#26366,#26367,#26368,
#26369,#26370,#26371,#26372,#26373,#26374,#26375,#26376,#26377,#26378,#26379,
#26380,#26381,#26382,#26383,#26384,#26385,#26386,#26387,#26388,#26389,#26390,
#26391,#26392,#26393,#26394,#26395,#26396,#26397,#26398,#26399,#26400,#26401,
#26402,#26403,#26404,#26405,#26406,#26407,#26408,#26409,#26410,#26411,#26412,
#26413,#26414,#26415,#26416,#26417,#26418,#26419,#26420,#26421,#26422,#26423,
#26424,#26425,#26426,#26427,#26428,#26429,#26430,#26431,#26432,#26433,#26434,
#26435,#26436,#26437,#26438,#26439,#26440,#26441),.UNSPECIFIED.,.F.,.F.,
(4,3,3,3,3,3,3,3,3,3,3,3,3,3,3,3,3,3,3,3,3,3,3,3,3,3,3,3,3,3,3,3,3,3,3,
3,3,3,3,3,3,3,3,3,4),(68.1996305298463,68.293774062422,68.3878103472842,
68.4817686413498,68.5756855520616,68.6695867368963,68.7634978330989,68.8575061207158,
68.9515635104959,69.0457808101111,69.1267658246704,69.2210043584385,69.3151150582339,
69.4091264736133,69.5030706216274,69.5969805575096,69.6908819309691,69.7848003773529,
69.8788200539803,69.9728952693211,70.0671225125857,70.121827019174,70.2160655529421,
70.3101762527375,70.4041876681169,70.498131816131,70.5920417520132,70.6859431254727,
70.7798615718566,70.8738812484839,70.9679564638248,71.0621837070894,71.1168882136777,
71.2111267474458,71.3052374472412,71.3992488626206,71.4931930106347,71.5871029465169,
71.6810043199765,71.7749227663603,71.8689424429877,71.9630176583286,72.0572449015932,
72.1119494081813,72.2566310325651),.UNSPECIFIED.);
#352=B_SPLINE_CURVE_WITH_KNOTS('',3,(#26447,#26448,#26449,#26450,#26451,
#26452,#26453,#26454,#26455,#26456,#26457,#26458,#26459,#26460,#26461,#26462,
#26463,#26464,#26465,#26466,#26467,#26468,#26469,#26470,#26471,#26472,#26473,
#26474,#26475,#26476,#26477,#26478,#26479,#26480,#26481,#26482,#26483,#26484,
#26485,#26486,#26487,#26488,#26489,#26490,#26491,#26492,#26493,#26494,#26495,
#26496,#26497,#26498,#26499,#26500,#26501,#26502,#26503,#26504,#26505,#26506,
#26507,#26508,#26509,#26510,#26511,#26512,#26513,#26514,#26515,#26516,#26517,
#26518,#26519,#26520,#26521,#26522,#26523,#26524,#26525,#26526,#26527,#26528,
#26529,#26530,#26531,#26532,#26533,#26534,#26535,#26536,#26537,#26538,#26539,
#26540,#26541,#26542,#26543,#26544,#26545,#26546,#26547,#26548,#26549,#26550,
#26551,#26552,#26553,#26554,#26555,#26556,#26557,#26558,#26559,#26560,#26561,
#26562,#26563,#26564,#26565,#26566,#26567,#26568,#26569,#26570,#26571,#26572,
#26573,#26574,#26575,#26576,#26577,#26578,#26579,#26580,#26581,#26582),
 .UNSPECIFIED.,.F.,.F.,(4,3,3,3,3,3,3,3,3,3,3,3,3,3,3,3,3,3,3,3,3,3,3,3,
3,3,3,3,3,3,3,3,3,3,3,3,3,3,3,3,3,3,3,3,3,4),(61.9166125687905,62.0105463165949,
62.1044519156713,62.1983550104404,62.292281235926,62.3863119480559,62.480403645108,
62.5746410275793,62.6071097819919,62.7013483157599,62.7954590155553,62.8894704309345,
62.9834145789486,63.0773245148308,63.1712258882903,63.2651443346738,63.3591640113012,
63.4532392266421,63.5474664699067,63.6021709764955,63.6964095102636,63.7905202100592,
63.8845316254386,63.9784757734527,64.072385709335,64.1662870827944,64.2602055291778,
64.3542252058052,64.4483004211459,64.5425276644105,64.5972321709991,64.6914707047674,
64.7855814045625,64.8795928199422,64.9735369679563,65.0674469038384,65.1613482772981,
65.2552667236817,65.3492864003091,65.44336161565,65.5375888589146,65.5922933655027,
65.6982067190135,65.803770718088,65.9087146730012,65.9734457251659),
 .UNSPECIFIED.);
#353=B_SPLINE_CURVE_WITH_KNOTS('',3,(#26583,#26584,#26585,#26586,#26587,
#26588,#26589,#26590,#26591,#26592,#26593,#26594,#26595,#26596,#26597,#26598,
#26599,#26600,#26601,#26602,#26603,#26604,#26605,#26606,#26607,#26608,#26609,
#26610,#26611,#26612,#26613,#26614,#26615,#26616,#26617,#26618,#26619,#26620,
#26621,#26622,#26623,#26624,#26625,#26626,#26627,#26628,#26629,#26630,#26631,
#26632,#26633,#26634,#26635,#26636,#26637,#26638,#26639,#26640,#26641,#26642,
#26643,#26644,#26645,#26646,#26647,#26648,#26649,#26650,#26651,#26652,#26653,
#26654,#26655,#26656,#26657,#26658),.UNSPECIFIED.,.F.,.F.,(4,3,3,3,3,3,
3,3,3,3,3,3,3,3,3,3,3,3,3,3,3,3,3,3,3,4),(65.9734457253856,66.0682195696543,
66.1630096695599,66.2578400499857,66.3527995240518,66.447831815984,66.5430314924363,
66.5873545600063,66.6815930937744,66.77570379357,66.8697152089495,66.9636593569636,
67.0575692928457,67.1514706663053,67.2453891126893,67.3394087893166,67.4334840046574,
67.527711247922,67.58241575451,67.6766408530215,67.7707454920501,67.8647555289504,
67.9586978558374,68.0526001292267,68.1465074888003,68.1989521886483),
 .UNSPECIFIED.);
#354=B_SPLINE_CURVE_WITH_KNOTS('',3,(#26660,#26661,#26662,#26663,#26664,
#26665,#26666,#26667,#26668,#26669,#26670,#26671,#26672,#26673,#26674,#26675,
#26676,#26677,#26678,#26679,#26680,#26681,#26682,#26683,#26684,#26685,#26686,
#26687,#26688,#26689,#26690,#26691,#26692,#26693,#26694,#26695,#26696,#26697,
#26698,#26699,#26700,#26701,#26702,#26703,#26704,#26705,#26706,#26707,#26708,
#26709,#26710,#26711,#26712,#26713,#26714,#26715,#26716,#26717,#26718,#26719,
#26720,#26721,#26722,#26723,#26724,#26725,#26726,#26727,#26728,#26729,#26730,
#26731,#26732,#26733,#26734,#26735),.UNSPECIFIED.,.F.,.F.,(4,3,3,3,3,3,
3,3,3,3,3,3,3,3,3,3,3,3,3,3,3,3,3,3,3,4),(65.9734457253856,66.1208876232955,
66.1415822411596,66.2358207749277,66.3299314747231,66.4239428901025,66.5178870381166,
66.6117969739988,66.7056983474584,66.7996167938421,66.8936364704694,66.9877116858102,
67.0819389290748,67.1366434356632,67.2308819694313,67.3249926692268,67.4190040846061,
67.5129482326202,67.6068581685024,67.700759541962,67.7946779883457,67.8886976649731,
67.982772880314,68.0770001235786,68.1317046301668,68.1996305298463),
 .UNSPECIFIED.);
#355=B_SPLINE_CURVE_WITH_KNOTS('',3,(#26736,#26737,#26738,#26739,#26740,
#26741,#26742,#26743,#26744,#26745,#26746,#26747,#26748,#26749,#26750,#26751,
#26752,#26753,#26754,#26755,#26756,#26757,#26758,#26759,#26760,#26761,#26762,
#26763,#26764,#26765,#26766,#26767,#26768,#26769,#26770,#26771,#26772,#26773,
#26774,#26775,#26776,#26777,#26778,#26779,#26780,#26781,#26782,#26783,#26784,
#26785,#26786,#26787,#26788,#26789,#26790,#26791,#26792,#26793,#26794,#26795,
#26796,#26797,#26798,#26799,#26800,#26801,#26802,#26803,#26804,#26805,#26806,
#26807,#26808,#26809,#26810,#26811,#26812,#26813,#26814,#26815,#26816,#26817,
#26818,#26819,#26820,#26821,#26822,#26823,#26824,#26825,#26826,#26827,#26828,
#26829,#26830,#26831,#26832,#26833,#26834,#26835,#26836,#26837,#26838,#26839,
#26840,#26841,#26842,#26843,#26844,#26845,#26846,#26847,#26848,#26849,#26850,
#26851,#26852,#26853,#26854,#26855,#26856,#26857,#26858,#26859,#26860,#26861,
#26862,#26863,#26864,#26865,#26866,#26867,#26868,#26869,#26870,#26871),
 .UNSPECIFIED.,.F.,.F.,(4,3,3,3,3,3,3,3,3,3,3,3,3,3,3,3,3,3,3,3,3,3,3,3,
3,3,3,3,3,3,3,3,3,3,3,3,3,3,3,3,3,3,3,3,3,4),(61.915536908638,62.009610141779,
62.1038362217474,62.1613374631452,62.2555759969133,62.3496866967087,62.4436981120881,
62.5376422601022,62.6315521959843,62.7254535694439,62.8193720158276,62.913391692455,
63.0074669077959,63.1016941510604,63.1563986576488,63.2506371914169,63.3447478912123,
63.4387593065916,63.5327034546057,63.6266133904879,63.7205147639474,63.8144332103312,
63.9084528869586,64.0025281022995,64.096755345564,64.1514598521524,64.2456983859205,
64.339809085716,64.4338205010953,64.5277646491094,64.6216745849916,64.7155759584511,
64.8094944048348,64.9035140814622,64.997589296803,65.0918165400676,65.146521046656,
65.2393639284447,65.3320574568457,65.4246665115197,65.5172182347163,65.6097397018221,
65.7023016612755,65.794880437501,65.8875747884578,65.9734457250788),
 .UNSPECIFIED.);
#356=B_SPLINE_CURVE_WITH_KNOTS('',3,(#26877,#26878,#26879,#26880,#26881,
#26882,#26883,#26884,#26885,#26886,#26887,#26888,#26889,#26890,#26891,#26892,
#26893,#26894,#26895,#26896,#26897,#26898,#26899,#26900,#26901,#26902,#26903,
#26904,#26905,#26906,#26907,#26908,#26909,#26910,#26911,#26912,#26913,#26914,
#26915,#26916,#26917,#26918,#26919,#26920,#26921,#26922,#26923,#26924,#26925,
#26926,#26927,#26928,#26929,#26930,#26931,#26932,#26933,#26934,#26935,#26936,
#26937,#26938,#26939,#26940,#26941,#26942,#26943,#26944,#26945,#26946,#26947,
#26948,#26949,#26950,#26951,#26952,#26953,#26954,#26955,#26956,#26957,#26958,
#26959,#26960,#26961,#26962,#26963,#26964,#26965,#26966,#26967,#26968,#26969,
#26970,#26971,#26972,#26973,#26974,#26975,#26976,#26977,#26978,#26979,#26980,
#26981,#26982,#26983,#26984,#26985,#26986,#26987,#26988,#26989,#26990,#26991,
#26992,#26993,#26994,#26995,#26996,#26997,#26998,#26999,#27000,#27001,#27002,
#27003,#27004,#27005,#27006,#27007,#27008,#27009,#27010,#27011,#27012,#27013,
#27014,#27015),.UNSPECIFIED.,.F.,.F.,(4,3,3,3,3,3,3,3,3,3,3,3,3,3,3,3,3,
3,3,3,3,3,3,3,3,3,3,3,3,3,3,3,3,3,3,3,3,3,3,3,3,3,3,3,3,3,4),(55.6328726554313,
55.6416814204666,55.7359199542347,55.8300306540301,55.9240420694095,56.0179862174236,
56.1118961533058,56.2057975267653,56.2997159731491,56.3937356497765,56.4878108651173,
56.5820381083819,56.6367426149702,56.7309811487383,56.8250918485337,56.9191032639131,
57.0130474119272,57.1069573478094,57.200858721269,57.2947771676527,57.3887968442801,
57.482872059621,57.5770993028855,57.6318038094738,57.7260423432419,57.8201530430373,
57.9141644584167,58.0081086064308,58.1020185423129,58.1959199157725,58.2898383621563,
58.3838580387837,58.4779332541246,58.5721604973891,58.6268650039775,58.7211035377456,
58.8152142375411,58.9092256529204,59.0031698009346,59.0970797368167,59.1909811102763,
59.28489955666,59.3789192332874,59.4729944486282,59.5672216918928,59.6219261984811,
59.690260418206),.UNSPECIFIED.);
#357=B_SPLINE_CURVE_WITH_KNOTS('',3,(#27016,#27017,#27018,#27019,#27020,
#27021,#27022,#27023,#27024,#27025,#27026,#27027,#27028,#27029,#27030,#27031,
#27032,#27033,#27034,#27035,#27036,#27037,#27038,#27039,#27040,#27041,#27042,
#27043,#27044,#27045,#27046,#27047,#27048,#27049,#27050,#27051,#27052,#27053,
#27054,#27055,#27056,#27057,#27058,#27059,#27060,#27061,#27062,#27063,#27064,
#27065,#27066,#27067,#27068,#27069,#27070,#27071,#27072,#27073,#27074,#27075,
#27076,#27077,#27078,#27079,#27080,#27081,#27082,#27083,#27084,#27085,#27086,
#27087,#27088,#27089,#27090,#27091),.UNSPECIFIED.,.F.,.F.,(4,3,3,3,3,3,
3,3,3,3,3,3,3,3,3,3,3,3,3,3,3,3,3,3,3,4),(59.6902604184034,59.7835566480732,
59.8767319494283,59.9698120649093,60.0628405197121,60.1558439723099,60.2488490519494,
60.3419437097565,60.4350818947519,60.5283799236479,60.6169873929847,60.7112259267528,
60.8053366265483,60.8993480419277,60.9932921899417,61.0872021258239,61.1811034992834,
61.275021945667,61.3690416222944,61.4631168376352,61.5573440808998,61.6120485874883,
61.7062744396242,61.8003879713356,61.8943961635387,61.9166125687905),
 .UNSPECIFIED.);
#358=B_SPLINE_CURVE_WITH_KNOTS('',3,(#27093,#27094,#27095,#27096,#27097,
#27098,#27099,#27100,#27101,#27102,#27103,#27104,#27105,#27106,#27107,#27108,
#27109,#27110,#27111,#27112,#27113,#27114,#27115,#27116,#27117,#27118,#27119,
#27120,#27121,#27122,#27123,#27124,#27125,#27126,#27127,#27128,#27129,#27130,
#27131,#27132,#27133,#27134,#27135,#27136,#27137,#27138,#27139,#27140,#27141,
#27142,#27143,#27144,#27145,#27146,#27147,#27148,#27149,#27150,#27151,#27152,
#27153,#27154,#27155,#27156,#27157,#27158,#27159,#27160,#27161,#27162,#27163,
#27164,#27165),.UNSPECIFIED.,.F.,.F.,(4,3,3,3,3,3,3,3,3,3,3,3,3,3,3,3,3,
3,3,3,3,3,3,3,4),(59.6902604183787,59.7892918179411,59.8886169604199,59.988091199275,
60.0878449487747,60.1712150741379,60.265453607906,60.3595643077015,60.4535757230808,
60.547519871095,60.6414298069772,60.7353311804367,60.8292496268203,60.9232693034477,
61.0173445187886,61.1115717620532,61.1662762686416,61.260489728568,61.3545858819447,
61.4485905716283,61.5425295541541,61.6364499411022,61.7303545142604,61.8243186029466,
61.915536908638),.UNSPECIFIED.);
#359=B_SPLINE_CURVE_WITH_KNOTS('',3,(#27166,#27167,#27168,#27169,#27170,
#27171,#27172,#27173,#27174,#27175,#27176,#27177,#27178,#27179,#27180,#27181,
#27182,#27183,#27184,#27185,#27186,#27187,#27188,#27189,#27190,#27191,#27192,
#27193,#27194,#27195,#27196,#27197,#27198,#27199,#27200,#27201,#27202,#27203,
#27204,#27205,#27206,#27207,#27208,#27209,#27210,#27211,#27212,#27213,#27214,
#27215,#27216,#27217,#27218,#27219,#27220,#27221,#27222,#27223,#27224,#27225,
#27226,#27227,#27228,#27229,#27230,#27231,#27232,#27233,#27234,#27235,#27236,
#27237,#27238,#27239,#27240,#27241,#27242,#27243,#27244,#27245,#27246,#27247,
#27248,#27249,#27250,#27251,#27252,#27253,#27254,#27255,#27256,#27257,#27258,
#27259,#27260,#27261,#27262,#27263,#27264,#27265,#27266,#27267,#27268,#27269,
#27270,#27271,#27272,#27273,#27274,#27275,#27276,#27277,#27278,#27279,#27280,
#27281,#27282,#27283,#27284,#27285,#27286,#27287,#27288,#27289,#27290,#27291,
#27292,#27293,#27294,#27295,#27296,#27297,#27298,#27299,#27300,#27301),
 .UNSPECIFIED.,.F.,.F.,(4,3,3,3,3,3,3,3,3,3,3,3,3,3,3,3,3,3,3,3,3,3,3,3,
3,3,3,3,3,3,3,3,3,3,3,3,3,3,3,3,3,3,3,3,3,4),(55.6331072412748,55.7270087028561,
55.8209182242538,55.9149238595219,56.0089769332002,56.1031920221626,56.1909702961235,
56.2852088298915,56.3793195296868,56.4733309450663,56.5672750930804,56.6611850289626,
56.7550864024222,56.849004848806,56.9430245254334,57.0370997407743,57.1313269840389,
57.1860314906271,57.2802700243952,57.3743807241906,57.46839213957,57.5623362875841,
57.6562462234663,57.7501475969257,57.8440660433094,57.9380857199368,58.0321609352776,
58.1263881785422,58.1810926851307,58.2753312188987,58.3694419186943,58.4634533340735,
58.5573974820876,58.6513074179696,58.7452087914292,58.8391272378128,58.9331469144401,
59.0272221297808,59.1214493730453,59.1761538796343,59.2745027508079,59.3726743921948,
59.4706312790709,59.5684582642373,59.6661366206867,59.690260418206),
 .UNSPECIFIED.);
#360=B_SPLINE_CURVE_WITH_KNOTS('',3,(#27307,#27308,#27309,#27310,#27311,
#27312,#27313,#27314,#27315,#27316,#27317,#27318,#27319,#27320,#27321,#27322,
#27323,#27324,#27325,#27326,#27327,#27328,#27329,#27330,#27331,#27332,#27333,
#27334,#27335,#27336,#27337,#27338,#27339,#27340,#27341,#27342,#27343,#27344,
#27345,#27346,#27347,#27348,#27349,#27350,#27351,#27352,#27353,#27354,#27355,
#27356,#27357,#27358,#27359,#27360,#27361,#27362,#27363,#27364,#27365,#27366,
#27367,#27368,#27369,#27370,#27371,#27372,#27373,#27374,#27375,#27376,#27377,
#27378,#27379,#27380,#27381,#27382,#27383,#27384,#27385,#27386,#27387,#27388,
#27389,#27390,#27391,#27392,#27393,#27394,#27395,#27396,#27397,#27398,#27399,
#27400,#27401,#27402,#27403,#27404,#27405,#27406,#27407,#27408,#27409,#27410,
#27411,#27412,#27413,#27414,#27415,#27416,#27417,#27418,#27419,#27420,#27421,
#27422,#27423,#27424,#27425,#27426,#27427,#27428,#27429,#27430,#27431,#27432,
#27433,#27434,#27435,#27436,#27437,#27438,#27439,#27440,#27441,#27442),
 .UNSPECIFIED.,.F.,.F.,(4,3,3,3,3,3,3,3,3,3,3,3,3,3,3,3,3,3,3,3,3,3,3,3,
3,3,3,3,3,3,3,3,3,3,3,3,3,3,3,3,3,3,3,3,3,4),(49.3492693022874,49.4432962859874,
49.5373824839442,49.6316163965574,49.6713142534449,49.765552787213,49.8596634870087,
49.9536749023884,50.0476190504025,50.1415289862847,50.2354303597442,50.3293488061279,
50.4233684827553,50.5174436980961,50.6116709413607,50.6663754479486,50.7606139817167,
50.8547246815122,50.9487360968916,51.0426802449057,51.1365901807879,51.2304915542473,
51.3244100006314,51.4184296772588,51.5125048925997,51.6067321358643,51.6614366424522,
51.7556751762202,51.8497858760156,51.9437972913951,52.0377414394091,52.1316513752914,
52.2255527487512,52.3194711951354,52.4134908717627,52.5075660871034,52.601793330368,
52.6564978369558,52.7503199962146,52.8433012289229,52.9361944978272,53.0290267156312,
53.12353881448,53.2163550637721,53.3117150873993,53.4070751110265),
 .UNSPECIFIED.);
#361=B_SPLINE_CURVE_WITH_KNOTS('',3,(#27443,#27444,#27445,#27446,#27447,
#27448,#27449,#27450,#27451,#27452,#27453,#27454,#27455,#27456,#27457,#27458,
#27459,#27460,#27461,#27462,#27463,#27464,#27465,#27466,#27467,#27468,#27469,
#27470,#27471,#27472,#27473,#27474,#27475,#27476,#27477,#27478,#27479,#27480,
#27481,#27482,#27483,#27484,#27485,#27486,#27487,#27488,#27489,#27490,#27491,
#27492,#27493,#27494,#27495,#27496,#27497,#27498,#27499,#27500,#27501,#27502,
#27503,#27504,#27505,#27506,#27507,#27508,#27509,#27510,#27511,#27512,#27513,
#27514,#27515),.UNSPECIFIED.,.F.,.F.,(4,3,3,3,3,3,3,3,3,3,3,3,3,3,3,3,3,
3,3,3,3,3,3,3,4),(53.4070751112921,53.5297330757898,53.6515590314594,53.7457975652275,
53.839908265023,53.9339196804023,54.0278638284164,54.1217737642986,54.2156751377582,
54.309593584142,54.4036132607693,54.4976884761102,54.5919157193747,54.646620225963,
54.7408593113648,54.8349704164143,54.9289820913343,55.0229258433417,55.1168351761681,
55.2107357394637,55.3046531682905,55.3986692222742,55.4927407296692,55.5869583613849,
55.6328726554313),.UNSPECIFIED.);
#362=B_SPLINE_CURVE_WITH_KNOTS('',3,(#27517,#27518,#27519,#27520,#27521,
#27522,#27523,#27524,#27525,#27526,#27527,#27528,#27529,#27530,#27531,#27532,
#27533,#27534,#27535,#27536,#27537,#27538,#27539,#27540,#27541,#27542,#27543,
#27544,#27545,#27546,#27547,#27548,#27549,#27550,#27551,#27552,#27553,#27554,
#27555,#27556,#27557,#27558,#27559,#27560,#27561,#27562,#27563,#27564,#27565,
#27566,#27567,#27568,#27569,#27570,#27571,#27572,#27573,#27574,#27575,#27576,
#27577,#27578,#27579,#27580,#27581,#27582,#27583,#27584,#27585,#27586,#27587,
#27588,#27589,#27590,#27591,#27592),.UNSPECIFIED.,.F.,.F.,(4,3,3,3,3,3,
3,3,3,3,3,3,3,3,3,3,3,3,3,3,3,3,3,3,3,4),(53.407075111341,53.4997993899299,
53.59243844576,53.6850327223763,53.7776092331113,53.8701949680753,53.9628735164128,
54.0556031024416,54.1484802213107,54.2008479071163,54.2950864408844,54.3891971406799,
54.4832085560591,54.5771527040732,54.6710626399553,54.7649640134149,54.8588824597986,
54.9529021364259,55.0469773517668,55.1412045950314,55.1959091016199,55.2901555293964,
55.3842501749379,55.4782569522969,55.5721977094091,55.6331072412748),
 .UNSPECIFIED.);
#363=B_SPLINE_CURVE_WITH_KNOTS('',3,(#27593,#27594,#27595,#27596,#27597,
#27598,#27599,#27600,#27601,#27602,#27603,#27604,#27605,#27606,#27607,#27608,
#27609,#27610,#27611,#27612,#27613,#27614,#27615,#27616,#27617,#27618,#27619,
#27620,#27621,#27622,#27623,#27624,#27625,#27626,#27627,#27628,#27629,#27630,
#27631,#27632,#27633,#27634,#27635,#27636,#27637,#27638,#27639,#27640,#27641,
#27642,#27643,#27644,#27645,#27646,#27647,#27648,#27649,#27650,#27651,#27652,
#27653,#27654,#27655,#27656,#27657,#27658,#27659,#27660,#27661,#27662,#27663,
#27664,#27665,#27666,#27667,#27668,#27669,#27670,#27671,#27672,#27673,#27674,
#27675,#27676,#27677,#27678,#27679,#27680,#27681,#27682,#27683,#27684,#27685,
#27686,#27687,#27688,#27689,#27690,#27691,#27692,#27693,#27694,#27695,#27696,
#27697,#27698,#27699,#27700,#27701,#27702,#27703,#27704,#27705,#27706,#27707,
#27708,#27709,#27710,#27711,#27712,#27713,#27714,#27715,#27716,#27717,#27718,
#27719,#27720,#27721,#27722,#27723,#27724,#27725,#27726,#27727,#27728),
 .UNSPECIFIED.,.F.,.F.,(4,3,3,3,3,3,3,3,3,3,3,3,3,3,3,3,3,3,3,3,3,3,3,3,
3,3,3,3,3,3,3,3,3,3,3,3,3,3,3,3,3,3,3,3,3,4),(49.3502405140517,49.4443159743505,
49.5413518686944,49.6352808952855,49.7291848439067,49.8230893567473,49.9170200691168,
50.0110568618701,50.1051573991158,50.1994005222569,50.2206031291018,50.3148416628699,
50.4089523626653,50.5029637780446,50.5969079260587,50.6908178619408,50.7847192354003,
50.878637681784,50.9726573584114,51.0667325737522,51.1609598170167,51.2156643236054,
51.3099028573735,51.404013557169,51.4980249725484,51.5919691205625,51.6858790564447,
51.7797804299042,51.873698876288,51.9677185529154,52.0617937682562,52.1560210115208,
52.2107255181091,52.3049640518772,52.3990747516726,52.493086167052,52.5870303150661,
52.6809402509483,52.7748416244078,52.8687600707916,52.962779747419,53.0568549627599,
53.1510822060245,53.2057867126127,53.3395856335398,53.4070751110265),
 .UNSPECIFIED.);
#364=B_SPLINE_CURVE_WITH_KNOTS('',3,(#27734,#27735,#27736,#27737,#27738,
#27739,#27740,#27741,#27742,#27743,#27744,#27745,#27746,#27747,#27748,#27749,
#27750,#27751,#27752,#27753,#27754,#27755,#27756,#27757,#27758,#27759,#27760,
#27761,#27762,#27763,#27764,#27765,#27766,#27767,#27768,#27769,#27770,#27771,
#27772,#27773,#27774,#27775,#27776,#27777,#27778,#27779,#27780,#27781,#27782,
#27783,#27784,#27785,#27786,#27787,#27788,#27789,#27790,#27791,#27792,#27793,
#27794,#27795,#27796,#27797,#27798,#27799,#27800,#27801,#27802,#27803,#27804,
#27805,#27806,#27807,#27808,#27809,#27810,#27811,#27812,#27813,#27814,#27815,
#27816,#27817,#27818,#27819,#27820,#27821,#27822,#27823,#27824,#27825,#27826,
#27827,#27828,#27829,#27830,#27831,#27832,#27833,#27834,#27835,#27836,#27837,
#27838,#27839,#27840,#27841,#27842,#27843,#27844,#27845,#27846,#27847,#27848,
#27849,#27850,#27851,#27852,#27853,#27854,#27855,#27856,#27857,#27858,#27859,
#27860,#27861,#27862,#27863,#27864,#27865,#27866,#27867,#27868,#27869),
 .UNSPECIFIED.,.F.,.F.,(4,3,3,3,3,3,3,3,3,3,3,3,3,3,3,3,3,3,3,3,3,3,3,3,
3,3,3,3,3,3,3,3,3,3,3,3,3,3,3,3,3,3,3,3,3,4),(43.0669410879269,43.1608548335968,
43.254755853933,43.3486697851862,43.442682624419,43.5367472614373,43.6309684564177,
43.7009470864233,43.7951856201919,43.889296319988,43.9833077353676,44.0772518833823,
44.1711618192651,44.2650631927253,44.3589816391098,44.4530013157377,44.5470765310791,
44.6413037743443,44.6960082809269,44.7902468146948,44.8843575144902,44.9783689298692,
45.0723130778831,45.1662230137652,45.2601243872245,45.3540428336081,45.4480625102353,
45.5421377255761,45.6363649688403,45.6910694754305,45.7853080091985,45.8794187089939,
45.9734301243732,46.0673742723873,46.1612842082693,46.2551855817288,46.3491040281125,
46.4431237047399,46.5371989200807,46.6314261633452,46.6861306699341,46.7882622974101,
46.890027682399,46.9915575618476,47.0927492023486,47.1238898035594),
 .UNSPECIFIED.);
#365=B_SPLINE_CURVE_WITH_KNOTS('',3,(#27870,#27871,#27872,#27873,#27874,
#27875,#27876,#27877,#27878,#27879,#27880,#27881,#27882,#27883,#27884,#27885,
#27886,#27887,#27888,#27889,#27890,#27891,#27892,#27893,#27894,#27895,#27896,
#27897,#27898,#27899,#27900,#27901,#27902,#27903,#27904,#27905,#27906,#27907,
#27908,#27909,#27910,#27911,#27912,#27913,#27914,#27915,#27916,#27917,#27918,
#27919,#27920,#27921,#27922,#27923,#27924,#27925,#27926,#27927,#27928,#27929,
#27930,#27931,#27932,#27933,#27934,#27935,#27936,#27937,#27938,#27939,#27940,
#27941,#27942,#27943,#27944,#27945),.UNSPECIFIED.,.F.,.F.,(4,3,3,3,3,3,
3,3,3,3,3,3,3,3,3,3,3,3,3,3,3,3,3,3,3,4),(47.1238898038468,47.2201237011967,
47.3164231550396,47.4128894374831,47.5094431103066,47.606199734555,47.6811918644377,
47.7754303982057,47.8695410980011,47.9635525133803,48.0574966613944,48.1514065972766,
48.245307970736,48.3392264171196,48.433246093747,48.5273213090879,48.6215485523525,
48.6762530589413,48.7704727733985,48.864573370564,48.95858070139,49.0562528516144,
49.1501600113785,49.2440515574863,49.3379704500663,49.3492693022874),
 .UNSPECIFIED.);
#366=B_SPLINE_CURVE_WITH_KNOTS('',3,(#27947,#27948,#27949,#27950,#27951,
#27952,#27953,#27954,#27955,#27956,#27957,#27958,#27959,#27960,#27961,#27962,
#27963,#27964,#27965,#27966,#27967,#27968,#27969,#27970,#27971,#27972,#27973,
#27974,#27975,#27976,#27977,#27978,#27979,#27980,#27981,#27982,#27983,#27984,
#27985,#27986,#27987,#27988,#27989,#27990,#27991,#27992,#27993,#27994,#27995,
#27996,#27997,#27998,#27999,#28000,#28001,#28002,#28003,#28004,#28005,#28006,
#28007,#28008,#28009,#28010,#28011,#28012,#28013,#28014,#28015,#28016,#28017,
#28018,#28019,#28020,#28021,#28022),.UNSPECIFIED.,.F.,.F.,(4,3,3,3,3,3,
3,3,3,3,3,3,3,3,3,3,3,3,3,3,3,3,3,3,3,4),(47.1238898038468,47.235419545591,
47.3296580793589,47.4237687791541,47.5177801945334,47.6117243425473,47.7056342784293,
47.7995356518887,47.8934540982721,47.9874737748993,48.08154899024,48.1757762335043,
48.2304807400946,48.3247192738627,48.4188299736581,48.5128413890375,48.6067855370516,
48.7006954729337,48.7945968463932,48.8885152927769,48.9825349694042,49.076610184745,
49.1708374280095,49.2255419345982,49.3197803108064,49.3502405140517),
 .UNSPECIFIED.);
#367=B_SPLINE_CURVE_WITH_KNOTS('',3,(#28023,#28024,#28025,#28026,#28027,
#28028,#28029,#28030,#28031,#28032,#28033,#28034,#28035,#28036,#28037,#28038,
#28039,#28040,#28041,#28042,#28043,#28044,#28045,#28046,#28047,#28048,#28049,
#28050,#28051,#28052,#28053,#28054,#28055,#28056,#28057,#28058,#28059,#28060,
#28061,#28062,#28063,#28064,#28065,#28066,#28067,#28068,#28069,#28070,#28071,
#28072,#28073,#28074,#28075,#28076,#28077,#28078,#28079,#28080,#28081,#28082,
#28083,#28084,#28085,#28086,#28087,#28088,#28089,#28090,#28091,#28092,#28093,
#28094,#28095,#28096,#28097,#28098,#28099,#28100,#28101,#28102,#28103,#28104,
#28105,#28106,#28107,#28108,#28109,#28110,#28111,#28112,#28113,#28114,#28115,
#28116,#28117,#28118,#28119,#28120,#28121,#28122,#28123,#28124,#28125,#28126,
#28127,#28128,#28129,#28130,#28131,#28132,#28133,#28134,#28135,#28136,#28137,
#28138,#28139,#28140,#28141,#28142,#28143,#28144,#28145,#28146,#28147,#28148,
#28149,#28150,#28151,#28152,#28153,#28154,#28155,#28156,#28157,#28158),
 .UNSPECIFIED.,.F.,.F.,(4,3,3,3,3,3,3,3,3,3,3,3,3,3,3,3,3,3,3,3,3,3,3,3,
3,3,3,3,3,3,3,3,3,3,3,3,3,3,3,3,3,3,3,3,3,4),(43.0659729437217,43.1605738556491,
43.2551747675765,43.3494133013489,43.4435240011486,43.5375354165324,43.631479564551,
43.7253895004376,43.8192908739017,43.91320932029,44.007228996922,44.1013042122674,
44.1955314555366,44.2502359620802,44.3444744958471,44.4385851956413,44.5325966110194,
44.6265407590322,44.7204506949132,44.8143520683715,44.9082705147539,45.0022901913801,
45.0963654067197,45.1905926499831,45.2452971565838,45.3395356903515,45.4336463901465,
45.5276578055255,45.6216019535392,45.7155118894209,45.8094132628799,45.9033317092632,
45.9973513858901,46.0914266012305,46.1856538444945,46.2403583510874,46.333353832453,
46.4262225404432,46.51898661054,46.6116939361495,46.7043714684739,46.7970461230525,
46.8897940511749,46.9825825279157,47.0754997299982,47.1238898036239),
 .UNSPECIFIED.);
#368=B_SPLINE_CURVE_WITH_KNOTS('',3,(#28164,#28165,#28166,#28167,#28168,
#28169,#28170,#28171,#28172,#28173,#28174,#28175,#28176,#28177,#28178,#28179,
#28180,#28181,#28182,#28183,#28184,#28185,#28186,#28187,#28188,#28189,#28190,
#28191,#28192,#28193,#28194,#28195,#28196,#28197,#28198,#28199,#28200,#28201,
#28202,#28203,#28204,#28205,#28206,#28207,#28208,#28209,#28210,#28211,#28212,
#28213,#28214,#28215,#28216,#28217,#28218,#28219,#28220,#28221,#28222,#28223,
#28224,#28225,#28226,#28227,#28228,#28229,#28230,#28231,#28232,#28233,#28234,
#28235,#28236,#28237,#28238,#28239,#28240,#28241,#28242,#28243,#28244,#28245,
#28246,#28247,#28248,#28249,#28250,#28251,#28252,#28253,#28254,#28255,#28256,
#28257,#28258,#28259,#28260,#28261,#28262,#28263,#28264,#28265,#28266,#28267,
#28268,#28269,#28270,#28271,#28272,#28273,#28274,#28275,#28276,#28277,#28278,
#28279,#28280,#28281,#28282,#28283,#28284,#28285,#28286,#28287,#28288,#28289,
#28290,#28291,#28292,#28293,#28294,#28295,#28296),.UNSPECIFIED.,.F.,.F.,
(4,3,3,3,3,3,3,3,3,3,3,3,3,3,3,3,3,3,3,3,3,3,3,3,3,3,3,3,3,3,3,3,3,3,3,
3,3,3,3,3,3,3,3,3,4),(36.7836225529413,36.8777922829933,36.9718487623956,
37.0666901570213,37.1606133284242,37.2545156160629,37.3484226595646,37.4439619745238,
37.5380085641333,37.6342942417675,37.7305799194016,37.8248184532023,37.9189291530308,
38.0129405684437,38.1068847164918,38.2007946524082,38.2946960259022,38.3886144723206,
38.4826341489828,38.5767093643585,38.6709366076577,38.7256411139052,38.8198796476661,
38.9139903474544,39.0080017628264,39.1019459108333,39.1958558467081,39.2897572201605,
39.3836756665371,39.4776953431573,39.571770558491,39.6659978017485,39.7207023084088,
39.8149408421724,39.9090515419633,40.0030629573379,40.0970071053473,40.1909170412247,
40.2848184146794,40.3787368610583,40.4727565376808,40.5668317530167,40.6610589962762,
40.7157635029124,40.8407044966672),.UNSPECIFIED.);
#369=B_SPLINE_CURVE_WITH_KNOTS('',3,(#28297,#28298,#28299,#28300,#28301,
#28302,#28303,#28304,#28305,#28306,#28307,#28308,#28309,#28310,#28311,#28312,
#28313,#28314,#28315,#28316,#28317,#28318,#28319,#28320,#28321,#28322,#28323,
#28324,#28325,#28326,#28327,#28328,#28329,#28330,#28331,#28332,#28333,#28334,
#28335,#28336,#28337,#28338,#28339,#28340,#28341,#28342,#28343,#28344,#28345,
#28346,#28347,#28348,#28349,#28350,#28351,#28352,#28353,#28354,#28355,#28356,
#28357,#28358,#28359,#28360,#28361,#28362,#28363,#28364,#28365,#28366,#28367,
#28368,#28369,#28370,#28371,#28372),.UNSPECIFIED.,.F.,.F.,(4,3,3,3,3,3,
3,3,3,3,3,3,3,3,3,3,3,3,3,3,3,3,3,3,3,4),(40.8407044968828,40.9335549962785,
41.0307137089207,41.1233759605245,41.2159998721551,41.3086124205635,41.4012405658138,
41.4939653595684,41.5867468664922,41.6796701952324,41.7108246974161,41.8050632311829,
41.8991739309771,41.993185346355,42.0871294943679,42.1810394302488,42.2749408037072,
42.3688592500896,42.4628789267157,42.5569541420554,42.6511813853187,42.7058858919197,
42.8001014455114,42.894205230012,42.9882080806231,43.0669410879269),
 .UNSPECIFIED.);
#370=B_SPLINE_CURVE_WITH_KNOTS('',3,(#28374,#28375,#28376,#28377,#28378,
#28379,#28380,#28381,#28382,#28383,#28384,#28385,#28386,#28387,#28388,#28389,
#28390,#28391,#28392,#28393,#28394,#28395,#28396,#28397,#28398,#28399,#28400,
#28401,#28402,#28403,#28404,#28405,#28406,#28407,#28408,#28409,#28410,#28411,
#28412,#28413,#28414,#28415,#28416,#28417,#28418,#28419,#28420,#28421,#28422,
#28423,#28424,#28425,#28426,#28427,#28428,#28429,#28430,#28431,#28432,#28433,
#28434,#28435,#28436,#28437,#28438,#28439,#28440,#28441,#28442,#28443,#28444,
#28445,#28446),.UNSPECIFIED.,.F.,.F.,(4,3,3,3,3,3,3,3,3,3,3,3,3,3,3,3,3,
3,3,3,3,3,3,3,4),(40.8407044968363,40.9467914672695,41.0491746662872,41.1571135224282,
41.2650523785693,41.3592909123302,41.4534016121184,41.5474130274904,41.6413571754972,
41.7352671113721,41.8291684848244,41.9230869312007,42.0171066078209,42.1111818231546,
42.205409066412,42.2601135730729,42.3543648088597,42.4484583704197,42.5424618174093,
42.636400902428,42.7303013160319,42.8242184381103,42.9181432733357,43.0121464759615,
43.0659729437217),.UNSPECIFIED.);
#371=B_SPLINE_CURVE_WITH_KNOTS('',3,(#28447,#28448,#28449,#28450,#28451,
#28452,#28453,#28454,#28455,#28456,#28457,#28458,#28459,#28460,#28461,#28462,
#28463,#28464,#28465,#28466,#28467,#28468,#28469,#28470,#28471,#28472,#28473,
#28474,#28475,#28476,#28477,#28478,#28479,#28480,#28481,#28482,#28483,#28484,
#28485,#28486,#28487,#28488,#28489,#28490,#28491,#28492,#28493,#28494,#28495,
#28496,#28497,#28498,#28499,#28500,#28501,#28502,#28503,#28504,#28505,#28506,
#28507,#28508,#28509,#28510,#28511,#28512,#28513,#28514,#28515,#28516,#28517,
#28518,#28519,#28520,#28521,#28522,#28523,#28524,#28525,#28526,#28527,#28528,
#28529,#28530,#28531,#28532,#28533,#28534,#28535,#28536,#28537,#28538,#28539,
#28540,#28541,#28542,#28543,#28544,#28545,#28546,#28547,#28548,#28549,#28550,
#28551,#28552,#28553,#28554,#28555,#28556,#28557,#28558,#28559,#28560,#28561,
#28562,#28563,#28564,#28565,#28566,#28567,#28568,#28569,#28570,#28571,#28572,
#28573,#28574,#28575,#28576,#28577,#28578,#28579,#28580,#28581,#28582),
 .UNSPECIFIED.,.F.,.F.,(4,3,3,3,3,3,3,3,3,3,3,3,3,3,3,3,3,3,3,3,3,3,3,3,
3,3,3,3,3,3,3,3,3,3,3,3,3,3,3,3,3,3,3,3,3,4),(36.7833811949732,36.8772844267835,
36.9712111255313,37.0652424873676,37.1593351364484,37.2535731276351,37.2848076005549,
37.3790461345677,37.473156834611,37.5671682502409,37.6611123985091,37.7550223346473,
37.8489237083645,37.942842155007,38.0368618318937,38.1309370474943,38.2251642910171,
38.2798687950585,38.3741073287897,38.4682180285484,38.562229443891,38.6561735918686,
38.7500835277143,38.8439849011377,38.9379033474859,39.0319230240781,39.1259982393842,
39.2202254826146,39.2749299895621,39.3691685232879,39.46327922304,39.5572906383755,
39.6512347863447,39.7451447221812,39.8390460955947,39.9329645419325,40.0269842185129,
40.1210594338062,40.2152866770234,40.2699911840657,40.3663474040034,40.4625550534326,
40.5586031867734,40.6545575383556,40.7504306622901,40.8407044966672),
 .UNSPECIFIED.);
#372=B_SPLINE_CURVE_WITH_KNOTS('',3,(#28588,#28589,#28590,#28591,#28592,
#28593,#28594,#28595,#28596,#28597,#28598,#28599,#28600,#28601,#28602,#28603,
#28604,#28605,#28606,#28607,#28608,#28609,#28610,#28611,#28612,#28613,#28614,
#28615,#28616,#28617,#28618,#28619,#28620,#28621,#28622,#28623,#28624,#28625,
#28626,#28627,#28628,#28629,#28630,#28631,#28632,#28633,#28634,#28635,#28636,
#28637,#28638,#28639,#28640,#28641,#28642,#28643,#28644,#28645,#28646,#28647,
#28648,#28649,#28650,#28651,#28652,#28653,#28654,#28655,#28656,#28657,#28658,
#28659,#28660,#28661,#28662,#28663,#28664,#28665,#28666,#28667,#28668,#28669,
#28670,#28671,#28672,#28673,#28674,#28675,#28676,#28677,#28678,#28679,#28680,
#28681,#28682,#28683,#28684,#28685,#28686,#28687,#28688,#28689,#28690,#28691,
#28692,#28693,#28694,#28695,#28696,#28697,#28698,#28699,#28700,#28701,#28702,
#28703,#28704,#28705,#28706,#28707,#28708,#28709,#28710,#28711,#28712,#28713,
#28714,#28715,#28716,#28717,#28718,#28719,#28720,#28721,#28722,#28723),
 .UNSPECIFIED.,.F.,.F.,(4,3,3,3,3,3,3,3,3,3,3,3,3,3,3,3,3,3,3,3,3,3,3,3,
3,3,3,3,3,3,3,3,3,3,3,3,3,3,3,3,3,3,3,3,3,4),(30.4996279272502,30.5936877447165,
30.6879063249188,30.7651515578763,30.8593900883337,30.9535007847613,31.0475121967206,
31.141456341251,31.2353662736114,31.3292676435152,31.4231860863138,31.5172057593323,
31.6112809710456,31.7055082106889,31.7602127523799,31.8544512879246,31.9485619895187,
32.0425734067164,32.13651755657,32.2304274943042,32.3243288696259,32.4182473178801,
32.5122669963787,32.606342213594,32.7005694587196,32.7552739468835,32.84951248052,
32.9436231801865,33.0376345954395,33.1315787433317,33.2254886790948,33.3193900524384,
33.4133084987091,33.5073281752292,33.6014033904657,33.6956306336318,33.7503351413872,
33.843198509978,33.9359114578974,34.0285393283358,34.1211092506416,34.2136482865597,
34.3062224486771,34.3988130903768,34.4915064402966,34.5575191892671),
 .UNSPECIFIED.);
#373=B_SPLINE_CURVE_WITH_KNOTS('',3,(#28724,#28725,#28726,#28727,#28728,
#28729,#28730,#28731,#28732,#28733,#28734,#28735,#28736,#28737,#28738,#28739,
#28740,#28741,#28742,#28743,#28744,#28745,#28746,#28747,#28748,#28749,#28750,
#28751,#28752,#28753,#28754,#28755,#28756,#28757,#28758,#28759,#28760,#28761,
#28762,#28763,#28764,#28765,#28766,#28767,#28768,#28769,#28770,#28771,#28772,
#28773,#28774,#28775,#28776,#28777,#28778,#28779,#28780,#28781,#28782,#28783,
#28784,#28785,#28786,#28787,#28788,#28789,#28790,#28791,#28792,#28793,#28794,
#28795,#28796,#28797,#28798,#28799),.UNSPECIFIED.,.F.,.F.,(4,3,3,3,3,3,
3,3,3,3,3,3,3,3,3,3,3,3,3,3,3,3,3,3,3,4),(34.5575191894877,34.6960958089033,
34.7453963358908,34.8396348699029,34.9337455699456,35.0277569855753,35.1217011338427,
35.2156110699801,35.3095124436966,35.4034308903384,35.4974505672243,35.5915257828243,
35.6857530263464,35.7404575303944,35.8346960641258,35.9288067638846,36.0228181792274,
36.1167623272052,36.2106722630512,36.3045736364748,36.3984920828229,36.4925117594152,
36.5865869747213,36.6808142179519,36.735518724898,36.7836225529413),
 .UNSPECIFIED.);
#374=B_SPLINE_CURVE_WITH_KNOTS('',3,(#28801,#28802,#28803,#28804,#28805,
#28806,#28807,#28808,#28809,#28810,#28811,#28812,#28813,#28814,#28815,#28816,
#28817,#28818,#28819,#28820,#28821,#28822,#28823,#28824,#28825,#28826,#28827,
#28828,#28829,#28830,#28831,#28832,#28833,#28834,#28835,#28836,#28837,#28838,
#28839,#28840,#28841,#28842,#28843,#28844,#28845,#28846,#28847,#28848,#28849,
#28850,#28851,#28852,#28853,#28854,#28855,#28856,#28857,#28858,#28859,#28860,
#28861,#28862,#28863,#28864,#28865,#28866,#28867,#28868,#28869,#28870,#28871,
#28872,#28873,#28874,#28875,#28876),.UNSPECIFIED.,.F.,.F.,(4,3,3,3,3,3,
3,3,3,3,3,3,3,3,3,3,3,3,3,3,3,3,3,3,3,4),(34.5575191894877,34.6505073831219,
34.7434447345139,34.8363579713218,34.9292737926231,35.0222802791695,35.1153312545951,
35.2085421544079,35.2946852115477,35.3889237451837,35.4830344448493,35.5770458601016,
35.6709900079932,35.7648999437556,35.8588013170986,35.9527197633688,36.0467394398882,
36.1408146551243,36.2350418982897,36.2897464060513,36.3839854271749,36.4781010657501,
36.57210461853,36.666043929314,36.7599457471408,36.7833811949732),
 .UNSPECIFIED.);
#375=B_SPLINE_CURVE_WITH_KNOTS('',3,(#28877,#28878,#28879,#28880,#28881,
#28882,#28883,#28884,#28885,#28886,#28887,#28888,#28889,#28890,#28891,#28892,
#28893,#28894,#28895,#28896,#28897,#28898,#28899,#28900,#28901,#28902,#28903,
#28904,#28905,#28906,#28907,#28908,#28909,#28910,#28911,#28912,#28913,#28914,
#28915,#28916,#28917,#28918,#28919,#28920,#28921,#28922,#28923,#28924,#28925,
#28926,#28927,#28928,#28929,#28930,#28931,#28932,#28933,#28934,#28935,#28936,
#28937,#28938,#28939,#28940,#28941,#28942,#28943,#28944,#28945,#28946,#28947,
#28948,#28949,#28950,#28951,#28952,#28953,#28954,#28955,#28956,#28957,#28958,
#28959,#28960,#28961,#28962,#28963,#28964,#28965,#28966,#28967,#28968,#28969,
#28970,#28971,#28972,#28973,#28974,#28975,#28976,#28977,#28978,#28979,#28980,
#28981,#28982,#28983,#28984,#28985,#28986,#28987,#28988,#28989,#28990,#28991,
#28992,#28993,#28994,#28995,#28996,#28997,#28998,#28999,#29000,#29001,#29002,
#29003,#29004,#29005,#29006,#29007,#29008,#29009,#29010,#29011,#29012),
 .UNSPECIFIED.,.F.,.F.,(4,3,3,3,3,3,3,3,3,3,3,3,3,3,3,3,3,3,3,3,3,3,3,3,
3,3,3,3,3,3,3,3,3,3,3,3,3,3,3,3,3,3,3,3,3,4),(30.5007612509717,30.5947790154448,
30.6887266897135,30.7826382504506,30.8765393493006,30.9704556219893,31.0644720738379,
31.1585423574244,31.25276671836,31.3144404335332,31.4086789798773,31.5027896923931,
31.5968011206189,31.6907452816136,31.7846552305545,31.8785566171349,31.9724750766856,
32.06649476647,32.1605699949819,32.254797251309,32.3095016280368,32.4037401619858,
32.497850861999,32.5918622776326,32.6858064259543,32.7797163621772,32.8736177360103,
32.9675361827999,33.0615558598808,33.1556310757027,33.2498583194874,33.3045628225404,
33.398801352991,33.4929120494117,33.586923461364,33.6808676058873,33.7747775382403,
33.8686789081369,33.9625973509281,34.0566170239391,34.1506922356449,34.2449194752806,
34.299624017044,34.4208944554796,34.5397648284115,34.557519189206),
 .UNSPECIFIED.);
#376=B_SPLINE_CURVE_WITH_KNOTS('',3,(#29018,#29019,#29020,#29021,#29022,
#29023,#29024,#29025),.UNSPECIFIED.,.F.,.F.,(4,1,1,1,1,4),(24.2174104409543,
24.7947843908547,25.7898455853583,26.7849067798619,27.7799679743655,28.2743336440772),
 .UNSPECIFIED.);
#377=B_SPLINE_CURVE_WITH_KNOTS('',3,(#29026,#29027,#29028,#29029,#29030,
#29031,#29032,#29033,#29034,#29035,#29036,#29037,#29038,#29039,#29040,#29041,
#29042,#29043,#29044,#29045,#29046,#29047,#29048,#29049,#29050,#29051,#29052,
#29053,#29054,#29055,#29056,#29057,#29058,#29059,#29060,#29061,#29062,#29063,
#29064,#29065,#29066,#29067,#29068,#29069,#29070,#29071,#29072,#29073,#29074,
#29075,#29076,#29077,#29078,#29079,#29080,#29081,#29082,#29083,#29084,#29085,
#29086,#29087,#29088,#29089,#29090,#29091,#29092,#29093,#29094,#29095,#29096,
#29097,#29098),.UNSPECIFIED.,.F.,.F.,(4,3,3,3,3,3,3,3,3,3,3,3,3,3,3,3,3,
3,3,3,3,3,3,3,4),(28.2743338823081,28.3725366417317,28.473159773516,28.5717415465316,
28.6733853577003,28.7750291688691,28.8692677151853,28.963378427673,29.0573898558701,
29.151334016836,29.2452439657479,29.3391453522992,29.4330638118205,29.5270835015756,
29.6211587300581,29.7153859863561,29.7700903633727,29.8643053297425,29.9584025213165,
30.0524077829851,30.1463468727215,30.2402636747242,30.3341644786122,30.4281151158429,
30.4996279272502),.UNSPECIFIED.);
#378=B_SPLINE_CURVE_WITH_KNOTS('',3,(#29100,#29101,#29102,#29103,#29104,
#29105,#29106,#29107,#29108,#29109,#29110,#29111,#29112,#29113,#29114,#29115,
#29116,#29117,#29118,#29119,#29120,#29121,#29122,#29123,#29124,#29125,#29126,
#29127,#29128,#29129,#29130,#29131,#29132,#29133,#29134,#29135,#29136,#29137,
#29138,#29139,#29140,#29141,#29142,#29143,#29144,#29145,#29146,#29147,#29148,
#29149,#29150,#29151,#29152,#29153,#29154,#29155,#29156,#29157,#29158,#29159,
#29160,#29161,#29162,#29163,#29164,#29165,#29166,#29167,#29168,#29169,#29170,
#29171,#29172,#29173,#29174,#29175),.UNSPECIFIED.,.F.,.F.,(4,3,3,3,3,3,
3,3,3,3,3,3,3,3,3,3,3,3,3,3,3,3,3,3,3,4),(28.2743338823081,28.3292568500224,
28.423495469431,28.5176062557521,28.6116177584166,28.7055619944834,28.7994720188599,
28.8933734811464,28.9872920165809,29.0813117820562,29.1753870862621,29.2696144175385,
29.324318044526,29.4185565889438,29.5126672998036,29.6066787266445,29.7006228866682,
29.7945328348948,29.8884342210195,29.9823526803752,30.0763723703673,30.1704475993146,
30.2646748564353,30.3193792390296,30.4135944930383,30.5007612509717),
 .UNSPECIFIED.);
#379=B_SPLINE_CURVE_WITH_KNOTS('',3,(#29176,#29177,#29178,#29179,#29180,
#29181,#29182,#29183,#29184,#29185,#29186,#29187,#29188,#29189,#29190,#29191,
#29192,#29193,#29194,#29195,#29196,#29197,#29198,#29199,#29200,#29201,#29202,
#29203,#29204,#29205,#29206,#29207,#29208,#29209,#29210,#29211,#29212,#29213,
#29214,#29215,#29216,#29217,#29218,#29219,#29220,#29221,#29222,#29223,#29224,
#29225,#29226,#29227,#29228,#29229,#29230,#29231,#29232,#29233,#29234,#29235,
#29236,#29237,#29238,#29239,#29240,#29241,#29242,#29243,#29244,#29245,#29246,
#29247,#29248,#29249,#29250,#29251,#29252,#29253,#29254,#29255,#29256,#29257,
#29258,#29259,#29260,#29261,#29262,#29263,#29264,#29265,#29266,#29267,#29268,
#29269,#29270,#29271,#29272,#29273,#29274,#29275,#29276,#29277,#29278,#29279,
#29280,#29281,#29282,#29283,#29284,#29285,#29286,#29287,#29288,#29289,#29290,
#29291,#29292,#29293,#29294,#29295,#29296,#29297,#29298,#29299,#29300,#29301,
#29302,#29303,#29304,#29305,#29306,#29307,#29308,#29309,#29310,#29311),
 .UNSPECIFIED.,.F.,.F.,(4,3,3,3,3,3,3,3,3,3,3,3,3,3,3,3,3,3,3,3,3,3,3,3,
3,3,3,3,3,3,3,3,3,3,3,3,3,3,3,3,3,3,3,3,3,4),(24.216482857356,24.3107193521127,
24.3490120720079,24.4432488148445,24.5373576970504,24.6313672708521,24.72530954913,
24.8192175985477,24.91311707111,25.0070336044477,25.1010513610802,25.1951246496571,
25.2893499744683,25.3440732665115,25.4383123567688,25.5324236179415,25.6264355987757,
25.7203803159484,25.8142908230647,25.9081927691272,26.0021117887765,26.0961320361662,
26.1902078217006,26.2844356286052,26.3391344610152,26.4333731465367,26.5274840022162,
26.6214955773734,26.7154398903322,26.809349994297,26.903251538779,26.9971701589291,
27.0911900124797,27.185265406789,27.2794928305046,27.3341956555188,27.4276603575711,
27.5209978653467,27.6151648674452,27.7083395791818,27.8014834289019,27.894622918338,
27.9895506592872,28.0828117812111,28.178572831673,28.2743338821349),
 .UNSPECIFIED.);
#380=B_SPLINE_CURVE_WITH_KNOTS('',3,(#29317,#29318,#29319,#29320,#29321,
#29322,#29323,#29324,#29325,#29326,#29327,#29328,#29329,#29330,#29331,#29332,
#29333,#29334,#29335,#29336,#29337,#29338,#29339,#29340,#29341,#29342,#29343,
#29344,#29345,#29346,#29347,#29348,#29349,#29350,#29351,#29352,#29353,#29354,
#29355,#29356,#29357,#29358,#29359,#29360,#29361,#29362,#29363,#29364,#29365,
#29366,#29367,#29368,#29369,#29370,#29371,#29372,#29373,#29374,#29375,#29376,
#29377,#29378,#29379,#29380,#29381,#29382,#29383,#29384,#29385,#29386,#29387,
#29388,#29389,#29390,#29391,#29392),.UNSPECIFIED.,.F.,.F.,(4,3,3,3,3,3,
3,3,3,3,3,3,3,3,3,3,3,3,3,3,3,3,3,3,3,4),(15.7079632679489,15.8009022570379,
15.8938127630074,15.9867214110195,16.0796548185911,16.1726969971519,16.2658032398934,
16.3590599897109,16.388522515979,16.482850675556,16.577050577067,16.6711506419944,
16.7651822193176,16.8591787913051,16.9531658921126,17.0471690407496,17.1412713132475,
17.235428054019,17.329734309839,17.3835837104827,17.4779692848255,17.5722355767653,
17.6663981576832,17.7604990407976,17.8545789396576,17.9336096034474),
 .UNSPECIFIED.);
#381=B_SPLINE_CURVE_WITH_KNOTS('',3,(#29394,#29395,#29396,#29397,#29398),
 .UNSPECIFIED.,.F.,.F.,(4,1,4),(14.3984001269718,15.3934613214754,15.7079548718395),
 .UNSPECIFIED.);
#382=B_SPLINE_CURVE_WITH_KNOTS('',3,(#29402,#29403,#29404,#29405,#29406,
#29407,#29408,#29409,#29410,#29411,#29412,#29413,#29414,#29415,#29416,#29417,
#29418,#29419,#29420,#29421,#29422,#29423,#29424,#29425,#29426,#29427,#29428,
#29429,#29430,#29431,#29432,#29433,#29434,#29435,#29436,#29437,#29438,#29439,
#29440,#29441,#29442,#29443,#29444,#29445,#29446,#29447,#29448,#29449,#29450,
#29451,#29452,#29453,#29454,#29455,#29456,#29457,#29458,#29459,#29460,#29461,
#29462,#29463,#29464,#29465),.UNSPECIFIED.,.F.,.F.,(4,3,3,3,3,3,3,3,3,3,
3,3,3,3,3,3,3,3,3,3,3,4),(13.875933913584,13.9698176198018,14.0635739700505,
14.1611487795215,14.2547391272248,14.3482980121981,14.4418514975605,14.5354256347481,
14.6291003941672,14.7228347639158,14.8167105981944,14.8441724458185,14.9372024528207,
15.0335475547118,15.1263491052847,15.2190970034976,15.3118181687131,15.4045394876794,
15.4973328718652,15.5901696304292,15.6831249272467,15.7079632679489),
 .UNSPECIFIED.);
#383=B_SPLINE_CURVE_WITH_KNOTS('',3,(#29466,#29467,#29468,#29469,#29470,
#29471,#29472),.UNSPECIFIED.,.F.,.F.,(4,1,1,1,4),(15.7079632679489,15.8392336403222,
16.8342948348258,17.8293560293294,17.9343967671566),.UNSPECIFIED.);
#384=B_SPLINE_CURVE_WITH_KNOTS('',3,(#29478,#29479,#29480,#29481,#29482,
#29483,#29484,#29485,#29486,#29487,#29488,#29489),.UNSPECIFIED.,.F.,.F.,
(4,2,2,2,2,4),(-0.0891744238985337,-0.0496035464748441,-0.0101627518981445,
-0.0043205186654138,-0.00194322075801571,0.),.UNSPECIFIED.);
#385=B_SPLINE_CURVE_WITH_KNOTS('',3,(#29497,#29498,#29499,#29500,#29501,
#29502,#29503,#29504,#29505,#29506,#29507,#29508,#29509,#29510,#29511,#29512,
#29513,#29514,#29515,#29516,#29517,#29518,#29519,#29520,#29521,#29522,#29523,
#29524,#29525,#29526,#29527,#29528,#29529,#29530,#29531,#29532,#29533,#29534,
#29535,#29536,#29537,#29538,#29539,#29540,#29541,#29542,#29543,#29544,#29545,
#29546,#29547,#29548,#29549,#29550,#29551,#29552,#29553,#29554,#29555,#29556,
#29557,#29558,#29559,#29560,#29561,#29562,#29563),.UNSPECIFIED.,.F.,.F.,
(4,3,3,3,3,3,3,3,3,3,3,3,3,3,3,3,3,3,3,3,3,3,4),(-119.380510126605,-119.281824003816,
-119.183277779352,-119.08484394797,-118.986471229893,-118.88812931942,-118.789787948957,
-118.691351781982,-118.592868088032,-118.494214874655,-118.41228214593,
-118.313062108565,-118.213979277463,-118.114384486708,-118.015471660298,
-117.916589188221,-117.817707520535,-117.717585878258,-117.618559601633,
-117.517890276529,-117.417220951426,-117.311975507606,-117.299671991106),
 .UNSPECIFIED.);
#386=B_SPLINE_CURVE_WITH_KNOTS('',3,(#29569,#29570,#29571,#29572,#29573,
#29574,#29575,#29576,#29577,#29578,#29579,#29580,#29581,#29582,#29583,#29584,
#29585,#29586,#29587,#29588,#29589,#29590,#29591,#29592,#29593,#29594,#29595,
#29596,#29597,#29598,#29599,#29600,#29601,#29602,#29603,#29604,#29605,#29606,
#29607,#29608,#29609,#29610,#29611,#29612,#29613,#29614,#29615,#29616,#29617,
#29618,#29619,#29620,#29621,#29622,#29623,#29624,#29625,#29626,#29627,#29628,
#29629,#29630,#29631,#29632,#29633,#29634,#29635,#29636,#29637,#29638,#29639,
#29640,#29641,#29642,#29643,#29644,#29645,#29646,#29647,#29648,#29649,#29650,
#29651,#29652,#29653,#29654,#29655,#29656,#29657,#29658,#29659,#29660,#29661,
#29662,#29663,#29664,#29665,#29666,#29667,#29668,#29669,#29670,#29671,#29672,
#29673,#29674,#29675,#29676,#29677,#29678,#29679,#29680,#29681,#29682,#29683,
#29684,#29685,#29686,#29687,#29688,#29689,#29690,#29691,#29692,#29693,#29694,
#29695,#29696,#29697,#29698,#29699,#29700,#29701,#29702,#29703,#29704,#29705,
#29706,#29707,#29708,#29709,#29710,#29711,#29712,#29713,#29714,#29715,#29716,
#29717,#29718,#29719,#29720,#29721,#29722,#29723,#29724,#29725,#29726,#29727,
#29728,#29729,#29730,#29731,#29732,#29733,#29734,#29735,#29736,#29737,#29738,
#29739,#29740,#29741,#29742,#29743,#29744,#29745,#29746,#29747,#29748,#29749,
#29750,#29751,#29752),.UNSPECIFIED.,.F.,.F.,(4,3,3,3,3,3,3,3,3,3,3,3,3,
3,3,3,3,3,3,3,3,3,3,3,3,3,3,3,3,3,3,3,3,3,3,3,3,3,3,3,3,3,3,3,3,3,3,3,3,
3,3,3,3,3,3,3,3,3,3,3,3,4),(114.761320057655,114.860067511219,114.958791860699,
115.057522860401,115.156355627907,115.25524135556,115.354296888589,115.427098562419,
115.526175962403,115.625113193801,115.724744014191,115.82350509915,115.922233863131,
116.020960064793,116.121259987825,116.220128053757,116.32114390534,116.422159756923,
116.521103426722,116.619906372427,116.719570694802,116.818197115993,116.916791368532,
117.015383389193,117.115842779751,117.214578838161,117.315899894793,117.417220951426,
117.516458226383,117.615554601375,117.715145544445,117.814062836174,117.912946357322,
118.011825660325,118.111939781727,118.21095533248,118.311618739205,118.41228214593,
118.511423730653,118.610426918485,118.710041471229,118.808872273556,118.907671994955,
119.006470285157,119.106688548976,119.205630694478,119.306487017455,119.407343340433,
119.505449657559,119.603415177681,119.703288847338,119.801083195662,119.898848954802,
119.99661701861,120.098063897692,120.195995241008,120.294006021494,120.392183906562,
120.402404534937,120.533901068514,120.662199975167,120.69007258227),
 .UNSPECIFIED.);
#387=B_SPLINE_CURVE_WITH_KNOTS('',3,(#29753,#29754,#29755,#29756,#29757,
#29758,#29759,#29760,#29761,#29762,#29763,#29764,#29765,#29766,#29767,#29768,
#29769,#29770,#29771,#29772),.UNSPECIFIED.,.F.,.F.,(4,2,2,2,2,2,2,2,2,4),
(-0.178840503134635,-0.141813169590022,-0.126245575166451,-0.120975056350671,
-0.117078626547339,-0.11313785577946,-0.109546939480627,-0.103794973539924,
-0.0894553738401638,-0.0891744238985337),.UNSPECIFIED.);
#388=B_SPLINE_CURVE_WITH_KNOTS('',3,(#29774,#29775,#29776,#29777,#29778,
#29779,#29780,#29781,#29782,#29783,#29784,#29785,#29786),.UNSPECIFIED.,
 .F.,.F.,(4,3,3,3,4),(-117.299671991106,-117.194784025774,-117.090099445131,
-116.985683593692,-116.946309934874),.UNSPECIFIED.);
#389=B_SPLINE_CURVE_WITH_KNOTS('',3,(#29787,#29788,#29789,#29790,#29791,
#29792,#29793,#29794,#29795,#29796),.UNSPECIFIED.,.F.,.F.,(4,1,1,1,1,1,
1,4),(-116.946309934874,-116.422159756923,-115.427098562419,-114.432037367915,
-113.436976173412,-112.441914978908,-111.446853784405,-111.016736858085),
 .UNSPECIFIED.);
#390=B_SPLINE_CURVE_WITH_KNOTS('',3,(#29802,#29803,#29804,#29805,#29806,
#29807,#29808,#29809,#29810,#29811,#29812,#29813,#29814,#29815,#29816,#29817,
#29818,#29819,#29820,#29821,#29822,#29823,#29824,#29825,#29826,#29827,#29828,
#29829,#29830,#29831,#29832,#29833,#29834,#29835,#29836,#29837,#29838,#29839,
#29840,#29841,#29842,#29843,#29844,#29845,#29846,#29847,#29848,#29849,#29850,
#29851,#29852,#29853,#29854,#29855,#29856,#29857,#29858,#29859,#29860,#29861,
#29862,#29863,#29864,#29865,#29866,#29867,#29868,#29869,#29870,#29871,#29872,
#29873,#29874,#29875,#29876,#29877,#29878,#29879,#29880,#29881,#29882,#29883,
#29884,#29885,#29886,#29887,#29888,#29889,#29890,#29891,#29892,#29893,#29894,
#29895,#29896,#29897,#29898,#29899,#29900,#29901,#29902,#29903,#29904,#29905,
#29906,#29907,#29908,#29909,#29910,#29911,#29912,#29913,#29914,#29915,#29916,
#29917,#29918,#29919,#29920,#29921,#29922,#29923,#29924,#29925,#29926,#29927,
#29928,#29929,#29930,#29931,#29932,#29933,#29934,#29935,#29936,#29937,#29938,
#29939,#29940,#29941,#29942,#29943,#29944,#29945,#29946,#29947,#29948,#29949,
#29950,#29951,#29952,#29953,#29954,#29955,#29956,#29957,#29958,#29959,#29960,
#29961,#29962,#29963,#29964,#29965,#29966,#29967,#29968,#29969,#29970,#29971,
#29972,#29973,#29974,#29975,#29976,#29977,#29978,#29979,#29980,#29981,#29982),
 .UNSPECIFIED.,.F.,.F.,(4,3,3,3,3,3,3,3,3,3,3,3,3,3,3,3,3,3,3,3,3,3,3,3,
3,3,3,3,3,3,3,3,3,3,3,3,3,3,3,3,3,3,3,3,3,3,3,3,3,3,3,3,3,3,3,3,3,3,3,3,
4),(108.477770244024,108.576804478106,108.675703662613,108.774496605418,
108.873231844062,108.971939195394,109.070648441376,109.169456830148,109.268313938915,
109.367346518269,109.456731395397,109.555791102734,109.654710371096,109.754345648446,
109.853088250073,109.951798378069,110.050505817417,110.150827510538,110.249676699491,
110.350734644696,110.451792589901,110.550849698287,110.649766361109,110.74940228902,
110.84814228808,110.946849820364,111.045554674319,111.14587945184,111.244726107047,
111.345789945725,111.446853784404,111.545914922601,111.644835605295,111.744470526997,
111.843214492961,111.941925963677,112.040634722456,112.140954786569,112.239805224716,
112.340860101812,112.441914978908,112.540977599963,112.639899812681,112.739534357772,
112.838279956175,112.936993093827,113.035703551551,113.136021707016,113.234873904593,
113.335925039003,113.436976173412,113.535605508397,113.634094697856,113.732471458206,
113.830787072003,113.929071919081,114.027356341127,114.125736595437,114.224164571909,
114.322764300366,114.406898669987),.UNSPECIFIED.);
#391=B_SPLINE_CURVE_WITH_KNOTS('',3,(#29983,#29984,#29985,#29986,#29987,
#29988,#29989,#29990,#29991,#29992,#29993,#29994,#29995,#29996,#29997,#29998),
 .UNSPECIFIED.,.F.,.F.,(4,3,3,3,3,4),(114.40689867021,114.432037367915,
114.531097614611,114.63003462159,114.72885969336,114.761320057655),
 .UNSPECIFIED.);
#392=B_SPLINE_CURVE_WITH_KNOTS('',3,(#30000,#30001,#30002,#30003),
 .UNSPECIFIED.,.F.,.F.,(4,4),(-111.016736858085,-110.663126671174),
 .UNSPECIFIED.);
#393=B_SPLINE_CURVE_WITH_KNOTS('',3,(#30004,#30005,#30006,#30007,#30008,
#30009,#30010,#30011,#30012,#30013,#30014,#30015,#30016,#30017,#30018,#30019,
#30020,#30021,#30022,#30023,#30024,#30025,#30026,#30027,#30028,#30029,#30030,
#30031,#30032,#30033,#30034,#30035,#30036,#30037,#30038,#30039,#30040,#30041,
#30042,#30043,#30044,#30045,#30046,#30047,#30048,#30049,#30050,#30051,#30052,
#30053,#30054,#30055,#30056,#30057,#30058,#30059,#30060,#30061,#30062,#30063,
#30064,#30065,#30066,#30067,#30068,#30069,#30070,#30071,#30072,#30073,#30074,
#30075,#30076,#30077,#30078,#30079,#30080,#30081,#30082,#30083,#30084,#30085,
#30086,#30087,#30088,#30089,#30090,#30091,#30092,#30093,#30094,#30095,#30096,
#30097,#30098,#30099,#30100,#30101,#30102,#30103,#30104,#30105,#30106,#30107,
#30108,#30109,#30110,#30111,#30112,#30113,#30114,#30115,#30116,#30117,#30118,
#30119,#30120,#30121,#30122,#30123,#30124,#30125,#30126,#30127,#30128,#30129,
#30130,#30131,#30132,#30133,#30134,#30135,#30136,#30137,#30138,#30139,#30140,
#30141,#30142,#30143,#30144,#30145,#30146,#30147,#30148,#30149,#30150,#30151,
#30152,#30153,#30154,#30155,#30156,#30157,#30158,#30159,#30160,#30161,#30162,
#30163,#30164,#30165,#30166,#30167,#30168,#30169,#30170,#30171,#30172,#30173,
#30174,#30175,#30176,#30177,#30178,#30179,#30180,#30181,#30182,#30183,#30184,
#30185,#30186,#30187,#30188,#30189,#30190,#30191,#30192,#30193,#30194,#30195,
#30196,#30197,#30198,#30199),.UNSPECIFIED.,.F.,.F.,(4,2,2,2,2,2,2,2,2,2,
2,2,2,2,2,2,2,2,2,2,2,2,2,2,2,2,2,2,2,2,2,2,2,2,2,2,2,2,2,2,2,2,2,2,2,2,
2,2,2,2,2,2,2,2,2,2,2,2,2,2,2,2,2,2,2,2,2,2,2,2,2,2,2,2,2,2,2,2,2,2,2,2,
2,2,2,2,2,2,2,2,2,2,2,2,2,2,2,4),(-3.17357790823559,-3.12979346273682,-3.12593076395734,
-3.12347643776689,-3.1211769410646,-3.119214678798,-3.11668020948361,-3.11253627497692,
-3.07720090000462,-3.04609543198994,-3.00836826368396,-3.00093513976047,
-2.9967042786001,-2.9935565107799,-2.98960312508386,-2.98286326098669,-2.9566808240345,
-2.89669536297659,-2.87623910016699,-2.87228075136747,-2.86995070680013,
-2.86799119315247,-2.86549692111373,-2.86148827761377,-2.83625400853403,
-2.78992482397229,-2.75579095842182,-2.7488298752571,-2.74482858885487,
-2.7413369307013,-2.73700951754869,-2.73032195565072,-2.68310823494367,
-2.64908548782712,-2.62510115459664,-2.62089062446662,-2.61859075072306,
-2.61662837427167,-2.61409394361257,-2.60995021278302,-2.57555402720399,
-2.50879733975849,-2.49919798758817,-2.49466266245402,-2.4911502642112,
-2.48727669215012,-2.48090199051045,-2.45904305875434,-2.40129094881048,
-2.38272990119718,-2.37206266247051,-2.36875609378411,-2.3666544435217,
-2.36464745659887,-2.3621651327232,-2.35602764800739,-2.30725456870824,
-2.27752702082482,-2.25217547315175,-2.24574098049604,-2.2418542696633,
-2.23834477455688,-2.23383396642056,-2.22436550020225,-2.16434426128313,
-2.12446738983707,-2.11899333033687,-2.11643903370558,-2.11449253073795,
-2.11221351407662,-2.10820956447202,-2.09073378455542,-2.02149873611586,
-2.00733261126076,-1.99693387191696,-1.99225281717305,-1.98872044498262,
-1.98491499560063,-1.97885224162176,-1.95988848354198,-1.94872277603346,
-1.89713060891502,-1.87959725169687,-1.87268661520277,-1.86751620560193,
-1.86502022242423,-1.86324811851203,-1.86099667659176,-1.85711269440354,
-1.84134505355604,-1.77041524509253,-1.74887593022735,-1.74275954437367,
-1.73894278031217,-1.73541501400231,-1.73084137269319,-1.72113555474525,
-1.67627843319428),.UNSPECIFIED.);
#394=B_SPLINE_CURVE_WITH_KNOTS('',3,(#30205,#30206,#30207,#30208,#30209,
#30210,#30211,#30212,#30213,#30214,#30215,#30216,#30217,#30218,#30219,#30220,
#30221,#30222,#30223,#30224,#30225,#30226,#30227,#30228,#30229,#30230,#30231,
#30232,#30233,#30234,#30235,#30236,#30237,#30238,#30239,#30240,#30241,#30242,
#30243,#30244,#30245,#30246,#30247,#30248,#30249,#30250,#30251,#30252,#30253,
#30254,#30255,#30256,#30257,#30258,#30259,#30260,#30261,#30262,#30263,#30264,
#30265,#30266,#30267,#30268,#30269,#30270,#30271,#30272,#30273,#30274,#30275,
#30276,#30277,#30278,#30279,#30280,#30281,#30282,#30283,#30284,#30285,#30286,
#30287,#30288,#30289,#30290,#30291,#30292,#30293,#30294,#30295,#30296,#30297,
#30298,#30299,#30300,#30301,#30302,#30303,#30304,#30305,#30306,#30307,#30308,
#30309,#30310,#30311,#30312,#30313,#30314,#30315,#30316,#30317,#30318,#30319,
#30320,#30321,#30322,#30323,#30324,#30325,#30326,#30327,#30328,#30329,#30330,
#30331,#30332,#30333,#30334,#30335,#30336,#30337,#30338,#30339,#30340,#30341,
#30342,#30343,#30344,#30345,#30346,#30347,#30348,#30349,#30350,#30351,#30352,
#30353,#30354,#30355,#30356,#30357,#30358,#30359,#30360,#30361,#30362,#30363,
#30364,#30365,#30366,#30367,#30368,#30369,#30370,#30371,#30372,#30373,#30374,
#30375,#30376,#30377,#30378,#30379,#30380,#30381,#30382,#30383,#30384,#30385),
 .UNSPECIFIED.,.F.,.F.,(4,3,3,3,3,3,3,3,3,3,3,3,3,3,3,3,3,3,3,3,3,3,3,3,
3,3,3,3,3,3,3,3,3,3,3,3,3,3,3,3,3,3,3,3,3,3,3,3,3,3,3,3,3,3,3,3,3,3,3,3,
4),(102.19402465094,102.293056429024,102.392278375189,102.491303033872,
102.590362152007,102.68928082678,102.78891625198,102.887658253753,102.98636778089,
103.085074619194,103.18539702149,103.284245615113,103.385304921744,103.486364228376,
103.585423359634,103.684342047628,103.783977469535,103.88271948467,103.981429025192,
104.080135876886,104.180458263384,104.27930687027,104.380366146575,104.481425422879,
104.580484508879,104.679403151563,104.779038584791,104.877780554818,104.976490050407,
105.075196857402,105.175519297397,105.274367860614,105.375427238998,105.476486617383,
105.575545749521,105.674464438071,105.774099859798,105.872841874706,105.97155141471,
106.070258265596,106.170580652169,106.269429257555,106.370488534721,106.471547811886,
106.570607021582,106.66952578848,106.769161190719,106.867903285305,106.966612905307,
107.065319836401,107.165642128898,107.264490814177,107.365549910283,107.46660900639,
107.565721146446,107.664694944783,107.763560266908,107.86234948203,107.961092970623,
108.059846334627,108.12371336303),.UNSPECIFIED.);
#395=B_SPLINE_CURVE_WITH_KNOTS('',3,(#30386,#30387,#30388,#30389,#30390,
#30391,#30392,#30393,#30394,#30395,#30396,#30397,#30398),.UNSPECIFIED.,
 .F.,.F.,(4,3,3,3,4),(108.12371336339,108.237935255045,108.353262022111,
108.461670200894,108.477770244024),.UNSPECIFIED.);
#396=B_SPLINE_CURVE_WITH_KNOTS('',3,(#30399,#30400,#30401,#30402,#30403,
#30404,#30405,#30406,#30407,#30408,#30409,#30410,#30411,#30412,#30413,#30414,
#30415,#30416,#30417,#30418,#30419,#30420,#30421,#30422,#30423,#30424,#30425,
#30426,#30427,#30428,#30429,#30430,#30431,#30432,#30433,#30434,#30435,#30436,
#30437,#30438,#30439,#30440,#30441,#30442,#30443,#30444,#30445,#30446,#30447,
#30448,#30449,#30450,#30451,#30452,#30453,#30454,#30455,#30456,#30457,#30458,
#30459,#30460,#30461,#30462,#30463,#30464,#30465,#30466,#30467,#30468,#30469,
#30470,#30471,#30472,#30473,#30474,#30475,#30476,#30477,#30478,#30479,#30480,
#30481,#30482,#30483,#30484,#30485,#30486,#30487,#30488,#30489,#30490,#30491,
#30492,#30493,#30494,#30495,#30496,#30497,#30498,#30499,#30500,#30501,#30502,
#30503,#30504,#30505,#30506,#30507,#30508,#30509,#30510,#30511,#30512,#30513,
#30514,#30515,#30516,#30517,#30518,#30519,#30520,#30521,#30522,#30523,#30524,
#30525,#30526,#30527,#30528,#30529,#30530,#30531,#30532,#30533,#30534,#30535,
#30536,#30537,#30538,#30539,#30540,#30541,#30542,#30543,#30544,#30545,#30546,
#30547,#30548,#30549,#30550,#30551,#30552,#30553,#30554,#30555,#30556,#30557,
#30558,#30559,#30560,#30561,#30562,#30563,#30564,#30565,#30566,#30567,#30568,
#30569,#30570,#30571,#30572,#30573,#30574,#30575,#30576,#30577,#30578,#30579,
#30580,#30581,#30582,#30583,#30584,#30585,#30586,#30587,#30588,#30589,#30590,
#30591,#30592,#30593,#30594,#30595,#30596,#30597,#30598,#30599,#30600,#30601,
#30602,#30603,#30604,#30605,#30606,#30607,#30608,#30609,#30610,#30611,#30612,
#30613,#30614,#30615,#30616,#30617,#30618,#30619,#30620,#30621,#30622,#30623,
#30624),.UNSPECIFIED.,.F.,.F.,(4,2,2,2,2,2,2,2,2,2,2,2,2,2,2,2,2,2,2,2,
2,2,2,2,2,2,2,2,2,2,2,2,2,2,2,2,2,2,2,2,2,2,2,2,2,2,2,2,2,2,2,2,2,2,2,2,
2,2,2,2,2,2,2,2,2,2,2,2,2,2,2,2,2,2,2,2,2,2,2,2,2,2,2,2,2,2,2,2,2,2,2,2,
2,2,2,2,2,2,2,2,2,2,2,2,2,2,2,2,2,2,2,2,4),(-1.67627843319428,-1.66639710885997,
-1.62175007372191,-1.61632633228209,-1.61378191144318,-1.61181909335474,
-1.60952721381829,-1.60546516618932,-1.5870545286888,-1.5488705408948,-1.50004385234283,
-1.49335660614414,-1.48902994844544,-1.4855392313552,-1.48153938705054,
-1.47458173804716,-1.44048275966846,-1.38713403887994,-1.36841168351906,
-1.36432944439178,-1.36203298095122,-1.36007074387167,-1.35753289569351,
-1.35214386950049,-1.30767616711323,-1.25263791439702,-1.24281819148523,
-1.23829164261158,-1.23477085926177,-1.23093219358501,-1.22471505248399,
-1.20204426838429,-1.15686220004863,-1.14448152278534,-1.11781581791389,
-1.11375476189054,-1.11124527065836,-1.10928538903317,-1.10696862856517,
-1.10267684680963,-1.07643690716525,-1.02366380264669,-0.996477277876009,
-0.989746221280685,-0.985757497749172,-0.982299187811502,-0.97797384203867,
-0.969455117625521,-0.95850625782231,-0.932100235446576,-0.895789011145295,
-0.86667208461556,-0.862589377129645,-0.86007352901182,-0.858113299618529,
-0.855801561005835,-0.851532940145751,-0.825961943601439,-0.775419296037052,
-0.745604062262852,-0.738711876987958,-0.73468666865785,-0.731198768333297,
-0.726907565002085,-0.718557857908503,-0.667291122726274,-0.618093004951914,
-0.611981572897479,-0.609504260270671,-0.607499069966088,-0.605396527039538,
-0.602083723675056,-0.591353893081907,-0.57262586593982,-0.51296750366228,
-0.492876941554744,-0.486691526098369,-0.482860144684468,-0.479337865418448,
-0.474720272561702,-0.464669518094046,-0.451119228271358,-0.413742392379747,
-0.367121008886682,-0.360855969057173,-0.358352433549508,-0.356522081176278,
-0.354472859369076,-0.351406222596919,-0.342702196891811,-0.328840114076413,
-0.264182848743525,-0.242089245399464,-0.235689991207248,-0.231812179741444,
-0.228450119783473,-0.228393888750984,-0.228342085052784,-0.228294229412539,
-0.228249910148991,-0.228208771500177,-0.223847818883286,-0.218968131988291,
-0.210884133534484,-0.194071607632333,-0.164215288729475,-0.11576510171549,
-0.109613820321097,-0.107129860694167,-0.105123125874876,-0.103023683126422,
-0.0997239845329725,-0.0900473953080078),.UNSPECIFIED.);
#397=B_SPLINE_CURVE_WITH_KNOTS('',3,(#30630,#30631,#30632,#30633,#30634,
#30635,#30636,#30637,#30638,#30639,#30640,#30641,#30642,#30643,#30644,#30645,
#30646,#30647,#30648,#30649,#30650,#30651,#30652,#30653,#30654,#30655,#30656,
#30657,#30658,#30659,#30660,#30661,#30662,#30663,#30664,#30665,#30666,#30667,
#30668,#30669,#30670,#30671,#30672,#30673,#30674,#30675,#30676,#30677,#30678,
#30679,#30680,#30681,#30682,#30683,#30684,#30685,#30686,#30687,#30688,#30689,
#30690,#30691,#30692,#30693,#30694,#30695,#30696,#30697,#30698,#30699,#30700,
#30701,#30702,#30703,#30704,#30705,#30706,#30707,#30708,#30709,#30710,#30711,
#30712,#30713,#30714,#30715,#30716,#30717,#30718,#30719,#30720,#30721,#30722,
#30723,#30724,#30725,#30726,#30727,#30728,#30729,#30730,#30731,#30732,#30733,
#30734,#30735,#30736,#30737,#30738,#30739,#30740,#30741,#30742,#30743,#30744,
#30745,#30746,#30747,#30748,#30749,#30750,#30751,#30752,#30753,#30754,#30755,
#30756,#30757,#30758,#30759,#30760,#30761,#30762,#30763,#30764,#30765,#30766,
#30767,#30768,#30769,#30770,#30771,#30772,#30773,#30774,#30775,#30776,#30777,
#30778,#30779,#30780,#30781,#30782,#30783,#30784,#30785,#30786,#30787,#30788,
#30789,#30790,#30791,#30792,#30793,#30794,#30795,#30796,#30797,#30798,#30799,
#30800,#30801,#30802,#30803,#30804,#30805,#30806,#30807,#30808,#30809,#30810),
 .UNSPECIFIED.,.F.,.F.,(4,3,3,3,3,3,3,3,3,3,3,3,3,3,3,3,3,3,3,3,3,3,3,3,
3,3,3,3,3,3,3,3,3,3,3,3,3,3,3,3,3,3,3,3,3,3,3,3,3,3,3,3,3,3,3,3,3,3,3,3,
4),(95.9117775219804,96.0099930662897,96.1081979885838,96.2113824581504,
96.309718345621,96.4081216556358,96.5066772687822,96.5209358668503,96.6199949843994,
96.7189136586225,96.8185490839639,96.9172910852772,97.0160006119892,97.1147074499024,
97.2150298527653,97.313878446087,97.4149377537205,97.5159970613539,97.615056179209,
97.7139748537395,97.8136102790043,97.9123522806262,98.0110618076464,98.1097686458675,
98.210091048365,98.3089396419895,98.4099989489235,98.5110582558575,98.6101173729991,
98.7090360468166,98.8086714722597,98.9074134731739,99.0061229994903,99.104829837012,
99.2051522403493,99.3040008332928,99.405060141827,99.5061194503612,99.6051785678429,
99.7040972419944,99.8037326673532,99.902474668585,100.001184195212,100.099891033037,
100.200213435994,100.299062029221,100.400121337043,100.501180644865,100.600239764403,
100.699158440622,100.798793865465,100.897535868779,100.996245397488,101.094952237394,
101.195274637887,101.294123233167,101.395182536267,101.496241839368,101.611067080966,
101.725797568223,101.84052805548),.UNSPECIFIED.);
#398=B_SPLINE_CURVE_WITH_KNOTS('',3,(#30811,#30812,#30813,#30814,#30815,
#30816,#30817,#30818,#30819,#30820,#30821,#30822,#30823),.UNSPECIFIED.,
 .F.,.F.,(4,3,3,3,4),(101.84052805585,101.939398955072,102.038252712645,
102.137156873093,102.19402465094),.UNSPECIFIED.);
#399=B_SPLINE_CURVE_WITH_KNOTS('',3,(#30825,#30826,#30827,#30828,#30829,
#30830,#30831,#30832),.UNSPECIFIED.,.F.,.F.,(4,2,2,4),(-0.0900473953080078,
-0.0891091977982808,-0.0706763169128908,-0.000735701929119057),
 .UNSPECIFIED.);
#400=B_SPLINE_CURVE_WITH_KNOTS('',3,(#30833,#30834,#30835,#30836,#30837,
#30838,#30839,#30840,#30841,#30842,#30843,#30844,#30845,#30846,#30847,#30848,
#30849,#30850,#30851,#30852,#30853,#30854,#30855,#30856,#30857,#30858,#30859,
#30860,#30861,#30862,#30863,#30864,#30865,#30866,#30867,#30868,#30869,#30870,
#30871,#30872,#30873,#30874,#30875,#30876,#30877,#30878,#30879,#30880,#30881,
#30882,#30883,#30884,#30885,#30886,#30887,#30888,#30889,#30890,#30891,#30892,
#30893,#30894,#30895,#30896,#30897,#30898,#30899,#30900,#30901,#30902,#30903,
#30904,#30905,#30906,#30907,#30908,#30909,#30910,#30911,#30912,#30913,#30914,
#30915,#30916,#30917,#30918,#30919,#30920,#30921,#30922,#30923,#30924,#30925,
#30926,#30927,#30928,#30929,#30930,#30931,#30932,#30933,#30934,#30935,#30936,
#30937,#30938,#30939,#30940,#30941,#30942,#30943,#30944,#30945,#30946,#30947,
#30948,#30949,#30950,#30951,#30952,#30953,#30954,#30955,#30956,#30957,#30958,
#30959,#30960,#30961,#30962,#30963,#30964,#30965,#30966,#30967,#30968,#30969,
#30970,#30971,#30972,#30973,#30974,#30975,#30976,#30977,#30978,#30979,#30980,
#30981,#30982,#30983,#30984,#30985,#30986,#30987,#30988,#30989,#30990,#30991,
#30992,#30993,#30994,#30995,#30996,#30997,#30998,#30999,#31000,#31001,#31002,
#31003,#31004,#31005,#31006,#31007,#31008,#31009,#31010,#31011,#31012,#31013,
#31014,#31015,#31016,#31017,#31018,#31019,#31020,#31021,#31022,#31023,#31024,
#31025,#31026,#31027,#31028,#31029,#31030,#31031,#31032,#31033,#31034,#31035,
#31036,#31037,#31038,#31039,#31040,#31041,#31042),.UNSPECIFIED.,.F.,.F.,
(4,2,2,2,2,2,2,2,2,2,2,2,2,2,2,2,2,2,2,2,2,2,2,2,2,2,2,2,2,2,2,2,2,2,2,
2,2,2,2,2,2,2,2,2,2,2,2,2,2,2,2,2,2,2,2,2,2,2,2,2,2,2,2,2,2,2,2,2,2,2,2,
2,2,2,2,2,2,2,2,2,2,2,2,2,2,2,2,2,2,2,2,2,2,2,2,2,2,2,2,2,2,2,2,2,4),(-3.17216731230386,
-3.16150091109955,-3.15706135222654,-3.15363950664677,-3.1502747241594,
-3.14646252263513,-3.14036139560858,-3.12101710243409,-3.05783810323741,
-3.04091305881212,-3.0341636521033,-3.02908772453886,-3.02661108861964,
-3.02484204505949,-3.02257972701094,-3.01864471304799,-3.00215905357304,
-2.99408950606481,-2.953475865593,-2.92627126967372,-2.9151120828329,-2.90902930873973,
-2.90496975873134,-2.90112262783562,-2.89780194758751,-2.89347770156811,
-2.88679502367664,-2.83824735383611,-2.80111658919068,-2.78782751153759,
-2.77938305099513,-2.77635209006198,-2.77431067792622,-2.77247480173877,
-2.76945821243725,-2.76173768551373,-2.7101503769379,-2.66333258814837,
-2.65508823582814,-2.65081934424015,-2.64733392916629,-2.64329404828012,
-2.63633306320586,-2.60522340607424,-2.5553195740956,-2.53860089344422,
-2.53190645453539,-2.52686271279235,-2.52439248683972,-2.52262420595838,
-2.52035757281562,-2.51640335833064,-2.49963996646639,-2.43551997335584,
-2.41807375326111,-2.40590910910997,-2.40093334314769,-2.39735360228157,
-2.39408864104896,-2.38969603515127,-2.38110010028033,-2.32202946415757,
-2.28071453761144,-2.2756957484835,-2.27323053107066,-2.27146285698618,
-2.26919286460552,-2.26522358835,-2.24823657897472,-2.19463172011816,-2.17096427140933,
-2.16077442882095,-2.15272423985745,-2.14849527527369,-2.14535015460792,
-2.14140171060477,-2.13467430370914,-2.10861404513114,-2.0549295124778,
-2.02844890262111,-2.02415126045534,-2.02183401788994,-2.0198753759667,
-2.01736956368279,-2.01331842440849,-1.98685232221298,-1.97235854549532,
-1.93550011379477,-1.90722258753614,-1.90058851049009,-1.89666025441831,
-1.89316225987929,-1.8887332258888,-1.87968128872629,-1.81601967290809,
-1.7789972838733,-1.77367015581183,-1.77114491115142,-1.7691846565658,-1.76688144080074,
-1.76276604492914,-1.74343783266141,-1.73496306212675,-1.68973337728938,
-1.67575143484598),.UNSPECIFIED.);
#401=B_SPLINE_CURVE_WITH_KNOTS('',3,(#31048,#31049,#31050,#31051,#31052,
#31053,#31054,#31055,#31056,#31057,#31058,#31059,#31060,#31061,#31062,#31063,
#31064,#31065,#31066,#31067,#31068,#31069,#31070,#31071,#31072,#31073,#31074,
#31075,#31076,#31077,#31078,#31079,#31080,#31081,#31082,#31083,#31084,#31085,
#31086,#31087,#31088,#31089,#31090,#31091,#31092,#31093,#31094,#31095,#31096,
#31097,#31098,#31099,#31100,#31101,#31102,#31103,#31104,#31105,#31106,#31107,
#31108,#31109,#31110,#31111,#31112,#31113,#31114,#31115,#31116,#31117,#31118,
#31119,#31120,#31121,#31122,#31123,#31124,#31125,#31126,#31127,#31128,#31129,
#31130,#31131,#31132,#31133,#31134,#31135,#31136,#31137,#31138,#31139,#31140,
#31141,#31142,#31143,#31144,#31145,#31146,#31147,#31148,#31149,#31150,#31151,
#31152,#31153,#31154,#31155,#31156,#31157,#31158,#31159,#31160,#31161,#31162,
#31163,#31164,#31165,#31166,#31167,#31168,#31169,#31170,#31171,#31172,#31173,
#31174,#31175,#31176,#31177,#31178,#31179,#31180,#31181,#31182,#31183,#31184,
#31185,#31186,#31187,#31188,#31189,#31190,#31191,#31192,#31193,#31194,#31195,
#31196,#31197,#31198,#31199,#31200,#31201,#31202,#31203,#31204,#31205,#31206,
#31207,#31208,#31209,#31210,#31211,#31212,#31213,#31214,#31215,#31216,#31217,
#31218,#31219,#31220,#31221,#31222,#31223,#31224,#31225,#31226,#31227,#31228,
#31229,#31230,#31231),.UNSPECIFIED.,.F.,.F.,(4,3,3,3,3,3,3,3,3,3,3,3,3,
3,3,3,3,3,3,3,3,3,3,3,3,3,3,3,3,3,3,3,3,3,3,3,3,3,3,3,3,3,3,3,3,3,3,3,3,
3,3,3,3,3,3,3,3,3,3,3,3,4),(89.6284739524251,89.7274264175165,89.8303192028056,
89.9290729357282,90.0277873136882,90.1264921291014,90.2252171561015,90.3240521540832,
90.422952333698,90.5220097719534,90.5505686998287,90.649627817412,90.7485464916702,
90.8481819170029,90.9469239183524,91.045633445101,91.1443402830514,91.2446626858716,
91.3435112792307,91.4445705867815,91.5456298943322,91.6446890119216,91.7436076861859,
91.8432431115171,91.9419851128728,92.0406946396275,92.139401477584,92.239723880397,
92.3385724737621,92.439631781299,92.5406910888359,92.6397502064153,92.7386688806695,
92.8383043060033,92.937046307349,93.0357558340939,93.1344626720407,93.2347850748654,
93.3336336682211,93.4346929757803,93.5357522833395,93.6348114009167,93.7337300751687,
93.833365500503,93.9321075018462,94.0308170285885,94.1295238665326,94.2298462693603,
94.3286948627131,94.4297541702781,94.5308134778431,94.6298725954642,94.7287912697602,
94.8284266950835,94.9271686964708,95.025878223257,95.1245850612449,95.2249074640203,
95.3237560574162,95.4248153648815,95.5258746723467,95.5573427486708),
 .UNSPECIFIED.);
#402=B_SPLINE_CURVE_WITH_KNOTS('',3,(#31232,#31233,#31234,#31235,#31236,
#31237,#31238,#31239,#31240,#31241,#31242,#31243,#31244),.UNSPECIFIED.,
 .F.,.F.,(4,3,3,3,4),(95.5573427489414,95.6558631102801,95.7542623785887,
95.8525566861535,95.9117775219804),.UNSPECIFIED.);
#403=B_SPLINE_CURVE_WITH_KNOTS('',3,(#31245,#31246,#31247,#31248,#31249,
#31250,#31251,#31252,#31253,#31254,#31255,#31256,#31257,#31258,#31259,#31260,
#31261,#31262,#31263,#31264,#31265,#31266,#31267,#31268,#31269,#31270,#31271,
#31272,#31273,#31274,#31275,#31276,#31277,#31278,#31279,#31280,#31281,#31282,
#31283,#31284,#31285,#31286,#31287,#31288,#31289,#31290,#31291,#31292,#31293,
#31294,#31295,#31296,#31297,#31298,#31299,#31300,#31301,#31302,#31303,#31304,
#31305,#31306,#31307,#31308,#31309,#31310,#31311,#31312,#31313,#31314,#31315,
#31316,#31317,#31318,#31319,#31320,#31321,#31322,#31323,#31324,#31325,#31326,
#31327,#31328,#31329,#31330,#31331,#31332,#31333,#31334,#31335,#31336,#31337,
#31338,#31339,#31340,#31341,#31342,#31343,#31344,#31345,#31346,#31347,#31348,
#31349,#31350,#31351,#31352,#31353,#31354,#31355,#31356,#31357,#31358,#31359,
#31360,#31361,#31362,#31363,#31364,#31365,#31366,#31367,#31368,#31369,#31370,
#31371,#31372,#31373,#31374,#31375,#31376,#31377,#31378,#31379,#31380,#31381,
#31382,#31383,#31384,#31385,#31386,#31387,#31388,#31389,#31390,#31391,#31392,
#31393,#31394,#31395,#31396,#31397,#31398,#31399,#31400,#31401,#31402,#31403,
#31404,#31405,#31406,#31407,#31408,#31409,#31410,#31411,#31412,#31413,#31414,
#31415,#31416,#31417,#31418,#31419,#31420,#31421,#31422,#31423,#31424,#31425,
#31426,#31427,#31428,#31429,#31430,#31431,#31432,#31433,#31434,#31435,#31436,
#31437,#31438,#31439,#31440,#31441,#31442,#31443,#31444,#31445,#31446,#31447,
#31448,#31449,#31450,#31451,#31452,#31453,#31454,#31455,#31456,#31457,#31458,
#31459,#31460,#31461,#31462,#31463,#31464,#31465,#31466,#31467,#31468),
 .UNSPECIFIED.,.F.,.F.,(4,2,2,2,2,2,2,2,2,2,2,2,2,2,2,2,2,2,2,2,2,2,2,2,
2,2,2,2,2,2,2,2,2,2,2,2,2,2,2,2,2,2,2,2,2,2,2,2,2,2,2,2,2,2,2,2,2,2,2,2,
2,2,2,2,2,2,2,2,2,2,2,2,2,2,2,2,2,2,2,2,2,2,2,2,2,2,2,2,2,2,2,2,2,2,2,2,
2,2,2,2,2,2,2,2,2,2,2,2,2,2,2,4),(-1.67575143484598,-1.65659760087301,-1.64968873704058,
-1.64570073195418,-1.64221080669793,-1.63787271447791,-1.63114388060775,
-1.58622326395788,-1.54071426114126,-1.52550359318917,-1.5216265495086,
-1.51940001325016,-1.51742632422234,-1.51477769681934,-1.50878127891758,
-1.48173292771081,-1.47983099492858,-1.46488570894065,-1.41028476343868,
-1.400576122209,-1.39600327537135,-1.3924770473776,-1.38866286298393,-1.38255261067803,
-1.3610563928036,-1.29043405636996,-1.27444728676971,-1.27054837538144,
-1.26829424495471,-1.2665237858399,-1.26403497073859,-1.25889721131732,
-1.25204112447926,-1.23471087891285,-1.18408446699519,-1.15440822229045,
-1.14752545855638,-1.14350309474887,-1.14001606076846,-1.1357238828875,
-1.12736564754565,-1.11667832001598,-1.09123282933259,-1.03282421715994,
-1.02230211225346,-1.01889285046758,-1.01676943157181,-1.01475474381244,
-1.01185869077247,-1.00435281590645,-0.993047045034347,-0.921226724243941,
-0.901629043921063,-0.895498994096946,-0.891680537389021,-0.88815580386089,
-0.883513966692085,-0.873323885144974,-0.85952679965963,-0.820934356568901,
-0.77612425276344,-0.769792771707386,-0.767278517724604,-0.765445912756933,
-0.763400964174954,-0.760352419423677,-0.751777995489701,-0.738201410154419,
-0.708411151081063,-0.656992866968003,-0.647044412847752,-0.642495912023615,
-0.638973390578904,-0.635148189088157,-0.628987059927146,-0.606928996177307,
-0.564005236263803,-0.525209872388838,-0.518760239326155,-0.516226278789947,
-0.514388705649824,-0.51234955444375,-0.509328995058965,-0.500959168860953,
-0.487830863114414,-0.450355188759478,-0.401848694733782,-0.395166042683844,
-0.390842015027932,-0.387353197742139,-0.383355286908634,-0.376400370451799,
-0.342298167552213,-0.28878119060417,-0.270267835775364,-0.266199440051551,
-0.263906847897739,-0.261983190249551,-0.259522377970279,-0.25678391564395,
-0.252219111522213,-0.242660989339562,-0.213242927003015,-0.154177680014348,
-0.145576792461579,-0.14118282947613,-0.137917405760792,-0.134337693350936,
-0.129362939181372,-0.117205649688445,-0.0997761726508418,-0.0900570484866832),
 .UNSPECIFIED.);
#404=B_SPLINE_CURVE_WITH_KNOTS('',3,(#31474,#31475,#31476,#31477,#31478,
#31479,#31480,#31481,#31482,#31483,#31484,#31485,#31486,#31487,#31488,#31489,
#31490,#31491,#31492,#31493,#31494,#31495,#31496,#31497,#31498,#31499,#31500,
#31501,#31502,#31503,#31504,#31505,#31506,#31507,#31508,#31509,#31510,#31511,
#31512,#31513,#31514,#31515,#31516,#31517,#31518,#31519,#31520,#31521,#31522,
#31523,#31524,#31525,#31526,#31527,#31528,#31529,#31530,#31531,#31532,#31533,
#31534,#31535,#31536,#31537,#31538,#31539,#31540,#31541,#31542,#31543,#31544,
#31545,#31546,#31547,#31548,#31549,#31550,#31551,#31552,#31553,#31554,#31555,
#31556,#31557,#31558,#31559,#31560,#31561,#31562,#31563,#31564,#31565,#31566,
#31567,#31568,#31569,#31570,#31571,#31572,#31573,#31574,#31575,#31576,#31577,
#31578,#31579,#31580,#31581,#31582,#31583,#31584,#31585,#31586,#31587,#31588,
#31589,#31590,#31591,#31592,#31593,#31594,#31595,#31596,#31597,#31598,#31599,
#31600,#31601,#31602,#31603,#31604,#31605,#31606,#31607,#31608,#31609,#31610,
#31611,#31612,#31613,#31614,#31615,#31616,#31617,#31618,#31619,#31620,#31621,
#31622,#31623,#31624,#31625,#31626,#31627,#31628,#31629,#31630,#31631,#31632,
#31633,#31634,#31635,#31636,#31637,#31638,#31639,#31640,#31641,#31642,#31643,
#31644,#31645,#31646,#31647,#31648,#31649,#31650,#31651,#31652,#31653,#31654,
#31655,#31656,#31657),.UNSPECIFIED.,.F.,.F.,(4,3,3,3,3,3,3,3,3,3,3,3,3,
3,3,3,3,3,3,3,3,3,3,3,3,3,3,3,3,3,3,3,3,3,3,3,3,3,3,3,3,3,3,3,3,3,3,3,3,
3,3,3,3,3,3,3,3,3,3,3,3,4),(83.3443274880435,83.4447291342008,83.5453184679384,
83.5851403383034,83.6841994558881,83.7831181301476,83.88275355548,83.9814955568309,
84.0802050835808,84.1789119215326,84.2792343243512,84.3780829177117,84.4791422252593,
84.580201532807,84.6792606503917,84.7781793246512,84.8778147499837,84.9765567513346,
85.0752662780845,85.1739731160364,85.2742955188549,85.3731441122155,85.474203419763,
85.5752627273106,85.6743218448953,85.7732405191548,85.8728759444872,85.9716179458382,
86.0703274725881,86.1690343105399,86.2693567133585,86.3682053067192,86.4692646142667,
86.5703239218142,86.6693830393988,86.7683017136584,86.8679371389908,86.9666791403416,
87.0653886670914,87.1640955050431,87.2644179078617,87.3632665012221,87.4643258087699,
87.5653851163178,87.6644442339022,87.7633629081615,87.862998333494,87.9617403348446,
88.0604498615943,88.1591566995457,88.2594791023646,88.3583276957249,88.4593870032732,
88.5604463108214,88.6586782050377,88.7567801508771,88.8547831364347,88.952718035666,
89.0506354266354,89.1485438993612,89.2465050935532,89.2741574414912),
 .UNSPECIFIED.);
#405=B_SPLINE_CURVE_WITH_KNOTS('',3,(#31658,#31659,#31660,#31661,#31662,
#31663,#31664,#31665,#31666,#31667,#31668,#31669,#31670),.UNSPECIFIED.,
 .F.,.F.,(4,3,3,3,4),(89.2741574417072,89.3952590898502,89.5183032212342,
89.555507505325,89.6284739524251),.UNSPECIFIED.);
#406=B_SPLINE_CURVE_WITH_KNOTS('',3,(#31672,#31673,#31674,#31675,#31676,
#31677,#31678,#31679,#31680,#31681,#31682,#31683,#31684,#31685,#31686,#31687,
#31688,#31689),.UNSPECIFIED.,.F.,.F.,(4,2,2,2,2,2,2,2,4),(-0.0900570484866832,
-0.0300743745962655,-0.0180942513927445,-0.0145216738161618,-0.0123622070809486,
-0.0104875353781127,-0.0085158896592708,-0.00500391853466027,-0.00073464173219576),
 .UNSPECIFIED.);
#407=B_SPLINE_CURVE_WITH_KNOTS('',3,(#31690,#31691,#31692,#31693,#31694,
#31695,#31696,#31697,#31698,#31699,#31700,#31701,#31702,#31703,#31704,#31705,
#31706,#31707,#31708,#31709,#31710,#31711,#31712,#31713,#31714,#31715,#31716,
#31717,#31718,#31719,#31720,#31721,#31722,#31723,#31724,#31725,#31726,#31727,
#31728,#31729,#31730,#31731,#31732,#31733,#31734,#31735,#31736,#31737,#31738,
#31739,#31740,#31741,#31742,#31743,#31744,#31745,#31746,#31747,#31748,#31749,
#31750,#31751,#31752,#31753,#31754,#31755,#31756,#31757,#31758,#31759,#31760,
#31761,#31762,#31763,#31764,#31765,#31766,#31767,#31768,#31769,#31770,#31771,
#31772,#31773,#31774,#31775,#31776,#31777,#31778,#31779,#31780,#31781,#31782,
#31783,#31784,#31785,#31786,#31787,#31788,#31789,#31790,#31791,#31792,#31793,
#31794,#31795,#31796,#31797,#31798,#31799,#31800,#31801,#31802,#31803,#31804,
#31805,#31806,#31807,#31808,#31809,#31810,#31811,#31812,#31813,#31814,#31815,
#31816,#31817,#31818,#31819,#31820,#31821,#31822,#31823,#31824,#31825,#31826,
#31827,#31828,#31829,#31830,#31831,#31832,#31833,#31834,#31835,#31836,#31837,
#31838,#31839,#31840,#31841,#31842,#31843,#31844,#31845,#31846,#31847,#31848,
#31849,#31850,#31851,#31852,#31853,#31854,#31855,#31856,#31857,#31858,#31859,
#31860,#31861,#31862,#31863,#31864,#31865,#31866,#31867,#31868,#31869,#31870,
#31871,#31872,#31873,#31874,#31875,#31876,#31877,#31878,#31879,#31880,#31881,
#31882,#31883,#31884,#31885,#31886,#31887,#31888,#31889,#31890,#31891,#31892,
#31893,#31894,#31895,#31896,#31897,#31898,#31899,#31900,#31901,#31902,#31903,
#31904,#31905,#31906,#31907,#31908,#31909),.UNSPECIFIED.,.F.,.F.,(4,2,2,
2,2,2,2,2,2,2,2,2,2,2,2,2,2,2,2,2,2,2,2,2,2,2,2,2,2,2,2,2,2,2,2,2,2,2,2,
2,2,2,2,2,2,2,2,2,2,2,2,2,2,2,2,2,2,2,2,2,2,2,2,2,2,2,2,2,2,2,2,2,2,2,2,
2,2,2,2,2,2,2,2,2,2,2,2,2,2,2,2,2,2,2,2,2,2,2,2,2,2,2,2,2,2,2,2,2,2,4),
(-3.17296637197709,-3.13078746919988,-3.0925286644018,-3.0695906434777,
-3.06335111484647,-3.0595079607854,-3.05598922374801,-3.05147385451278,
-3.0417129483066,-2.98561694806597,-2.95420895217546,-2.94428148541909,
-2.93959386722636,-2.93680582930531,-2.93435532750786,-2.93434349414453,
-2.93433151630648,-2.93431938943293,-2.93430710881415,-2.93429466956216,
-2.93428206659688,-2.9342692946296,-2.93425634818182,-2.93424322154498,
-2.93422990875741,-2.93421640363605,-2.93420269972696,-2.93418879031003,
-2.93228208241657,-2.92997144626731,-2.92582524274472,-2.90605137058816,
-2.85385911403481,-2.81974157680881,-2.81278384511443,-2.80878448979208,
-2.80529451940085,-2.80096920112055,-2.79428488068219,-2.74575956037338,
-2.70825470123193,-2.6951685751157,-2.68681667134174,-2.68379799411075,
-2.68175875606987,-2.67992004905516,-2.67738315897735,-2.67091881198376,
-2.6322882637127,-2.59602562765379,-2.56796164317022,-2.56133965675876,
-2.55741315550891,-2.55391338865715,-2.54947758509592,-2.54039555090182,
-2.47692937905085,-2.43981823134715,-2.43442438368728,-2.43188589670098,
-2.42992391273856,-2.42762864129485,-2.42355053547913,-2.40489238177681,
-2.35145350166597,-2.31734295794089,-2.31038555351585,-2.30638626893895,
-2.30289629153778,-2.29857087551525,-2.29188623289546,-2.24325844439625,
-2.20598393968121,-2.19281836607498,-2.18442992384185,-2.18140619833199,
-2.17936592317891,-2.17752814189548,-2.17499489180802,-2.16855252078573,
-2.12928902664488,-2.07311645703369,-2.06174160674081,-2.05689341140303,
-2.05333524928393,-2.04959430980873,-2.04382580005754,-2.02725785281374,
-1.97075000790547,-1.93599678355961,-1.93149930624142,-1.92913949463042,
-1.9271829674771,-1.92472774704299,-1.92084669559392,-1.89904951802421,
-1.85287952211509,-1.82784062804831,-1.81726477658645,-1.80897527249778,
-1.80469648362572,-1.80120960724638,-1.79717544842081,-1.79024279660622,
-1.75968796282355,-1.70942068280025,-1.68441845478752,-1.68017082479052,
-1.67786370871181,-1.67616180579166),.UNSPECIFIED.);
#408=B_SPLINE_CURVE_WITH_KNOTS('',3,(#31915,#31916,#31917,#31918,#31919,
#31920,#31921,#31922,#31923,#31924,#31925,#31926,#31927,#31928,#31929,#31930,
#31931,#31932,#31933,#31934,#31935,#31936,#31937,#31938,#31939,#31940,#31941,
#31942,#31943,#31944,#31945,#31946,#31947,#31948,#31949,#31950,#31951,#31952,
#31953,#31954,#31955,#31956,#31957,#31958,#31959,#31960,#31961,#31962,#31963,
#31964,#31965,#31966,#31967,#31968,#31969,#31970,#31971,#31972,#31973,#31974,
#31975,#31976,#31977,#31978,#31979,#31980,#31981,#31982,#31983,#31984,#31985,
#31986,#31987,#31988,#31989,#31990,#31991,#31992,#31993,#31994,#31995,#31996,
#31997,#31998,#31999,#32000,#32001,#32002,#32003,#32004,#32005,#32006,#32007,
#32008,#32009,#32010,#32011,#32012,#32013,#32014,#32015,#32016,#32017,#32018,
#32019,#32020,#32021,#32022,#32023,#32024,#32025,#32026,#32027,#32028,#32029,
#32030,#32031,#32032,#32033,#32034,#32035,#32036,#32037,#32038,#32039,#32040,
#32041,#32042,#32043,#32044,#32045,#32046,#32047,#32048,#32049,#32050,#32051,
#32052,#32053,#32054,#32055,#32056,#32057,#32058,#32059,#32060,#32061,#32062,
#32063,#32064,#32065,#32066,#32067,#32068,#32069,#32070,#32071,#32072,#32073,
#32074,#32075,#32076,#32077,#32078,#32079,#32080,#32081,#32082,#32083,#32084,
#32085,#32086,#32087,#32088,#32089,#32090,#32091,#32092,#32093,#32094,#32095),
 .UNSPECIFIED.,.F.,.F.,(4,3,3,3,3,3,3,3,3,3,3,3,3,3,3,3,3,3,3,3,3,3,3,3,
3,3,3,3,3,3,3,3,3,3,3,3,3,3,3,3,3,3,3,3,3,3,3,3,3,3,3,3,3,3,3,3,3,3,3,3,
4),(77.0622185302826,77.159800081767,77.2573831119389,77.3550617349471,
77.4527912027954,77.5506849731481,77.6147731712817,77.7138322888664,77.8127509631257,
77.9123863884582,78.0111283898091,78.109837916559,78.2085447545109,78.3088671573295,
78.4077157506899,78.5087750582376,78.6098343657853,78.7088934833699,78.8078121576293,
78.9074475829618,79.0061895843126,79.1048991110625,79.2036059490143,79.3039283518329,
79.4027769451934,79.5038362527411,79.6048955602889,79.7039546778735,79.8028733521328,
79.9025087774653,80.0012507788162,80.0999603055662,80.1986671435177,80.2989895463364,
80.3978381396968,80.4988974472446,80.5999567547925,80.6990158723772,80.7979345466366,
80.8975699719691,80.9963119733199,81.0950215000699,81.1937283380219,81.2940507408404,
81.3928993342009,81.4939586417485,81.5950179492961,81.6940770668809,81.79299574114,
81.8926311664725,81.9913731678234,82.0900826945733,82.1887895325252,82.2891119353438,
82.3879605287044,82.4890198362521,82.5900791437998,82.6998271120124,82.8092455102998,
82.9180995588121,82.990972133972),.UNSPECIFIED.);
#409=B_SPLINE_CURVE_WITH_KNOTS('',3,(#32096,#32097,#32098,#32099,#32100,
#32101,#32102,#32103,#32104,#32105,#32106,#32107,#32108),.UNSPECIFIED.,
 .F.,.F.,(4,3,3,3,4),(82.9909721343116,83.0910899849471,83.1912299180565,
83.2914717478673,83.3443274880435),.UNSPECIFIED.);
#410=B_SPLINE_CURVE_WITH_KNOTS('',3,(#32109,#32110,#32111,#32112,#32113,
#32114,#32115,#32116,#32117,#32118,#32119,#32120,#32121,#32122,#32123,#32124,
#32125,#32126,#32127,#32128,#32129,#32130,#32131,#32132,#32133,#32134,#32135,
#32136,#32137,#32138,#32139,#32140,#32141,#32142,#32143,#32144,#32145,#32146,
#32147,#32148,#32149,#32150,#32151,#32152,#32153,#32154,#32155,#32156,#32157,
#32158,#32159,#32160,#32161,#32162,#32163,#32164,#32165,#32166,#32167,#32168,
#32169,#32170,#32171,#32172,#32173,#32174,#32175,#32176,#32177,#32178,#32179,
#32180,#32181,#32182,#32183,#32184,#32185,#32186,#32187,#32188,#32189,#32190,
#32191,#32192,#32193,#32194,#32195,#32196,#32197,#32198,#32199,#32200,#32201,
#32202,#32203,#32204,#32205,#32206,#32207,#32208,#32209,#32210,#32211,#32212,
#32213,#32214,#32215,#32216,#32217,#32218,#32219,#32220,#32221,#32222,#32223,
#32224,#32225,#32226,#32227,#32228,#32229,#32230,#32231,#32232,#32233,#32234,
#32235,#32236,#32237,#32238,#32239,#32240,#32241,#32242,#32243,#32244,#32245,
#32246,#32247,#32248,#32249,#32250,#32251,#32252,#32253,#32254,#32255,#32256,
#32257,#32258,#32259,#32260,#32261,#32262,#32263,#32264,#32265,#32266,#32267,
#32268,#32269,#32270,#32271,#32272,#32273,#32274,#32275,#32276,#32277,#32278,
#32279,#32280,#32281,#32282,#32283,#32284,#32285,#32286,#32287,#32288,#32289,
#32290,#32291,#32292,#32293,#32294,#32295,#32296,#32297,#32298,#32299,#32300,
#32301,#32302,#32303,#32304,#32305,#32306,#32307,#32308,#32309,#32310,#32311,
#32312,#32313,#32314,#32315,#32316,#32317,#32318,#32319,#32320,#32321,#32322,
#32323,#32324,#32325,#32326,#32327,#32328,#32329,#32330,#32331,#32332,#32333,
#32334,#32335,#32336,#32337,#32338,#32339,#32340,#32341,#32342),
 .UNSPECIFIED.,.F.,.F.,(4,2,2,2,2,2,2,2,2,2,2,2,2,2,2,2,2,2,2,2,2,2,2,2,
2,2,2,2,2,2,2,2,2,2,2,2,2,2,2,2,2,2,2,2,2,2,2,2,2,2,2,2,2,2,2,2,2,2,2,2,
2,2,2,2,2,2,2,2,2,2,2,2,2,2,2,2,2,2,2,2,2,2,2,2,2,2,2,2,2,2,2,2,2,2,2,2,
2,2,2,2,2,2,2,2,2,2,2,2,2,2,2,2,2,2,2,2,4),(-1.67616180579166,-1.67590324059147,
-1.67338170220638,-1.66927931773268,-1.63900712545492,-1.58695747241575,
-1.5630710905474,-1.55650970438415,-1.55259648265019,-1.54909445605647,
-1.54463652286485,-1.5354391752262,-1.50000443508411,-1.4450906792585,-1.43219539103183,
-1.42852504090574,-1.42634360912866,-1.42435545860539,-1.42161169852704,
-1.41506611382747,-1.40565769974616,-1.37702624774906,-1.31670134210244,
-1.30726514297897,-1.30276169796662,-1.29925447831602,-1.29536676792491,
-1.28892233960465,-1.26340720815674,-1.20490588541381,-1.18218710761623,
-1.17826903002877,-1.17580260541207,-1.17384558215083,-1.17149529857281,
-1.16704348282125,-1.1347874113362,-1.08477727224885,-1.06070206024459,
-1.05412593336901,-1.05020949460017,-1.0467080581074,-1.04225562170707,
-1.03308691244677,-0.997876251810065,-0.942777711211275,-0.929810669456865,
-0.926133595562848,-0.923950674736683,-0.921963058706431,-0.919222669962956,
-0.912697241400724,-0.880402724237487,-0.82225357056646,-0.807401858428773,
-0.801866291913438,-0.798543681397679,-0.795003477859689,-0.790264614188273,
-0.779531050021669,-0.764763543817644,-0.721045767084842,-0.706929024066574,
-0.680115484606524,-0.676048880761138,-0.673538033476851,-0.671578459373667,
-0.669263673327676,-0.664979672206178,-0.638947608603592,-0.586888922367753,
-0.558886681525968,-0.552107329240199,-0.548108164150461,-0.544618561544081,
-0.540293960443175,-0.531775997788042,-0.520827702395861,-0.494420521592979,
-0.457967415154464,-0.429013006457582,-0.424933936310385,-0.422419463944681,
-0.420459738043952,-0.418147924234948,-0.413877461091165,-0.388232119442468,
-0.337345190076549,-0.307934774758003,-0.301067016493568,-0.297047910273152,
-0.293560378716109,-0.293517093482187,-0.293476237509801,-0.293437665027781,
-0.29340123983713,-0.293366834616729,-0.293334330293681,-0.29330361545272,
-0.293274585787413,-0.293247143603894,-0.29322119736386,-0.29319666124197,
-0.288971835318852,-0.280285996621542,-0.26895192213428,-0.241080750136327,
-0.206362284970749,-0.177891574683012,-0.173820872606083,-0.171308973212394,
-0.169349551514988,-0.167036092461159,-0.162757477725552,-0.136870408833084,
-0.0972604102131988,-0.0902219335216519),.UNSPECIFIED.);
#411=B_SPLINE_CURVE_WITH_KNOTS('',3,(#32348,#32349,#32350,#32351,#32352,
#32353,#32354,#32355,#32356,#32357,#32358,#32359,#32360,#32361,#32362,#32363,
#32364,#32365,#32366,#32367,#32368,#32369,#32370,#32371,#32372,#32373,#32374,
#32375,#32376,#32377,#32378,#32379,#32380,#32381,#32382,#32383,#32384,#32385,
#32386,#32387,#32388,#32389,#32390,#32391,#32392,#32393,#32394,#32395,#32396,
#32397,#32398,#32399,#32400,#32401,#32402,#32403,#32404,#32405,#32406,#32407,
#32408,#32409,#32410,#32411,#32412,#32413,#32414,#32415,#32416,#32417,#32418,
#32419,#32420,#32421,#32422,#32423,#32424,#32425,#32426,#32427,#32428,#32429,
#32430,#32431,#32432,#32433,#32434,#32435,#32436,#32437,#32438,#32439,#32440,
#32441,#32442,#32443,#32444,#32445,#32446,#32447,#32448,#32449,#32450,#32451,
#32452,#32453,#32454,#32455,#32456,#32457,#32458,#32459,#32460,#32461,#32462,
#32463,#32464,#32465,#32466,#32467,#32468,#32469,#32470,#32471,#32472,#32473,
#32474,#32475,#32476,#32477,#32478,#32479,#32480,#32481,#32482,#32483,#32484,
#32485,#32486,#32487,#32488,#32489,#32490,#32491,#32492,#32493,#32494,#32495,
#32496,#32497,#32498,#32499,#32500,#32501,#32502,#32503,#32504,#32505,#32506,
#32507,#32508,#32509,#32510,#32511,#32512,#32513,#32514,#32515,#32516,#32517,
#32518,#32519,#32520,#32521,#32522,#32523,#32524,#32525,#32526,#32527,#32528),
 .UNSPECIFIED.,.F.,.F.,(4,3,3,3,3,3,3,3,3,3,3,3,3,3,3,3,3,3,3,3,3,3,3,3,
3,3,3,3,3,3,3,3,3,3,3,3,3,3,3,3,3,3,3,3,3,3,3,3,3,3,3,3,3,3,3,3,3,3,3,3,
4),(70.779075450487,70.8779573340721,70.976739703664,71.0754687734666,71.174174353704,
71.2728862237033,71.3716999427462,71.4705663306546,71.5696036128791,71.64440600426,
71.7434651218446,71.842383796104,71.9420192214365,72.0407612227874,72.1394707495373,
72.238177587489,72.3384999903077,72.4373485836681,72.5384078912159,72.6394671987636,
72.7385263163483,72.8374449906077,72.9370804159402,73.035822417291,73.134531944041,
73.2332387819928,73.3335611848114,73.4324097781719,73.5334690857196,73.6345283932673,
73.7335875108519,73.8325061851114,73.9321416104438,74.0308836117947,74.1295931385446,
74.2282999764964,74.328622379315,74.4274709726755,74.5285302802232,74.6295895877709,
74.7286487053555,74.827567379615,74.9272028049474,75.0259448062983,75.1246543330482,
75.223361171,75.3236835738186,75.4225321671791,75.5235914747268,75.6246507822745,
75.7237098998592,75.8226285741186,75.9222639994511,76.0210060008019,76.1197155275519,
76.2184223655036,76.3187447683222,76.4175933616827,76.5186526692304,76.6197119767781,
76.707786827132),.UNSPECIFIED.);
#412=B_SPLINE_CURVE_WITH_KNOTS('',3,(#32529,#32530,#32531,#32532,#32533,
#32534,#32535,#32536,#32537,#32538,#32539,#32540,#32541),.UNSPECIFIED.,
 .F.,.F.,(4,3,3,3,4),(76.7077868273942,76.8056326709673,76.9033659624181,
77.0010095032294,77.0622185302826),.UNSPECIFIED.);
#413=B_SPLINE_CURVE_WITH_KNOTS('',3,(#32543,#32544,#32545,#32546,#32547,
#32548,#32549,#32550,#32551,#32552,#32553,#32554,#32555,#32556,#32557,#32558,
#32559,#32560,#32561,#32562),.UNSPECIFIED.,.F.,.F.,(4,2,2,2,2,2,2,2,2,4),
(-0.0902219335216519,-0.0726583194898945,-0.0548807383335625,-0.0489604234752576,
-0.0451871616823215,-0.0416448559837934,-0.0381656831375037,-0.0335591450836605,
-0.0219875622138333,-0.000734571677354467),.UNSPECIFIED.);
#414=B_SPLINE_CURVE_WITH_KNOTS('',3,(#32563,#32564,#32565,#32566,#32567,
#32568,#32569,#32570,#32571,#32572,#32573,#32574,#32575,#32576,#32577,#32578,
#32579,#32580,#32581,#32582,#32583,#32584,#32585,#32586,#32587,#32588,#32589,
#32590,#32591,#32592,#32593,#32594,#32595,#32596,#32597,#32598,#32599,#32600,
#32601,#32602,#32603,#32604,#32605,#32606,#32607,#32608,#32609,#32610,#32611,
#32612,#32613,#32614,#32615,#32616,#32617,#32618,#32619,#32620,#32621,#32622,
#32623,#32624,#32625,#32626,#32627,#32628,#32629,#32630,#32631,#32632,#32633,
#32634,#32635,#32636,#32637,#32638,#32639,#32640,#32641,#32642,#32643,#32644,
#32645,#32646,#32647,#32648,#32649,#32650,#32651,#32652,#32653,#32654,#32655,
#32656,#32657,#32658,#32659,#32660,#32661,#32662,#32663,#32664,#32665,#32666,
#32667,#32668,#32669,#32670,#32671,#32672,#32673,#32674,#32675,#32676,#32677,
#32678,#32679,#32680,#32681,#32682,#32683,#32684,#32685,#32686,#32687,#32688,
#32689,#32690,#32691,#32692,#32693,#32694,#32695,#32696,#32697,#32698,#32699,
#32700,#32701,#32702,#32703,#32704,#32705,#32706,#32707,#32708,#32709,#32710,
#32711,#32712,#32713,#32714,#32715,#32716,#32717,#32718,#32719,#32720,#32721,
#32722,#32723,#32724,#32725,#32726,#32727,#32728,#32729,#32730,#32731,#32732,
#32733,#32734,#32735,#32736,#32737,#32738,#32739,#32740,#32741,#32742,#32743,
#32744,#32745,#32746,#32747,#32748,#32749,#32750,#32751,#32752,#32753,#32754,
#32755,#32756,#32757,#32758,#32759,#32760,#32761,#32762,#32763,#32764,#32765,
#32766,#32767,#32768,#32769,#32770),.UNSPECIFIED.,.F.,.F.,(4,2,2,2,2,2,
2,2,2,2,2,2,2,2,2,2,2,2,2,2,2,2,2,2,2,2,2,2,2,2,2,2,2,2,2,2,2,2,2,2,2,2,
2,2,2,2,2,2,2,2,2,2,2,2,2,2,2,2,2,2,2,2,2,2,2,2,2,2,2,2,2,2,2,2,2,2,2,2,
2,2,2,2,2,2,2,2,2,2,2,2,2,2,2,2,2,2,2,2,2,2,2,2,2,4),(-3.17255687017752,
-3.12637703617202,-3.10731238378642,-3.09645286141489,-3.09312618082806,
-3.09102078364667,-3.08901797848521,-3.08654893600502,-3.08048399926583,
-3.03015395700328,-2.99518292861147,-2.98214811192475,-2.9724776644585,
-2.9680745089668,-2.9647436284611,-2.96100286704291,-2.95523478465193,-2.93866917271469,
-2.87509434693847,-2.85609132604166,-2.84880636641023,-2.84342110699485,
-2.84088437453105,-2.83892268500488,-2.8366265188053,-2.83254396436203,
-2.8138052891689,-2.77081297205662,-2.73093660955173,-2.72119675699531,
-2.71663647969869,-2.71312220255679,-2.70926402702509,-2.7029547969899,
-2.68173202399022,-2.62335191115039,-2.59593027505255,-2.59160157084977,
-2.58927722486086,-2.58731842144972,-2.58481987107659,-2.5807946572808,
-2.55503861369596,-2.54153489467532,-2.49643847865547,-2.4737917097306,
-2.46757733058487,-2.46373972940524,-2.46021950234468,-2.45569308688616,
-2.44587120514403,-2.39099050241885,-2.34647231815942,-2.34106477153636,
-2.33852372765471,-2.33656156666864,-2.33426818511227,-2.33019826053288,
-2.31164778324914,-2.30244987001193,-2.29051103749268,-2.26115855679399,
-2.23661142484505,-2.22617192208892,-2.21796631126521,-2.2137043849023,
-2.21055472614897,-2.20662640323419,-2.19999664637356,-2.17520900703381,
-2.12033477075688,-2.10217056605457,-2.09509763809575,-2.08983378484832,
-2.08732012688649,-2.08536012178259,-2.08304690234235,-2.07888935945493,
-2.05881144511315,-1.99213472436227,-1.97817395567435,-1.9678916226495,
-1.96323242059507,-1.95970436939832,-1.95635822076576,-1.95069862832457,
-1.93496910985383,-1.87042844786639,-1.85135140988253,-1.84404783533786,
-1.83865190141036,-1.8361130709971,-1.83415111741865,-1.83185622657302,
-1.82777959190046,-1.80914482675449,-1.75568531757039,-1.72157350370027,
-1.71461622657685,-1.71061705644185,-1.70712720307786,-1.70280197209477,
-1.6961176756079,-1.67598768218192),.UNSPECIFIED.);
#415=B_SPLINE_CURVE_WITH_KNOTS('',3,(#32776,#32777,#32778,#32779,#32780,
#32781,#32782,#32783,#32784,#32785,#32786,#32787,#32788,#32789,#32790,#32791,
#32792,#32793,#32794,#32795,#32796,#32797,#32798,#32799,#32800,#32801,#32802,
#32803,#32804,#32805,#32806,#32807,#32808,#32809,#32810,#32811,#32812,#32813,
#32814,#32815,#32816,#32817,#32818,#32819,#32820,#32821,#32822,#32823,#32824,
#32825,#32826,#32827,#32828,#32829,#32830,#32831,#32832,#32833,#32834,#32835,
#32836,#32837,#32838,#32839,#32840,#32841,#32842,#32843,#32844,#32845,#32846,
#32847,#32848,#32849,#32850,#32851,#32852,#32853,#32854,#32855,#32856,#32857,
#32858,#32859,#32860,#32861,#32862,#32863,#32864,#32865,#32866,#32867,#32868,
#32869,#32870,#32871,#32872,#32873,#32874,#32875,#32876,#32877,#32878,#32879,
#32880,#32881,#32882,#32883,#32884,#32885,#32886,#32887,#32888,#32889,#32890,
#32891,#32892,#32893,#32894,#32895,#32896,#32897,#32898,#32899,#32900,#32901,
#32902,#32903,#32904,#32905,#32906,#32907,#32908,#32909,#32910,#32911,#32912,
#32913,#32914,#32915,#32916,#32917,#32918,#32919,#32920,#32921,#32922,#32923,
#32924,#32925,#32926,#32927,#32928,#32929,#32930,#32931,#32932,#32933,#32934,
#32935,#32936,#32937,#32938,#32939,#32940,#32941,#32942,#32943,#32944,#32945,
#32946,#32947,#32948,#32949,#32950,#32951,#32952,#32953,#32954,#32955,#32956),
 .UNSPECIFIED.,.F.,.F.,(4,3,3,3,3,3,3,3,3,3,3,3,3,3,3,3,3,3,3,3,3,3,3,3,
3,3,3,3,3,3,3,3,3,3,3,3,3,3,3,3,3,3,3,3,3,3,3,3,3,3,3,3,3,3,3,3,3,3,3,3,
4),(64.4947309352028,64.5971327257698,64.6789776427347,64.7780367603194,
64.8769554345788,64.9765908599112,65.0753328612621,65.1740423880121,65.2727492259639,
65.3730716287825,65.4719202221431,65.5729795296907,65.6740388372384,65.7730979548231,
65.8720166290824,65.9716520544149,66.0703940557658,66.1691035825158,66.2678104204676,
66.3681328232862,66.4669814166466,66.5680407241943,66.669100031742,66.7681591493266,
66.8670778235863,66.9667132489188,67.0654552502696,67.1641647770196,67.2628716149713,
67.3631940177899,67.4620426111503,67.563101918698,67.6641612262456,67.7632203438303,
67.8621390180898,67.9617744434222,68.0605164447731,68.1592259715233,68.2579328094751,
68.3582552122936,68.4571038056543,68.5581631132017,68.6592224207492,68.7582815383338,
68.8572002125931,68.9568356379256,69.0555776392765,69.1542871660265,69.2529940039784,
69.353316406797,69.4521650001575,69.5532243077052,69.6542836152528,69.7520048359883,
69.8496009043764,69.9471033152912,70.0445434457332,70.1419872142465,70.2394270962248,
70.3369604616551,70.4246015195609),.UNSPECIFIED.);
#416=B_SPLINE_CURVE_WITH_KNOTS('',3,(#32957,#32958,#32959,#32960,#32961,
#32962,#32963,#32964,#32965,#32966,#32967,#32968,#32969),.UNSPECIFIED.,
 .F.,.F.,(4,3,3,3,4),(70.4246015199524,70.5582169253846,70.6493448097564,
70.7484011690592,70.779075450487),.UNSPECIFIED.);
#417=B_SPLINE_CURVE_WITH_KNOTS('',3,(#32970,#32971,#32972,#32973,#32974,
#32975,#32976,#32977,#32978,#32979,#32980,#32981,#32982,#32983,#32984,#32985,
#32986,#32987,#32988,#32989,#32990,#32991,#32992,#32993,#32994,#32995,#32996,
#32997,#32998,#32999,#33000,#33001,#33002,#33003,#33004,#33005,#33006,#33007,
#33008,#33009,#33010,#33011,#33012,#33013,#33014,#33015,#33016,#33017,#33018,
#33019,#33020,#33021,#33022,#33023,#33024,#33025,#33026,#33027,#33028,#33029,
#33030,#33031,#33032,#33033,#33034,#33035,#33036,#33037,#33038,#33039,#33040,
#33041,#33042,#33043,#33044,#33045,#33046,#33047,#33048,#33049,#33050,#33051,
#33052,#33053,#33054,#33055,#33056,#33057,#33058,#33059,#33060,#33061,#33062,
#33063,#33064,#33065,#33066,#33067,#33068,#33069,#33070,#33071,#33072,#33073,
#33074,#33075,#33076,#33077,#33078,#33079,#33080,#33081,#33082,#33083,#33084,
#33085,#33086,#33087,#33088,#33089,#33090,#33091,#33092,#33093,#33094,#33095,
#33096,#33097,#33098,#33099,#33100,#33101,#33102,#33103,#33104,#33105,#33106,
#33107,#33108,#33109,#33110,#33111,#33112,#33113,#33114,#33115,#33116,#33117,
#33118,#33119,#33120,#33121,#33122,#33123,#33124,#33125,#33126,#33127,#33128,
#33129,#33130,#33131,#33132,#33133,#33134,#33135,#33136,#33137,#33138,#33139,
#33140,#33141,#33142,#33143,#33144,#33145,#33146,#33147,#33148,#33149,#33150,
#33151,#33152,#33153,#33154,#33155,#33156,#33157,#33158,#33159,#33160,#33161,
#33162,#33163,#33164,#33165,#33166,#33167,#33168,#33169,#33170,#33171,#33172,
#33173,#33174,#33175,#33176,#33177,#33178,#33179,#33180,#33181,#33182,#33183,
#33184,#33185,#33186,#33187,#33188,#33189,#33190,#33191),.UNSPECIFIED.,
 .F.,.F.,(4,2,2,2,2,2,2,2,2,2,2,2,2,2,2,2,2,2,2,2,2,2,2,2,2,2,2,2,2,2,2,
2,2,2,2,2,2,2,2,2,2,2,2,2,2,2,2,2,2,2,2,2,2,2,2,2,2,2,2,2,2,2,2,2,2,2,2,
2,2,2,2,2,2,2,2,2,2,2,2,2,2,2,2,2,2,2,2,2,2,2,2,2,2,2,2,2,2,2,2,2,2,2,2,
2,2,2,2,2,2,2,4),(-1.67598768218192,-1.64781802973257,-1.61129200490768,
-1.59068631767884,-1.58662859151187,-1.58436231468612,-1.58259340344101,
-1.58012109046356,-1.57506885255693,-1.56835983506212,-1.55158797940551,
-1.50156219162751,-1.49928274739267,-1.47034641909263,-1.46350659234859,
-1.45949352857199,-1.4560050068863,-1.45169875058855,-1.44327302165624,
-1.3950818856265,-1.34262895883037,-1.33667164920921,-1.33425237643543,
-1.33226221628564,-1.33013538111098,-1.32671169469097,-1.31492668526521,
-1.293349568365,-1.28016256034407,-1.22378661028309,-1.21403922495425,-1.20952648862046,
-1.20600830713213,-1.20216424306298,-1.19591980341672,-1.17291949412122,
-1.1324594421586,-1.09230875019351,-1.08583460035202,-1.08329609004918,
-1.08145702347058,-1.07941838777931,-1.07640228371058,-1.06806842766069,
-1.05501966955518,-1.01745094942914,-0.968879935990084,-0.962195341532359,
-0.957870079997983,-0.954380282063035,-0.950381263816085,-0.943424463195269,
-0.909314139420925,-0.855795355488474,-0.83726055985558,-0.833191864005302,
-0.830898819053043,-0.828936728818177,-0.82639546768346,-0.820986409217987,
-0.813659033888703,-0.7944853757041,-0.729658190600643,-0.714221158355355,
-0.70860348948435,-0.705265450932967,-0.701733752306944,-0.697048982826981,
-0.686622315631573,-0.672406078420063,-0.602405137493447,-0.58578216499317,
-0.581836951263677,-0.579571959272974,-0.57780281332374,-0.575328571867578,
-0.570266685426739,-0.563541200546925,-0.546707599066957,-0.496554966091625,
-0.484131392750421,-0.464145258862735,-0.457971797803325,-0.454143137060589,
-0.450620235454031,-0.44599726963226,-0.435916220811467,-0.422312523715144,
-0.384676579876693,-0.338425674441042,-0.332156138326956,-0.329651907815647,
-0.327821439567445,-0.32577256727383,-0.322707282051559,-0.314012696228027,
-0.300171376462531,-0.235809667458605,-0.213437476766805,-0.207015727125252,
-0.203133119718856,-0.19962503682749,-0.199583845669812,-0.19954628633179,
-0.199511981429396,-0.195123927313244,-0.18594143980428,-0.173719309919359,
-0.142286043005557,-0.0938487373820991,-0.0899211228894936),
 .UNSPECIFIED.);
#418=B_SPLINE_CURVE_WITH_KNOTS('',3,(#33197,#33198,#33199,#33200,#33201,
#33202,#33203,#33204,#33205,#33206,#33207,#33208,#33209,#33210,#33211,#33212,
#33213,#33214,#33215,#33216,#33217,#33218,#33219,#33220,#33221,#33222,#33223,
#33224,#33225,#33226,#33227,#33228,#33229,#33230,#33231,#33232,#33233,#33234,
#33235,#33236,#33237,#33238,#33239,#33240,#33241,#33242,#33243,#33244,#33245,
#33246,#33247,#33248,#33249,#33250,#33251,#33252,#33253,#33254,#33255,#33256,
#33257,#33258,#33259,#33260,#33261,#33262,#33263,#33264,#33265,#33266,#33267,
#33268,#33269,#33270,#33271,#33272,#33273,#33274,#33275,#33276,#33277,#33278,
#33279,#33280,#33281,#33282,#33283,#33284,#33285,#33286,#33287,#33288,#33289,
#33290,#33291,#33292,#33293,#33294,#33295,#33296,#33297,#33298,#33299,#33300,
#33301,#33302,#33303,#33304,#33305,#33306,#33307,#33308,#33309,#33310,#33311,
#33312,#33313,#33314,#33315,#33316,#33317,#33318,#33319,#33320,#33321,#33322,
#33323,#33324,#33325,#33326,#33327,#33328,#33329,#33330,#33331,#33332,#33333,
#33334,#33335,#33336,#33337,#33338,#33339,#33340,#33341,#33342,#33343,#33344,
#33345,#33346,#33347,#33348,#33349,#33350,#33351,#33352,#33353,#33354,#33355,
#33356,#33357,#33358,#33359,#33360,#33361,#33362,#33363,#33364,#33365,#33366,
#33367,#33368,#33369,#33370,#33371,#33372,#33373,#33374,#33375,#33376,#33377),
 .UNSPECIFIED.,.F.,.F.,(4,3,3,3,3,3,3,3,3,3,3,3,3,3,3,3,3,3,3,3,3,3,3,3,
3,3,3,3,3,3,3,3,3,3,3,3,3,3,3,3,3,3,3,3,3,3,3,3,3,3,3,3,3,3,3,3,3,3,3,3,
4),(58.21253113431,58.3098151884965,58.4095140103006,58.5069204673879,58.6077654715505,
58.7086104757131,58.8076695932978,58.9065882675572,59.0062236928896,59.1049656942405,
59.2036752209904,59.3023820589422,59.4027044617608,59.5015530551214,59.602612362669,
59.7036716702167,59.8027307878014,59.9016494620607,60.0012848873931,60.1000268887439,
60.1987364154939,60.2974432534456,60.3977656562643,60.4966142496248,60.5976735571725,
60.6987328647203,60.7977919823049,60.8967106565645,60.9963460818969,61.0950880832477,
61.1937976099976,61.2925044479495,61.3928268507681,61.4916754441286,61.5927347516762,
61.6937940592239,61.7928531768085,61.8917718510678,61.9914072764003,62.0901492777511,
62.188858804501,62.2875656424526,62.3878880452713,62.4867366386318,62.5877959461796,
62.6888552537275,62.787914371312,62.8868330455714,62.9864684709039,63.0852104722547,
63.1839199990046,63.2826268369563,63.382949239775,63.4817978331354,63.5828571406832,
63.6839164482311,63.7900912025854,63.8959105065072,64.0015055025791,64.1067929756915,
64.1414162124316),.UNSPECIFIED.);
#419=B_SPLINE_CURVE_WITH_KNOTS('',3,(#33378,#33379,#33380,#33381,#33382,
#33383,#33384,#33385,#33386,#33387,#33388,#33389,#33390),.UNSPECIFIED.,
 .F.,.F.,(4,3,3,3,4),(64.1414162127729,64.2432632295712,64.3451869470676,
64.4472800358431,64.4947309352028),.UNSPECIFIED.);
#420=B_SPLINE_CURVE_WITH_KNOTS('',3,(#33392,#33393,#33394,#33395,#33396,
#33397,#33398,#33399,#33400,#33401,#33402,#33403,#33404,#33405,#33406,#33407),
 .UNSPECIFIED.,.F.,.F.,(4,2,2,2,2,2,2,4),(-0.0899211228894936,-0.0825382572484242,
-0.0790353552956432,-0.0768911011408069,-0.0748873442578905,-0.0720511616616847,
-0.0649348746284129,-0.00073565181987095),.UNSPECIFIED.);
#421=B_SPLINE_CURVE_WITH_KNOTS('',3,(#33408,#33409,#33410,#33411,#33412,
#33413,#33414,#33415,#33416,#33417,#33418,#33419,#33420,#33421,#33422,#33423,
#33424,#33425,#33426,#33427,#33428,#33429,#33430,#33431,#33432,#33433,#33434,
#33435,#33436,#33437,#33438,#33439,#33440,#33441,#33442,#33443,#33444,#33445,
#33446,#33447,#33448,#33449,#33450,#33451,#33452,#33453,#33454,#33455,#33456,
#33457,#33458,#33459,#33460,#33461,#33462,#33463,#33464,#33465,#33466,#33467,
#33468,#33469,#33470,#33471,#33472,#33473,#33474,#33475,#33476,#33477,#33478,
#33479,#33480,#33481,#33482,#33483,#33484,#33485,#33486,#33487,#33488,#33489,
#33490,#33491,#33492,#33493,#33494,#33495,#33496,#33497,#33498,#33499,#33500,
#33501,#33502,#33503,#33504,#33505,#33506,#33507,#33508,#33509,#33510,#33511,
#33512,#33513,#33514,#33515,#33516,#33517,#33518,#33519,#33520,#33521,#33522,
#33523,#33524,#33525,#33526,#33527,#33528,#33529,#33530,#33531,#33532,#33533,
#33534,#33535,#33536,#33537,#33538,#33539,#33540,#33541,#33542,#33543,#33544,
#33545,#33546,#33547,#33548,#33549,#33550,#33551,#33552,#33553,#33554,#33555,
#33556,#33557,#33558,#33559,#33560,#33561,#33562,#33563,#33564,#33565,#33566,
#33567,#33568,#33569,#33570,#33571,#33572,#33573,#33574,#33575,#33576,#33577,
#33578,#33579,#33580,#33581,#33582,#33583,#33584,#33585,#33586,#33587,#33588,
#33589,#33590,#33591,#33592,#33593,#33594,#33595,#33596,#33597,#33598,#33599,
#33600,#33601,#33602,#33603,#33604,#33605,#33606,#33607,#33608,#33609,#33610,
#33611,#33612,#33613,#33614,#33615,#33616,#33617,#33618,#33619,#33620,#33621,
#33622,#33623,#33624,#33625,#33626,#33627,#33628,#33629,#33630,#33631,#33632,
#33633,#33634,#33635,#33636,#33637,#33638,#33639,#33640,#33641,#33642,#33643,
#33644,#33645,#33646,#33647,#33648,#33649,#33650,#33651,#33652,#33653,#33654,
#33655,#33656,#33657,#33658,#33659,#33660,#33661),.UNSPECIFIED.,.F.,.F.,
(4,2,2,2,2,2,2,2,2,2,2,2,2,2,2,2,2,2,2,2,2,2,2,2,2,2,2,2,2,2,2,2,2,2,2,
2,2,2,2,2,2,2,2,2,2,2,2,2,2,2,2,2,2,2,2,2,2,2,2,2,2,2,2,2,2,2,2,2,2,2,2,
2,2,2,2,2,2,2,2,2,2,2,2,2,2,2,2,2,2,2,2,2,2,2,2,2,2,2,2,2,2,2,2,2,2,2,2,
2,2,2,2,2,2,2,2,2,2,2,2,2,2,2,2,2,2,2,4),(-3.17295317748813,-3.13881949854016,
-3.13254270590914,-3.12840291351881,-3.12507038797027,-3.12192404985369,
-3.11797162534583,-3.11123133273975,-3.08501080934386,-3.05522340437467,
-3.03074665335081,-3.00497439810983,-3.0006991674959,-2.99838609230363,
-2.99642612004274,-2.99391236753246,-2.9898364238491,-2.9611176016517,-2.92662814993266,
-2.89871982649288,-2.88737551382644,-2.87868711235728,-2.8744600006815,
-2.8744364134477,-2.87441147941909,-2.87438511682015,-2.8743572384032,-2.87432775102356,
-2.87429655520012,-2.8742635446276,-2.87422860563979,-2.87419161662758,
-2.87415244742281,-2.8741109586162,-2.87406700082171,-2.87402041387674,
-2.87397102598451,-2.87391865277373,-2.87386309629366,-2.87380414393727,
-2.87374156727799,-2.87367512083198,-2.87360454074046,-2.87352954338432,
-2.87344982393563,-2.8733929887828,-2.87331706586271,-2.87321562690077,
-2.87308008082605,-2.86957491218778,-2.86509160468945,-2.85576294460097,
-2.79450934558193,-2.75558287221551,-2.75017890530165,-2.74763840595148,
-2.74567613933805,-2.74338202098676,-2.73930937866326,-2.7207181388602,
-2.66720596802176,-2.63308569150018,-2.62612750684263,-2.62212790243688,
-2.61863772129548,-2.61431215038077,-2.60762745597193,-2.55911536298477,
-2.52163446164379,-2.50852108535286,-2.50015649708243,-2.49713595237334,
-2.49509624506778,-2.49325773677067,-2.49072191109271,-2.48426452412769,
-2.44550110633697,-2.40249047862435,-2.38040457173732,-2.37423929543012,
-2.37041226741027,-2.36688856816085,-2.3623392562156,-2.3523918819042,-2.30086983474745,
-2.27116430152585,-2.25760646902335,-2.24903891214524,-2.24599061920154,
-2.24394519611649,-2.24211167596562,-2.23959552548921,-2.23325599985454,
-2.18850062422496,-2.13301145627603,-2.12470306567651,-2.12042041084192,
-2.11693326434142,-2.1129020124388,-2.10598235030052,-2.07566510148396,
-2.02527526430655,-2.00827971161612,-2.00151107708111,-1.99642364881248,
-1.9939443902317,-1.99217469169529,-1.98991322019257,-1.98598337853484,
-1.96958029229012,-1.90508280392682,-1.88759985645926,-1.87541527587832,
-1.87043544890947,-1.86685418031766,-1.86358877407033,-1.85919699769326,
-1.8506070444512,-1.79142675495546,-1.75017420819679,-1.7451558612457,-1.74269029675122,
-1.74092214038338,-1.73865120440277,-1.7346795553971,-1.71766968926413,
-1.67592320998144),.UNSPECIFIED.);
#422=B_SPLINE_CURVE_WITH_KNOTS('',3,(#33667,#33668,#33669,#33670,#33671,
#33672,#33673,#33674,#33675,#33676,#33677,#33678,#33679,#33680,#33681,#33682,
#33683,#33684,#33685,#33686,#33687,#33688,#33689,#33690,#33691,#33692,#33693,
#33694,#33695,#33696,#33697,#33698,#33699,#33700,#33701,#33702,#33703,#33704,
#33705,#33706,#33707,#33708,#33709,#33710,#33711,#33712,#33713,#33714,#33715,
#33716,#33717,#33718,#33719,#33720,#33721,#33722,#33723,#33724,#33725,#33726,
#33727,#33728,#33729,#33730,#33731,#33732,#33733,#33734,#33735,#33736,#33737,
#33738,#33739,#33740,#33741,#33742,#33743,#33744,#33745,#33746,#33747,#33748,
#33749,#33750,#33751,#33752,#33753,#33754,#33755,#33756,#33757,#33758,#33759,
#33760,#33761,#33762,#33763,#33764,#33765,#33766,#33767,#33768,#33769,#33770,
#33771,#33772,#33773,#33774,#33775,#33776,#33777,#33778,#33779,#33780,#33781,
#33782,#33783,#33784,#33785,#33786,#33787,#33788,#33789,#33790,#33791,#33792,
#33793,#33794,#33795,#33796,#33797,#33798,#33799,#33800,#33801,#33802,#33803,
#33804,#33805,#33806,#33807,#33808,#33809,#33810,#33811,#33812,#33813,#33814,
#33815,#33816,#33817,#33818,#33819,#33820,#33821,#33822,#33823,#33824,#33825,
#33826,#33827,#33828,#33829,#33830,#33831,#33832,#33833,#33834,#33835,#33836,
#33837,#33838,#33839,#33840,#33841,#33842,#33843,#33844,#33845,#33846,#33847),
 .UNSPECIFIED.,.F.,.F.,(4,3,3,3,3,3,3,3,3,3,3,3,3,3,3,3,3,3,3,3,3,3,3,3,
3,3,3,3,3,3,3,3,3,3,3,3,3,3,3,3,3,3,3,3,3,3,3,3,3,3,3,3,3,3,3,3,3,3,3,3,
4),(51.9295889271401,52.030670724834,52.1294177394015,52.2281292244128,
52.3268349684299,52.4296870534953,52.5285312410374,52.6274451637171,52.7265117204176,
52.7382433086914,52.8373024262761,52.9362211005355,53.035856525868,53.1345985272188,
53.2333080539688,53.3320148919206,53.4323372947392,53.5311858880997,53.6322451956473,
53.733304503195,53.8323636207797,53.9312822950391,54.0309177203715,54.1296597217224,
54.2283692484724,54.3270760864241,54.4273984892428,54.5262470826032,54.6273063901509,
54.7283656976986,54.8274248152832,54.9263434895427,55.0259789148751,55.124720916226,
55.2234304429759,55.3221372809276,55.4224596837463,55.5213082771068,55.6223675846545,
55.7234268922022,55.8224860097869,55.9214046840463,56.0210401093787,56.1197821107296,
56.2184916374796,56.3171984754314,56.41752087825,56.5163694716105,56.6174287791582,
56.7184880867059,56.8175472042906,56.91646587855,57.0161013038825,57.1148433052334,
57.2135528319833,57.3122596699352,57.4125820727538,57.5114306661142,57.6124899736619,
57.7135492812095,57.8582309055932),.UNSPECIFIED.);
#423=B_SPLINE_CURVE_WITH_KNOTS('',3,(#33848,#33849,#33850,#33851,#33852,
#33853,#33854,#33855,#33856,#33857,#33858,#33859,#33860),.UNSPECIFIED.,
 .F.,.F.,(4,3,3,3,4),(57.8582309058229,57.9557212708262,58.053112517412,
58.150435644654,58.21253113431),.UNSPECIFIED.);
#424=B_SPLINE_CURVE_WITH_KNOTS('',3,(#33861,#33862,#33863,#33864,#33865,
#33866,#33867,#33868,#33869,#33870,#33871,#33872,#33873,#33874,#33875,#33876,
#33877,#33878,#33879,#33880,#33881,#33882,#33883,#33884,#33885,#33886,#33887,
#33888,#33889,#33890,#33891,#33892,#33893,#33894,#33895,#33896,#33897,#33898,
#33899,#33900,#33901,#33902,#33903,#33904,#33905,#33906,#33907,#33908,#33909,
#33910,#33911,#33912,#33913,#33914,#33915,#33916,#33917,#33918,#33919,#33920,
#33921,#33922,#33923,#33924,#33925,#33926,#33927,#33928,#33929,#33930,#33931,
#33932,#33933,#33934,#33935,#33936,#33937,#33938,#33939,#33940,#33941,#33942,
#33943,#33944,#33945,#33946,#33947,#33948,#33949,#33950,#33951,#33952,#33953,
#33954,#33955,#33956,#33957,#33958,#33959,#33960,#33961,#33962,#33963,#33964,
#33965,#33966,#33967,#33968,#33969,#33970,#33971,#33972,#33973,#33974,#33975,
#33976,#33977,#33978,#33979,#33980,#33981,#33982,#33983,#33984,#33985,#33986,
#33987,#33988,#33989,#33990,#33991,#33992,#33993,#33994,#33995,#33996,#33997,
#33998,#33999,#34000,#34001,#34002,#34003,#34004,#34005,#34006,#34007,#34008,
#34009,#34010,#34011,#34012,#34013,#34014,#34015,#34016,#34017,#34018,#34019,
#34020,#34021,#34022,#34023,#34024,#34025,#34026,#34027,#34028,#34029,#34030,
#34031,#34032,#34033,#34034,#34035,#34036,#34037,#34038,#34039,#34040,#34041,
#34042,#34043,#34044,#34045,#34046,#34047,#34048,#34049,#34050,#34051,#34052,
#34053,#34054,#34055,#34056,#34057,#34058,#34059,#34060,#34061,#34062,#34063,
#34064,#34065,#34066,#34067,#34068,#34069,#34070,#34071,#34072,#34073,#34074,
#34075,#34076,#34077,#34078,#34079,#34080,#34081,#34082,#34083,#34084,#34085,
#34086,#34087,#34088,#34089,#34090,#34091,#34092,#34093,#34094,#34095,#34096,
#34097,#34098,#34099,#34100,#34101,#34102,#34103,#34104,#34105,#34106,#34107,
#34108,#34109,#34110,#34111,#34112,#34113,#34114,#34115,#34116,#34117,#34118,
#34119,#34120,#34121,#34122,#34123,#34124,#34125,#34126,#34127,#34128,#34129,
#34130,#34131,#34132,#34133,#34134,#34135,#34136,#34137,#34138,#34139,#34140,
#34141,#34142,#34143,#34144),.UNSPECIFIED.,.F.,.F.,(4,2,2,2,2,2,2,2,2,2,
2,2,2,2,2,2,2,2,2,2,2,2,2,2,2,2,2,2,2,2,2,2,2,2,2,2,2,2,2,2,2,2,2,2,2,2,
2,2,2,2,2,2,2,2,2,2,2,2,2,2,2,2,2,2,2,2,2,2,2,2,2,2,2,2,2,2,2,2,2,2,2,2,
2,2,2,2,2,2,2,2,2,2,2,2,2,2,2,2,2,2,2,2,2,2,2,2,2,2,2,2,2,2,2,2,2,2,2,2,
2,2,2,2,2,2,2,2,2,2,2,2,2,2,2,2,2,2,2,2,2,2,2,4),(-1.67592320998144,-1.64801987356236,
-1.63382763456696,-1.62341555588315,-1.61873363522818,-1.61520263671616,
-1.61140060802024,-1.60534751231179,-1.58644977368995,-1.55255126979351,
-1.50058225176569,-1.49450383036933,-1.49210459370419,-1.49011959022917,
-1.48798398052661,-1.48451948762301,-1.47231678925401,-1.44954183418719,
-1.39715730539802,-1.37591560258209,-1.36960485512921,-1.36574678339733,
-1.36223327665017,-1.35767496110344,-1.34794300656535,-1.30812976654373,
-1.26525775355338,-1.24641153155549,-1.24232347314032,-1.24002631665237,
-1.23806518190785,-1.235530956359,-1.2301573812203,-1.22289180980846,-1.20396354763412,
-1.14057172608681,-1.12375311573915,-1.11795315223345,-1.11420606475655,
-1.11065229109488,-1.10582614633735,-1.09457850972797,-1.05189306089402,
-0.999138571291884,-0.992634191801533,-0.990090867899693,-0.988250830218791,
-0.986214138505041,-0.983206029528501,-0.974926774739709,-0.918371911446345,
-0.875678779087676,-0.868990641786553,-0.864664937209232,-0.861175981087088,
-0.857179241571935,-0.85022980876337,-0.816245099449129,-0.763823548761383,
-0.744201390372336,-0.740069840368587,-0.737762978002056,-0.735803135369725,
-0.733282929926665,-0.727982113991956,-0.697844496036856,-0.684698883442765,
-0.628300630357481,-0.618558241503323,-0.614047196493481,-0.610530073999733,
-0.606686904126458,-0.600443323483241,-0.577438742636601,-0.536955774331928,
-0.496827218990667,-0.490379968424935,-0.487846408578358,-0.486008942353855,
-0.483969688502199,-0.480948600462394,-0.472574889440919,-0.459438111384135,
-0.422120589282921,-0.373470484552808,-0.366787522559929,-0.362463410562818,
-0.358974600626299,-0.354976780873375,-0.348022237096805,-0.313927516957458,
-0.26393248475239,-0.242215310075114,-0.238339088188428,-0.235885712801448,
-0.233993280108135,-0.233974273408042,-0.233955712653511,-0.233937580843393,
-0.233919861832381,-0.233902540274617,-0.23388560157789,-0.233869031867375,
-0.233852817934698,-0.233836947198216,-0.233821407641112,-0.233806187816045,
-0.233791276823863,-0.233776664239748,-0.233762340095032,-0.233748294873074,
-0.233734519460936,-0.233721005171065,-0.233707743668982,-0.233694726943997,
-0.233681947358699,-0.233669397574497,-0.233657070550256,-0.233644959535232,
-0.23363305807667,-0.23362135993261,-0.233609859115898,-0.23359854988632,
-0.233587426734408,-0.233576484351445,-0.233565717605655,-0.233555121573784,
-0.233544691527589,-0.233534422903674,-0.233524311295459,-0.231035451518287,
-0.22823743117379,-0.223523867326237,-0.213515204647212,-0.181647151558495,
-0.126191035270392,-0.116398316434333,-0.11187816708323,-0.108359849878644,
-0.104521338766822,-0.0982987539848973,-0.0902547838960883),
 .UNSPECIFIED.);
#425=B_SPLINE_CURVE_WITH_KNOTS('',3,(#34150,#34151,#34152,#34153,#34154,
#34155,#34156,#34157,#34158,#34159,#34160,#34161,#34162,#34163,#34164,#34165,
#34166,#34167,#34168,#34169,#34170,#34171,#34172,#34173,#34174,#34175,#34176,
#34177,#34178,#34179,#34180,#34181,#34182,#34183,#34184,#34185,#34186,#34187,
#34188,#34189,#34190,#34191,#34192,#34193,#34194,#34195,#34196,#34197,#34198,
#34199,#34200,#34201,#34202,#34203,#34204,#34205,#34206,#34207,#34208,#34209,
#34210,#34211,#34212,#34213,#34214,#34215,#34216,#34217,#34218,#34219,#34220,
#34221,#34222,#34223,#34224,#34225,#34226,#34227,#34228,#34229,#34230,#34231,
#34232,#34233,#34234,#34235,#34236,#34237,#34238,#34239,#34240,#34241,#34242,
#34243,#34244,#34245,#34246,#34247,#34248,#34249,#34250,#34251,#34252,#34253,
#34254,#34255,#34256,#34257,#34258,#34259,#34260,#34261,#34262,#34263,#34264,
#34265,#34266,#34267,#34268,#34269,#34270,#34271,#34272,#34273,#34274,#34275,
#34276,#34277,#34278,#34279,#34280,#34281,#34282,#34283,#34284,#34285,#34286,
#34287,#34288,#34289,#34290,#34291,#34292,#34293,#34294,#34295,#34296,#34297,
#34298,#34299,#34300,#34301,#34302,#34303,#34304,#34305,#34306,#34307,#34308,
#34309,#34310,#34311,#34312,#34313,#34314,#34315,#34316,#34317,#34318,#34319,
#34320,#34321,#34322,#34323,#34324,#34325,#34326,#34327,#34328,#34329,#34330,
#34331,#34332,#34333),.UNSPECIFIED.,.F.,.F.,(4,3,3,3,3,3,3,3,3,3,3,3,3,
3,3,3,3,3,3,3,3,3,3,3,3,3,3,3,3,3,3,3,3,3,3,3,3,3,3,3,3,3,3,3,3,3,3,3,3,
3,3,3,3,3,3,3,3,3,3,3,3,4),(45.6452512469328,45.7501622262758,45.7728149471661,
45.8718740647508,45.9707927390103,46.0704281643427,46.1691701656936,46.2678796924436,
46.3665865303954,46.466908933214,46.5657575265745,46.6668168341221,46.7678761416697,
46.8669352592544,46.9658539335138,47.0654893588463,47.1642313601972,47.2629408869471,
47.3616477248989,47.4619701277175,47.560818721078,47.6618780286257,47.7629373361734,
47.861996453758,47.9609151280175,48.0605505533499,48.1592925547008,48.2580020814507,
48.3567089194025,48.4570313222211,48.5558799155816,48.6569392231293,48.757998530677,
48.8570576482617,48.955976322521,49.0556117478535,49.1543537492043,49.2530632759543,
49.351770113906,49.4520925167247,49.5509411100851,49.6520004176329,49.7530597251806,
49.8521188427653,49.9510375170247,50.0506729423571,50.149414943708,50.248124470458,
50.3468313084098,50.4471537112284,50.5460023045889,50.6470616121365,50.7481209196842,
50.8457129935022,50.9431428324126,51.0404816382021,51.1377609277275,51.2350121400975,
51.3323110164859,51.4296360130139,51.5270774501444,51.5750455980497),
 .UNSPECIFIED.);
#426=B_SPLINE_CURVE_WITH_KNOTS('',3,(#34334,#34335,#34336,#34337,#34338,
#34339,#34340,#34341,#34342,#34343,#34344,#34345,#34346),.UNSPECIFIED.,
 .F.,.F.,(4,3,3,3,4),(51.5750455984136,51.7300295918754,51.7431821141878,
51.8422151608463,51.9295889271401),.UNSPECIFIED.);
#427=B_SPLINE_CURVE_WITH_KNOTS('',3,(#34348,#34349,#34350,#34351,#34352,
#34353),.UNSPECIFIED.,.F.,.F.,(4,2,4),(-0.0902547838960883,-0.0755381864946324,
-0.000735838667914899),.UNSPECIFIED.);
#428=B_SPLINE_CURVE_WITH_KNOTS('',3,(#34354,#34355,#34356,#34357,#34358,
#34359,#34360,#34361,#34362,#34363,#34364,#34365,#34366,#34367,#34368,#34369,
#34370,#34371,#34372,#34373,#34374,#34375,#34376,#34377,#34378,#34379,#34380,
#34381,#34382,#34383,#34384,#34385,#34386,#34387,#34388,#34389,#34390,#34391,
#34392,#34393,#34394,#34395,#34396,#34397,#34398,#34399,#34400,#34401,#34402,
#34403,#34404,#34405,#34406,#34407,#34408,#34409,#34410,#34411,#34412,#34413,
#34414,#34415,#34416,#34417,#34418,#34419,#34420,#34421,#34422,#34423,#34424,
#34425,#34426,#34427,#34428,#34429,#34430,#34431,#34432,#34433,#34434,#34435,
#34436,#34437,#34438,#34439,#34440,#34441,#34442,#34443,#34444,#34445,#34446,
#34447,#34448,#34449,#34450,#34451,#34452,#34453,#34454,#34455,#34456,#34457,
#34458,#34459,#34460,#34461,#34462,#34463,#34464,#34465,#34466,#34467,#34468,
#34469,#34470,#34471,#34472,#34473,#34474,#34475,#34476,#34477,#34478,#34479,
#34480,#34481,#34482,#34483,#34484,#34485,#34486,#34487,#34488,#34489,#34490,
#34491,#34492,#34493,#34494,#34495,#34496,#34497,#34498,#34499,#34500,#34501,
#34502,#34503,#34504,#34505,#34506,#34507,#34508,#34509,#34510,#34511,#34512,
#34513,#34514,#34515,#34516,#34517,#34518,#34519,#34520,#34521,#34522,#34523,
#34524,#34525,#34526,#34527,#34528,#34529,#34530,#34531,#34532,#34533,#34534,
#34535,#34536,#34537,#34538,#34539,#34540,#34541,#34542,#34543,#34544,#34545,
#34546,#34547,#34548,#34549,#34550,#34551,#34552,#34553,#34554,#34555,#34556,
#34557),.UNSPECIFIED.,.F.,.F.,(4,2,2,2,2,2,2,2,2,2,2,2,2,2,2,2,2,2,2,2,
2,2,2,2,2,2,2,2,2,2,2,2,2,2,2,2,2,2,2,2,2,2,2,2,2,2,2,2,2,2,2,2,2,2,2,2,
2,2,2,2,2,2,2,2,2,2,2,2,2,2,2,2,2,2,2,2,2,2,2,2,2,2,2,2,2,2,2,2,2,2,2,2,
2,2,2,2,2,2,2,2,2,4),(-3.17298666581179,-3.16563141916398,-3.16059756997835,
-3.15835235769896,-3.15650595198463,-3.15462878690909,-3.15209114925753,
-3.1479350984291,-3.13236830659073,-3.06800305622745,-3.04166816243616,
-3.03516350889059,-3.03126242370672,-3.02775762557886,-3.02327736620085,
-3.01396460456103,-2.95248174887367,-2.92459997801962,-2.91533808156676,
-2.91087169695868,-2.90817241857315,-2.90574168526152,-2.90381935963668,
-2.90150573483734,-2.8973465919083,-2.87726454855109,-2.81059087786807,
-2.79663008411779,-2.78634765729626,-2.78168834538372,-2.77816018411837,
-2.77481391115882,-2.76915405957496,-2.75342346764264,-2.69613911881825,
-2.6610955226833,-2.65659319807143,-2.65423231370343,-2.65227574303146,
-2.64982153022093,-2.64594399790897,-2.62423560721442,-2.57802327778507,
-2.55294696862275,-2.54236062444264,-2.53406458939325,-2.52978436337409,
-2.526297263886,-2.52226390750591,-2.51533527089136,-2.48485795017648,-2.43454581906813,
-2.41761362011077,-2.41086169515979,-2.40578398538528,-2.40330659278867,
-2.40153705482741,-2.39927416826418,-2.39533830573911,-2.37885141408669,
-2.3086733539788,-2.29444180510874,-2.28400750064803,-2.2793214002882,-2.27578953883554,
-2.27245197735828,-2.26683659806314,-2.2514154710157,-2.18662120967513,
-2.16744718799289,-2.15654586787731,-2.15321460908982,-2.15110818648012,
-2.14910600115559,-2.14663939466139,-2.14058855242489,-2.08999986217308,
-2.0444108637344,-2.0331619659822,-2.0283350017407,-2.02478053842007,-2.021032646738,
-2.01523127308426,-1.99840699957501,-1.94213711660028,-1.91048059898588,
-1.90401588276398,-1.90128582086879,-1.89929993583942,-1.89711264558408,
-1.89341535429896,-1.88023206284989,-1.82539214966138,-1.79014171544812,
-1.78096875465978,-1.77651574521964,-1.77301453179121,-1.76909904415105,
-1.76252619374566,-1.73848491173098,-1.6885199140946,-1.67620980708928),
 .UNSPECIFIED.);
#429=B_SPLINE_CURVE_WITH_KNOTS('',3,(#34563,#34564,#34565,#34566,#34567,
#34568,#34569,#34570,#34571,#34572,#34573,#34574,#34575,#34576,#34577,#34578,
#34579,#34580,#34581,#34582,#34583,#34584,#34585,#34586,#34587,#34588,#34589,
#34590,#34591,#34592,#34593,#34594,#34595,#34596,#34597,#34598,#34599,#34600,
#34601,#34602,#34603,#34604,#34605,#34606,#34607,#34608,#34609,#34610,#34611,
#34612,#34613,#34614,#34615,#34616,#34617,#34618,#34619,#34620,#34621,#34622,
#34623,#34624,#34625,#34626,#34627,#34628,#34629,#34630,#34631,#34632,#34633,
#34634,#34635,#34636,#34637,#34638,#34639,#34640,#34641,#34642,#34643,#34644,
#34645,#34646,#34647,#34648,#34649,#34650,#34651,#34652,#34653,#34654,#34655,
#34656,#34657,#34658,#34659,#34660,#34661,#34662,#34663,#34664,#34665,#34666,
#34667,#34668,#34669,#34670,#34671,#34672,#34673,#34674,#34675,#34676,#34677,
#34678,#34679,#34680,#34681,#34682,#34683,#34684,#34685,#34686,#34687,#34688,
#34689,#34690,#34691,#34692,#34693,#34694,#34695,#34696,#34697,#34698,#34699,
#34700,#34701,#34702,#34703,#34704,#34705,#34706,#34707,#34708,#34709,#34710,
#34711,#34712,#34713,#34714,#34715,#34716,#34717,#34718,#34719,#34720,#34721,
#34722,#34723,#34724,#34725,#34726,#34727,#34728,#34729,#34730,#34731,#34732,
#34733,#34734,#34735,#34736,#34737,#34738,#34739,#34740,#34741,#34742,#34743),
 .UNSPECIFIED.,.F.,.F.,(4,3,3,3,3,3,3,3,3,3,3,3,3,3,3,3,3,3,3,3,3,3,3,3,
3,3,3,3,3,3,3,3,3,3,3,3,3,3,3,3,3,3,3,3,3,3,3,3,3,3,3,3,3,3,3,3,3,3,3,3,
4),(39.3627615986102,39.4600795768122,39.5574939443465,39.6549619992771,
39.7525891288265,39.8024477801445,39.9015068977292,40.0004255719887,40.1000609973211,
40.198802998672,40.2975125254219,40.3962193633735,40.4965417661922,40.5953903595526,
40.6964496671004,40.7975089746481,40.8965680922328,40.9954867664921,41.0951221918246,
41.1938641931755,41.2925737199253,41.391280557877,41.4916029606957,41.5904515540561,
41.6915108616039,41.7925701691517,41.8916292867363,41.9905479609956,42.0901833863281,
42.1889253876789,42.2876349144288,42.3863417523807,42.4866641551993,42.5855127485597,
42.6865720561075,42.7876313636553,42.88669048124,42.9856091554994,43.0852445808319,
43.1839865821828,43.2826961089327,43.3814029468844,43.481725349703,43.5805739430635,
43.6816332506112,43.7826925581589,43.8817516757436,43.9806703500033,44.0803057753357,
44.1790477766866,44.2777573034363,44.3764641413878,44.4767865442065,44.575635137567,
44.6766944451147,44.7777537526625,44.8811334637461,44.9842446946404,45.0871977961312,
45.1899571772778,45.2918602912341),.UNSPECIFIED.);
#430=B_SPLINE_CURVE_WITH_KNOTS('',3,(#34744,#34745,#34746,#34747,#34748,
#34749,#34750,#34751,#34752,#34753,#34754,#34755,#34756),.UNSPECIFIED.,
 .F.,.F.,(4,3,3,3,4),(45.2918602914973,45.3960300286389,45.5003580305241,
45.6049489906218,45.6452512469328),.UNSPECIFIED.);
#431=B_SPLINE_CURVE_WITH_KNOTS('',3,(#34757,#34758,#34759,#34760,#34761,
#34762,#34763,#34764,#34765,#34766,#34767,#34768,#34769,#34770,#34771,#34772,
#34773,#34774,#34775,#34776,#34777,#34778,#34779,#34780,#34781,#34782,#34783,
#34784,#34785,#34786,#34787,#34788,#34789,#34790,#34791,#34792,#34793,#34794,
#34795,#34796,#34797,#34798,#34799,#34800,#34801,#34802,#34803,#34804,#34805,
#34806,#34807,#34808,#34809,#34810,#34811,#34812,#34813,#34814,#34815,#34816,
#34817,#34818,#34819,#34820,#34821,#34822,#34823,#34824,#34825,#34826,#34827,
#34828,#34829,#34830,#34831,#34832,#34833,#34834,#34835,#34836,#34837,#34838,
#34839,#34840,#34841,#34842,#34843,#34844,#34845,#34846,#34847,#34848,#34849,
#34850,#34851,#34852,#34853,#34854,#34855,#34856,#34857,#34858,#34859,#34860,
#34861,#34862,#34863,#34864,#34865,#34866,#34867,#34868,#34869,#34870,#34871,
#34872,#34873,#34874,#34875,#34876,#34877,#34878,#34879,#34880,#34881,#34882,
#34883,#34884,#34885,#34886,#34887,#34888,#34889,#34890,#34891,#34892,#34893,
#34894,#34895,#34896,#34897,#34898,#34899,#34900,#34901,#34902,#34903,#34904,
#34905,#34906,#34907,#34908,#34909,#34910,#34911,#34912,#34913,#34914,#34915,
#34916,#34917,#34918,#34919,#34920,#34921,#34922,#34923,#34924,#34925,#34926,
#34927,#34928,#34929,#34930,#34931,#34932,#34933,#34934,#34935,#34936,#34937,
#34938,#34939,#34940,#34941,#34942,#34943,#34944,#34945,#34946,#34947,#34948,
#34949,#34950,#34951,#34952,#34953,#34954,#34955,#34956,#34957,#34958,#34959,
#34960,#34961,#34962,#34963,#34964,#34965,#34966,#34967,#34968,#34969,#34970,
#34971,#34972,#34973,#34974,#34975,#34976),.UNSPECIFIED.,.F.,.F.,(4,2,2,
2,2,2,2,2,2,2,2,2,2,2,2,2,2,2,2,2,2,2,2,2,2,2,2,2,2,2,2,2,2,2,2,2,2,2,2,
2,2,2,2,2,2,2,2,2,2,2,2,2,2,2,2,2,2,2,2,2,2,2,2,2,2,2,2,2,2,2,2,2,2,2,2,
2,2,2,2,2,2,2,2,2,2,2,2,2,2,2,2,2,2,2,2,2,2,2,2,2,2,2,2,2,2,2,2,2,2,4),
(-1.67620980708928,-1.66640396248898,-1.65442852491712,-1.65098613315536,
-1.64885529433634,-1.64686758732065,-1.64445767447368,-1.63831256449055,
-1.58708365957732,-1.54037389911875,-1.53029087362987,-1.52571772696811,
-1.52219105788161,-1.51837618836454,-1.51226438188968,-1.49075755169447,
-1.42005532763171,-1.40413557489153,-1.40024128409183,-1.39798802132766,
-1.39621711346142,-1.39372619749178,-1.38857873613451,-1.38170622448344,
-1.36431448504218,-1.31340038515004,-1.28405334736977,-1.27718886084294,
-1.2731703025766,-1.26968242211879,-1.26538389909587,-1.25699601434651,
-1.21275366991191,-1.16582932985959,-1.15254605342861,-1.14883941199621,
-1.14665003850391,-1.14466484676266,-1.1419393032769,-1.1355014577652,-1.10412259193519,
-1.04868002323832,-1.03090739425258,-1.02498730949448,-1.02121384829015,
-1.01767111313951,-1.01291550301722,-1.00208462613817,-0.987140444444101,
-0.94240665056427,-0.925877880191999,-0.919080720755033,-0.901983154629366,
-0.898005848074418,-0.895733662995074,-0.893965765407025,-0.891502116813433,
-0.886493201876764,-0.845610100424215,-0.785938569314373,-0.776441463805464,
-0.77192684995559,-0.768418640465444,-0.764537670644353,-0.758122775715849,
-0.732993785994031,-0.703728287952091,-0.654306317631853,-0.648205655514477,
-0.645730575823987,-0.643726325894904,-0.641623699313264,-0.638308892099879,
-0.627555868853611,-0.60876537285979,-0.548097229529708,-0.528933710734291,
-0.52285039706297,-0.519041897927518,-0.515513389284958,-0.510847394425225,
-0.500523998685228,-0.486491083448626,-0.418878452089067,-0.399835748695025,
-0.395736202912422,-0.393436352806003,-0.391475382090186,-0.388944557094879,
-0.383589399826682,-0.376356216443083,-0.357557645879962,-0.296761032303342,
-0.277709131803074,-0.271638333137631,-0.267832487266175,-0.264373154669794,
-0.259895189605234,-0.254907261259269,-0.246554379639805,-0.228921935900892,
-0.162569436010408,-0.148050774553925,-0.144232290987578,-0.142018380918343,
-0.140040963712573,-0.137367023269518,-0.131228439263144,-0.102837806382509,
-0.0901712924560195),.UNSPECIFIED.);
#432=B_SPLINE_CURVE_WITH_KNOTS('',3,(#34982,#34983,#34984,#34985,#34986,
#34987,#34988,#34989,#34990,#34991,#34992,#34993,#34994,#34995,#34996,#34997,
#34998,#34999,#35000,#35001,#35002,#35003,#35004,#35005,#35006,#35007,#35008,
#35009,#35010,#35011,#35012,#35013,#35014,#35015,#35016,#35017,#35018,#35019,
#35020,#35021,#35022,#35023,#35024,#35025,#35026,#35027,#35028,#35029,#35030,
#35031,#35032,#35033,#35034,#35035,#35036,#35037,#35038,#35039,#35040,#35041,
#35042,#35043,#35044,#35045,#35046,#35047,#35048,#35049,#35050,#35051,#35052,
#35053,#35054,#35055,#35056,#35057,#35058,#35059,#35060,#35061,#35062,#35063,
#35064,#35065,#35066,#35067,#35068,#35069,#35070,#35071,#35072,#35073,#35074,
#35075,#35076,#35077,#35078,#35079,#35080,#35081,#35082,#35083,#35084,#35085,
#35086,#35087,#35088,#35089,#35090,#35091,#35092,#35093,#35094,#35095,#35096,
#35097,#35098,#35099,#35100,#35101,#35102,#35103,#35104,#35105,#35106,#35107,
#35108,#35109,#35110,#35111,#35112,#35113,#35114,#35115,#35116,#35117,#35118,
#35119,#35120,#35121,#35122,#35123,#35124,#35125,#35126,#35127,#35128,#35129,
#35130,#35131,#35132,#35133,#35134,#35135,#35136,#35137,#35138,#35139,#35140,
#35141,#35142,#35143,#35144,#35145,#35146,#35147,#35148,#35149,#35150,#35151,
#35152,#35153,#35154,#35155,#35156,#35157,#35158,#35159,#35160,#35161,#35162),
 .UNSPECIFIED.,.F.,.F.,(4,3,3,3,3,3,3,3,3,3,3,3,3,3,3,3,3,3,3,3,3,3,3,3,
3,3,3,3,3,3,3,3,3,3,3,3,3,3,3,3,3,3,3,3,3,3,3,3,3,3,3,3,3,3,3,3,3,3,3,3,
4),(33.0800282649154,33.1788010120089,33.2775248054047,33.3762294491433,
33.4749447203013,33.5737644425482,33.672640731442,33.7716835211257,33.8320806131228,
33.9311397307074,34.0300584049668,34.1296938302993,34.2284358316501,34.3271453584001,
34.4258521963519,34.5261745991705,34.6250231925309,34.7260825000787,34.8271418076264,
34.9262009252112,35.0251195994707,35.1247550248031,35.2234970261541,35.3222065529041,
35.420913390856,35.5212357936745,35.6200843870351,35.7211436945826,35.82220300213,
35.9212621197146,36.020180793974,36.1198162193064,36.2185582206573,36.3172677474071,
36.4159745853588,36.5162969881775,36.615145581538,36.7162048890858,36.8172641966336,
36.9163233142182,37.0152419884777,37.1148774138101,37.213619415161,37.3123289419109,
37.4110357798627,37.5113581826814,37.6102067760418,37.7112660835895,37.8123253911372,
37.9113845087219,38.0103031829814,38.1099386083138,38.2086806096647,38.3073901364147,
38.4060969743665,38.5064193771851,38.6052679705456,38.7063272780932,38.8073865856408,
38.9480297229085,39.0086749840545),.UNSPECIFIED.);
#433=B_SPLINE_CURVE_WITH_KNOTS('',3,(#35163,#35164,#35165,#35166,#35167,
#35168,#35169,#35170,#35171,#35172,#35173,#35174,#35175),.UNSPECIFIED.,
 .F.,.F.,(4,3,3,3,4),(39.0086749844289,39.1061283327374,39.2034999696831,
39.3008301777854,39.3627615986102),.UNSPECIFIED.);
#434=B_SPLINE_CURVE_WITH_KNOTS('',3,(#35177,#35178,#35179,#35180,#35181,
#35182,#35183,#35184,#35185,#35186,#35187,#35188,#35189,#35190,#35191,#35192,
#35193,#35194),.UNSPECIFIED.,.F.,.F.,(4,2,2,2,2,2,2,2,4),(-0.0901712924560195,
-0.0419045892551838,-0.0257637905534428,-0.0200541212030024,-0.0163260946354891,
-0.0130012968151968,-0.00952881353369847,-0.00531895993925087,-0.000734738427498389),
 .UNSPECIFIED.);
#435=B_SPLINE_CURVE_WITH_KNOTS('',3,(#35195,#35196,#35197,#35198,#35199,
#35200,#35201,#35202,#35203,#35204,#35205,#35206,#35207,#35208,#35209,#35210,
#35211,#35212,#35213,#35214,#35215,#35216,#35217,#35218,#35219,#35220,#35221,
#35222,#35223,#35224,#35225,#35226,#35227,#35228,#35229,#35230,#35231,#35232,
#35233,#35234,#35235,#35236,#35237,#35238,#35239,#35240,#35241,#35242,#35243,
#35244,#35245,#35246,#35247,#35248,#35249,#35250,#35251,#35252,#35253,#35254,
#35255,#35256,#35257,#35258,#35259,#35260,#35261,#35262,#35263,#35264,#35265,
#35266,#35267,#35268,#35269,#35270,#35271,#35272,#35273,#35274,#35275,#35276,
#35277,#35278,#35279,#35280,#35281,#35282,#35283,#35284,#35285,#35286,#35287,
#35288,#35289,#35290,#35291,#35292,#35293,#35294,#35295,#35296,#35297,#35298,
#35299,#35300,#35301,#35302,#35303,#35304,#35305,#35306,#35307,#35308,#35309,
#35310,#35311,#35312,#35313,#35314,#35315,#35316,#35317,#35318,#35319,#35320,
#35321,#35322,#35323,#35324,#35325,#35326,#35327,#35328,#35329,#35330,#35331,
#35332,#35333,#35334,#35335,#35336,#35337,#35338,#35339,#35340,#35341,#35342,
#35343,#35344,#35345,#35346,#35347,#35348,#35349,#35350,#35351,#35352,#35353,
#35354,#35355,#35356,#35357,#35358,#35359,#35360,#35361,#35362,#35363,#35364,
#35365,#35366,#35367,#35368,#35369,#35370,#35371,#35372,#35373,#35374,#35375,
#35376,#35377,#35378,#35379,#35380,#35381,#35382,#35383,#35384,#35385,#35386,
#35387,#35388,#35389,#35390,#35391,#35392,#35393,#35394,#35395,#35396,#35397,
#35398,#35399,#35400,#35401,#35402,#35403,#35404,#35405,#35406,#35407,#35408,
#35409,#35410,#35411,#35412,#35413,#35414),.UNSPECIFIED.,.F.,.F.,(4,2,2,
2,2,2,2,2,2,2,2,2,2,2,2,2,2,2,2,2,2,2,2,2,2,2,2,2,2,2,2,2,2,2,2,2,2,2,2,
2,2,2,2,2,2,2,2,2,2,2,2,2,2,2,2,2,2,2,2,2,2,2,2,2,2,2,2,2,2,2,2,2,2,2,2,
2,2,2,2,2,2,2,2,2,2,2,2,2,2,2,2,2,2,2,2,2,2,2,2,2,2,2,2,2,2,2,2,2,2,4),
(-3.17213860495443,-3.1305769562313,-3.1011543313151,-3.07940569487357,
-3.06755913278467,-3.06412937072432,-3.06200121614224,-3.06001183753837,
-3.05759557415168,-3.05141079880141,-3.00074436630835,-2.95610171727953,
-2.94799787544405,-2.94311028336209,-2.9388423190976,-2.93878581376589,
-2.93872617091512,-2.93866302170105,-2.93859593747089,-2.93852441661367,
-2.93844786771765,-2.93836558771644,-2.93827673316758,-2.93818028195483,
-2.93807498135861,-2.93795927634505,-2.93463290382022,-2.93058354075275,
-2.92358311452377,-2.89261504641914,-2.85020348039682,-2.8283124036129,
-2.81641575970837,-2.81298110322945,-2.8108519274099,-2.80886323377176,
-2.80644949850555,-2.80028041505933,-2.74937910858284,-2.69963783857535,
-2.69130680027413,-2.68701988286206,-2.68353288471406,-2.67950584130784,
-2.67260340068405,-2.64258311380944,-2.59209004602213,-2.56675694200023,
-2.56249770513191,-2.56018826617702,-2.55822828324274,-2.55571053571208,
-2.55162043853799,-2.52205241740852,-2.48615474983624,-2.450024113373,-2.44073933772684,
-2.43626485570551,-2.43276121089515,-2.42885794036158,-2.42234136089115,
-2.39902370075791,-2.34278808641017,-2.32441657854521,-2.31382489314394,
-2.31052782164752,-2.30842895870605,-2.30642185025093,-2.30393641996668,
-2.29777657575977,-2.24939876308865,-2.2131415114354,-2.19982771577643,
-2.18991321886205,-2.18532086469977,-2.18180245458665,-2.17796012698621,
-2.17172298777249,-2.15115357121809,-2.09207049766749,-2.07339437663057,
-2.06268427389943,-2.05937400263014,-2.05727221534484,-2.05526703028496,
-2.05278894115209,-2.04667183055632,-1.99759164633159,-1.94556170241649,
-1.93758819768458,-1.93337427330436,-1.93022975370303,-1.92626816563616,
-1.91948356943942,-1.89257179180857,-1.83960741097014,-1.82179683775734,
-1.81481528442673,-1.80960433593195,-1.80710113985355,-1.80514217479726,
-1.80282176944635,-1.79863123416595,-1.77791047766794,-1.72651371559181,
-1.69262381260827,-1.68567753170966,-1.68168099400651,-1.67819127484788,
-1.67563146043802),.UNSPECIFIED.);
#436=B_SPLINE_CURVE_WITH_KNOTS('',3,(#35420,#35421,#35422,#35423,#35424,
#35425,#35426,#35427,#35428,#35429,#35430,#35431,#35432,#35433,#35434,#35435,
#35436,#35437,#35438,#35439,#35440,#35441,#35442,#35443,#35444,#35445,#35446,
#35447,#35448,#35449,#35450,#35451,#35452,#35453,#35454,#35455,#35456,#35457,
#35458,#35459,#35460,#35461,#35462,#35463,#35464,#35465,#35466,#35467,#35468,
#35469,#35470,#35471,#35472,#35473,#35474,#35475,#35476,#35477,#35478,#35479,
#35480,#35481,#35482,#35483,#35484,#35485,#35486,#35487,#35488,#35489,#35490,
#35491,#35492,#35493,#35494,#35495,#35496,#35497,#35498,#35499,#35500,#35501,
#35502,#35503,#35504,#35505,#35506,#35507,#35508,#35509,#35510,#35511,#35512,
#35513,#35514,#35515,#35516,#35517,#35518,#35519,#35520,#35521,#35522,#35523,
#35524,#35525,#35526,#35527,#35528,#35529,#35530,#35531,#35532,#35533,#35534,
#35535,#35536,#35537,#35538,#35539,#35540,#35541,#35542,#35543,#35544,#35545,
#35546,#35547,#35548,#35549,#35550,#35551,#35552,#35553,#35554,#35555,#35556,
#35557,#35558,#35559,#35560,#35561,#35562,#35563,#35564,#35565,#35566,#35567,
#35568,#35569,#35570,#35571,#35572,#35573,#35574,#35575,#35576,#35577,#35578,
#35579,#35580,#35581,#35582,#35583,#35584,#35585,#35586,#35587,#35588,#35589,
#35590,#35591,#35592,#35593,#35594,#35595,#35596,#35597,#35598,#35599,#35600),
 .UNSPECIFIED.,.F.,.F.,(4,3,3,3,3,3,3,3,3,3,3,3,3,3,3,3,3,3,3,3,3,3,3,3,
3,3,3,3,3,3,3,3,3,3,3,3,3,3,3,3,3,3,3,3,3,3,3,3,3,3,3,3,3,3,3,3,3,3,3,3,
4),(26.7958893988467,26.8666522515975,26.9657113691745,27.0646300434264,
27.1642654687607,27.2630074701039,27.3617169968462,27.4604238347903,27.560746237618,
27.659594830971,27.760654138536,27.8617134461011,27.9607725636811,28.0596912379358,
28.1593266632694,28.2580686646153,28.3567781913602,28.4554850293069,28.5558074321313,
28.6546560254866,28.7557153330456,28.8567746406047,28.9558337581938,29.0547524324578,
29.1543878577891,29.2531298591447,29.3518393858993,29.4505462238559,29.550868626669,
29.6497172200342,29.7507765275713,29.8518358351083,29.9508949526917,30.0498136269499,
30.1494490522826,30.2481910536322,30.3469005803809,30.4456074183313,30.5459298211515,
30.6447784145107,30.7458377220613,30.846897029612,30.9459561471962,31.0448748214552,
31.1445102467877,31.2432522481381,31.3419617748876,31.440668612839,31.5409910156581,
31.6398396090181,31.7408989165668,31.8419582241156,31.9397107034369,32.0379330750836,
32.1354344299566,32.2328770951219,32.3302923655519,32.4290916933166,32.5265951482246,
32.6260424124176,32.7254896766106),.UNSPECIFIED.);
#437=B_SPLINE_CURVE_WITH_KNOTS('',3,(#35601,#35602,#35603,#35604,#35605,
#35606,#35607,#35608,#35609,#35610,#35611,#35612,#35613),.UNSPECIFIED.,
 .F.,.F.,(4,3,3,3,4),(32.7254896768748,32.8370194186192,32.9360800605226,
33.034988358453,33.0800282649154),.UNSPECIFIED.);
#438=B_SPLINE_CURVE_WITH_KNOTS('',3,(#35614,#35615,#35616,#35617,#35618,
#35619,#35620,#35621,#35622,#35623,#35624,#35625,#35626,#35627,#35628,#35629,
#35630,#35631,#35632,#35633,#35634,#35635,#35636,#35637,#35638,#35639,#35640,
#35641,#35642,#35643,#35644,#35645,#35646,#35647,#35648,#35649,#35650,#35651,
#35652,#35653,#35654,#35655,#35656,#35657,#35658,#35659,#35660,#35661,#35662,
#35663,#35664,#35665,#35666,#35667,#35668,#35669,#35670,#35671,#35672,#35673,
#35674,#35675,#35676,#35677,#35678,#35679,#35680,#35681,#35682,#35683,#35684,
#35685,#35686,#35687,#35688,#35689,#35690,#35691,#35692,#35693,#35694,#35695,
#35696,#35697,#35698,#35699,#35700,#35701,#35702,#35703,#35704,#35705,#35706,
#35707,#35708,#35709,#35710,#35711,#35712,#35713,#35714,#35715,#35716,#35717,
#35718,#35719,#35720,#35721,#35722,#35723,#35724,#35725,#35726,#35727,#35728,
#35729,#35730,#35731,#35732,#35733,#35734,#35735,#35736,#35737,#35738,#35739,
#35740,#35741,#35742,#35743,#35744,#35745,#35746,#35747,#35748,#35749,#35750,
#35751,#35752,#35753,#35754,#35755,#35756,#35757,#35758,#35759,#35760,#35761,
#35762,#35763,#35764,#35765,#35766,#35767,#35768,#35769,#35770,#35771,#35772,
#35773,#35774,#35775,#35776,#35777,#35778,#35779,#35780,#35781,#35782,#35783,
#35784,#35785,#35786,#35787,#35788,#35789,#35790,#35791,#35792,#35793,#35794,
#35795,#35796,#35797,#35798,#35799,#35800,#35801,#35802,#35803,#35804,#35805,
#35806,#35807,#35808,#35809,#35810,#35811,#35812,#35813,#35814,#35815,#35816,
#35817,#35818,#35819,#35820,#35821,#35822,#35823,#35824,#35825,#35826,#35827),
 .UNSPECIFIED.,.F.,.F.,(4,2,2,2,2,2,2,2,2,2,2,2,2,2,2,2,2,2,2,2,2,2,2,2,
2,2,2,2,2,2,2,2,2,2,2,2,2,2,2,2,2,2,2,2,2,2,2,2,2,2,2,2,2,2,2,2,2,2,2,2,
2,2,2,2,2,2,2,2,2,2,2,2,2,2,2,2,2,2,2,2,2,2,2,2,2,2,2,2,2,2,2,2,2,2,2,2,
2,2,2,2,2,2,2,2,2,2,4),(-1.67563146043802,-1.67386340543512,-1.66716963604788,
-1.62004883247232,-1.58613256227116,-1.57812154314721,-1.56164137422588,
-1.55770653562442,-1.55544409047493,-1.55367482768604,-1.55119769607692,
-1.54612013620645,-1.53936756252354,-1.52243077556491,-1.47211079425904,
-1.44161344681044,-1.43468430113439,-1.43065124715619,-1.4271647674396,
-1.42288575641767,-1.41459350625165,-1.40401381610217,-1.37896072319609,
-1.35009178044402,-1.34249707529684,-1.31153884432721,-1.30742659067437,
-1.30490234200958,-1.30294196663873,-1.30063756072213,-1.29640143650009,
-1.27169965427544,-1.22186607519781,-1.19059645293358,-1.18362628927154,
-1.17958411893583,-1.17609853363485,-1.17183171184376,-1.16359860289831,
-1.11906762448112,-1.07207694077685,-1.05889386108005,-1.05519697111931,
-1.05300993992704,-1.05102431851501,-1.04829464233656,-1.04183100449143,
-1.01017901911471,-0.953933685971024,-0.937056764507021,-0.931249132624984,
-0.927500254438264,-0.923947048010284,-0.91912522029482,-0.90790420809942,
-0.853500325655078,-0.812323806393507,-0.805882857328167,-0.803350148009882,
-0.801512740246387,-0.799472878164731,-0.796449742909075,-0.788062982445321,
-0.774898473240685,-0.737603586528475,-0.688961050274329,-0.682277256365227,
-0.677952588488077,-0.674463318632621,-0.670464959340183,-0.663509444542555,
-0.629409107630959,-0.575942090823529,-0.557366179423912,-0.553295455319311,
-0.551002160769359,-0.549040447091492,-0.546500440077176,-0.541096774914267,
-0.533778536942428,-0.514639994577777,-0.449906076524378,-0.434379647271338,
-0.428744882578528,-0.425403933652341,-0.421874459938085,-0.417201654005583,
-0.406839825564649,-0.392738490504648,-0.324253248694902,-0.3061122984198,
-0.302065712893207,-0.299777868167652,-0.297834089769661,-0.295347737666655,
-0.290212683319745,-0.2832643398259,-0.265580625678848,-0.212103045580461,
-0.185437985291434,-0.178669690013046,-0.174711832992602,-0.171567133299975,
-0.167348948614878,-0.15935377467112,-0.130573393771694,-0.0898485202972664),
 .UNSPECIFIED.);
#439=B_SPLINE_CURVE_WITH_KNOTS('',3,(#35833,#35834,#35835,#35836,#35837,
#35838,#35839,#35840,#35841,#35842,#35843,#35844,#35845,#35846,#35847,#35848,
#35849,#35850,#35851,#35852,#35853,#35854,#35855,#35856,#35857,#35858,#35859,
#35860,#35861,#35862,#35863,#35864,#35865,#35866,#35867,#35868,#35869,#35870,
#35871,#35872,#35873,#35874,#35875,#35876,#35877,#35878,#35879,#35880,#35881,
#35882,#35883,#35884,#35885,#35886,#35887,#35888,#35889,#35890,#35891,#35892,
#35893,#35894,#35895,#35896,#35897,#35898,#35899,#35900,#35901,#35902,#35903,
#35904,#35905,#35906,#35907,#35908,#35909,#35910,#35911,#35912,#35913,#35914,
#35915,#35916,#35917,#35918,#35919,#35920,#35921,#35922,#35923,#35924,#35925,
#35926,#35927,#35928,#35929,#35930,#35931,#35932,#35933,#35934,#35935,#35936,
#35937,#35938,#35939,#35940,#35941,#35942,#35943,#35944,#35945,#35946,#35947,
#35948,#35949,#35950,#35951,#35952,#35953,#35954,#35955,#35956,#35957,#35958,
#35959,#35960,#35961,#35962,#35963,#35964,#35965,#35966,#35967,#35968,#35969,
#35970,#35971,#35972,#35973,#35974,#35975,#35976,#35977,#35978,#35979,#35980,
#35981,#35982,#35983,#35984,#35985,#35986,#35987,#35988,#35989,#35990,#35991,
#35992,#35993,#35994,#35995,#35996,#35997,#35998,#35999,#36000,#36001,#36002,
#36003,#36004,#36005,#36006,#36007,#36008,#36009,#36010,#36011,#36012,#36013),
 .UNSPECIFIED.,.F.,.F.,(4,3,3,3,3,3,3,3,3,3,3,3,3,3,3,3,3,3,3,3,3,3,3,3,
3,3,3,3,3,3,3,3,3,3,3,3,3,3,3,3,3,3,3,3,3,3,3,3,3,3,3,3,3,3,3,3,3,3,3,3,
4),(20.512957591123,20.6107155250157,20.7085181868304,20.8064945872437,
20.8962850845758,20.9953442020216,21.0942628761449,21.1938983015117,21.2926403027342,
21.3913498293589,21.4900566671889,21.5903790701615,21.68922766341,21.7902869712447,
21.8913462790794,21.9904053962616,22.0893240701107,22.1889594955448,22.2877014964694,
22.3864110227881,22.4851178603042,22.5854402636239,22.6842888565421,22.7853481650626,
22.8864074735831,22.985466591425,23.0843852659453,23.1840206912129,23.2827626928314,
23.3814722198508,23.4801790580737,23.580501460577,23.6793500542096,23.7804093611482,
23.8814686680867,23.9805277856326,24.0794464598534,24.1790818851955,24.277823886508,
24.37653341322,24.4752402511339,24.575562653998,24.6744112473215,24.7754705549559,
24.8765298625903,24.9755889801305,25.0745076543444,25.1741430796881,25.2728850809916,
25.3715946076934,25.4703014455965,25.5706238484709,25.669472441782,25.7705317494379,
25.8715910570939,25.9728761868512,26.0739977695077,26.1749480071203,26.2757973954954,
26.376561049584,26.4423043696953),.UNSPECIFIED.);
#440=B_SPLINE_CURVE_WITH_KNOTS('',3,(#36014,#36015,#36016,#36017,#36018,
#36019,#36020,#36021,#36022,#36023,#36024,#36025,#36026),.UNSPECIFIED.,
 .F.,.F.,(4,3,3,3,4),(26.4423043699706,26.5495705688098,26.6571264572063,
26.7650823065106,26.7958893988467),.UNSPECIFIED.);
#441=B_SPLINE_CURVE_WITH_KNOTS('',3,(#36028,#36029,#36030,#36031,#36032,
#36033,#36034,#36035,#36036,#36037,#36038,#36039,#36040,#36041,#36042,#36043,
#36044,#36045,#36046,#36047),.UNSPECIFIED.,.F.,.F.,(4,2,2,2,2,2,2,2,2,4),
(-0.0898485202972664,-0.088519391729811,-0.055828355046822,-0.0516951276582153,
-0.0491646822441494,-0.047203825256235,-0.0449039201267464,-0.0424484392440899,
-0.0385816794505213,-0.000734785208168012),.UNSPECIFIED.);
#442=B_SPLINE_CURVE_WITH_KNOTS('',3,(#36048,#36049,#36050,#36051,#36052,
#36053,#36054,#36055,#36056,#36057,#36058,#36059,#36060,#36061,#36062,#36063,
#36064,#36065,#36066,#36067,#36068,#36069,#36070,#36071,#36072,#36073,#36074,
#36075,#36076,#36077,#36078,#36079,#36080,#36081,#36082,#36083,#36084,#36085,
#36086,#36087,#36088,#36089,#36090,#36091,#36092,#36093,#36094,#36095,#36096,
#36097,#36098,#36099,#36100,#36101,#36102,#36103,#36104,#36105,#36106,#36107,
#36108,#36109,#36110,#36111,#36112,#36113,#36114,#36115,#36116,#36117,#36118,
#36119,#36120,#36121,#36122,#36123,#36124,#36125,#36126,#36127,#36128,#36129,
#36130,#36131,#36132,#36133,#36134,#36135,#36136,#36137,#36138,#36139,#36140,
#36141,#36142,#36143,#36144,#36145,#36146,#36147,#36148,#36149,#36150,#36151,
#36152,#36153,#36154,#36155,#36156,#36157,#36158,#36159,#36160,#36161,#36162,
#36163,#36164,#36165,#36166,#36167,#36168,#36169,#36170,#36171,#36172,#36173,
#36174,#36175,#36176,#36177,#36178,#36179,#36180,#36181,#36182,#36183,#36184,
#36185,#36186,#36187,#36188,#36189,#36190,#36191,#36192,#36193,#36194,#36195,
#36196,#36197,#36198,#36199,#36200,#36201,#36202,#36203,#36204,#36205,#36206,
#36207,#36208,#36209,#36210,#36211,#36212,#36213,#36214,#36215,#36216,#36217,
#36218,#36219,#36220,#36221,#36222,#36223,#36224,#36225,#36226,#36227,#36228,
#36229,#36230,#36231,#36232,#36233,#36234,#36235,#36236,#36237,#36238,#36239),
 .UNSPECIFIED.,.F.,.F.,(4,2,2,2,2,2,2,2,2,2,2,2,2,2,2,2,2,2,2,2,2,2,2,2,
2,2,2,2,2,2,2,2,2,2,2,2,2,2,2,2,2,2,2,2,2,2,2,2,2,2,2,2,2,2,2,2,2,2,2,2,
2,2,2,2,2,2,2,2,2,2,2,2,2,2,2,2,2,2,2,2,2,2,2,2,2,2,2,2,2,2,2,2,2,2,2,4),
(-3.17305528611881,-3.12119598485782,-3.10694997652477,-3.09999708888609,
-3.09599853846014,-3.09250811032236,-3.08818072111211,-3.081490309315,-3.03342159340058,
-2.99274582943489,-2.98132422407236,-2.97385514052582,-2.97101260883616,
-2.96897096893944,-2.96713402424151,-2.96411408264857,-2.95637669928287,
-2.8832775912868,-2.85508809567373,-2.84845826867864,-2.84453020763418,
-2.84103095571322,-2.83659838943983,-2.82753227050961,-2.76396187037434,
-2.72693156883095,-2.72154125280845,-2.71900352543636,-2.71704170994051,
-2.71474614698292,-2.71066639720707,-2.69197707082225,-2.63857324484164,
-2.60446818881316,-2.59751135516865,-2.59351234002292,-2.59002256336977,
-2.58569735161569,-2.57901293907899,-2.53684202504075,-2.47981143701736,
-2.47150581351878,-2.46849361347391,-2.46645574528543,-2.46461590921309,
-2.46157953045154,-2.45373928276605,-2.37990453612947,-2.35250493155654,
-2.34592780132056,-2.34201155910593,-2.33851079216589,-2.33405988214605,
-2.3248967722079,-2.26213151552723,-2.2244837019353,-2.21908248588282,-2.21654290289892,
-2.21458116984241,-2.2122874722992,-2.20821510969055,-2.18961572829298,
-2.13613031711779,-2.10202031010675,-2.09506400109957,-2.09106545166044,
-2.08757617756413,-2.08325171325803,-2.0765686952944,-2.0280387753872,-1.99051817903146,
-1.97745807415392,-1.96911862154623,-1.96610204001727,-1.96406351487456,
-1.96222489682589,-1.95968742708636,-1.95321809107746,-1.91469568611194,
-1.87153696877301,-1.84941278137741,-1.84324518000014,-1.83941828947981,
-1.83589577240727,-1.83134946655419,-1.82141478159157,-1.76954856914802,
-1.74010019936102,-1.72660385128643,-1.71806482397902,-1.71502088900458,
-1.71297673750873,-1.71114307354735,-1.70862510368386,-1.7022724913293,
-1.67601819536357),.UNSPECIFIED.);
#443=B_SPLINE_CURVE_WITH_KNOTS('',3,(#36245,#36246,#36247,#36248,#36249,
#36250,#36251,#36252,#36253,#36254,#36255,#36256,#36257,#36258,#36259,#36260,
#36261,#36262,#36263,#36264,#36265,#36266,#36267,#36268,#36269,#36270,#36271,
#36272,#36273,#36274,#36275,#36276,#36277,#36278,#36279,#36280,#36281,#36282,
#36283,#36284,#36285,#36286,#36287,#36288,#36289,#36290,#36291,#36292,#36293,
#36294,#36295,#36296,#36297,#36298,#36299,#36300,#36301,#36302,#36303,#36304,
#36305,#36306,#36307,#36308,#36309,#36310,#36311,#36312,#36313,#36314,#36315,
#36316,#36317,#36318,#36319,#36320,#36321,#36322,#36323,#36324,#36325,#36326,
#36327,#36328,#36329,#36330,#36331,#36332,#36333,#36334,#36335,#36336,#36337,
#36338,#36339,#36340,#36341,#36342,#36343,#36344,#36345,#36346,#36347,#36348,
#36349,#36350,#36351,#36352,#36353,#36354,#36355,#36356,#36357,#36358,#36359,
#36360,#36361,#36362,#36363,#36364,#36365,#36366,#36367,#36368,#36369,#36370,
#36371,#36372,#36373,#36374,#36375,#36376,#36377,#36378,#36379,#36380,#36381,
#36382,#36383,#36384,#36385,#36386,#36387,#36388,#36389,#36390,#36391,#36392,
#36393,#36394,#36395,#36396,#36397,#36398,#36399,#36400,#36401,#36402,#36403,
#36404,#36405,#36406,#36407,#36408,#36409,#36410,#36411,#36412,#36413,#36414,
#36415,#36416,#36417,#36418,#36419,#36420,#36421,#36422),.UNSPECIFIED.,
 .F.,.F.,(4,3,3,3,3,3,3,3,3,3,3,3,3,3,3,3,3,3,3,3,3,3,3,3,3,3,3,3,3,3,3,
3,3,3,3,3,3,3,3,3,3,3,3,3,3,3,3,3,3,3,3,3,3,3,3,3,3,3,3,4),(14.2304071265534,
14.3291482971637,14.4278575780463,14.5265647543816,14.6264030451747,14.7252525926983,
14.8255852551262,14.9259179175542,15.0249770463333,15.1238957322449,15.2235311547215,
15.3222731687617,15.4209827085634,15.5196895599131,15.6200119479492,15.718860555431,
15.8199198337444,15.9209791120578,16.0200382004424,16.1189568450004,16.2185922776956,
16.3173342483389,16.4160437440714,16.5147505507373,16.6150729896934,16.7139215514226,
16.814980928992,16.9160403065614,17.0150994373653,17.1140181250032,17.2136535470109,
17.312395562029,17.411105102524,17.5098119542802,17.6101343409764,17.7089829481464,
17.8100422246057,17.911101501065,18.0101606188399,18.1090792933301,18.2087147186099,
18.30745672029,18.4061662474056,18.504873085759,18.6051954882114,18.704044082059,
18.8051033888138,18.9061626955686,19.005221809666,19.1041404803751,19.2037759065872,
19.3025179042597,19.4012274272912,19.4999342614895,19.6002566686351,19.6991052581938,
19.800164574133,19.9012238900722,20.0301714761758,20.1591190622793),
 .UNSPECIFIED.);
#444=B_SPLINE_CURVE_WITH_KNOTS('',3,(#36423,#36424,#36425,#36426,#36427,
#36428,#36429,#36430,#36431,#36432,#36433,#36434,#36435),.UNSPECIFIED.,
 .F.,.F.,(4,3,3,3,4),(20.1591190625157,20.2568630541379,20.3545467744327,
20.4522206668084,20.512957591123),.UNSPECIFIED.);
#445=B_SPLINE_CURVE_WITH_KNOTS('',3,(#36436,#36437,#36438,#36439,#36440,
#36441,#36442,#36443,#36444,#36445,#36446,#36447,#36448,#36449,#36450,#36451,
#36452,#36453,#36454,#36455,#36456,#36457,#36458,#36459,#36460,#36461,#36462,
#36463,#36464,#36465,#36466,#36467,#36468,#36469,#36470,#36471,#36472,#36473,
#36474,#36475,#36476,#36477,#36478,#36479,#36480,#36481,#36482,#36483,#36484,
#36485,#36486,#36487,#36488,#36489,#36490,#36491,#36492,#36493,#36494,#36495,
#36496,#36497,#36498,#36499,#36500,#36501,#36502,#36503,#36504,#36505,#36506,
#36507,#36508,#36509,#36510,#36511,#36512,#36513,#36514,#36515,#36516,#36517,
#36518,#36519,#36520,#36521,#36522,#36523,#36524,#36525,#36526,#36527,#36528,
#36529,#36530,#36531,#36532,#36533,#36534,#36535,#36536,#36537,#36538,#36539,
#36540,#36541,#36542,#36543,#36544,#36545,#36546,#36547,#36548,#36549,#36550,
#36551,#36552,#36553,#36554,#36555,#36556,#36557,#36558,#36559,#36560,#36561,
#36562,#36563,#36564,#36565,#36566,#36567,#36568,#36569,#36570,#36571,#36572,
#36573,#36574,#36575,#36576,#36577,#36578,#36579,#36580,#36581,#36582,#36583,
#36584,#36585,#36586,#36587,#36588,#36589,#36590,#36591,#36592,#36593,#36594,
#36595,#36596,#36597,#36598,#36599,#36600,#36601,#36602,#36603,#36604,#36605,
#36606,#36607,#36608,#36609,#36610,#36611,#36612,#36613,#36614,#36615,#36616,
#36617,#36618,#36619,#36620,#36621,#36622,#36623,#36624,#36625,#36626,#36627,
#36628,#36629,#36630,#36631,#36632,#36633,#36634,#36635,#36636,#36637,#36638,
#36639,#36640,#36641,#36642,#36643,#36644,#36645),.UNSPECIFIED.,.F.,.F.,
(4,2,2,2,2,2,2,2,2,2,2,2,2,2,2,2,2,2,2,2,2,2,2,2,2,2,2,2,2,2,2,2,2,2,2,
2,2,2,2,2,2,2,2,2,2,2,2,2,2,2,2,2,2,2,2,2,2,2,2,2,2,2,2,2,2,2,2,2,2,2,2,
2,2,2,2,2,2,2,2,2,2,2,2,2,2,2,2,2,2,2,2,2,2,2,2,2,2,2,2,2,2,2,2,2,4),(-1.67601819536357,
-1.65790025499768,-1.61896284412362,-1.60509562768696,-1.59486655864749,
-1.59021745821083,-1.58669143392088,-1.58287567134888,-1.57675893988783,
-1.55519531241609,-1.48395421543031,-1.46857009413773,-1.4647172953657,
-1.46247364218787,-1.46070116686806,-1.45819612567498,-1.4529754007906,
-1.44597622680274,-1.42809635724663,-1.37479644466355,-1.34823059336616,
-1.34146861434871,-1.33751204574301,-1.33436706400397,-1.33014682113187,
-1.32214207392476,-1.31202687293987,-1.28862509419608,-1.25835229108425,
-1.24086345010961,-1.21824854332673,-1.2143351572252,-1.21187038725554,
-1.20991377772064,-1.20756290828643,-1.20310707712571,-1.17062074321288,
-1.12038416497146,-1.09670656245716,-1.09017793969407,-1.08627230939772,
-1.08276959461745,-1.07830049764668,-1.06904232599539,-1.03312176721833,
-1.00178015394779,-0.967567612180327,-0.963427606838462,-0.960895207831793,
-0.958934267849848,-0.956635946957671,-0.952427836578429,-0.928448821204537,
-0.894431230410167,-0.847246193343973,-0.840556552502571,-0.836230258557596,
-0.832741076230961,-0.828744351174761,-0.821795653901332,-0.787833356059805,
-0.735643723495315,-0.715781079097813,-0.711636231704487,-0.709326296461956,
-0.707366653453092,-0.704850326843802,-0.699570167470669,-0.692467608790283,
-0.674183788867987,-0.618574581215839,-0.594565641896955,-0.587995754370924,
-0.584081261981406,-0.580580464692471,-0.57612733547081,-0.566951714772156,
-0.531678367384627,-0.476953464893904,-0.463757039289214,-0.460058964574486,
-0.457871710637919,-0.455886158413932,-0.453157021728804,-0.446696800430247,
-0.415080292744081,-0.358932806466596,-0.341955533618985,-0.336135123207361,
-0.332383491413861,-0.328831597930515,-0.324017674883814,-0.312843500835583,
-0.258969096150844,-0.217169344008483,-0.210749869566655,-0.208220789721541,
-0.206384342851417,-0.204343743325026,-0.201503213626732,-0.194026652308553,
-0.182594928304509,-0.14240303572949,-0.0938347109390278,-0.0902767619888763),
 .UNSPECIFIED.);
#446=B_SPLINE_CURVE_WITH_KNOTS('',3,(#36651,#36652,#36653,#36654,#36655,
#36656,#36657,#36658,#36659,#36660,#36661,#36662,#36663),.UNSPECIFIED.,
 .F.,.F.,(4,3,3,3,4),(-4.20357826990315,-4.10478695491414,-4.00583745897424,
-3.98024477801445,-3.84897440564112),.UNSPECIFIED.);
#447=B_SPLINE_CURVE_WITH_KNOTS('',3,(#36665,#36666,#36667,#36668,#36669,
#36670,#36671,#36672,#36673,#36674,#36675,#36676,#36677,#36678,#36679,#36680,
#36681,#36682,#36683,#36684,#36685,#36686,#36687,#36688,#36689,#36690,#36691,
#36692,#36693,#36694,#36695,#36696,#36697,#36698,#36699,#36700,#36701,#36702,
#36703,#36704,#36705,#36706,#36707,#36708,#36709,#36710,#36711,#36712,#36713,
#36714,#36715,#36716,#36717,#36718,#36719,#36720,#36721,#36722,#36723,#36724,
#36725,#36726,#36727,#36728,#36729,#36730,#36731,#36732,#36733,#36734,#36735,
#36736,#36737,#36738,#36739,#36740,#36741,#36742,#36743,#36744,#36745,#36746,
#36747,#36748,#36749,#36750,#36751,#36752,#36753,#36754,#36755,#36756,#36757,
#36758,#36759,#36760,#36761,#36762,#36763,#36764,#36765,#36766,#36767,#36768,
#36769,#36770,#36771,#36772,#36773,#36774,#36775,#36776,#36777,#36778,#36779,
#36780,#36781,#36782,#36783,#36784,#36785),.UNSPECIFIED.,.F.,.F.,(4,3,3,
3,3,3,3,3,3,3,3,3,3,3,3,3,3,3,3,3,3,3,3,3,3,3,3,3,3,3,3,3,3,3,3,3,3,3,3,
3,4),(-3.84897440539329,-3.75125999555739,-3.65367480658484,-3.55616073132701,
-3.45868648046565,-3.36122081576358,-3.26366927760976,-3.16607558945825,
-3.06831667010992,-2.98518358351084,-2.88604218773156,-2.78703918957161,
-2.68742458950106,-2.58859397716361,-2.48979444543964,-2.39099634432946,
-2.2907778554989,-2.19183589568085,-2.09097914234403,-1.99012238900722,
-1.89201567343051,-1.79404975393482,-1.69417618400592,-1.59638143615237,
-1.49861527802913,-1.40084681613672,-1.29940041072845,-1.2014686750187,
-1.10345750403516,-1.00527923358739,-0.99506119450361,-0.893332626667933,
-0.791764351772391,-0.690356289583907,-0.58904245229151,-0.487798384630709,
-0.386599710304198,-0.28539210708937,-0.184186082512049,-0.0829053445198521,
-3.08113896577085E-14),.UNSPECIFIED.);
#448=B_SPLINE_CURVE_WITH_KNOTS('',3,(#36789,#36790,#36791,#36792,#36793,
#36794,#36795,#36796,#36797,#36798,#36799,#36800,#36801,#36802,#36803,#36804,
#36805,#36806,#36807,#36808,#36809,#36810,#36811,#36812,#36813,#36814,#36815,
#36816,#36817,#36818,#36819,#36820,#36821,#36822,#36823,#36824,#36825,#36826,
#36827,#36828,#36829,#36830,#36831,#36832,#36833,#36834,#36835,#36836,#36837,
#36838,#36839,#36840,#36841,#36842,#36843,#36844,#36845,#36846,#36847,#36848,
#36849,#36850,#36851,#36852,#36853,#36854,#36855,#36856,#36857,#36858,#36859,
#36860,#36861,#36862,#36863,#36864,#36865,#36866,#36867,#36868,#36869,#36870,
#36871,#36872,#36873,#36874,#36875,#36876,#36877,#36878,#36879,#36880,#36881,
#36882,#36883,#36884,#36885,#36886,#36887,#36888,#36889,#36890,#36891,#36892,
#36893,#36894,#36895,#36896,#36897,#36898,#36899,#36900,#36901,#36902,#36903,
#36904,#36905,#36906,#36907,#36908,#36909,#36910,#36911,#36912,#36913,#36914,
#36915,#36916,#36917,#36918,#36919,#36920,#36921,#36922,#36923,#36924,#36925,
#36926,#36927,#36928,#36929,#36930,#36931,#36932,#36933,#36934,#36935,#36936,
#36937,#36938,#36939,#36940,#36941,#36942,#36943,#36944,#36945,#36946,#36947,
#36948,#36949,#36950,#36951,#36952,#36953,#36954,#36955,#36956,#36957,#36958,
#36959,#36960),.UNSPECIFIED.,.F.,.F.,(4,3,3,3,3,3,3,3,3,3,3,3,3,3,3,3,3,
3,3,3,3,3,3,3,3,3,3,3,3,3,3,3,3,3,3,3,3,3,3,3,3,3,3,3,3,3,3,3,3,3,3,3,3,
3,3,3,3,4),(2.01695560162626,2.11564189726858,2.21418829647648,2.31262230469899,
2.41099520084271,2.50933729039148,2.60767884072445,2.70611518766494,2.80459906192678,
2.9032524542413,2.98518358351084,3.08440364663108,3.18348650423872,3.28308128846069,
3.3819941430274,3.48087664382076,3.57975834074699,3.67987995006385,3.77890625693714,
3.87957551747579,3.98024477801444,4.07919428955199,4.1780018264564,4.27766484471411,
4.37629277757328,4.47488738556402,4.57347860632559,4.67393544787371,4.77266786606485,
4.87398691929145,4.97530597251806,5.07438444725685,5.17332252305007,5.27295310354652,
5.37171446613478,5.47044329472867,5.56916934814539,5.66946880286446,5.76833619817666,
5.86935168259916,5.97036716702167,6.06944373196721,6.16838022720496,6.268011243995,
6.36677184867722,6.46550023158715,6.56422615356924,6.66452670555825,6.76339475286863,
6.86441155719695,6.96542836152528,7.06514996643927,7.16472649372704,7.26418682012562,
7.36355392634545,7.46286736071847,7.56216603022671,7.59274844815647),
 .UNSPECIFIED.);
#449=B_SPLINE_CURVE_WITH_KNOTS('',3,(#36961,#36962,#36963,#36964,#36965,
#36966,#36967,#36968,#36969,#36970,#36971,#36972,#36973),.UNSPECIFIED.,
 .F.,.F.,(4,3,3,3,4),(7.59274844852976,7.7041800085765,7.8161317130083,
7.928691988329,7.9466267193592),.UNSPECIFIED.);
#450=B_SPLINE_CURVE_WITH_KNOTS('',3,(#36976,#36977,#36978,#36979,#36980,
#36981,#36982,#36983,#36984,#36985,#36986,#36987,#36988,#36989,#36990,#36991,
#36992,#36993,#36994,#36995,#36996,#36997,#36998,#36999,#37000,#37001,#37002,
#37003,#37004,#37005,#37006,#37007,#37008,#37009,#37010,#37011,#37012,#37013,
#37014,#37015,#37016,#37017,#37018,#37019,#37020,#37021,#37022,#37023,#37024,
#37025,#37026,#37027,#37028,#37029,#37030,#37031,#37032,#37033,#37034,#37035,
#37036,#37037,#37038,#37039,#37040,#37041,#37042,#37043,#37044,#37045,#37046,
#37047,#37048,#37049,#37050,#37051,#37052,#37053,#37054,#37055,#37056,#37057,
#37058,#37059,#37060,#37061,#37062,#37063,#37064,#37065,#37066,#37067,#37068,
#37069,#37070,#37071,#37072,#37073,#37074,#37075,#37076,#37077,#37078,#37079,
#37080,#37081,#37082,#37083,#37084,#37085,#37086,#37087,#37088,#37089,#37090,
#37091,#37092,#37093,#37094,#37095,#37096,#37097,#37098,#37099,#37100,#37101,
#37102,#37103,#37104,#37105,#37106,#37107,#37108,#37109,#37110,#37111,#37112,
#37113,#37114,#37115,#37116,#37117,#37118,#37119,#37120,#37121,#37122,#37123,
#37124,#37125,#37126,#37127,#37128,#37129,#37130,#37131,#37132,#37133,#37134,
#37135,#37136,#37137,#37138,#37139,#37140,#37141,#37142,#37143,#37144,#37145,
#37146,#37147,#37148,#37149,#37150,#37151,#37152,#37153,#37154,#37155,#37156,
#37157,#37158,#37159),.UNSPECIFIED.,.F.,.F.,(4,3,3,3,3,3,3,3,3,3,3,3,3,
3,3,3,3,3,3,3,3,3,3,3,3,3,3,3,3,3,3,3,3,3,3,3,3,3,3,3,3,3,3,3,3,3,3,3,3,
3,3,3,3,3,3,3,3,3,3,3,3,4),(7.9466267193592,7.96048955602889,8.05955222869409,
8.15847448196122,8.25810901553263,8.35685462726907,8.45556776802807,8.55427821863936,
8.65459635161265,8.75344851699117,8.85449963376183,8.9555507505325,9.05461163472714,
9.15353211785238,9.25316709625034,9.35191099658619,9.450622452008,9.54933124579016,
9.64965142060165,9.74850201721232,9.84955698112422,9.95061194503612,10.0496691800778,
10.148585942413,10.2482218420539,10.3469618738397,10.4456694137526,10.544374250258,
10.6446989725784,10.7435455487723,10.844609344156,10.9456731395397,11.0447328420797,
11.1436521066727,11.243287385094,11.3420299854808,11.4407401131877,11.5394475531969,
11.6397692484085,11.738618440354,11.8396763871987,11.9407343340433,12.039793611144,
12.1387124494771,12.2383478343608,12.3370900097446,12.4357997138898,12.5345067323694,
12.6348289314138,12.7336777112374,12.8347366198922,12.9357955285469,13.0340412306013,
13.1321472235822,13.2301416920862,13.3280762000881,13.4259815616605,13.5238885532223,
13.6218885616932,13.7199390884583,13.8181477780583,13.875933755129),
 .UNSPECIFIED.);
#451=B_SPLINE_CURVE_WITH_KNOTS('',3,(#37160,#37161,#37162,#37163,#37164,
#37165,#37166,#37167,#37168,#37169,#37170,#37171,#37172),.UNSPECIFIED.,
 .F.,.F.,(4,3,3,3,4),(13.8759337553361,13.9308567230506,14.0299036910203,
14.1301554087868,14.2304071265534),.UNSPECIFIED.);
#452=B_SPLINE_CURVE_WITH_KNOTS('',3,(#37174,#37175,#37176,#37177,#37178,
#37179,#37180,#37181,#37182,#37183,#37184,#37185,#37186,#37187,#37188,#37189),
 .UNSPECIFIED.,.F.,.F.,(4,2,2,2,2,2,2,4),(-0.0902767619888763,-0.0871517738827283,
-0.0828276961846434,-0.0793389329993606,-0.0753411934293112,-0.0683868759572198,
-0.0544509421788097,-0.000738945914559194),.UNSPECIFIED.);
#453=B_SPLINE_CURVE_WITH_KNOTS('',3,(#37190,#37191,#37192,#37193,#37194,
#37195,#37196,#37197,#37198,#37199,#37200,#37201,#37202,#37203,#37204,#37205,
#37206,#37207,#37208,#37209,#37210,#37211,#37212,#37213,#37214,#37215,#37216,
#37217,#37218,#37219,#37220,#37221,#37222,#37223,#37224,#37225,#37226,#37227,
#37228,#37229,#37230,#37231,#37232,#37233,#37234,#37235,#37236,#37237,#37238,
#37239,#37240,#37241,#37242,#37243,#37244,#37245,#37246,#37247,#37248,#37249,
#37250,#37251,#37252,#37253,#37254,#37255,#37256,#37257,#37258,#37259,#37260,
#37261,#37262,#37263,#37264,#37265,#37266,#37267,#37268,#37269,#37270,#37271,
#37272,#37273,#37274,#37275,#37276,#37277,#37278,#37279,#37280,#37281,#37282,
#37283,#37284,#37285,#37286,#37287,#37288,#37289,#37290,#37291,#37292,#37293,
#37294,#37295,#37296,#37297,#37298,#37299,#37300,#37301,#37302,#37303,#37304,
#37305,#37306,#37307,#37308,#37309,#37310,#37311,#37312,#37313,#37314,#37315,
#37316,#37317,#37318,#37319,#37320,#37321,#37322,#37323,#37324,#37325,#37326,
#37327,#37328,#37329,#37330,#37331,#37332,#37333,#37334,#37335,#37336,#37337,
#37338,#37339,#37340,#37341,#37342,#37343,#37344,#37345,#37346,#37347,#37348,
#37349,#37350,#37351,#37352,#37353,#37354,#37355,#37356,#37357,#37358,#37359,
#37360,#37361,#37362,#37363,#37364,#37365,#37366,#37367,#37368,#37369,#37370),
 .UNSPECIFIED.,.F.,.F.,(4,3,3,3,3,3,3,3,3,3,3,3,3,3,3,3,3,3,3,3,3,3,3,3,
3,3,3,3,3,3,3,3,3,3,3,3,3,3,3,3,3,3,3,3,3,3,3,3,3,3,3,3,3,3,3,3,3,3,3,3,
4),(-10.1321597128208,-9.98380287347192,-9.95061194503611,-9.85155080805362,
-9.75263012655875,-9.65299520455547,-9.55425123974632,-9.45553977016634,
-9.3568310125024,-9.25651094700993,-9.15766050991737,-9.05660563022494,
-8.95555075053251,-8.85648813509386,-8.75756592802855,-8.6579313815286,
-8.55918578882376,-8.46047265687315,-8.36176220484683,-8.26144404264234,
-8.1625918506966,-8.06154070336275,-7.96048955602889,-7.86144585639168,
-7.76254262764497,-7.66290334438001,-7.56417674344362,-7.46548256638777,
-7.3667910070416,-7.26645034566252,-7.16761670121533,-7.06652253137031,
-6.96542836152528,-6.8663497016468,-6.76741156214399,-6.6677810127537,-6.56901987256432,
-6.47029137085155,-6.37156574645098,-6.27126610159365,-6.1723993736445,
-6.07138327033308,-5.97036716702167,-5.87128979664853,-5.77235259505363,
-5.67272176723669,-5.57396071232545,-5.47523197841698,-5.37650580681207,
-5.27620584823857,-5.17733781201762,-5.07632189226784,-4.97530597251806,
-4.87639029978064,-4.7776031596478,-4.67891439036993,-4.58029393416826,
-4.4816847956452,-4.38308674516142,-4.28441542602605,-4.20357826990315),
 .UNSPECIFIED.);
#454=B_SPLINE_CURVE_WITH_KNOTS('',3,(#37373,#37374,#37375,#37376,#37377,
#37378,#37379,#37380),.UNSPECIFIED.,.F.,.F.,(4,1,1,1,1,4),(17.9343967671566,
18.824417223833,19.8194784183366,20.8145396128402,21.8096008073438,21.9911485751284),
 .UNSPECIFIED.);
#455=B_SPLINE_CURVE_WITH_KNOTS('',3,(#37381,#37382,#37383,#37384,#37385,
#37386),.UNSPECIFIED.,.F.,.F.,(4,1,1,4),(21.9911485751284,22.8046620018474,
23.799723196351,24.2174104409543),.UNSPECIFIED.);
#456=B_SPLINE_CURVE_WITH_KNOTS('',3,(#37388,#37389,#37390,#37391,#37392,
#37393,#37394,#37395,#37396,#37397,#37398,#37399,#37400,#37401,#37402,#37403,
#37404,#37405,#37406,#37407,#37408,#37409,#37410,#37411,#37412,#37413,#37414,
#37415,#37416,#37417,#37418,#37419,#37420,#37421,#37422,#37423,#37424,#37425,
#37426,#37427,#37428,#37429,#37430,#37431,#37432,#37433,#37434,#37435,#37436,
#37437,#37438,#37439,#37440,#37441,#37442,#37443,#37444,#37445,#37446,#37447,
#37448,#37449,#37450,#37451,#37452,#37453,#37454,#37455,#37456,#37457,#37458,
#37459,#37460,#37461,#37462,#37463),.UNSPECIFIED.,.F.,.F.,(4,3,3,3,3,3,
3,3,3,3,3,3,3,3,3,3,3,3,3,3,3,3,3,3,3,4),(21.9911485753542,22.0971791978026,
22.2036796189916,22.3107685681831,22.3588896830007,22.453131598846,22.5472457024974,
22.6412605386286,22.7352081181162,22.8291214907904,22.9230263020776,23.0169481830416,
23.110971268134,23.2050498822345,23.2992804751442,23.3539508775043,23.4481997979404,
23.5442351803674,23.638238265709,23.7321788858051,23.8260827259759,23.9236827588209,
24.0176263675221,24.1116026174092,24.2056723410817,24.216482857356),
 .UNSPECIFIED.);
#457=B_SPLINE_CURVE_WITH_KNOTS('',3,(#37464,#37465,#37466,#37467,#37468,
#37469,#37470,#37471,#37472,#37473,#37474,#37475,#37476,#37477,#37478,#37479,
#37480,#37481,#37482,#37483,#37484,#37485,#37486,#37487,#37488,#37489,#37490,
#37491,#37492,#37493,#37494,#37495,#37496,#37497,#37498,#37499,#37500,#37501,
#37502,#37503,#37504,#37505,#37506,#37507,#37508,#37509,#37510,#37511,#37512,
#37513,#37514,#37515,#37516,#37517,#37518,#37519,#37520,#37521,#37522,#37523,
#37524,#37525,#37526,#37527,#37528,#37529,#37530,#37531,#37532,#37533,#37534,
#37535,#37536,#37537,#37538,#37539,#37540,#37541,#37542,#37543,#37544,#37545,
#37546,#37547,#37548,#37549,#37550,#37551,#37552,#37553,#37554,#37555,#37556,
#37557,#37558,#37559,#37560,#37561,#37562,#37563,#37564,#37565,#37566,#37567,
#37568,#37569,#37570,#37571,#37572,#37573,#37574,#37575,#37576,#37577,#37578,
#37579,#37580,#37581,#37582,#37583,#37584,#37585,#37586,#37587,#37588,#37589,
#37590,#37591,#37592,#37593,#37594,#37595,#37596,#37597,#37598,#37599),
 .UNSPECIFIED.,.F.,.F.,(4,3,3,3,3,3,3,3,3,3,3,3,3,3,3,3,3,3,3,3,3,3,3,3,
3,3,3,3,3,3,3,3,3,3,3,3,3,3,3,3,3,3,3,3,3,4),(17.9336096034474,18.0276908933547,
18.1218726198763,18.2161072832475,18.3104984450518,18.3786449049863,18.4727791665438,
18.566784204418,18.6606887201774,18.7545245606333,18.8483253559992,18.9421168868663,
19.0359249189042,19.1298339751119,19.2237982875258,19.3179152766156,19.3737060994899,
19.4679630484211,19.5620922042144,19.6561220902177,19.7500846514864,19.8440129578934,
19.9379326359175,20.0318692976143,20.1259069400813,20.2200000068637,20.3142447427367,
20.3687672939935,20.4630224260692,20.5571500629404,20.6511787288197,20.7451405242449,
20.8390683466272,20.9329878241461,21.0269245707971,21.1209627371732,21.2150565766248,
21.3093024733283,21.3638284884971,21.4586972705057,21.5534341189419,21.6480638995539,
21.7426049418883,21.8370934443179,21.9315675426925,21.9911485751284),
 .UNSPECIFIED.);
#458=B_SPLINE_CURVE_WITH_KNOTS('',3,(#37602,#37603,#37604,#37605,#37606,
#37607,#37608,#37609,#37610,#37611,#37612,#37613,#37614,#37615,#37616,#37617,
#37618,#37619,#37620,#37621,#37622,#37623,#37624,#37625,#37626,#37627,#37628,
#37629,#37630,#37631,#37632,#37633,#37634,#37635,#37636,#37637,#37638,#37639,
#37640,#37641,#37642,#37643,#37644,#37645,#37646,#37647,#37648,#37649,#37650,
#37651,#37652,#37653,#37654,#37655,#37656,#37657,#37658,#37659,#37660,#37661,
#37662,#37663,#37664,#37665,#37666,#37667,#37668,#37669,#37670,#37671,#37672,
#37673,#37674,#37675,#37676,#37677,#37678,#37679,#37680,#37681,#37682,#37683,
#37684,#37685,#37686,#37687,#37688,#37689,#37690,#37691,#37692,#37693,#37694,
#37695,#37696,#37697,#37698,#37699,#37700,#37701,#37702,#37703,#37704,#37705,
#37706,#37707,#37708,#37709,#37710,#37711,#37712,#37713,#37714,#37715,#37716,
#37717,#37718,#37719,#37720,#37721,#37722,#37723,#37724,#37725,#37726,#37727,
#37728,#37729,#37730,#37731,#37732,#37733,#37734,#37735,#37736,#37737,#37738,
#37739,#37740,#37741,#37742,#37743,#37744,#37745,#37746,#37747,#37748,#37749,
#37750,#37751,#37752,#37753,#37754,#37755,#37756,#37757,#37758,#37759,#37760,
#37761,#37762,#37763,#37764,#37765,#37766,#37767,#37768,#37769,#37770,#37771,
#37772,#37773,#37774,#37775,#37776,#37777,#37778,#37779,#37780,#37781,#37782,
#37783,#37784,#37785),.UNSPECIFIED.,.F.,.F.,(4,3,3,3,3,3,3,3,3,3,3,3,3,
3,3,3,3,3,3,3,3,3,3,3,3,3,3,3,3,3,3,3,3,3,3,3,3,3,3,3,3,3,3,3,3,3,3,3,3,
3,3,3,3,3,3,3,3,3,3,3,3,4),(7.94663621176237,7.96048955602889,8.05955426029293,
8.15847856564649,8.25811258875724,8.35686028739783,8.45557552348595,8.5542880750255,
8.65460374390225,8.75345800260633,8.85450437656942,8.9555507505325,9.05461196409969,
9.15353278770629,9.25316768237252,9.35191194799743,9.45062377725602,9.54933295295884,
9.64965270097816,9.74850369575663,9.84955782039637,9.95061194503612,10.0496683369466,
10.1485842429707,10.2482203550418,10.3469595045535,10.4456661543797,10.5443700941613,
10.6446958555059,10.7435415276227,10.8446073335812,10.9456731395397,11.0447332366077,
11.1436529000012,11.2432880792565,11.3420310859267,11.4407416218237,11.5394494713804,
11.6397706870461,11.738620287719,11.8396773108812,11.9407343340433,12.0397936403621,
12.1387125095246,12.2383478869024,12.3370900968523,12.4357998368967,12.5345068925667,
12.6348290515617,12.7336778714118,12.8347366999794,12.9357955285469,13.0340410984849,
13.1321469572857,13.2301412890246,13.32807565869,13.4259808804952,13.5238877309982,
13.6218875972222,13.7199379808394,13.8181465272218,13.8759337551308),
 .UNSPECIFIED.);
#459=B_SPLINE_CURVE_WITH_KNOTS('',3,(#37786,#37787,#37788,#37789,#37790,
#37791,#37792,#37793,#37794,#37795,#37796,#37797,#37798),.UNSPECIFIED.,
 .F.,.F.,(4,3,3,3,4),(13.8759337553362,13.9308567230506,14.0299037614613,
14.1301606402168,14.2304175189723),.UNSPECIFIED.);
#460=B_SPLINE_CURVE_WITH_KNOTS('',3,(#37799,#37800,#37801,#37802,#37803,
#37804,#37805,#37806,#37807,#37808,#37809,#37810,#37811,#37812,#37813,#37814,
#37815,#37816,#37817,#37818,#37819,#37820,#37821,#37822,#37823,#37824,#37825,
#37826,#37827,#37828,#37829,#37830,#37831,#37832,#37833,#37834,#37835,#37836,
#37837,#37838,#37839,#37840,#37841,#37842,#37843,#37844,#37845,#37846,#37847,
#37848,#37849,#37850,#37851,#37852,#37853,#37854,#37855,#37856,#37857,#37858,
#37859,#37860,#37861,#37862,#37863,#37864,#37865,#37866,#37867,#37868,#37869,
#37870,#37871,#37872,#37873,#37874,#37875,#37876,#37877,#37878,#37879,#37880,
#37881,#37882,#37883,#37884,#37885,#37886,#37887,#37888,#37889,#37890,#37891,
#37892,#37893,#37894,#37895,#37896,#37897,#37898,#37899,#37900,#37901,#37902,
#37903,#37904,#37905,#37906,#37907,#37908,#37909,#37910,#37911,#37912,#37913,
#37914,#37915,#37916,#37917,#37918,#37919,#37920,#37921,#37922,#37923,#37924,
#37925,#37926,#37927,#37928,#37929,#37930,#37931,#37932,#37933,#37934,#37935,
#37936,#37937,#37938,#37939,#37940,#37941,#37942,#37943,#37944,#37945,#37946,
#37947,#37948,#37949,#37950,#37951,#37952,#37953,#37954,#37955,#37956,#37957,
#37958,#37959,#37960,#37961,#37962,#37963,#37964,#37965,#37966,#37967,#37968,
#37969,#37970,#37971,#37972,#37973,#37974,#37975,#37976,#37977,#37978,#37979,
#37980,#37981,#37982,#37983,#37984,#37985,#37986,#37987,#37988,#37989,#37990,
#37991,#37992,#37993,#37994,#37995,#37996,#37997,#37998,#37999,#38000,#38001,
#38002,#38003,#38004,#38005,#38006,#38007,#38008,#38009,#38010,#38011,#38012,
#38013,#38014),.UNSPECIFIED.,.F.,.F.,(4,2,2,2,2,2,2,2,2,2,2,2,2,2,2,2,2,
2,2,2,2,2,2,2,2,2,2,2,2,2,2,2,2,2,2,2,2,2,2,2,2,2,2,2,2,2,2,2,2,2,2,2,2,
2,2,2,2,2,2,2,2,2,2,2,2,2,2,2,2,2,2,2,2,2,2,2,2,2,2,2,2,2,2,2,2,2,2,2,2,
2,2,2,2,2,2,2,2,2,2,2,2,2,2,2,2,2,2,4),(-1.67566337115906,-1.67120280065352,
-1.66726462128888,-1.66376769450309,-1.6593533715074,-1.65037907026849,
-1.58608340457434,-1.54833271630198,-1.54422098019783,-1.54169685999936,
-1.53973643199843,-1.53743177573583,-1.53319487640862,-1.50847890562579,
-1.45861073239527,-1.42736542077124,-1.42039558024787,-1.41635304716419,
-1.41286681818005,-1.4085987839144,-1.40036193884745,-1.35513827352513,
-1.30690664318352,-1.29535139711433,-1.29182033823835,-1.28966953119213,
-1.28766728590246,-1.28484499900533,-1.27782445047594,-1.26749550757044,
-1.2337952532973,-1.18093350517499,-1.17103122946286,-1.16648914127488,
-1.16296548088014,-1.15913288833492,-1.15294607384776,-1.13063081054186,
-1.08678693108625,-1.07049635409441,-1.0596647395255,-1.0448694921111,-1.0410267620009,
-1.0388072323975,-1.03683256472885,-1.03417153449766,-1.02809754080505,
-1.00030329743465,-0.980650030647354,-0.92985854140192,-0.919893440014821,
-0.915343865946071,-0.911823267533509,-0.908002954572419,-0.901856027950359,
-0.87992633456036,-0.837456771983163,-0.79801271437362,-0.791575854261773,
-0.789044804597,-0.787208692572457,-0.785169324595953,-0.782147444534211,
-0.773768467704869,-0.760621899397138,-0.723106531134634,-0.67453467344312,
-0.667845909333403,-0.663518345032452,-0.660026956015257,-0.656026387260442,
-0.649067493270492,-0.614943041357905,-0.583937145289183,-0.565893892558729,
-0.543422439879807,-0.539511130531841,-0.537045046536865,-0.535082597996337,
-0.532717497650554,-0.528224751178082,-0.494449832370743,-0.440408974454265,
-0.421425209527758,-0.415353353066085,-0.411540367366554,-0.407999540220032,
-0.403304853582722,-0.392864074507233,-0.378634910208049,-0.308664620705708,
-0.291943317772405,-0.287990326349166,-0.285723052767593,-0.283785578936228,
-0.281289562982911,-0.276005321504606,-0.268808352370668,-0.250107053490611,
-0.191316020790503,-0.170087279042834,-0.163801700873181,-0.159966627906554,
-0.156479460721741,-0.151963516330361,-0.142356961979044,-0.10337591065964,
-0.0899054331255484),.UNSPECIFIED.);
#461=B_SPLINE_CURVE_WITH_KNOTS('',3,(#38017,#38018,#38019,#38020,#38021,
#38022,#38023,#38024),.UNSPECIFIED.,.F.,.F.,(4,1,1,1,1,4),(17.9344061060102,
18.824417223833,19.8194784183366,20.8145396128402,21.8096008073438,21.9911485751285),
 .UNSPECIFIED.);
#462=B_SPLINE_CURVE_WITH_KNOTS('',3,(#38025,#38026,#38027,#38028,#38029,
#38030),.UNSPECIFIED.,.F.,.F.,(4,1,1,4),(21.9911485751285,22.8046620018475,
23.7997231963511,24.2174208605652),.UNSPECIFIED.);
#463=B_SPLINE_CURVE_WITH_KNOTS('',3,(#38032,#38033,#38034,#38035,#38036,
#38037,#38038,#38039,#38040,#38041,#38042,#38043,#38044,#38045,#38046,#38047,
#38048,#38049,#38050,#38051,#38052,#38053,#38054,#38055,#38056,#38057,#38058,
#38059,#38060,#38061,#38062,#38063,#38064,#38065,#38066,#38067,#38068,#38069,
#38070,#38071,#38072,#38073,#38074,#38075,#38076,#38077,#38078,#38079,#38080,
#38081,#38082,#38083,#38084,#38085,#38086,#38087,#38088,#38089,#38090,#38091,
#38092,#38093,#38094,#38095,#38096,#38097,#38098,#38099,#38100,#38101,#38102,
#38103,#38104,#38105,#38106,#38107),.UNSPECIFIED.,.F.,.F.,(4,3,3,3,3,3,
3,3,3,3,3,3,3,3,3,3,3,3,3,3,3,3,3,3,3,4),(21.9911485753567,22.0971717254703,
22.2036644377552,22.3107455936571,22.3588896830007,22.4531335315797,22.5472495865776,
22.6412663898706,22.7352159519276,22.8291313159636,22.9230381249701,23.0169620075806,
23.1109870881314,23.2050676971499,23.2993002644203,23.3539508775043,23.448200109615,
23.5442368061655,23.6382402270581,23.73218119163,23.8260853847912,23.9236874590982,
24.0176314416696,24.1116080720406,24.2056781869892,24.2164936820193),
 .UNSPECIFIED.);
#464=B_SPLINE_CURVE_WITH_KNOTS('',3,(#38108,#38109,#38110,#38111,#38112,
#38113,#38114,#38115,#38116,#38117,#38118,#38119,#38120,#38121,#38122,#38123,
#38124,#38125,#38126,#38127,#38128,#38129,#38130,#38131,#38132,#38133,#38134,
#38135,#38136,#38137,#38138,#38139,#38140,#38141,#38142,#38143,#38144,#38145,
#38146,#38147,#38148,#38149,#38150,#38151,#38152,#38153,#38154,#38155,#38156,
#38157,#38158,#38159,#38160,#38161,#38162,#38163,#38164,#38165,#38166,#38167,
#38168,#38169,#38170,#38171,#38172,#38173,#38174,#38175,#38176,#38177,#38178,
#38179,#38180,#38181,#38182,#38183,#38184,#38185,#38186,#38187,#38188,#38189,
#38190,#38191,#38192,#38193,#38194,#38195,#38196,#38197,#38198,#38199,#38200,
#38201,#38202,#38203,#38204,#38205,#38206,#38207,#38208,#38209,#38210,#38211,
#38212,#38213,#38214,#38215,#38216,#38217,#38218,#38219,#38220,#38221,#38222,
#38223,#38224,#38225,#38226,#38227,#38228,#38229,#38230,#38231,#38232,#38233,
#38234,#38235,#38236,#38237,#38238,#38239,#38240,#38241,#38242,#38243),
 .UNSPECIFIED.,.F.,.F.,(4,3,3,3,3,3,3,3,3,3,3,3,3,3,3,3,3,3,3,3,3,3,3,3,
3,3,3,3,3,3,3,3,3,3,3,3,3,3,3,3,3,3,3,3,3,4),(17.9336209525117,18.0277115439587,
18.1219027474085,18.2161469932096,18.3105478396887,18.3786449049862,18.4727572299532,
18.5667400362569,18.6606220561052,18.7544350950428,18.8482129069823,18.9419812987881,
19.0357660622794,19.12965178978,19.223592703853,19.3176864139379,19.3737060994898,
19.4679725846016,19.5621113667816,19.6561509555016,19.7501232927928,19.8440614168356,
19.9379909420193,20.0319374683321,20.1259849418975,20.2200878353086,20.3143422937485,
20.3687672939934,20.4630245655481,20.5571543984776,20.6511853137657,20.7451494294165,
20.8390796150494,20.9330014961429,21.0269406840253,21.1209813348621,21.2150776868747,
21.309326116205,21.3638284884971,21.4586930400753,21.5534255947856,21.6480510252089,
21.7425876513507,21.8370717007576,21.9315413125657,21.9911485751285),
 .UNSPECIFIED.);
#465=B_SPLINE_CURVE_WITH_KNOTS('',3,(#38245,#38246,#38247,#38248,#38249,
#38250,#38251,#38252,#38253,#38254,#38255,#38256,#38257,#38258,#38259,#38260,
#38261,#38262,#38263,#38264,#38265,#38266,#38267,#38268,#38269,#38270,#38271,
#38272,#38273,#38274,#38275,#38276,#38277,#38278,#38279,#38280,#38281,#38282,
#38283,#38284,#38285,#38286,#38287,#38288,#38289,#38290,#38291,#38292,#38293,
#38294,#38295,#38296,#38297,#38298,#38299,#38300,#38301,#38302,#38303,#38304,
#38305,#38306,#38307,#38308,#38309,#38310,#38311,#38312,#38313,#38314,#38315,
#38316,#38317,#38318,#38319,#38320,#38321,#38322,#38323,#38324,#38325,#38326,
#38327,#38328,#38329,#38330,#38331,#38332),.UNSPECIFIED.,.F.,.F.,(4,3,3,
3,3,3,3,3,3,3,3,3,3,3,3,3,3,3,3,3,3,3,3,3,3,3,3,3,3,4),(-0.569248610399504,
-0.543620267538966,-0.517275308318863,-0.510365772288032,-0.504797425837249,
-0.476915498166719,-0.449033570496189,-0.44252399619976,-0.414641409554834,
-0.386493730355128,-0.358554115912246,-0.344587775116203,-0.340093641025723,
-0.311161006381323,-0.302297526319618,-0.274516016182276,-0.24600118036232,
-0.234427379674768,-0.228081846962352,-0.199138916344677,-0.169673832321506,
-0.139875499189353,-0.12331359040414,-0.118150586823425,-0.113404796669263,
-0.082855962759546,-0.0522791701779296,-0.0223319110835381,-0.00827276376604753,
-4.5575133329622E-5),.UNSPECIFIED.);
#466=B_SPLINE_CURVE_WITH_KNOTS('',3,(#38333,#38334,#38335,#38336,#38337,
#38338,#38339,#38340,#38341,#38342,#38343,#38344,#38345,#38346,#38347,#38348,
#38349,#38350,#38351,#38352,#38353,#38354,#38355,#38356,#38357,#38358,#38359,
#38360,#38361,#38362,#38363,#38364,#38365,#38366,#38367,#38368,#38369,#38370,
#38371,#38372,#38373,#38374,#38375,#38376,#38377,#38378,#38379,#38380,#38381,
#38382,#38383,#38384,#38385,#38386,#38387,#38388,#38389,#38390,#38391,#38392,
#38393,#38394,#38395,#38396,#38397,#38398,#38399,#38400,#38401,#38402,#38403,
#38404,#38405,#38406,#38407,#38408,#38409,#38410,#38411,#38412,#38413,#38414,
#38415,#38416,#38417,#38418,#38419,#38420,#38421,#38422,#38423,#38424,#38425,
#38426),.UNSPECIFIED.,.F.,.F.,(4,3,3,3,3,3,3,3,3,3,3,3,3,3,3,3,3,3,3,3,
3,3,3,3,3,3,3,3,3,3,3,4),(-0.566847306048012,-0.536671615274114,-0.508620133545833,
-0.497368804130827,-0.489151108516999,-0.459017262376303,-0.429054732234886,
-0.424465688360989,-0.419732324172897,-0.390343746603834,-0.361246162165409,
-0.332930307421861,-0.318054544345632,-0.31168393575571,-0.307251657998185,
-0.279282126811528,-0.273681209148948,-0.244539503877978,-0.215397798607007,
-0.20526406080706,-0.200835933876738,-0.173001262381593,-0.145191835190121,
-0.117980004611901,-0.104040576094789,-0.0999820633207585,-0.0958220791342219,
-0.0691487206705904,-0.0429261084718551,-0.0175178608047413,-0.00680668378120295,
0.),.UNSPECIFIED.);
#467=B_SPLINE_CURVE_WITH_KNOTS('',3,(#38927,#38928,#38929,#38930,#38931,
#38932,#38933,#38934,#38935,#38936,#38937,#38938,#38939,#38940,#38941,#38942,
#38943,#38944,#38945,#38946,#38947,#38948,#38949,#38950,#38951,#38952,#38953,
#38954,#38955,#38956,#38957,#38958,#38959,#38960,#38961,#38962,#38963,#38964,
#38965,#38966,#38967,#38968,#38969,#38970,#38971,#38972,#38973,#38974,#38975,
#38976,#38977,#38978,#38979,#38980,#38981,#38982,#38983,#38984,#38985,#38986,
#38987,#38988,#38989,#38990,#38991,#38992,#38993,#38994,#38995,#38996,#38997,
#38998,#38999,#39000,#39001,#39002,#39003,#39004,#39005,#39006,#39007,#39008,
#39009,#39010,#39011,#39012,#39013,#39014),.UNSPECIFIED.,.F.,.F.,(4,3,3,
3,3,3,3,3,3,3,3,3,3,3,3,3,3,3,3,3,3,3,3,3,3,3,3,3,3,4),(2.82480432200989E-15,
0.0255907113803957,0.0517115692667785,0.0784881552197149,0.0965722362830325,
0.102694013405744,0.130071949357647,0.157822871079344,0.185608274535105,
0.195879267308504,0.202565921639154,0.206307055202583,0.236218131652208,
0.266129208101832,0.294041562878489,0.304150158806137,0.310346957232328,
0.314587143109714,0.342995349661446,0.371961471638149,0.401417288131293,
0.421839549604331,0.426720525203164,0.456769376649525,0.482228947818515,
0.491806157628287,0.499594300990965,0.530091426825922,0.558607661325485,
0.566782725939973),.UNSPECIFIED.);
#468=B_SPLINE_CURVE_WITH_KNOTS('',3,(#39515,#39516,#39517,#39518,#39519,
#39520,#39521,#39522,#39523,#39524,#39525,#39526,#39527,#39528,#39529,#39530,
#39531,#39532,#39533,#39534,#39535,#39536,#39537,#39538,#39539,#39540,#39541,
#39542,#39543,#39544,#39545,#39546,#39547,#39548,#39549,#39550,#39551,#39552,
#39553,#39554,#39555,#39556,#39557,#39558,#39559,#39560,#39561,#39562,#39563,
#39564,#39565,#39566,#39567,#39568,#39569,#39570,#39571,#39572,#39573,#39574,
#39575,#39576,#39577,#39578,#39579,#39580,#39581,#39582,#39583,#39584,#39585,
#39586,#39587,#39588,#39589,#39590,#39591,#39592,#39593,#39594,#39595,#39596,
#39597,#39598,#39599,#39600,#39601,#39602,#39603,#39604,#39605),
 .UNSPECIFIED.,.F.,.F.,(4,3,3,3,3,3,3,3,3,3,3,3,3,3,3,3,3,3,3,3,3,3,3,3,
3,3,3,3,3,3,4),(0.,0.0300171424118715,0.0604767221703259,0.0909614341218146,
0.115102967540566,0.120639952334797,0.150400143466383,0.179964556841017,
0.208757681432093,0.230868013600899,0.235298565007282,0.264095539603867,
0.292892514200451,0.294713444433599,0.323669923579346,0.332474977672906,
0.339298452935022,0.344533949196672,0.37258896016374,0.400766388632645,
0.428518995586946,0.4381296236022,0.44395402827716,0.448920751577058,0.475994417150381,
0.498576104022106,0.507824680125155,0.516910851418298,0.542764323146054,
0.562418700022881,0.569248610399432),.UNSPECIFIED.);
#469=B_SPLINE_CURVE_WITH_KNOTS('',3,(#39608,#39609,#39610,#39611,#39612,
#39613,#39614,#39615,#39616,#39617,#39618,#39619,#39620,#39621,#39622,#39623,
#39624,#39625,#39626,#39627,#39628,#39629,#39630,#39631,#39632,#39633,#39634,
#39635,#39636,#39637,#39638,#39639,#39640,#39641,#39642,#39643,#39644,#39645,
#39646,#39647,#39648,#39649,#39650,#39651,#39652,#39653,#39654,#39655,#39656,
#39657,#39658,#39659,#39660,#39661,#39662,#39663,#39664,#39665,#39666,#39667,
#39668,#39669,#39670,#39671,#39672,#39673,#39674,#39675,#39676,#39677,#39678,
#39679,#39680,#39681,#39682,#39683,#39684,#39685,#39686,#39687,#39688,#39689,
#39690,#39691,#39692,#39693,#39694,#39695),.UNSPECIFIED.,.F.,.F.,(4,3,3,
3,3,3,3,3,3,3,3,3,3,3,3,3,3,3,3,3,3,3,3,3,3,3,3,3,3,4),(-0.569248610399404,
-0.543256008460987,-0.51726340652257,-0.510386891772649,-0.504799190792994,
-0.477751536649517,-0.455804039579998,-0.449084589588299,-0.442520438246206,
-0.414640209544556,-0.386493193867354,-0.358551902567642,-0.344585820477761,
-0.340095051696883,-0.311162205934168,-0.302297526319553,-0.274512659934108,
-0.245995923672874,-0.234411538368291,-0.228082474140717,-0.199101564186637,
-0.169609516621985,-0.139817484612857,-0.118141598597594,-0.113403755408093,
-0.0828544964287721,-0.0522777598708405,-0.0223298996975752,-0.00827276376605614,
-3.66886802170398E-5),.UNSPECIFIED.);
#470=B_SPLINE_CURVE_WITH_KNOTS('',3,(#39696,#39697,#39698,#39699,#39700,
#39701,#39702,#39703,#39704,#39705,#39706,#39707,#39708,#39709,#39710,#39711,
#39712,#39713,#39714,#39715,#39716,#39717,#39718,#39719,#39720,#39721,#39722,
#39723,#39724,#39725,#39726,#39727,#39728,#39729,#39730,#39731,#39732,#39733,
#39734,#39735,#39736,#39737,#39738,#39739,#39740,#39741,#39742,#39743,#39744,
#39745,#39746,#39747,#39748,#39749,#39750,#39751,#39752,#39753,#39754,#39755,
#39756,#39757,#39758,#39759,#39760,#39761,#39762,#39763,#39764,#39765,#39766,
#39767,#39768,#39769,#39770,#39771,#39772,#39773,#39774,#39775,#39776,#39777,
#39778,#39779,#39780,#39781,#39782,#39783,#39784,#39785,#39786,#39787,#39788,
#39789),.UNSPECIFIED.,.F.,.F.,(4,3,3,3,3,3,3,3,3,3,3,3,3,3,3,3,3,3,3,3,
3,3,3,3,3,3,3,3,3,3,3,4),(-0.566847306048046,-0.536423709701718,-0.50605441769512,
-0.496627814140597,-0.490481618468529,-0.460353524838767,-0.430379918137283,
-0.424467116489513,-0.418175703681424,-0.38879497848851,-0.359717952452969,
-0.331422325041021,-0.31805487155635,-0.311685352544617,-0.307252153320408,
-0.279281311857458,-0.273681209148987,-0.244539457621602,-0.215397706094217,
-0.205263802913415,-0.200835700491466,-0.173001176808448,-0.145191581540721,
-0.11797816426377,-0.104038996818512,-0.0999813512410115,-0.0958216236861764,
-0.069100446739826,-0.0431518956349564,-0.0175111779746322,-0.00680668378123909,
0.),.UNSPECIFIED.);
#471=B_SPLINE_CURVE_WITH_KNOTS('',3,(#40290,#40291,#40292,#40293,#40294,
#40295,#40296,#40297,#40298,#40299,#40300,#40301,#40302,#40303,#40304,#40305,
#40306,#40307,#40308,#40309,#40310,#40311,#40312,#40313,#40314,#40315,#40316,
#40317,#40318,#40319,#40320,#40321,#40322,#40323,#40324,#40325,#40326,#40327,
#40328,#40329,#40330,#40331,#40332,#40333,#40334,#40335,#40336,#40337,#40338,
#40339,#40340,#40341,#40342,#40343,#40344,#40345,#40346,#40347,#40348,#40349,
#40350,#40351,#40352,#40353,#40354,#40355,#40356,#40357,#40358,#40359,#40360,
#40361,#40362,#40363,#40364,#40365,#40366,#40367,#40368,#40369,#40370,#40371,
#40372,#40373,#40374,#40375,#40376,#40377),.UNSPECIFIED.,.F.,.F.,(4,3,3,
3,3,3,3,3,3,3,3,3,3,3,3,3,3,3,3,3,3,3,3,3,3,3,3,3,3,4),(7.74627845254649E-15,
0.0255384719591611,0.0516106888482134,0.0783325514691107,0.0899901572052831,
0.0973264106699432,0.102694480428545,0.130069272970533,0.157818590910839,
0.185604967740116,0.195878534404192,0.202565264334309,0.206306310167482,
0.236217759134657,0.266129208101832,0.294113525899595,0.310415969469161,
0.314649901542024,0.34306364441444,0.372033774758409,0.401490366934477,
0.422001683954396,0.426785325677536,0.456835670166022,0.482278667955884,
0.491831076392005,0.499580324142813,0.530077574030736,0.55860766132547,
0.566782993632779),.UNSPECIFIED.);
#472=B_SPLINE_CURVE_WITH_KNOTS('',3,(#40878,#40879,#40880,#40881,#40882,
#40883,#40884,#40885,#40886,#40887,#40888,#40889,#40890,#40891,#40892,#40893,
#40894,#40895,#40896,#40897,#40898,#40899,#40900,#40901,#40902,#40903,#40904,
#40905,#40906,#40907,#40908,#40909,#40910,#40911,#40912,#40913,#40914,#40915,
#40916,#40917,#40918,#40919,#40920,#40921,#40922,#40923,#40924,#40925,#40926,
#40927,#40928,#40929,#40930,#40931,#40932,#40933,#40934,#40935,#40936,#40937,
#40938,#40939,#40940,#40941,#40942,#40943,#40944,#40945,#40946,#40947,#40948,
#40949,#40950,#40951,#40952,#40953,#40954,#40955,#40956,#40957,#40958,#40959,
#40960,#40961,#40962,#40963,#40964,#40965,#40966,#40967,#40968,#40969,#40970,
#40971),.UNSPECIFIED.,.F.,.F.,(4,3,3,3,3,3,3,3,3,3,3,3,3,3,3,3,3,3,3,3,
3,3,3,3,3,3,3,3,3,3,3,4),(5.65216427767104E-15,0.0300138468892199,0.0604718986070861,
0.090957520735419,0.115098416893496,0.120639356618796,0.150402829187302,
0.180004389620233,0.208931385640857,0.22092145313717,0.230873872217119,
0.235299701846774,0.264096922839113,0.292894143831452,0.294713444433604,
0.323669767997715,0.332475376686475,0.339302265504674,0.343483980235969,
0.371527376856032,0.399706760133745,0.427472592753052,0.438139069525203,
0.443961451456035,0.449567836675998,0.476635483291862,0.498576344057142,
0.50782599044979,0.516923305096603,0.54277922365799,0.562418700022943,0.569248610399501),
 .UNSPECIFIED.);
#940=SHAPE_REPRESENTATION_RELATIONSHIP('SRR','None',#94492,#955);
#955=ADVANCED_BREP_SHAPE_REPRESENTATION('',(#985),#94401);
#970=STYLED_ITEM('',(#94577),#985);
#985=MANIFOLD_SOLID_BREP('Body1',#8255);
#1012=FACE_BOUND('',#1666,.T.);
#1013=FACE_BOUND('',#1668,.T.);
#1090=PLANE('',#8605);
#1091=PLANE('',#8606);
#1092=PLANE('',#8607);
#1093=PLANE('',#8608);
#1094=PLANE('',#8612);
#1095=PLANE('',#8613);
#1204=FACE_OUTER_BOUND('',#1576,.T.);
#1205=FACE_OUTER_BOUND('',#1577,.T.);
#1206=FACE_OUTER_BOUND('',#1578,.T.);
#1207=FACE_OUTER_BOUND('',#1579,.T.);
#1208=FACE_OUTER_BOUND('',#1580,.T.);
#1209=FACE_OUTER_BOUND('',#1581,.T.);
#1210=FACE_OUTER_BOUND('',#1582,.T.);
#1211=FACE_OUTER_BOUND('',#1583,.T.);
#1212=FACE_OUTER_BOUND('',#1584,.T.);
#1213=FACE_OUTER_BOUND('',#1585,.T.);
#1214=FACE_OUTER_BOUND('',#1586,.T.);
#1215=FACE_OUTER_BOUND('',#1587,.T.);
#1216=FACE_OUTER_BOUND('',#1588,.T.);
#1217=FACE_OUTER_BOUND('',#1589,.T.);
#1218=FACE_OUTER_BOUND('',#1590,.T.);
#1219=FACE_OUTER_BOUND('',#1591,.T.);
#1220=FACE_OUTER_BOUND('',#1592,.T.);
#1221=FACE_OUTER_BOUND('',#1593,.T.);
#1222=FACE_OUTER_BOUND('',#1594,.T.);
#1223=FACE_OUTER_BOUND('',#1595,.T.);
#1224=FACE_OUTER_BOUND('',#1596,.T.);
#1225=FACE_OUTER_BOUND('',#1597,.T.);
#1226=FACE_OUTER_BOUND('',#1598,.T.);
#1227=FACE_OUTER_BOUND('',#1599,.T.);
#1228=FACE_OUTER_BOUND('',#1600,.T.);
#1229=FACE_OUTER_BOUND('',#1601,.T.);
#1230=FACE_OUTER_BOUND('',#1602,.T.);
#1231=FACE_OUTER_BOUND('',#1603,.T.);
#1232=FACE_OUTER_BOUND('',#1604,.T.);
#1233=FACE_OUTER_BOUND('',#1605,.T.);
#1234=FACE_OUTER_BOUND('',#1606,.T.);
#1235=FACE_OUTER_BOUND('',#1607,.T.);
#1236=FACE_OUTER_BOUND('',#1608,.T.);
#1237=FACE_OUTER_BOUND('',#1609,.T.);
#1238=FACE_OUTER_BOUND('',#1610,.T.);
#1239=FACE_OUTER_BOUND('',#1611,.T.);
#1240=FACE_OUTER_BOUND('',#1612,.T.);
#1241=FACE_OUTER_BOUND('',#1613,.T.);
#1242=FACE_OUTER_BOUND('',#1614,.T.);
#1243=FACE_OUTER_BOUND('',#1615,.T.);
#1244=FACE_OUTER_BOUND('',#1616,.T.);
#1245=FACE_OUTER_BOUND('',#1617,.T.);
#1246=FACE_OUTER_BOUND('',#1618,.T.);
#1247=FACE_OUTER_BOUND('',#1619,.T.);
#1248=FACE_OUTER_BOUND('',#1620,.T.);
#1249=FACE_OUTER_BOUND('',#1621,.T.);
#1250=FACE_OUTER_BOUND('',#1622,.T.);
#1251=FACE_OUTER_BOUND('',#1623,.T.);
#1252=FACE_OUTER_BOUND('',#1624,.T.);
#1253=FACE_OUTER_BOUND('',#1625,.T.);
#1254=FACE_OUTER_BOUND('',#1626,.T.);
#1255=FACE_OUTER_BOUND('',#1627,.T.);
#1256=FACE_OUTER_BOUND('',#1628,.T.);
#1257=FACE_OUTER_BOUND('',#1629,.T.);
#1258=FACE_OUTER_BOUND('',#1630,.T.);
#1259=FACE_OUTER_BOUND('',#1631,.T.);
#1260=FACE_OUTER_BOUND('',#1632,.T.);
#1261=FACE_OUTER_BOUND('',#1633,.T.);
#1262=FACE_OUTER_BOUND('',#1634,.T.);
#1263=FACE_OUTER_BOUND('',#1635,.T.);
#1264=FACE_OUTER_BOUND('',#1636,.T.);
#1265=FACE_OUTER_BOUND('',#1637,.T.);
#1266=FACE_OUTER_BOUND('',#1638,.T.);
#1267=FACE_OUTER_BOUND('',#1639,.T.);
#1268=FACE_OUTER_BOUND('',#1640,.T.);
#1269=FACE_OUTER_BOUND('',#1641,.T.);
#1270=FACE_OUTER_BOUND('',#1642,.T.);
#1271=FACE_OUTER_BOUND('',#1643,.T.);
#1272=FACE_OUTER_BOUND('',#1644,.T.);
#1273=FACE_OUTER_BOUND('',#1645,.T.);
#1274=FACE_OUTER_BOUND('',#1646,.T.);
#1275=FACE_OUTER_BOUND('',#1647,.T.);
#1276=FACE_OUTER_BOUND('',#1648,.T.);
#1277=FACE_OUTER_BOUND('',#1649,.T.);
#1278=FACE_OUTER_BOUND('',#1650,.T.);
#1279=FACE_OUTER_BOUND('',#1651,.T.);
#1280=FACE_OUTER_BOUND('',#1652,.T.);
#1281=FACE_OUTER_BOUND('',#1653,.T.);
#1282=FACE_OUTER_BOUND('',#1654,.T.);
#1283=FACE_OUTER_BOUND('',#1655,.T.);
#1284=FACE_OUTER_BOUND('',#1656,.T.);
#1285=FACE_OUTER_BOUND('',#1657,.T.);
#1286=FACE_OUTER_BOUND('',#1658,.T.);
#1287=FACE_OUTER_BOUND('',#1659,.T.);
#1288=FACE_OUTER_BOUND('',#1660,.T.);
#1289=FACE_OUTER_BOUND('',#1661,.T.);
#1290=FACE_OUTER_BOUND('',#1662,.T.);
#1291=FACE_OUTER_BOUND('',#1663,.T.);
#1292=FACE_OUTER_BOUND('',#1664,.T.);
#1293=FACE_OUTER_BOUND('',#1665,.T.);
#1294=FACE_OUTER_BOUND('',#1667,.T.);
#1576=EDGE_LOOP('',(#5322,#5323,#5324,#5325));
#1577=EDGE_LOOP('',(#5326,#5327,#5328,#5329,#5330,#5331));
#1578=EDGE_LOOP('',(#5332,#5333,#5334,#5335,#5336,#5337));
#1579=EDGE_LOOP('',(#5338,#5339,#5340,#5341,#5342,#5343));
#1580=EDGE_LOOP('',(#5344,#5345,#5346,#5347,#5348,#5349));
#1581=EDGE_LOOP('',(#5350,#5351,#5352,#5353,#5354,#5355));
#1582=EDGE_LOOP('',(#5356,#5357,#5358,#5359,#5360,#5361));
#1583=EDGE_LOOP('',(#5362,#5363,#5364,#5365,#5366,#5367));
#1584=EDGE_LOOP('',(#5368,#5369,#5370,#5371,#5372,#5373));
#1585=EDGE_LOOP('',(#5374,#5375,#5376,#5377,#5378,#5379));
#1586=EDGE_LOOP('',(#5380,#5381,#5382,#5383,#5384,#5385));
#1587=EDGE_LOOP('',(#5386,#5387,#5388,#5389,#5390,#5391));
#1588=EDGE_LOOP('',(#5392,#5393,#5394,#5395,#5396,#5397));
#1589=EDGE_LOOP('',(#5398,#5399,#5400,#5401,#5402,#5403));
#1590=EDGE_LOOP('',(#5404,#5405,#5406,#5407,#5408,#5409));
#1591=EDGE_LOOP('',(#5410,#5411,#5412,#5413,#5414,#5415));
#1592=EDGE_LOOP('',(#5416,#5417,#5418,#5419,#5420,#5421));
#1593=EDGE_LOOP('',(#5422,#5423,#5424,#5425,#5426,#5427));
#1594=EDGE_LOOP('',(#5428,#5429,#5430,#5431,#5432,#5433));
#1595=EDGE_LOOP('',(#5434,#5435,#5436,#5437,#5438,#5439,#5440,#5441));
#1596=EDGE_LOOP('',(#5442,#5443,#5444,#5445,#5446,#5447));
#1597=EDGE_LOOP('',(#5448,#5449,#5450,#5451,#5452));
#1598=EDGE_LOOP('',(#5453,#5454,#5455,#5456,#5457,#5458));
#1599=EDGE_LOOP('',(#5459,#5460,#5461,#5462,#5463));
#1600=EDGE_LOOP('',(#5464,#5465,#5466,#5467,#5468,#5469));
#1601=EDGE_LOOP('',(#5470,#5471,#5472,#5473,#5474));
#1602=EDGE_LOOP('',(#5475,#5476,#5477,#5478,#5479,#5480));
#1603=EDGE_LOOP('',(#5481,#5482,#5483,#5484,#5485));
#1604=EDGE_LOOP('',(#5486,#5487,#5488,#5489,#5490,#5491));
#1605=EDGE_LOOP('',(#5492,#5493,#5494,#5495,#5496));
#1606=EDGE_LOOP('',(#5497,#5498,#5499,#5500,#5501,#5502));
#1607=EDGE_LOOP('',(#5503,#5504,#5505,#5506,#5507));
#1608=EDGE_LOOP('',(#5508,#5509,#5510,#5511,#5512,#5513));
#1609=EDGE_LOOP('',(#5514,#5515,#5516,#5517,#5518));
#1610=EDGE_LOOP('',(#5519,#5520,#5521,#5522,#5523,#5524));
#1611=EDGE_LOOP('',(#5525,#5526,#5527,#5528,#5529));
#1612=EDGE_LOOP('',(#5530,#5531,#5532,#5533,#5534,#5535));
#1613=EDGE_LOOP('',(#5536,#5537,#5538,#5539,#5540,#5541));
#1614=EDGE_LOOP('',(#5542,#5543,#5544,#5545));
#1615=EDGE_LOOP('',(#5546,#5547,#5548,#5549,#5550,#5551));
#1616=EDGE_LOOP('',(#5552,#5553,#5554,#5555,#5556,#5557));
#1617=EDGE_LOOP('',(#5558,#5559,#5560,#5561,#5562,#5563));
#1618=EDGE_LOOP('',(#5564,#5565,#5566,#5567,#5568,#5569));
#1619=EDGE_LOOP('',(#5570,#5571,#5572,#5573,#5574,#5575));
#1620=EDGE_LOOP('',(#5576,#5577,#5578,#5579,#5580,#5581));
#1621=EDGE_LOOP('',(#5582,#5583,#5584,#5585,#5586,#5587));
#1622=EDGE_LOOP('',(#5588,#5589,#5590,#5591,#5592,#5593));
#1623=EDGE_LOOP('',(#5594,#5595,#5596,#5597,#5598,#5599));
#1624=EDGE_LOOP('',(#5600,#5601,#5602,#5603,#5604,#5605));
#1625=EDGE_LOOP('',(#5606,#5607,#5608,#5609,#5610,#5611));
#1626=EDGE_LOOP('',(#5612,#5613,#5614,#5615,#5616,#5617));
#1627=EDGE_LOOP('',(#5618,#5619,#5620,#5621,#5622,#5623));
#1628=EDGE_LOOP('',(#5624,#5625,#5626,#5627,#5628,#5629));
#1629=EDGE_LOOP('',(#5630,#5631,#5632,#5633,#5634,#5635));
#1630=EDGE_LOOP('',(#5636,#5637,#5638,#5639,#5640,#5641));
#1631=EDGE_LOOP('',(#5642,#5643,#5644,#5645,#5646,#5647));
#1632=EDGE_LOOP('',(#5648,#5649,#5650,#5651,#5652,#5653));
#1633=EDGE_LOOP('',(#5654,#5655,#5656,#5657,#5658,#5659,#5660,#5661));
#1634=EDGE_LOOP('',(#5662,#5663,#5664,#5665,#5666,#5667));
#1635=EDGE_LOOP('',(#5668,#5669,#5670,#5671,#5672,#5673));
#1636=EDGE_LOOP('',(#5674,#5675,#5676,#5677,#5678));
#1637=EDGE_LOOP('',(#5679,#5680,#5681,#5682,#5683,#5684));
#1638=EDGE_LOOP('',(#5685,#5686,#5687,#5688,#5689));
#1639=EDGE_LOOP('',(#5690,#5691,#5692,#5693,#5694,#5695));
#1640=EDGE_LOOP('',(#5696,#5697,#5698,#5699,#5700));
#1641=EDGE_LOOP('',(#5701,#5702,#5703,#5704,#5705,#5706));
#1642=EDGE_LOOP('',(#5707,#5708,#5709,#5710,#5711));
#1643=EDGE_LOOP('',(#5712,#5713,#5714,#5715,#5716,#5717));
#1644=EDGE_LOOP('',(#5718,#5719,#5720,#5721,#5722));
#1645=EDGE_LOOP('',(#5723,#5724,#5725,#5726,#5727,#5728));
#1646=EDGE_LOOP('',(#5729,#5730,#5731,#5732,#5733));
#1647=EDGE_LOOP('',(#5734,#5735,#5736,#5737,#5738,#5739));
#1648=EDGE_LOOP('',(#5740,#5741,#5742,#5743,#5744));
#1649=EDGE_LOOP('',(#5745,#5746,#5747,#5748,#5749,#5750));
#1650=EDGE_LOOP('',(#5751,#5752,#5753,#5754,#5755));
#1651=EDGE_LOOP('',(#5756,#5757,#5758,#5759,#5760,#5761));
#1652=EDGE_LOOP('',(#5762,#5763,#5764,#5765,#5766,#5767));
#1653=EDGE_LOOP('',(#5768,#5769,#5770,#5771,#5772,#5773));
#1654=EDGE_LOOP('',(#5774,#5775,#5776,#5777,#5778));
#1655=EDGE_LOOP('',(#5779,#5780,#5781,#5782,#5783,#5784));
#1656=EDGE_LOOP('',(#5785,#5786,#5787,#5788,#5789));
#1657=EDGE_LOOP('',(#5790,#5791,#5792,#5793,#5794,#5795,#5796,#5797,#5798,
#5799,#5800,#5801,#5802,#5803,#5804,#5805,#5806,#5807,#5808,#5809,#5810,
#5811,#5812,#5813,#5814,#5815,#5816,#5817,#5818,#5819,#5820,#5821,#5822,
#5823,#5824,#5825,#5826,#5827,#5828,#5829,#5830,#5831,#5832,#5833,#5834,
#5835,#5836,#5837,#5838,#5839,#5840,#5841,#5842,#5843,#5844,#5845,#5846,
#5847,#5848,#5849,#5850,#5851,#5852,#5853,#5854,#5855,#5856,#5857,#5858,
#5859,#5860));
#1658=EDGE_LOOP('',(#5861,#5862,#5863,#5864,#5865,#5866,#5867,#5868,#5869,
#5870,#5871,#5872,#5873,#5874,#5875,#5876,#5877,#5878,#5879,#5880,#5881,
#5882,#5883,#5884,#5885,#5886,#5887,#5888,#5889,#5890,#5891,#5892,#5893,
#5894,#5895,#5896,#5897,#5898,#5899,#5900,#5901,#5902,#5903,#5904,#5905,
#5906,#5907,#5908,#5909,#5910,#5911,#5912,#5913,#5914,#5915,#5916,#5917,
#5918,#5919,#5920,#5921,#5922,#5923,#5924,#5925,#5926,#5927,#5928,#5929,
#5930,#5931,#5932,#5933,#5934,#5935,#5936,#5937,#5938,#5939,#5940));
#1659=EDGE_LOOP('',(#5941));
#1660=EDGE_LOOP('',(#5942,#5943,#5944,#5945,#5946));
#1661=EDGE_LOOP('',(#5947,#5948,#5949,#5950,#5951,#5952,#5953,#5954,#5955,
#5956,#5957,#5958,#5959,#5960,#5961,#5962,#5963,#5964,#5965,#5966,#5967,
#5968,#5969,#5970,#5971,#5972,#5973,#5974,#5975,#5976,#5977,#5978,#5979,
#5980,#5981,#5982,#5983,#5984,#5985,#5986,#5987,#5988,#5989,#5990,#5991,
#5992,#5993,#5994,#5995,#5996,#5997,#5998,#5999,#6000,#6001,#6002,#6003,
#6004,#6005,#6006,#6007,#6008,#6009,#6010,#6011,#6012,#6013,#6014,#6015,
#6016,#6017,#6018));
#1662=EDGE_LOOP('',(#6019,#6020,#6021,#6022,#6023,#6024,#6025,#6026,#6027,
#6028,#6029,#6030,#6031,#6032,#6033,#6034,#6035,#6036,#6037,#6038,#6039,
#6040,#6041,#6042,#6043,#6044,#6045,#6046,#6047,#6048,#6049,#6050,#6051,
#6052,#6053,#6054,#6055,#6056,#6057,#6058,#6059,#6060,#6061,#6062,#6063,
#6064,#6065,#6066,#6067,#6068,#6069,#6070,#6071,#6072,#6073,#6074,#6075,
#6076,#6077,#6078,#6079,#6080,#6081,#6082,#6083,#6084,#6085,#6086,#6087,
#6088,#6089,#6090,#6091,#6092,#6093,#6094,#6095,#6096,#6097,#6098));
#1663=EDGE_LOOP('',(#6099));
#1664=EDGE_LOOP('',(#6100,#6101,#6102,#6103));
#1665=EDGE_LOOP('',(#6104));
#1666=EDGE_LOOP('',(#6105,#6106,#6107,#6108));
#1667=EDGE_LOOP('',(#6109));
#1668=EDGE_LOOP('',(#6110,#6111,#6112,#6113));
#2018=LINE('',#10606,#2416);
#2019=LINE('',#10783,#2417);
#2020=LINE('',#11085,#2418);
#2021=LINE('',#11314,#2419);
#2022=LINE('',#11546,#2420);
#2023=LINE('',#11776,#2421);
#2024=LINE('',#12008,#2422);
#2025=LINE('',#12243,#2423);
#2026=LINE('',#12475,#2424);
#2027=LINE('',#12705,#2425);
#2028=LINE('',#12810,#2426);
#2029=LINE('',#12844,#2427);
#2030=LINE('',#13007,#2428);
#2031=LINE('',#13237,#2429);
#2032=LINE('',#13469,#2430);
#2033=LINE('',#13701,#2431);
#2034=LINE('',#13930,#2432);
#2035=LINE('',#14163,#2433);
#2036=LINE('',#14395,#2434);
#2037=LINE('',#14556,#2435);
#2038=LINE('',#14573,#2436);
#2039=LINE('',#14647,#2437);
#2040=LINE('',#15070,#2438);
#2041=LINE('',#15538,#2439);
#2042=LINE('',#15958,#2440);
#2043=LINE('',#16359,#2441);
#2044=LINE('',#16776,#2442);
#2045=LINE('',#17208,#2443);
#2046=LINE('',#17660,#2444);
#2047=LINE('',#18123,#2445);
#2048=LINE('',#18533,#2446);
#2049=LINE('',#18966,#2447);
#2050=LINE('',#19392,#2448);
#2051=LINE('',#19804,#2449);
#2052=LINE('',#20234,#2450);
#2053=LINE('',#20715,#2451);
#2054=LINE('',#21129,#2452);
#2055=LINE('',#21560,#2453);
#2056=LINE('',#21975,#2454);
#2057=LINE('',#22312,#2455);
#2058=LINE('',#22419,#2456);
#2059=LINE('',#22654,#2457);
#2060=LINE('',#23011,#2458);
#2061=LINE('',#23441,#2459);
#2062=LINE('',#23871,#2460);
#2063=LINE('',#24298,#2461);
#2064=LINE('',#24728,#2462);
#2065=LINE('',#25158,#2463);
#2066=LINE('',#25588,#2464);
#2067=LINE('',#26021,#2465);
#2068=LINE('',#26445,#2466);
#2069=LINE('',#26875,#2467);
#2070=LINE('',#27305,#2468);
#2071=LINE('',#27732,#2469);
#2072=LINE('',#28162,#2470);
#2073=LINE('',#28586,#2471);
#2074=LINE('',#29016,#2472);
#2075=LINE('',#29315,#2473);
#2076=LINE('',#29476,#2474);
#2077=LINE('',#29493,#2475);
#2078=LINE('',#29567,#2476);
#2079=LINE('',#29800,#2477);
#2080=LINE('',#30203,#2478);
#2081=LINE('',#30628,#2479);
#2082=LINE('',#31046,#2480);
#2083=LINE('',#31472,#2481);
#2084=LINE('',#31913,#2482);
#2085=LINE('',#32346,#2483);
#2086=LINE('',#32774,#2484);
#2087=LINE('',#33195,#2485);
#2088=LINE('',#33665,#2486);
#2089=LINE('',#34148,#2487);
#2090=LINE('',#34561,#2488);
#2091=LINE('',#34980,#2489);
#2092=LINE('',#35418,#2490);
#2093=LINE('',#35831,#2491);
#2094=LINE('',#36243,#2492);
#2095=LINE('',#36649,#2493);
#2096=LINE('',#40977,#2494);
#2416=VECTOR('',#9192,3.0735);
#2417=VECTOR('',#9197,3.0735);
#2418=VECTOR('',#9200,3.0735);
#2419=VECTOR('',#9203,3.0735);
#2420=VECTOR('',#9206,3.0735);
#2421=VECTOR('',#9209,3.0735);
#2422=VECTOR('',#9212,3.0735);
#2423=VECTOR('',#9215,3.0735);
#2424=VECTOR('',#9218,3.0735);
#2425=VECTOR('',#9221,3.0735);
#2426=VECTOR('',#9224,3.0735);
#2427=VECTOR('',#9227,3.0735);
#2428=VECTOR('',#9230,3.0735);
#2429=VECTOR('',#9233,3.0735);
#2430=VECTOR('',#9236,3.0735);
#2431=VECTOR('',#9239,3.0735);
#2432=VECTOR('',#9242,3.0735);
#2433=VECTOR('',#9245,3.0735);
#2434=VECTOR('',#9248,3.0735);
#2435=VECTOR('',#9253,2.5175);
#2436=VECTOR('',#9256,2.5175);
#2437=VECTOR('',#9263,2.5175);
#2438=VECTOR('',#9266,2.5175);
#2439=VECTOR('',#9269,2.5175);
#2440=VECTOR('',#9272,2.5175);
#2441=VECTOR('',#9275,2.5175);
#2442=VECTOR('',#9278,2.5175);
#2443=VECTOR('',#9281,2.5175);
#2444=VECTOR('',#9284,2.5175);
#2445=VECTOR('',#9287,2.5175);
#2446=VECTOR('',#9290,2.5175);
#2447=VECTOR('',#9293,2.5175);
#2448=VECTOR('',#9296,2.5175);
#2449=VECTOR('',#9299,2.5175);
#2450=VECTOR('',#9302,2.5175);
#2451=VECTOR('',#9305,2.5175);
#2452=VECTOR('',#9308,2.5175);
#2453=VECTOR('',#9311,2.5175);
#2454=VECTOR('',#9314,2.5175);
#2455=VECTOR('',#9319,3.0735);
#2456=VECTOR('',#9324,3.0735);
#2457=VECTOR('',#9327,3.0735);
#2458=VECTOR('',#9330,3.0735);
#2459=VECTOR('',#9333,3.0735);
#2460=VECTOR('',#9336,3.0735);
#2461=VECTOR('',#9339,3.0735);
#2462=VECTOR('',#9342,3.0735);
#2463=VECTOR('',#9345,3.0735);
#2464=VECTOR('',#9348,3.0735);
#2465=VECTOR('',#9351,3.0735);
#2466=VECTOR('',#9354,3.0735);
#2467=VECTOR('',#9357,3.0735);
#2468=VECTOR('',#9360,3.0735);
#2469=VECTOR('',#9363,3.0735);
#2470=VECTOR('',#9366,3.0735);
#2471=VECTOR('',#9369,3.0735);
#2472=VECTOR('',#9372,3.0735);
#2473=VECTOR('',#9375,3.0735);
#2474=VECTOR('',#9380,2.5175);
#2475=VECTOR('',#9383,2.5175);
#2476=VECTOR('',#9390,2.5175);
#2477=VECTOR('',#9393,2.5175);
#2478=VECTOR('',#9396,2.5175);
#2479=VECTOR('',#9399,2.5175);
#2480=VECTOR('',#9402,2.5175);
#2481=VECTOR('',#9405,2.5175);
#2482=VECTOR('',#9408,2.5175);
#2483=VECTOR('',#9411,2.5175);
#2484=VECTOR('',#9414,2.5175);
#2485=VECTOR('',#9417,2.5175);
#2486=VECTOR('',#9420,2.5175);
#2487=VECTOR('',#9423,2.5175);
#2488=VECTOR('',#9426,2.5175);
#2489=VECTOR('',#9429,2.5175);
#2490=VECTOR('',#9432,2.5175);
#2491=VECTOR('',#9435,2.5175);
#2492=VECTOR('',#9438,2.5175);
#2493=VECTOR('',#9441,2.5175);
#2494=VECTOR('',#9464,8.);
#2756=CIRCLE('',#8514,3.0735);
#2757=CIRCLE('',#8533,3.0735);
#2758=CIRCLE('',#8535,2.5175);
#2759=CIRCLE('',#8536,2.5175);
#2760=CIRCLE('',#8537,2.5175);
#2761=CIRCLE('',#8556,2.5175);
#2762=CIRCLE('',#8558,3.0735);
#2763=CIRCLE('',#8577,3.0735);
#2764=CIRCLE('',#8579,2.5175);
#2765=CIRCLE('',#8580,2.5175);
#2766=CIRCLE('',#8581,2.5175);
#2767=CIRCLE('',#8600,2.5175);
#2768=CIRCLE('',#8610,8.);
#2769=CIRCLE('',#8611,8.);
#2922=VERTEX_POINT('',#10604);
#2923=VERTEX_POINT('',#10605);
#2924=VERTEX_POINT('',#10607);
#2925=VERTEX_POINT('',#10684);
#2926=VERTEX_POINT('',#10781);
#2927=VERTEX_POINT('',#10782);
#2928=VERTEX_POINT('',#10784);
#2929=VERTEX_POINT('',#10994);
#2930=VERTEX_POINT('',#11083);
#2931=VERTEX_POINT('',#11084);
#2932=VERTEX_POINT('',#11086);
#2933=VERTEX_POINT('',#11296);
#2934=VERTEX_POINT('',#11312);
#2935=VERTEX_POINT('',#11313);
#2936=VERTEX_POINT('',#11315);
#2937=VERTEX_POINT('',#11528);
#2938=VERTEX_POINT('',#11544);
#2939=VERTEX_POINT('',#11545);
#2940=VERTEX_POINT('',#11547);
#2941=VERTEX_POINT('',#11757);
#2942=VERTEX_POINT('',#11774);
#2943=VERTEX_POINT('',#11775);
#2944=VERTEX_POINT('',#11777);
#2945=VERTEX_POINT('',#11990);
#2946=VERTEX_POINT('',#12006);
#2947=VERTEX_POINT('',#12007);
#2948=VERTEX_POINT('',#12009);
#2949=VERTEX_POINT('',#12225);
#2950=VERTEX_POINT('',#12241);
#2951=VERTEX_POINT('',#12242);
#2952=VERTEX_POINT('',#12244);
#2953=VERTEX_POINT('',#12457);
#2954=VERTEX_POINT('',#12473);
#2955=VERTEX_POINT('',#12474);
#2956=VERTEX_POINT('',#12476);
#2957=VERTEX_POINT('',#12686);
#2958=VERTEX_POINT('',#12703);
#2959=VERTEX_POINT('',#12704);
#2960=VERTEX_POINT('',#12706);
#2961=VERTEX_POINT('',#12792);
#2962=VERTEX_POINT('',#12808);
#2963=VERTEX_POINT('',#12809);
#2964=VERTEX_POINT('',#12811);
#2965=VERTEX_POINT('',#12826);
#2966=VERTEX_POINT('',#12842);
#2967=VERTEX_POINT('',#12843);
#2968=VERTEX_POINT('',#12845);
#2969=VERTEX_POINT('',#12860);
#2970=VERTEX_POINT('',#13005);
#2971=VERTEX_POINT('',#13006);
#2972=VERTEX_POINT('',#13008);
#2973=VERTEX_POINT('',#13024);
#2974=VERTEX_POINT('',#13235);
#2975=VERTEX_POINT('',#13236);
#2976=VERTEX_POINT('',#13238);
#2977=VERTEX_POINT('',#13253);
#2978=VERTEX_POINT('',#13467);
#2979=VERTEX_POINT('',#13468);
#2980=VERTEX_POINT('',#13470);
#2981=VERTEX_POINT('',#13485);
#2982=VERTEX_POINT('',#13699);
#2983=VERTEX_POINT('',#13700);
#2984=VERTEX_POINT('',#13702);
#2985=VERTEX_POINT('',#13717);
#2986=VERTEX_POINT('',#13928);
#2987=VERTEX_POINT('',#13929);
#2988=VERTEX_POINT('',#13931);
#2989=VERTEX_POINT('',#13947);
#2990=VERTEX_POINT('',#14161);
#2991=VERTEX_POINT('',#14162);
#2992=VERTEX_POINT('',#14164);
#2993=VERTEX_POINT('',#14179);
#2994=VERTEX_POINT('',#14393);
#2995=VERTEX_POINT('',#14394);
#2996=VERTEX_POINT('',#14396);
#2997=VERTEX_POINT('',#14473);
#2998=VERTEX_POINT('',#14479);
#2999=VERTEX_POINT('',#14481);
#3000=VERTEX_POINT('',#14554);
#3001=VERTEX_POINT('',#14555);
#3002=VERTEX_POINT('',#14557);
#3003=VERTEX_POINT('',#14570);
#3004=VERTEX_POINT('',#14572);
#3005=VERTEX_POINT('',#14575);
#3006=VERTEX_POINT('',#14645);
#3007=VERTEX_POINT('',#14646);
#3008=VERTEX_POINT('',#14648);
#3009=VERTEX_POINT('',#14853);
#3010=VERTEX_POINT('',#15068);
#3011=VERTEX_POINT('',#15069);
#3012=VERTEX_POINT('',#15071);
#3013=VERTEX_POINT('',#15536);
#3014=VERTEX_POINT('',#15537);
#3015=VERTEX_POINT('',#15539);
#3016=VERTEX_POINT('',#15734);
#3017=VERTEX_POINT('',#15956);
#3018=VERTEX_POINT('',#15957);
#3019=VERTEX_POINT('',#15959);
#3020=VERTEX_POINT('',#16357);
#3021=VERTEX_POINT('',#16358);
#3022=VERTEX_POINT('',#16360);
#3023=VERTEX_POINT('',#16558);
#3024=VERTEX_POINT('',#16774);
#3025=VERTEX_POINT('',#16775);
#3026=VERTEX_POINT('',#16777);
#3027=VERTEX_POINT('',#17206);
#3028=VERTEX_POINT('',#17207);
#3029=VERTEX_POINT('',#17209);
#3030=VERTEX_POINT('',#17404);
#3031=VERTEX_POINT('',#17658);
#3032=VERTEX_POINT('',#17659);
#3033=VERTEX_POINT('',#17661);
#3034=VERTEX_POINT('',#18121);
#3035=VERTEX_POINT('',#18122);
#3036=VERTEX_POINT('',#18124);
#3037=VERTEX_POINT('',#18319);
#3038=VERTEX_POINT('',#18531);
#3039=VERTEX_POINT('',#18532);
#3040=VERTEX_POINT('',#18534);
#3041=VERTEX_POINT('',#18964);
#3042=VERTEX_POINT('',#18965);
#3043=VERTEX_POINT('',#18967);
#3044=VERTEX_POINT('',#19162);
#3045=VERTEX_POINT('',#19390);
#3046=VERTEX_POINT('',#19391);
#3047=VERTEX_POINT('',#19393);
#3048=VERTEX_POINT('',#19802);
#3049=VERTEX_POINT('',#19803);
#3050=VERTEX_POINT('',#19805);
#3051=VERTEX_POINT('',#20000);
#3052=VERTEX_POINT('',#20232);
#3053=VERTEX_POINT('',#20233);
#3054=VERTEX_POINT('',#20235);
#3055=VERTEX_POINT('',#20713);
#3056=VERTEX_POINT('',#20714);
#3057=VERTEX_POINT('',#20716);
#3058=VERTEX_POINT('',#20911);
#3059=VERTEX_POINT('',#21127);
#3060=VERTEX_POINT('',#21128);
#3061=VERTEX_POINT('',#21130);
#3062=VERTEX_POINT('',#21558);
#3063=VERTEX_POINT('',#21559);
#3064=VERTEX_POINT('',#21561);
#3065=VERTEX_POINT('',#21753);
#3066=VERTEX_POINT('',#21973);
#3067=VERTEX_POINT('',#21974);
#3068=VERTEX_POINT('',#21976);
#3069=VERTEX_POINT('',#21999);
#3070=VERTEX_POINT('',#22121);
#3071=VERTEX_POINT('',#22123);
#3072=VERTEX_POINT('',#22310);
#3073=VERTEX_POINT('',#22311);
#3074=VERTEX_POINT('',#22313);
#3075=VERTEX_POINT('',#22320);
#3076=VERTEX_POINT('',#22417);
#3077=VERTEX_POINT('',#22418);
#3078=VERTEX_POINT('',#22420);
#3079=VERTEX_POINT('',#22563);
#3080=VERTEX_POINT('',#22652);
#3081=VERTEX_POINT('',#22653);
#3082=VERTEX_POINT('',#22655);
#3083=VERTEX_POINT('',#22865);
#3084=VERTEX_POINT('',#23009);
#3085=VERTEX_POINT('',#23010);
#3086=VERTEX_POINT('',#23012);
#3087=VERTEX_POINT('',#23225);
#3088=VERTEX_POINT('',#23439);
#3089=VERTEX_POINT('',#23440);
#3090=VERTEX_POINT('',#23442);
#3091=VERTEX_POINT('',#23652);
#3092=VERTEX_POINT('',#23869);
#3093=VERTEX_POINT('',#23870);
#3094=VERTEX_POINT('',#23872);
#3095=VERTEX_POINT('',#24085);
#3096=VERTEX_POINT('',#24296);
#3097=VERTEX_POINT('',#24297);
#3098=VERTEX_POINT('',#24299);
#3099=VERTEX_POINT('',#24515);
#3100=VERTEX_POINT('',#24726);
#3101=VERTEX_POINT('',#24727);
#3102=VERTEX_POINT('',#24729);
#3103=VERTEX_POINT('',#24942);
#3104=VERTEX_POINT('',#25156);
#3105=VERTEX_POINT('',#25157);
#3106=VERTEX_POINT('',#25159);
#3107=VERTEX_POINT('',#25369);
#3108=VERTEX_POINT('',#25586);
#3109=VERTEX_POINT('',#25587);
#3110=VERTEX_POINT('',#25589);
#3111=VERTEX_POINT('',#25805);
#3112=VERTEX_POINT('',#26019);
#3113=VERTEX_POINT('',#26020);
#3114=VERTEX_POINT('',#26022);
#3115=VERTEX_POINT('',#26232);
#3116=VERTEX_POINT('',#26443);
#3117=VERTEX_POINT('',#26444);
#3118=VERTEX_POINT('',#26446);
#3119=VERTEX_POINT('',#26659);
#3120=VERTEX_POINT('',#26873);
#3121=VERTEX_POINT('',#26874);
#3122=VERTEX_POINT('',#26876);
#3123=VERTEX_POINT('',#27092);
#3124=VERTEX_POINT('',#27303);
#3125=VERTEX_POINT('',#27304);
#3126=VERTEX_POINT('',#27306);
#3127=VERTEX_POINT('',#27516);
#3128=VERTEX_POINT('',#27730);
#3129=VERTEX_POINT('',#27731);
#3130=VERTEX_POINT('',#27733);
#3131=VERTEX_POINT('',#27946);
#3132=VERTEX_POINT('',#28160);
#3133=VERTEX_POINT('',#28161);
#3134=VERTEX_POINT('',#28163);
#3135=VERTEX_POINT('',#28373);
#3136=VERTEX_POINT('',#28584);
#3137=VERTEX_POINT('',#28585);
#3138=VERTEX_POINT('',#28587);
#3139=VERTEX_POINT('',#28800);
#3140=VERTEX_POINT('',#29014);
#3141=VERTEX_POINT('',#29015);
#3142=VERTEX_POINT('',#29017);
#3143=VERTEX_POINT('',#29099);
#3144=VERTEX_POINT('',#29313);
#3145=VERTEX_POINT('',#29314);
#3146=VERTEX_POINT('',#29316);
#3147=VERTEX_POINT('',#29393);
#3148=VERTEX_POINT('',#29399);
#3149=VERTEX_POINT('',#29401);
#3150=VERTEX_POINT('',#29474);
#3151=VERTEX_POINT('',#29475);
#3152=VERTEX_POINT('',#29477);
#3153=VERTEX_POINT('',#29490);
#3154=VERTEX_POINT('',#29492);
#3155=VERTEX_POINT('',#29495);
#3156=VERTEX_POINT('',#29565);
#3157=VERTEX_POINT('',#29566);
#3158=VERTEX_POINT('',#29568);
#3159=VERTEX_POINT('',#29773);
#3160=VERTEX_POINT('',#29798);
#3161=VERTEX_POINT('',#29799);
#3162=VERTEX_POINT('',#29801);
#3163=VERTEX_POINT('',#29999);
#3164=VERTEX_POINT('',#30201);
#3165=VERTEX_POINT('',#30202);
#3166=VERTEX_POINT('',#30204);
#3167=VERTEX_POINT('',#30626);
#3168=VERTEX_POINT('',#30627);
#3169=VERTEX_POINT('',#30629);
#3170=VERTEX_POINT('',#30824);
#3171=VERTEX_POINT('',#31044);
#3172=VERTEX_POINT('',#31045);
#3173=VERTEX_POINT('',#31047);
#3174=VERTEX_POINT('',#31470);
#3175=VERTEX_POINT('',#31471);
#3176=VERTEX_POINT('',#31473);
#3177=VERTEX_POINT('',#31671);
#3178=VERTEX_POINT('',#31911);
#3179=VERTEX_POINT('',#31912);
#3180=VERTEX_POINT('',#31914);
#3181=VERTEX_POINT('',#32344);
#3182=VERTEX_POINT('',#32345);
#3183=VERTEX_POINT('',#32347);
#3184=VERTEX_POINT('',#32542);
#3185=VERTEX_POINT('',#32772);
#3186=VERTEX_POINT('',#32773);
#3187=VERTEX_POINT('',#32775);
#3188=VERTEX_POINT('',#33193);
#3189=VERTEX_POINT('',#33194);
#3190=VERTEX_POINT('',#33196);
#3191=VERTEX_POINT('',#33391);
#3192=VERTEX_POINT('',#33663);
#3193=VERTEX_POINT('',#33664);
#3194=VERTEX_POINT('',#33666);
#3195=VERTEX_POINT('',#34146);
#3196=VERTEX_POINT('',#34147);
#3197=VERTEX_POINT('',#34149);
#3198=VERTEX_POINT('',#34347);
#3199=VERTEX_POINT('',#34559);
#3200=VERTEX_POINT('',#34560);
#3201=VERTEX_POINT('',#34562);
#3202=VERTEX_POINT('',#34978);
#3203=VERTEX_POINT('',#34979);
#3204=VERTEX_POINT('',#34981);
#3205=VERTEX_POINT('',#35176);
#3206=VERTEX_POINT('',#35416);
#3207=VERTEX_POINT('',#35417);
#3208=VERTEX_POINT('',#35419);
#3209=VERTEX_POINT('',#35829);
#3210=VERTEX_POINT('',#35830);
#3211=VERTEX_POINT('',#35832);
#3212=VERTEX_POINT('',#36027);
#3213=VERTEX_POINT('',#36241);
#3214=VERTEX_POINT('',#36242);
#3215=VERTEX_POINT('',#36244);
#3216=VERTEX_POINT('',#36647);
#3217=VERTEX_POINT('',#36648);
#3218=VERTEX_POINT('',#36650);
#3219=VERTEX_POINT('',#36664);
#3220=VERTEX_POINT('',#36786);
#3221=VERTEX_POINT('',#36788);
#3222=VERTEX_POINT('',#36975);
#3223=VERTEX_POINT('',#37173);
#3224=VERTEX_POINT('',#37372);
#3225=VERTEX_POINT('',#37387);
#3226=VERTEX_POINT('',#37601);
#3227=VERTEX_POINT('',#38016);
#3228=VERTEX_POINT('',#38031);
#3229=VERTEX_POINT('',#40974);
#3230=VERTEX_POINT('',#40976);
#3926=EDGE_CURVE('',#2922,#2923,#2018,.T.);
#3927=EDGE_CURVE('',#2923,#2924,#170,.T.);
#3928=EDGE_CURVE('',#2925,#2924,#2756,.T.);
#3929=EDGE_CURVE('',#2922,#2925,#171,.T.);
#3930=EDGE_CURVE('',#2926,#2927,#2019,.T.);
#3931=EDGE_CURVE('',#2927,#2928,#172,.T.);
#3932=EDGE_CURVE('',#2928,#2923,#173,.T.);
#3933=EDGE_CURVE('',#2929,#2922,#174,.T.);
#3934=EDGE_CURVE('',#2926,#2929,#175,.T.);
#3935=EDGE_CURVE('',#2930,#2931,#2020,.T.);
#3936=EDGE_CURVE('',#2931,#2932,#176,.T.);
#3937=EDGE_CURVE('',#2932,#2927,#177,.T.);
#3938=EDGE_CURVE('',#2933,#2926,#178,.T.);
#3939=EDGE_CURVE('',#2930,#2933,#179,.T.);
#3940=EDGE_CURVE('',#2934,#2935,#2021,.T.);
#3941=EDGE_CURVE('',#2935,#2936,#180,.T.);
#3942=EDGE_CURVE('',#2936,#2931,#181,.T.);
#3943=EDGE_CURVE('',#2937,#2930,#182,.T.);
#3944=EDGE_CURVE('',#2934,#2937,#183,.T.);
#3945=EDGE_CURVE('',#2938,#2939,#2022,.T.);
#3946=EDGE_CURVE('',#2939,#2940,#184,.T.);
#3947=EDGE_CURVE('',#2940,#2935,#185,.T.);
#3948=EDGE_CURVE('',#2941,#2934,#186,.T.);
#3949=EDGE_CURVE('',#2938,#2941,#187,.T.);
#3950=EDGE_CURVE('',#2942,#2943,#2023,.T.);
#3951=EDGE_CURVE('',#2943,#2944,#188,.T.);
#3952=EDGE_CURVE('',#2944,#2939,#189,.T.);
#3953=EDGE_CURVE('',#2945,#2938,#190,.T.);
#3954=EDGE_CURVE('',#2942,#2945,#191,.T.);
#3955=EDGE_CURVE('',#2946,#2947,#2024,.T.);
#3956=EDGE_CURVE('',#2947,#2948,#192,.T.);
#3957=EDGE_CURVE('',#2948,#2943,#193,.T.);
#3958=EDGE_CURVE('',#2949,#2942,#194,.T.);
#3959=EDGE_CURVE('',#2946,#2949,#195,.T.);
#3960=EDGE_CURVE('',#2950,#2951,#2025,.T.);
#3961=EDGE_CURVE('',#2951,#2952,#196,.T.);
#3962=EDGE_CURVE('',#2952,#2947,#197,.T.);
#3963=EDGE_CURVE('',#2953,#2946,#198,.T.);
#3964=EDGE_CURVE('',#2950,#2953,#199,.T.);
#3965=EDGE_CURVE('',#2954,#2955,#2026,.T.);
#3966=EDGE_CURVE('',#2955,#2956,#200,.T.);
#3967=EDGE_CURVE('',#2956,#2951,#201,.T.);
#3968=EDGE_CURVE('',#2957,#2950,#202,.T.);
#3969=EDGE_CURVE('',#2954,#2957,#203,.T.);
#3970=EDGE_CURVE('',#2958,#2959,#2027,.T.);
#3971=EDGE_CURVE('',#2959,#2960,#204,.T.);
#3972=EDGE_CURVE('',#2960,#2955,#205,.T.);
#3973=EDGE_CURVE('',#2961,#2954,#206,.T.);
#3974=EDGE_CURVE('',#2958,#2961,#207,.T.);
#3975=EDGE_CURVE('',#2962,#2963,#2028,.T.);
#3976=EDGE_CURVE('',#2963,#2964,#208,.T.);
#3977=EDGE_CURVE('',#2964,#2959,#209,.T.);
#3978=EDGE_CURVE('',#2965,#2958,#210,.T.);
#3979=EDGE_CURVE('',#2962,#2965,#211,.T.);
#3980=EDGE_CURVE('',#2966,#2967,#2029,.T.);
#3981=EDGE_CURVE('',#2967,#2968,#212,.T.);
#3982=EDGE_CURVE('',#2968,#2963,#213,.T.);
#3983=EDGE_CURVE('',#2969,#2962,#214,.T.);
#3984=EDGE_CURVE('',#2966,#2969,#215,.T.);
#3985=EDGE_CURVE('',#2970,#2971,#2030,.T.);
#3986=EDGE_CURVE('',#2971,#2972,#216,.T.);
#3987=EDGE_CURVE('',#2972,#2967,#217,.T.);
#3988=EDGE_CURVE('',#2973,#2966,#218,.T.);
#3989=EDGE_CURVE('',#2970,#2973,#219,.T.);
#3990=EDGE_CURVE('',#2974,#2975,#2031,.T.);
#3991=EDGE_CURVE('',#2975,#2976,#220,.T.);
#3992=EDGE_CURVE('',#2976,#2971,#221,.T.);
#3993=EDGE_CURVE('',#2977,#2970,#222,.T.);
#3994=EDGE_CURVE('',#2974,#2977,#223,.T.);
#3995=EDGE_CURVE('',#2978,#2979,#2032,.T.);
#3996=EDGE_CURVE('',#2979,#2980,#224,.T.);
#3997=EDGE_CURVE('',#2980,#2975,#225,.T.);
#3998=EDGE_CURVE('',#2981,#2974,#226,.T.);
#3999=EDGE_CURVE('',#2978,#2981,#227,.T.);
#4000=EDGE_CURVE('',#2982,#2983,#2033,.T.);
#4001=EDGE_CURVE('',#2983,#2984,#228,.T.);
#4002=EDGE_CURVE('',#2984,#2979,#229,.T.);
#4003=EDGE_CURVE('',#2985,#2978,#230,.T.);
#4004=EDGE_CURVE('',#2982,#2985,#231,.T.);
#4005=EDGE_CURVE('',#2986,#2987,#2034,.T.);
#4006=EDGE_CURVE('',#2987,#2988,#232,.T.);
#4007=EDGE_CURVE('',#2988,#2983,#233,.T.);
#4008=EDGE_CURVE('',#2989,#2982,#234,.T.);
#4009=EDGE_CURVE('',#2986,#2989,#235,.T.);
#4010=EDGE_CURVE('',#2990,#2991,#2035,.T.);
#4011=EDGE_CURVE('',#2991,#2992,#236,.T.);
#4012=EDGE_CURVE('',#2992,#2987,#237,.T.);
#4013=EDGE_CURVE('',#2993,#2986,#238,.T.);
#4014=EDGE_CURVE('',#2990,#2993,#239,.T.);
#4015=EDGE_CURVE('',#2994,#2995,#2036,.T.);
#4016=EDGE_CURVE('',#2996,#2994,#240,.T.);
#4017=EDGE_CURVE('',#2997,#2996,#241,.T.);
#4018=EDGE_CURVE('',#2998,#2997,#2757,.T.);
#4019=EDGE_CURVE('',#2998,#2999,#242,.T.);
#4020=EDGE_CURVE('',#2999,#2995,#243,.T.);
#4021=EDGE_CURVE('',#3000,#3001,#2037,.T.);
#4022=EDGE_CURVE('',#3001,#3002,#244,.T.);
#4023=EDGE_CURVE('',#3002,#3003,#2758,.T.);
#4024=EDGE_CURVE('',#3003,#3004,#2038,.T.);
#4025=EDGE_CURVE('',#3004,#3004,#2759,.F.);
#4026=EDGE_CURVE('',#3003,#3005,#2760,.T.);
#4027=EDGE_CURVE('',#3005,#3000,#245,.T.);
#4028=EDGE_CURVE('',#3006,#3007,#2039,.T.);
#4029=EDGE_CURVE('',#3007,#3008,#246,.T.);
#4030=EDGE_CURVE('',#3008,#3001,#247,.T.);
#4031=EDGE_CURVE('',#3000,#3009,#248,.T.);
#4032=EDGE_CURVE('',#3009,#3006,#249,.T.);
#4033=EDGE_CURVE('',#3010,#3011,#2040,.T.);
#4034=EDGE_CURVE('',#3011,#3012,#250,.T.);
#4035=EDGE_CURVE('',#3012,#3007,#251,.T.);
#4036=EDGE_CURVE('',#3006,#3010,#252,.T.);
#4037=EDGE_CURVE('',#3013,#3014,#2041,.T.);
#4038=EDGE_CURVE('',#3014,#3015,#253,.T.);
#4039=EDGE_CURVE('',#3015,#3011,#254,.T.);
#4040=EDGE_CURVE('',#3010,#3016,#255,.T.);
#4041=EDGE_CURVE('',#3016,#3013,#256,.T.);
#4042=EDGE_CURVE('',#3017,#3018,#2042,.T.);
#4043=EDGE_CURVE('',#3018,#3019,#257,.T.);
#4044=EDGE_CURVE('',#3019,#3014,#258,.T.);
#4045=EDGE_CURVE('',#3013,#3017,#259,.T.);
#4046=EDGE_CURVE('',#3020,#3021,#2043,.T.);
#4047=EDGE_CURVE('',#3021,#3022,#260,.T.);
#4048=EDGE_CURVE('',#3022,#3018,#261,.T.);
#4049=EDGE_CURVE('',#3017,#3023,#262,.T.);
#4050=EDGE_CURVE('',#3023,#3020,#263,.T.);
#4051=EDGE_CURVE('',#3024,#3025,#2044,.T.);
#4052=EDGE_CURVE('',#3025,#3026,#264,.T.);
#4053=EDGE_CURVE('',#3026,#3021,#265,.T.);
#4054=EDGE_CURVE('',#3020,#3024,#266,.T.);
#4055=EDGE_CURVE('',#3027,#3028,#2045,.T.);
#4056=EDGE_CURVE('',#3028,#3029,#267,.T.);
#4057=EDGE_CURVE('',#3029,#3025,#268,.T.);
#4058=EDGE_CURVE('',#3024,#3030,#269,.T.);
#4059=EDGE_CURVE('',#3030,#3027,#270,.T.);
#4060=EDGE_CURVE('',#3031,#3032,#2046,.T.);
#4061=EDGE_CURVE('',#3032,#3033,#271,.T.);
#4062=EDGE_CURVE('',#3033,#3028,#272,.T.);
#4063=EDGE_CURVE('',#3027,#3031,#273,.T.);
#4064=EDGE_CURVE('',#3034,#3035,#2047,.T.);
#4065=EDGE_CURVE('',#3035,#3036,#274,.T.);
#4066=EDGE_CURVE('',#3036,#3032,#275,.T.);
#4067=EDGE_CURVE('',#3031,#3037,#276,.T.);
#4068=EDGE_CURVE('',#3037,#3034,#277,.T.);
#4069=EDGE_CURVE('',#3038,#3039,#2048,.T.);
#4070=EDGE_CURVE('',#3039,#3040,#278,.T.);
#4071=EDGE_CURVE('',#3040,#3035,#279,.T.);
#4072=EDGE_CURVE('',#3034,#3038,#280,.T.);
#4073=EDGE_CURVE('',#3041,#3042,#2049,.T.);
#4074=EDGE_CURVE('',#3042,#3043,#281,.T.);
#4075=EDGE_CURVE('',#3043,#3039,#282,.T.);
#4076=EDGE_CURVE('',#3038,#3044,#283,.T.);
#4077=EDGE_CURVE('',#3044,#3041,#284,.T.);
#4078=EDGE_CURVE('',#3045,#3046,#2050,.T.);
#4079=EDGE_CURVE('',#3046,#3047,#285,.T.);
#4080=EDGE_CURVE('',#3047,#3042,#286,.T.);
#4081=EDGE_CURVE('',#3041,#3045,#287,.T.);
#4082=EDGE_CURVE('',#3048,#3049,#2051,.T.);
#4083=EDGE_CURVE('',#3049,#3050,#288,.T.);
#4084=EDGE_CURVE('',#3050,#3046,#289,.T.);
#4085=EDGE_CURVE('',#3045,#3051,#290,.T.);
#4086=EDGE_CURVE('',#3051,#3048,#291,.T.);
#4087=EDGE_CURVE('',#3052,#3053,#2052,.T.);
#4088=EDGE_CURVE('',#3053,#3054,#292,.T.);
#4089=EDGE_CURVE('',#3054,#3049,#293,.T.);
#4090=EDGE_CURVE('',#3048,#3052,#294,.T.);
#4091=EDGE_CURVE('',#3055,#3056,#2053,.T.);
#4092=EDGE_CURVE('',#3056,#3057,#295,.T.);
#4093=EDGE_CURVE('',#3057,#3053,#296,.T.);
#4094=EDGE_CURVE('',#3052,#3058,#297,.T.);
#4095=EDGE_CURVE('',#3058,#3055,#298,.T.);
#4096=EDGE_CURVE('',#3059,#3060,#2054,.T.);
#4097=EDGE_CURVE('',#3060,#3061,#299,.T.);
#4098=EDGE_CURVE('',#3061,#3056,#300,.T.);
#4099=EDGE_CURVE('',#3055,#3059,#301,.T.);
#4100=EDGE_CURVE('',#3062,#3063,#2055,.T.);
#4101=EDGE_CURVE('',#3063,#3064,#302,.T.);
#4102=EDGE_CURVE('',#3064,#3060,#303,.T.);
#4103=EDGE_CURVE('',#3059,#3065,#304,.T.);
#4104=EDGE_CURVE('',#3065,#3062,#305,.T.);
#4105=EDGE_CURVE('',#3066,#3067,#2056,.T.);
#4106=EDGE_CURVE('',#3066,#3068,#306,.T.);
#4107=EDGE_CURVE('',#3068,#3069,#307,.T.);
#4108=EDGE_CURVE('',#3070,#3069,#2761,.F.);
#4109=EDGE_CURVE('',#3070,#3071,#308,.T.);
#4110=EDGE_CURVE('',#3071,#3067,#309,.T.);
#4111=EDGE_CURVE('',#3072,#3073,#2057,.T.);
#4112=EDGE_CURVE('',#3073,#3074,#310,.T.);
#4113=EDGE_CURVE('',#3075,#3074,#2762,.T.);
#4114=EDGE_CURVE('',#3072,#3075,#311,.T.);
#4115=EDGE_CURVE('',#3076,#3077,#2058,.T.);
#4116=EDGE_CURVE('',#3077,#3078,#312,.T.);
#4117=EDGE_CURVE('',#3078,#3073,#313,.T.);
#4118=EDGE_CURVE('',#3079,#3072,#314,.T.);
#4119=EDGE_CURVE('',#3076,#3079,#315,.T.);
#4120=EDGE_CURVE('',#3080,#3081,#2059,.T.);
#4121=EDGE_CURVE('',#3081,#3082,#316,.T.);
#4122=EDGE_CURVE('',#3082,#3077,#317,.T.);
#4123=EDGE_CURVE('',#3083,#3076,#318,.T.);
#4124=EDGE_CURVE('',#3080,#3083,#319,.T.);
#4125=EDGE_CURVE('',#3084,#3085,#2060,.T.);
#4126=EDGE_CURVE('',#3085,#3086,#320,.T.);
#4127=EDGE_CURVE('',#3086,#3081,#321,.T.);
#4128=EDGE_CURVE('',#3087,#3080,#322,.T.);
#4129=EDGE_CURVE('',#3084,#3087,#323,.T.);
#4130=EDGE_CURVE('',#3088,#3089,#2061,.T.);
#4131=EDGE_CURVE('',#3089,#3090,#324,.T.);
#4132=EDGE_CURVE('',#3090,#3085,#325,.T.);
#4133=EDGE_CURVE('',#3091,#3084,#326,.T.);
#4134=EDGE_CURVE('',#3088,#3091,#327,.T.);
#4135=EDGE_CURVE('',#3092,#3093,#2062,.T.);
#4136=EDGE_CURVE('',#3093,#3094,#328,.T.);
#4137=EDGE_CURVE('',#3094,#3089,#329,.T.);
#4138=EDGE_CURVE('',#3095,#3088,#330,.T.);
#4139=EDGE_CURVE('',#3092,#3095,#331,.T.);
#4140=EDGE_CURVE('',#3096,#3097,#2063,.T.);
#4141=EDGE_CURVE('',#3097,#3098,#332,.T.);
#4142=EDGE_CURVE('',#3098,#3093,#333,.T.);
#4143=EDGE_CURVE('',#3099,#3092,#334,.T.);
#4144=EDGE_CURVE('',#3096,#3099,#335,.T.);
#4145=EDGE_CURVE('',#3100,#3101,#2064,.T.);
#4146=EDGE_CURVE('',#3101,#3102,#336,.T.);
#4147=EDGE_CURVE('',#3102,#3097,#337,.T.);
#4148=EDGE_CURVE('',#3103,#3096,#338,.T.);
#4149=EDGE_CURVE('',#3100,#3103,#339,.T.);
#4150=EDGE_CURVE('',#3104,#3105,#2065,.T.);
#4151=EDGE_CURVE('',#3105,#3106,#340,.T.);
#4152=EDGE_CURVE('',#3106,#3101,#341,.T.);
#4153=EDGE_CURVE('',#3107,#3100,#342,.T.);
#4154=EDGE_CURVE('',#3104,#3107,#343,.T.);
#4155=EDGE_CURVE('',#3108,#3109,#2066,.T.);
#4156=EDGE_CURVE('',#3109,#3110,#344,.T.);
#4157=EDGE_CURVE('',#3110,#3105,#345,.T.);
#4158=EDGE_CURVE('',#3111,#3104,#346,.T.);
#4159=EDGE_CURVE('',#3108,#3111,#347,.T.);
#4160=EDGE_CURVE('',#3112,#3113,#2067,.T.);
#4161=EDGE_CURVE('',#3113,#3114,#348,.T.);
#4162=EDGE_CURVE('',#3114,#3109,#349,.T.);
#4163=EDGE_CURVE('',#3115,#3108,#350,.T.);
#4164=EDGE_CURVE('',#3112,#3115,#351,.T.);
#4165=EDGE_CURVE('',#3116,#3117,#2068,.T.);
#4166=EDGE_CURVE('',#3117,#3118,#352,.T.);
#4167=EDGE_CURVE('',#3118,#3113,#353,.T.);
#4168=EDGE_CURVE('',#3119,#3112,#354,.T.);
#4169=EDGE_CURVE('',#3116,#3119,#355,.T.);
#4170=EDGE_CURVE('',#3120,#3121,#2069,.T.);
#4171=EDGE_CURVE('',#3121,#3122,#356,.T.);
#4172=EDGE_CURVE('',#3122,#3117,#357,.T.);
#4173=EDGE_CURVE('',#3123,#3116,#358,.T.);
#4174=EDGE_CURVE('',#3120,#3123,#359,.T.);
#4175=EDGE_CURVE('',#3124,#3125,#2070,.T.);
#4176=EDGE_CURVE('',#3125,#3126,#360,.T.);
#4177=EDGE_CURVE('',#3126,#3121,#361,.T.);
#4178=EDGE_CURVE('',#3127,#3120,#362,.T.);
#4179=EDGE_CURVE('',#3124,#3127,#363,.T.);
#4180=EDGE_CURVE('',#3128,#3129,#2071,.T.);
#4181=EDGE_CURVE('',#3129,#3130,#364,.T.);
#4182=EDGE_CURVE('',#3130,#3125,#365,.T.);
#4183=EDGE_CURVE('',#3131,#3124,#366,.T.);
#4184=EDGE_CURVE('',#3128,#3131,#367,.T.);
#4185=EDGE_CURVE('',#3132,#3133,#2072,.T.);
#4186=EDGE_CURVE('',#3133,#3134,#368,.T.);
#4187=EDGE_CURVE('',#3134,#3129,#369,.T.);
#4188=EDGE_CURVE('',#3135,#3128,#370,.T.);
#4189=EDGE_CURVE('',#3132,#3135,#371,.T.);
#4190=EDGE_CURVE('',#3136,#3137,#2073,.T.);
#4191=EDGE_CURVE('',#3137,#3138,#372,.T.);
#4192=EDGE_CURVE('',#3138,#3133,#373,.T.);
#4193=EDGE_CURVE('',#3139,#3132,#374,.T.);
#4194=EDGE_CURVE('',#3136,#3139,#375,.T.);
#4195=EDGE_CURVE('',#3140,#3141,#2074,.T.);
#4196=EDGE_CURVE('',#3141,#3142,#376,.T.);
#4197=EDGE_CURVE('',#3142,#3137,#377,.T.);
#4198=EDGE_CURVE('',#3143,#3136,#378,.T.);
#4199=EDGE_CURVE('',#3140,#3143,#379,.T.);
#4200=EDGE_CURVE('',#3144,#3145,#2075,.T.);
#4201=EDGE_CURVE('',#3146,#3144,#380,.T.);
#4202=EDGE_CURVE('',#3147,#3146,#381,.T.);
#4203=EDGE_CURVE('',#3148,#3147,#2763,.T.);
#4204=EDGE_CURVE('',#3148,#3149,#382,.T.);
#4205=EDGE_CURVE('',#3149,#3145,#383,.T.);
#4206=EDGE_CURVE('',#3150,#3151,#2076,.T.);
#4207=EDGE_CURVE('',#3151,#3152,#384,.T.);
#4208=EDGE_CURVE('',#3152,#3153,#2764,.T.);
#4209=EDGE_CURVE('',#3153,#3154,#2077,.T.);
#4210=EDGE_CURVE('',#3154,#3154,#2765,.F.);
#4211=EDGE_CURVE('',#3153,#3155,#2766,.T.);
#4212=EDGE_CURVE('',#3155,#3150,#385,.T.);
#4213=EDGE_CURVE('',#3156,#3157,#2078,.T.);
#4214=EDGE_CURVE('',#3157,#3158,#386,.T.);
#4215=EDGE_CURVE('',#3158,#3151,#387,.T.);
#4216=EDGE_CURVE('',#3150,#3159,#388,.T.);
#4217=EDGE_CURVE('',#3159,#3156,#389,.T.);
#4218=EDGE_CURVE('',#3160,#3161,#2079,.T.);
#4219=EDGE_CURVE('',#3161,#3162,#390,.T.);
#4220=EDGE_CURVE('',#3162,#3157,#391,.T.);
#4221=EDGE_CURVE('',#3156,#3163,#392,.T.);
#4222=EDGE_CURVE('',#3163,#3160,#393,.T.);
#4223=EDGE_CURVE('',#3164,#3165,#2080,.T.);
#4224=EDGE_CURVE('',#3165,#3166,#394,.T.);
#4225=EDGE_CURVE('',#3166,#3161,#395,.T.);
#4226=EDGE_CURVE('',#3160,#3164,#396,.T.);
#4227=EDGE_CURVE('',#3167,#3168,#2081,.T.);
#4228=EDGE_CURVE('',#3168,#3169,#397,.T.);
#4229=EDGE_CURVE('',#3169,#3165,#398,.T.);
#4230=EDGE_CURVE('',#3164,#3170,#399,.T.);
#4231=EDGE_CURVE('',#3170,#3167,#400,.T.);
#4232=EDGE_CURVE('',#3171,#3172,#2082,.T.);
#4233=EDGE_CURVE('',#3172,#3173,#401,.T.);
#4234=EDGE_CURVE('',#3173,#3168,#402,.T.);
#4235=EDGE_CURVE('',#3167,#3171,#403,.T.);
#4236=EDGE_CURVE('',#3174,#3175,#2083,.T.);
#4237=EDGE_CURVE('',#3175,#3176,#404,.T.);
#4238=EDGE_CURVE('',#3176,#3172,#405,.T.);
#4239=EDGE_CURVE('',#3171,#3177,#406,.T.);
#4240=EDGE_CURVE('',#3177,#3174,#407,.T.);
#4241=EDGE_CURVE('',#3178,#3179,#2084,.T.);
#4242=EDGE_CURVE('',#3179,#3180,#408,.T.);
#4243=EDGE_CURVE('',#3180,#3175,#409,.T.);
#4244=EDGE_CURVE('',#3174,#3178,#410,.T.);
#4245=EDGE_CURVE('',#3181,#3182,#2085,.T.);
#4246=EDGE_CURVE('',#3182,#3183,#411,.T.);
#4247=EDGE_CURVE('',#3183,#3179,#412,.T.);
#4248=EDGE_CURVE('',#3178,#3184,#413,.T.);
#4249=EDGE_CURVE('',#3184,#3181,#414,.T.);
#4250=EDGE_CURVE('',#3185,#3186,#2086,.T.);
#4251=EDGE_CURVE('',#3186,#3187,#415,.T.);
#4252=EDGE_CURVE('',#3187,#3182,#416,.T.);
#4253=EDGE_CURVE('',#3181,#3185,#417,.T.);
#4254=EDGE_CURVE('',#3188,#3189,#2087,.T.);
#4255=EDGE_CURVE('',#3189,#3190,#418,.T.);
#4256=EDGE_CURVE('',#3190,#3186,#419,.T.);
#4257=EDGE_CURVE('',#3185,#3191,#420,.T.);
#4258=EDGE_CURVE('',#3191,#3188,#421,.T.);
#4259=EDGE_CURVE('',#3192,#3193,#2088,.T.);
#4260=EDGE_CURVE('',#3193,#3194,#422,.T.);
#4261=EDGE_CURVE('',#3194,#3189,#423,.T.);
#4262=EDGE_CURVE('',#3188,#3192,#424,.T.);
#4263=EDGE_CURVE('',#3195,#3196,#2089,.T.);
#4264=EDGE_CURVE('',#3196,#3197,#425,.T.);
#4265=EDGE_CURVE('',#3197,#3193,#426,.T.);
#4266=EDGE_CURVE('',#3192,#3198,#427,.T.);
#4267=EDGE_CURVE('',#3198,#3195,#428,.T.);
#4268=EDGE_CURVE('',#3199,#3200,#2090,.T.);
#4269=EDGE_CURVE('',#3200,#3201,#429,.T.);
#4270=EDGE_CURVE('',#3201,#3196,#430,.T.);
#4271=EDGE_CURVE('',#3195,#3199,#431,.T.);
#4272=EDGE_CURVE('',#3202,#3203,#2091,.T.);
#4273=EDGE_CURVE('',#3203,#3204,#432,.T.);
#4274=EDGE_CURVE('',#3204,#3200,#433,.T.);
#4275=EDGE_CURVE('',#3199,#3205,#434,.T.);
#4276=EDGE_CURVE('',#3205,#3202,#435,.T.);
#4277=EDGE_CURVE('',#3206,#3207,#2092,.T.);
#4278=EDGE_CURVE('',#3207,#3208,#436,.T.);
#4279=EDGE_CURVE('',#3208,#3203,#437,.T.);
#4280=EDGE_CURVE('',#3202,#3206,#438,.T.);
#4281=EDGE_CURVE('',#3209,#3210,#2093,.T.);
#4282=EDGE_CURVE('',#3210,#3211,#439,.T.);
#4283=EDGE_CURVE('',#3211,#3207,#440,.T.);
#4284=EDGE_CURVE('',#3206,#3212,#441,.T.);
#4285=EDGE_CURVE('',#3212,#3209,#442,.T.);
#4286=EDGE_CURVE('',#3213,#3214,#2094,.T.);
#4287=EDGE_CURVE('',#3214,#3215,#443,.T.);
#4288=EDGE_CURVE('',#3215,#3210,#444,.T.);
#4289=EDGE_CURVE('',#3209,#3213,#445,.T.);
#4290=EDGE_CURVE('',#3216,#3217,#2095,.T.);
#4291=EDGE_CURVE('',#3216,#3218,#446,.T.);
#4292=EDGE_CURVE('',#3218,#3219,#447,.T.);
#4293=EDGE_CURVE('',#3220,#3219,#2767,.T.);
#4294=EDGE_CURVE('',#3220,#3221,#448,.T.);
#4295=EDGE_CURVE('',#3221,#3217,#449,.T.);
#4296=EDGE_CURVE('',#3217,#3222,#450,.T.);
#4297=EDGE_CURVE('',#3222,#3214,#451,.T.);
#4298=EDGE_CURVE('',#3213,#3223,#452,.T.);
#4299=EDGE_CURVE('',#3223,#3216,#453,.T.);
#4300=EDGE_CURVE('',#3145,#3224,#454,.T.);
#4301=EDGE_CURVE('',#3224,#3141,#455,.T.);
#4302=EDGE_CURVE('',#3225,#3140,#456,.T.);
#4303=EDGE_CURVE('',#3144,#3225,#457,.T.);
#4304=EDGE_CURVE('',#3067,#3226,#458,.T.);
#4305=EDGE_CURVE('',#3226,#3063,#459,.T.);
#4306=EDGE_CURVE('',#3062,#3066,#460,.T.);
#4307=EDGE_CURVE('',#2995,#3227,#461,.T.);
#4308=EDGE_CURVE('',#3227,#2991,#462,.T.);
#4309=EDGE_CURVE('',#3228,#2990,#463,.T.);
#4310=EDGE_CURVE('',#2994,#3228,#464,.T.);
#4311=EDGE_CURVE('',#3002,#2925,#465,.T.);
#4312=EDGE_CURVE('',#2924,#3005,#466,.T.);
#4313=EDGE_CURVE('',#3069,#2998,#467,.T.);
#4314=EDGE_CURVE('',#2997,#3070,#468,.T.);
#4315=EDGE_CURVE('',#3152,#3075,#469,.T.);
#4316=EDGE_CURVE('',#3074,#3155,#470,.T.);
#4317=EDGE_CURVE('',#3219,#3148,#471,.T.);
#4318=EDGE_CURVE('',#3147,#3220,#472,.T.);
#4319=EDGE_CURVE('',#3229,#3229,#2768,.T.);
#4320=EDGE_CURVE('',#3229,#3230,#2096,.T.);
#4321=EDGE_CURVE('',#3230,#3230,#2769,.T.);
#5322=ORIENTED_EDGE('',*,*,#3926,.T.);
#5323=ORIENTED_EDGE('',*,*,#3927,.T.);
#5324=ORIENTED_EDGE('',*,*,#3928,.F.);
#5325=ORIENTED_EDGE('',*,*,#3929,.F.);
#5326=ORIENTED_EDGE('',*,*,#3930,.T.);
#5327=ORIENTED_EDGE('',*,*,#3931,.T.);
#5328=ORIENTED_EDGE('',*,*,#3932,.T.);
#5329=ORIENTED_EDGE('',*,*,#3926,.F.);
#5330=ORIENTED_EDGE('',*,*,#3933,.F.);
#5331=ORIENTED_EDGE('',*,*,#3934,.F.);
#5332=ORIENTED_EDGE('',*,*,#3935,.T.);
#5333=ORIENTED_EDGE('',*,*,#3936,.T.);
#5334=ORIENTED_EDGE('',*,*,#3937,.T.);
#5335=ORIENTED_EDGE('',*,*,#3930,.F.);
#5336=ORIENTED_EDGE('',*,*,#3938,.F.);
#5337=ORIENTED_EDGE('',*,*,#3939,.F.);
#5338=ORIENTED_EDGE('',*,*,#3940,.T.);
#5339=ORIENTED_EDGE('',*,*,#3941,.T.);
#5340=ORIENTED_EDGE('',*,*,#3942,.T.);
#5341=ORIENTED_EDGE('',*,*,#3935,.F.);
#5342=ORIENTED_EDGE('',*,*,#3943,.F.);
#5343=ORIENTED_EDGE('',*,*,#3944,.F.);
#5344=ORIENTED_EDGE('',*,*,#3945,.T.);
#5345=ORIENTED_EDGE('',*,*,#3946,.T.);
#5346=ORIENTED_EDGE('',*,*,#3947,.T.);
#5347=ORIENTED_EDGE('',*,*,#3940,.F.);
#5348=ORIENTED_EDGE('',*,*,#3948,.F.);
#5349=ORIENTED_EDGE('',*,*,#3949,.F.);
#5350=ORIENTED_EDGE('',*,*,#3950,.T.);
#5351=ORIENTED_EDGE('',*,*,#3951,.T.);
#5352=ORIENTED_EDGE('',*,*,#3952,.T.);
#5353=ORIENTED_EDGE('',*,*,#3945,.F.);
#5354=ORIENTED_EDGE('',*,*,#3953,.F.);
#5355=ORIENTED_EDGE('',*,*,#3954,.F.);
#5356=ORIENTED_EDGE('',*,*,#3955,.T.);
#5357=ORIENTED_EDGE('',*,*,#3956,.T.);
#5358=ORIENTED_EDGE('',*,*,#3957,.T.);
#5359=ORIENTED_EDGE('',*,*,#3950,.F.);
#5360=ORIENTED_EDGE('',*,*,#3958,.F.);
#5361=ORIENTED_EDGE('',*,*,#3959,.F.);
#5362=ORIENTED_EDGE('',*,*,#3960,.T.);
#5363=ORIENTED_EDGE('',*,*,#3961,.T.);
#5364=ORIENTED_EDGE('',*,*,#3962,.T.);
#5365=ORIENTED_EDGE('',*,*,#3955,.F.);
#5366=ORIENTED_EDGE('',*,*,#3963,.F.);
#5367=ORIENTED_EDGE('',*,*,#3964,.F.);
#5368=ORIENTED_EDGE('',*,*,#3965,.T.);
#5369=ORIENTED_EDGE('',*,*,#3966,.T.);
#5370=ORIENTED_EDGE('',*,*,#3967,.T.);
#5371=ORIENTED_EDGE('',*,*,#3960,.F.);
#5372=ORIENTED_EDGE('',*,*,#3968,.F.);
#5373=ORIENTED_EDGE('',*,*,#3969,.F.);
#5374=ORIENTED_EDGE('',*,*,#3970,.T.);
#5375=ORIENTED_EDGE('',*,*,#3971,.T.);
#5376=ORIENTED_EDGE('',*,*,#3972,.T.);
#5377=ORIENTED_EDGE('',*,*,#3965,.F.);
#5378=ORIENTED_EDGE('',*,*,#3973,.F.);
#5379=ORIENTED_EDGE('',*,*,#3974,.F.);
#5380=ORIENTED_EDGE('',*,*,#3975,.T.);
#5381=ORIENTED_EDGE('',*,*,#3976,.T.);
#5382=ORIENTED_EDGE('',*,*,#3977,.T.);
#5383=ORIENTED_EDGE('',*,*,#3970,.F.);
#5384=ORIENTED_EDGE('',*,*,#3978,.F.);
#5385=ORIENTED_EDGE('',*,*,#3979,.F.);
#5386=ORIENTED_EDGE('',*,*,#3980,.T.);
#5387=ORIENTED_EDGE('',*,*,#3981,.T.);
#5388=ORIENTED_EDGE('',*,*,#3982,.T.);
#5389=ORIENTED_EDGE('',*,*,#3975,.F.);
#5390=ORIENTED_EDGE('',*,*,#3983,.F.);
#5391=ORIENTED_EDGE('',*,*,#3984,.F.);
#5392=ORIENTED_EDGE('',*,*,#3985,.T.);
#5393=ORIENTED_EDGE('',*,*,#3986,.T.);
#5394=ORIENTED_EDGE('',*,*,#3987,.T.);
#5395=ORIENTED_EDGE('',*,*,#3980,.F.);
#5396=ORIENTED_EDGE('',*,*,#3988,.F.);
#5397=ORIENTED_EDGE('',*,*,#3989,.F.);
#5398=ORIENTED_EDGE('',*,*,#3990,.T.);
#5399=ORIENTED_EDGE('',*,*,#3991,.T.);
#5400=ORIENTED_EDGE('',*,*,#3992,.T.);
#5401=ORIENTED_EDGE('',*,*,#3985,.F.);
#5402=ORIENTED_EDGE('',*,*,#3993,.F.);
#5403=ORIENTED_EDGE('',*,*,#3994,.F.);
#5404=ORIENTED_EDGE('',*,*,#3995,.T.);
#5405=ORIENTED_EDGE('',*,*,#3996,.T.);
#5406=ORIENTED_EDGE('',*,*,#3997,.T.);
#5407=ORIENTED_EDGE('',*,*,#3990,.F.);
#5408=ORIENTED_EDGE('',*,*,#3998,.F.);
#5409=ORIENTED_EDGE('',*,*,#3999,.F.);
#5410=ORIENTED_EDGE('',*,*,#4000,.T.);
#5411=ORIENTED_EDGE('',*,*,#4001,.T.);
#5412=ORIENTED_EDGE('',*,*,#4002,.T.);
#5413=ORIENTED_EDGE('',*,*,#3995,.F.);
#5414=ORIENTED_EDGE('',*,*,#4003,.F.);
#5415=ORIENTED_EDGE('',*,*,#4004,.F.);
#5416=ORIENTED_EDGE('',*,*,#4005,.T.);
#5417=ORIENTED_EDGE('',*,*,#4006,.T.);
#5418=ORIENTED_EDGE('',*,*,#4007,.T.);
#5419=ORIENTED_EDGE('',*,*,#4000,.F.);
#5420=ORIENTED_EDGE('',*,*,#4008,.F.);
#5421=ORIENTED_EDGE('',*,*,#4009,.F.);
#5422=ORIENTED_EDGE('',*,*,#4010,.T.);
#5423=ORIENTED_EDGE('',*,*,#4011,.T.);
#5424=ORIENTED_EDGE('',*,*,#4012,.T.);
#5425=ORIENTED_EDGE('',*,*,#4005,.F.);
#5426=ORIENTED_EDGE('',*,*,#4013,.F.);
#5427=ORIENTED_EDGE('',*,*,#4014,.F.);
#5428=ORIENTED_EDGE('',*,*,#4015,.F.);
#5429=ORIENTED_EDGE('',*,*,#4016,.F.);
#5430=ORIENTED_EDGE('',*,*,#4017,.F.);
#5431=ORIENTED_EDGE('',*,*,#4018,.F.);
#5432=ORIENTED_EDGE('',*,*,#4019,.T.);
#5433=ORIENTED_EDGE('',*,*,#4020,.T.);
#5434=ORIENTED_EDGE('',*,*,#4021,.T.);
#5435=ORIENTED_EDGE('',*,*,#4022,.T.);
#5436=ORIENTED_EDGE('',*,*,#4023,.T.);
#5437=ORIENTED_EDGE('',*,*,#4024,.T.);
#5438=ORIENTED_EDGE('',*,*,#4025,.T.);
#5439=ORIENTED_EDGE('',*,*,#4024,.F.);
#5440=ORIENTED_EDGE('',*,*,#4026,.T.);
#5441=ORIENTED_EDGE('',*,*,#4027,.T.);
#5442=ORIENTED_EDGE('',*,*,#4028,.T.);
#5443=ORIENTED_EDGE('',*,*,#4029,.T.);
#5444=ORIENTED_EDGE('',*,*,#4030,.T.);
#5445=ORIENTED_EDGE('',*,*,#4021,.F.);
#5446=ORIENTED_EDGE('',*,*,#4031,.T.);
#5447=ORIENTED_EDGE('',*,*,#4032,.T.);
#5448=ORIENTED_EDGE('',*,*,#4033,.T.);
#5449=ORIENTED_EDGE('',*,*,#4034,.T.);
#5450=ORIENTED_EDGE('',*,*,#4035,.T.);
#5451=ORIENTED_EDGE('',*,*,#4028,.F.);
#5452=ORIENTED_EDGE('',*,*,#4036,.T.);
#5453=ORIENTED_EDGE('',*,*,#4037,.T.);
#5454=ORIENTED_EDGE('',*,*,#4038,.T.);
#5455=ORIENTED_EDGE('',*,*,#4039,.T.);
#5456=ORIENTED_EDGE('',*,*,#4033,.F.);
#5457=ORIENTED_EDGE('',*,*,#4040,.T.);
#5458=ORIENTED_EDGE('',*,*,#4041,.T.);
#5459=ORIENTED_EDGE('',*,*,#4042,.T.);
#5460=ORIENTED_EDGE('',*,*,#4043,.T.);
#5461=ORIENTED_EDGE('',*,*,#4044,.T.);
#5462=ORIENTED_EDGE('',*,*,#4037,.F.);
#5463=ORIENTED_EDGE('',*,*,#4045,.T.);
#5464=ORIENTED_EDGE('',*,*,#4046,.T.);
#5465=ORIENTED_EDGE('',*,*,#4047,.T.);
#5466=ORIENTED_EDGE('',*,*,#4048,.T.);
#5467=ORIENTED_EDGE('',*,*,#4042,.F.);
#5468=ORIENTED_EDGE('',*,*,#4049,.T.);
#5469=ORIENTED_EDGE('',*,*,#4050,.T.);
#5470=ORIENTED_EDGE('',*,*,#4051,.T.);
#5471=ORIENTED_EDGE('',*,*,#4052,.T.);
#5472=ORIENTED_EDGE('',*,*,#4053,.T.);
#5473=ORIENTED_EDGE('',*,*,#4046,.F.);
#5474=ORIENTED_EDGE('',*,*,#4054,.T.);
#5475=ORIENTED_EDGE('',*,*,#4055,.T.);
#5476=ORIENTED_EDGE('',*,*,#4056,.T.);
#5477=ORIENTED_EDGE('',*,*,#4057,.T.);
#5478=ORIENTED_EDGE('',*,*,#4051,.F.);
#5479=ORIENTED_EDGE('',*,*,#4058,.T.);
#5480=ORIENTED_EDGE('',*,*,#4059,.T.);
#5481=ORIENTED_EDGE('',*,*,#4060,.T.);
#5482=ORIENTED_EDGE('',*,*,#4061,.T.);
#5483=ORIENTED_EDGE('',*,*,#4062,.T.);
#5484=ORIENTED_EDGE('',*,*,#4055,.F.);
#5485=ORIENTED_EDGE('',*,*,#4063,.T.);
#5486=ORIENTED_EDGE('',*,*,#4064,.T.);
#5487=ORIENTED_EDGE('',*,*,#4065,.T.);
#5488=ORIENTED_EDGE('',*,*,#4066,.T.);
#5489=ORIENTED_EDGE('',*,*,#4060,.F.);
#5490=ORIENTED_EDGE('',*,*,#4067,.T.);
#5491=ORIENTED_EDGE('',*,*,#4068,.T.);
#5492=ORIENTED_EDGE('',*,*,#4069,.T.);
#5493=ORIENTED_EDGE('',*,*,#4070,.T.);
#5494=ORIENTED_EDGE('',*,*,#4071,.T.);
#5495=ORIENTED_EDGE('',*,*,#4064,.F.);
#5496=ORIENTED_EDGE('',*,*,#4072,.T.);
#5497=ORIENTED_EDGE('',*,*,#4073,.T.);
#5498=ORIENTED_EDGE('',*,*,#4074,.T.);
#5499=ORIENTED_EDGE('',*,*,#4075,.T.);
#5500=ORIENTED_EDGE('',*,*,#4069,.F.);
#5501=ORIENTED_EDGE('',*,*,#4076,.T.);
#5502=ORIENTED_EDGE('',*,*,#4077,.T.);
#5503=ORIENTED_EDGE('',*,*,#4078,.T.);
#5504=ORIENTED_EDGE('',*,*,#4079,.T.);
#5505=ORIENTED_EDGE('',*,*,#4080,.T.);
#5506=ORIENTED_EDGE('',*,*,#4073,.F.);
#5507=ORIENTED_EDGE('',*,*,#4081,.T.);
#5508=ORIENTED_EDGE('',*,*,#4082,.T.);
#5509=ORIENTED_EDGE('',*,*,#4083,.T.);
#5510=ORIENTED_EDGE('',*,*,#4084,.T.);
#5511=ORIENTED_EDGE('',*,*,#4078,.F.);
#5512=ORIENTED_EDGE('',*,*,#4085,.T.);
#5513=ORIENTED_EDGE('',*,*,#4086,.T.);
#5514=ORIENTED_EDGE('',*,*,#4087,.T.);
#5515=ORIENTED_EDGE('',*,*,#4088,.T.);
#5516=ORIENTED_EDGE('',*,*,#4089,.T.);
#5517=ORIENTED_EDGE('',*,*,#4082,.F.);
#5518=ORIENTED_EDGE('',*,*,#4090,.T.);
#5519=ORIENTED_EDGE('',*,*,#4091,.T.);
#5520=ORIENTED_EDGE('',*,*,#4092,.T.);
#5521=ORIENTED_EDGE('',*,*,#4093,.T.);
#5522=ORIENTED_EDGE('',*,*,#4087,.F.);
#5523=ORIENTED_EDGE('',*,*,#4094,.T.);
#5524=ORIENTED_EDGE('',*,*,#4095,.T.);
#5525=ORIENTED_EDGE('',*,*,#4096,.T.);
#5526=ORIENTED_EDGE('',*,*,#4097,.T.);
#5527=ORIENTED_EDGE('',*,*,#4098,.T.);
#5528=ORIENTED_EDGE('',*,*,#4091,.F.);
#5529=ORIENTED_EDGE('',*,*,#4099,.T.);
#5530=ORIENTED_EDGE('',*,*,#4100,.T.);
#5531=ORIENTED_EDGE('',*,*,#4101,.T.);
#5532=ORIENTED_EDGE('',*,*,#4102,.T.);
#5533=ORIENTED_EDGE('',*,*,#4096,.F.);
#5534=ORIENTED_EDGE('',*,*,#4103,.T.);
#5535=ORIENTED_EDGE('',*,*,#4104,.T.);
#5536=ORIENTED_EDGE('',*,*,#4105,.F.);
#5537=ORIENTED_EDGE('',*,*,#4106,.T.);
#5538=ORIENTED_EDGE('',*,*,#4107,.T.);
#5539=ORIENTED_EDGE('',*,*,#4108,.F.);
#5540=ORIENTED_EDGE('',*,*,#4109,.T.);
#5541=ORIENTED_EDGE('',*,*,#4110,.T.);
#5542=ORIENTED_EDGE('',*,*,#4111,.T.);
#5543=ORIENTED_EDGE('',*,*,#4112,.T.);
#5544=ORIENTED_EDGE('',*,*,#4113,.F.);
#5545=ORIENTED_EDGE('',*,*,#4114,.F.);
#5546=ORIENTED_EDGE('',*,*,#4115,.T.);
#5547=ORIENTED_EDGE('',*,*,#4116,.T.);
#5548=ORIENTED_EDGE('',*,*,#4117,.T.);
#5549=ORIENTED_EDGE('',*,*,#4111,.F.);
#5550=ORIENTED_EDGE('',*,*,#4118,.F.);
#5551=ORIENTED_EDGE('',*,*,#4119,.F.);
#5552=ORIENTED_EDGE('',*,*,#4120,.T.);
#5553=ORIENTED_EDGE('',*,*,#4121,.T.);
#5554=ORIENTED_EDGE('',*,*,#4122,.T.);
#5555=ORIENTED_EDGE('',*,*,#4115,.F.);
#5556=ORIENTED_EDGE('',*,*,#4123,.F.);
#5557=ORIENTED_EDGE('',*,*,#4124,.F.);
#5558=ORIENTED_EDGE('',*,*,#4125,.T.);
#5559=ORIENTED_EDGE('',*,*,#4126,.T.);
#5560=ORIENTED_EDGE('',*,*,#4127,.T.);
#5561=ORIENTED_EDGE('',*,*,#4120,.F.);
#5562=ORIENTED_EDGE('',*,*,#4128,.F.);
#5563=ORIENTED_EDGE('',*,*,#4129,.F.);
#5564=ORIENTED_EDGE('',*,*,#4130,.T.);
#5565=ORIENTED_EDGE('',*,*,#4131,.T.);
#5566=ORIENTED_EDGE('',*,*,#4132,.T.);
#5567=ORIENTED_EDGE('',*,*,#4125,.F.);
#5568=ORIENTED_EDGE('',*,*,#4133,.F.);
#5569=ORIENTED_EDGE('',*,*,#4134,.F.);
#5570=ORIENTED_EDGE('',*,*,#4135,.T.);
#5571=ORIENTED_EDGE('',*,*,#4136,.T.);
#5572=ORIENTED_EDGE('',*,*,#4137,.T.);
#5573=ORIENTED_EDGE('',*,*,#4130,.F.);
#5574=ORIENTED_EDGE('',*,*,#4138,.F.);
#5575=ORIENTED_EDGE('',*,*,#4139,.F.);
#5576=ORIENTED_EDGE('',*,*,#4140,.T.);
#5577=ORIENTED_EDGE('',*,*,#4141,.T.);
#5578=ORIENTED_EDGE('',*,*,#4142,.T.);
#5579=ORIENTED_EDGE('',*,*,#4135,.F.);
#5580=ORIENTED_EDGE('',*,*,#4143,.F.);
#5581=ORIENTED_EDGE('',*,*,#4144,.F.);
#5582=ORIENTED_EDGE('',*,*,#4145,.T.);
#5583=ORIENTED_EDGE('',*,*,#4146,.T.);
#5584=ORIENTED_EDGE('',*,*,#4147,.T.);
#5585=ORIENTED_EDGE('',*,*,#4140,.F.);
#5586=ORIENTED_EDGE('',*,*,#4148,.F.);
#5587=ORIENTED_EDGE('',*,*,#4149,.F.);
#5588=ORIENTED_EDGE('',*,*,#4150,.T.);
#5589=ORIENTED_EDGE('',*,*,#4151,.T.);
#5590=ORIENTED_EDGE('',*,*,#4152,.T.);
#5591=ORIENTED_EDGE('',*,*,#4145,.F.);
#5592=ORIENTED_EDGE('',*,*,#4153,.F.);
#5593=ORIENTED_EDGE('',*,*,#4154,.F.);
#5594=ORIENTED_EDGE('',*,*,#4155,.T.);
#5595=ORIENTED_EDGE('',*,*,#4156,.T.);
#5596=ORIENTED_EDGE('',*,*,#4157,.T.);
#5597=ORIENTED_EDGE('',*,*,#4150,.F.);
#5598=ORIENTED_EDGE('',*,*,#4158,.F.);
#5599=ORIENTED_EDGE('',*,*,#4159,.F.);
#5600=ORIENTED_EDGE('',*,*,#4160,.T.);
#5601=ORIENTED_EDGE('',*,*,#4161,.T.);
#5602=ORIENTED_EDGE('',*,*,#4162,.T.);
#5603=ORIENTED_EDGE('',*,*,#4155,.F.);
#5604=ORIENTED_EDGE('',*,*,#4163,.F.);
#5605=ORIENTED_EDGE('',*,*,#4164,.F.);
#5606=ORIENTED_EDGE('',*,*,#4165,.T.);
#5607=ORIENTED_EDGE('',*,*,#4166,.T.);
#5608=ORIENTED_EDGE('',*,*,#4167,.T.);
#5609=ORIENTED_EDGE('',*,*,#4160,.F.);
#5610=ORIENTED_EDGE('',*,*,#4168,.F.);
#5611=ORIENTED_EDGE('',*,*,#4169,.F.);
#5612=ORIENTED_EDGE('',*,*,#4170,.T.);
#5613=ORIENTED_EDGE('',*,*,#4171,.T.);
#5614=ORIENTED_EDGE('',*,*,#4172,.T.);
#5615=ORIENTED_EDGE('',*,*,#4165,.F.);
#5616=ORIENTED_EDGE('',*,*,#4173,.F.);
#5617=ORIENTED_EDGE('',*,*,#4174,.F.);
#5618=ORIENTED_EDGE('',*,*,#4175,.T.);
#5619=ORIENTED_EDGE('',*,*,#4176,.T.);
#5620=ORIENTED_EDGE('',*,*,#4177,.T.);
#5621=ORIENTED_EDGE('',*,*,#4170,.F.);
#5622=ORIENTED_EDGE('',*,*,#4178,.F.);
#5623=ORIENTED_EDGE('',*,*,#4179,.F.);
#5624=ORIENTED_EDGE('',*,*,#4180,.T.);
#5625=ORIENTED_EDGE('',*,*,#4181,.T.);
#5626=ORIENTED_EDGE('',*,*,#4182,.T.);
#5627=ORIENTED_EDGE('',*,*,#4175,.F.);
#5628=ORIENTED_EDGE('',*,*,#4183,.F.);
#5629=ORIENTED_EDGE('',*,*,#4184,.F.);
#5630=ORIENTED_EDGE('',*,*,#4185,.T.);
#5631=ORIENTED_EDGE('',*,*,#4186,.T.);
#5632=ORIENTED_EDGE('',*,*,#4187,.T.);
#5633=ORIENTED_EDGE('',*,*,#4180,.F.);
#5634=ORIENTED_EDGE('',*,*,#4188,.F.);
#5635=ORIENTED_EDGE('',*,*,#4189,.F.);
#5636=ORIENTED_EDGE('',*,*,#4190,.T.);
#5637=ORIENTED_EDGE('',*,*,#4191,.T.);
#5638=ORIENTED_EDGE('',*,*,#4192,.T.);
#5639=ORIENTED_EDGE('',*,*,#4185,.F.);
#5640=ORIENTED_EDGE('',*,*,#4193,.F.);
#5641=ORIENTED_EDGE('',*,*,#4194,.F.);
#5642=ORIENTED_EDGE('',*,*,#4195,.T.);
#5643=ORIENTED_EDGE('',*,*,#4196,.T.);
#5644=ORIENTED_EDGE('',*,*,#4197,.T.);
#5645=ORIENTED_EDGE('',*,*,#4190,.F.);
#5646=ORIENTED_EDGE('',*,*,#4198,.F.);
#5647=ORIENTED_EDGE('',*,*,#4199,.F.);
#5648=ORIENTED_EDGE('',*,*,#4200,.F.);
#5649=ORIENTED_EDGE('',*,*,#4201,.F.);
#5650=ORIENTED_EDGE('',*,*,#4202,.F.);
#5651=ORIENTED_EDGE('',*,*,#4203,.F.);
#5652=ORIENTED_EDGE('',*,*,#4204,.T.);
#5653=ORIENTED_EDGE('',*,*,#4205,.T.);
#5654=ORIENTED_EDGE('',*,*,#4206,.T.);
#5655=ORIENTED_EDGE('',*,*,#4207,.T.);
#5656=ORIENTED_EDGE('',*,*,#4208,.T.);
#5657=ORIENTED_EDGE('',*,*,#4209,.T.);
#5658=ORIENTED_EDGE('',*,*,#4210,.T.);
#5659=ORIENTED_EDGE('',*,*,#4209,.F.);
#5660=ORIENTED_EDGE('',*,*,#4211,.T.);
#5661=ORIENTED_EDGE('',*,*,#4212,.T.);
#5662=ORIENTED_EDGE('',*,*,#4213,.T.);
#5663=ORIENTED_EDGE('',*,*,#4214,.T.);
#5664=ORIENTED_EDGE('',*,*,#4215,.T.);
#5665=ORIENTED_EDGE('',*,*,#4206,.F.);
#5666=ORIENTED_EDGE('',*,*,#4216,.T.);
#5667=ORIENTED_EDGE('',*,*,#4217,.T.);
#5668=ORIENTED_EDGE('',*,*,#4218,.T.);
#5669=ORIENTED_EDGE('',*,*,#4219,.T.);
#5670=ORIENTED_EDGE('',*,*,#4220,.T.);
#5671=ORIENTED_EDGE('',*,*,#4213,.F.);
#5672=ORIENTED_EDGE('',*,*,#4221,.T.);
#5673=ORIENTED_EDGE('',*,*,#4222,.T.);
#5674=ORIENTED_EDGE('',*,*,#4223,.T.);
#5675=ORIENTED_EDGE('',*,*,#4224,.T.);
#5676=ORIENTED_EDGE('',*,*,#4225,.T.);
#5677=ORIENTED_EDGE('',*,*,#4218,.F.);
#5678=ORIENTED_EDGE('',*,*,#4226,.T.);
#5679=ORIENTED_EDGE('',*,*,#4227,.T.);
#5680=ORIENTED_EDGE('',*,*,#4228,.T.);
#5681=ORIENTED_EDGE('',*,*,#4229,.T.);
#5682=ORIENTED_EDGE('',*,*,#4223,.F.);
#5683=ORIENTED_EDGE('',*,*,#4230,.T.);
#5684=ORIENTED_EDGE('',*,*,#4231,.T.);
#5685=ORIENTED_EDGE('',*,*,#4232,.T.);
#5686=ORIENTED_EDGE('',*,*,#4233,.T.);
#5687=ORIENTED_EDGE('',*,*,#4234,.T.);
#5688=ORIENTED_EDGE('',*,*,#4227,.F.);
#5689=ORIENTED_EDGE('',*,*,#4235,.T.);
#5690=ORIENTED_EDGE('',*,*,#4236,.T.);
#5691=ORIENTED_EDGE('',*,*,#4237,.T.);
#5692=ORIENTED_EDGE('',*,*,#4238,.T.);
#5693=ORIENTED_EDGE('',*,*,#4232,.F.);
#5694=ORIENTED_EDGE('',*,*,#4239,.T.);
#5695=ORIENTED_EDGE('',*,*,#4240,.T.);
#5696=ORIENTED_EDGE('',*,*,#4241,.T.);
#5697=ORIENTED_EDGE('',*,*,#4242,.T.);
#5698=ORIENTED_EDGE('',*,*,#4243,.T.);
#5699=ORIENTED_EDGE('',*,*,#4236,.F.);
#5700=ORIENTED_EDGE('',*,*,#4244,.T.);
#5701=ORIENTED_EDGE('',*,*,#4245,.T.);
#5702=ORIENTED_EDGE('',*,*,#4246,.T.);
#5703=ORIENTED_EDGE('',*,*,#4247,.T.);
#5704=ORIENTED_EDGE('',*,*,#4241,.F.);
#5705=ORIENTED_EDGE('',*,*,#4248,.T.);
#5706=ORIENTED_EDGE('',*,*,#4249,.T.);
#5707=ORIENTED_EDGE('',*,*,#4250,.T.);
#5708=ORIENTED_EDGE('',*,*,#4251,.T.);
#5709=ORIENTED_EDGE('',*,*,#4252,.T.);
#5710=ORIENTED_EDGE('',*,*,#4245,.F.);
#5711=ORIENTED_EDGE('',*,*,#4253,.T.);
#5712=ORIENTED_EDGE('',*,*,#4254,.T.);
#5713=ORIENTED_EDGE('',*,*,#4255,.T.);
#5714=ORIENTED_EDGE('',*,*,#4256,.T.);
#5715=ORIENTED_EDGE('',*,*,#4250,.F.);
#5716=ORIENTED_EDGE('',*,*,#4257,.T.);
#5717=ORIENTED_EDGE('',*,*,#4258,.T.);
#5718=ORIENTED_EDGE('',*,*,#4259,.T.);
#5719=ORIENTED_EDGE('',*,*,#4260,.T.);
#5720=ORIENTED_EDGE('',*,*,#4261,.T.);
#5721=ORIENTED_EDGE('',*,*,#4254,.F.);
#5722=ORIENTED_EDGE('',*,*,#4262,.T.);
#5723=ORIENTED_EDGE('',*,*,#4263,.T.);
#5724=ORIENTED_EDGE('',*,*,#4264,.T.);
#5725=ORIENTED_EDGE('',*,*,#4265,.T.);
#5726=ORIENTED_EDGE('',*,*,#4259,.F.);
#5727=ORIENTED_EDGE('',*,*,#4266,.T.);
#5728=ORIENTED_EDGE('',*,*,#4267,.T.);
#5729=ORIENTED_EDGE('',*,*,#4268,.T.);
#5730=ORIENTED_EDGE('',*,*,#4269,.T.);
#5731=ORIENTED_EDGE('',*,*,#4270,.T.);
#5732=ORIENTED_EDGE('',*,*,#4263,.F.);
#5733=ORIENTED_EDGE('',*,*,#4271,.T.);
#5734=ORIENTED_EDGE('',*,*,#4272,.T.);
#5735=ORIENTED_EDGE('',*,*,#4273,.T.);
#5736=ORIENTED_EDGE('',*,*,#4274,.T.);
#5737=ORIENTED_EDGE('',*,*,#4268,.F.);
#5738=ORIENTED_EDGE('',*,*,#4275,.T.);
#5739=ORIENTED_EDGE('',*,*,#4276,.T.);
#5740=ORIENTED_EDGE('',*,*,#4277,.T.);
#5741=ORIENTED_EDGE('',*,*,#4278,.T.);
#5742=ORIENTED_EDGE('',*,*,#4279,.T.);
#5743=ORIENTED_EDGE('',*,*,#4272,.F.);
#5744=ORIENTED_EDGE('',*,*,#4280,.T.);
#5745=ORIENTED_EDGE('',*,*,#4281,.T.);
#5746=ORIENTED_EDGE('',*,*,#4282,.T.);
#5747=ORIENTED_EDGE('',*,*,#4283,.T.);
#5748=ORIENTED_EDGE('',*,*,#4277,.F.);
#5749=ORIENTED_EDGE('',*,*,#4284,.T.);
#5750=ORIENTED_EDGE('',*,*,#4285,.T.);
#5751=ORIENTED_EDGE('',*,*,#4286,.T.);
#5752=ORIENTED_EDGE('',*,*,#4287,.T.);
#5753=ORIENTED_EDGE('',*,*,#4288,.T.);
#5754=ORIENTED_EDGE('',*,*,#4281,.F.);
#5755=ORIENTED_EDGE('',*,*,#4289,.T.);
#5756=ORIENTED_EDGE('',*,*,#4290,.F.);
#5757=ORIENTED_EDGE('',*,*,#4291,.T.);
#5758=ORIENTED_EDGE('',*,*,#4292,.T.);
#5759=ORIENTED_EDGE('',*,*,#4293,.F.);
#5760=ORIENTED_EDGE('',*,*,#4294,.T.);
#5761=ORIENTED_EDGE('',*,*,#4295,.T.);
#5762=ORIENTED_EDGE('',*,*,#4290,.T.);
#5763=ORIENTED_EDGE('',*,*,#4296,.T.);
#5764=ORIENTED_EDGE('',*,*,#4297,.T.);
#5765=ORIENTED_EDGE('',*,*,#4286,.F.);
#5766=ORIENTED_EDGE('',*,*,#4298,.T.);
#5767=ORIENTED_EDGE('',*,*,#4299,.T.);
#5768=ORIENTED_EDGE('',*,*,#4200,.T.);
#5769=ORIENTED_EDGE('',*,*,#4300,.T.);
#5770=ORIENTED_EDGE('',*,*,#4301,.T.);
#5771=ORIENTED_EDGE('',*,*,#4195,.F.);
#5772=ORIENTED_EDGE('',*,*,#4302,.F.);
#5773=ORIENTED_EDGE('',*,*,#4303,.F.);
#5774=ORIENTED_EDGE('',*,*,#4105,.T.);
#5775=ORIENTED_EDGE('',*,*,#4304,.T.);
#5776=ORIENTED_EDGE('',*,*,#4305,.T.);
#5777=ORIENTED_EDGE('',*,*,#4100,.F.);
#5778=ORIENTED_EDGE('',*,*,#4306,.T.);
#5779=ORIENTED_EDGE('',*,*,#4015,.T.);
#5780=ORIENTED_EDGE('',*,*,#4307,.T.);
#5781=ORIENTED_EDGE('',*,*,#4308,.T.);
#5782=ORIENTED_EDGE('',*,*,#4010,.F.);
#5783=ORIENTED_EDGE('',*,*,#4309,.F.);
#5784=ORIENTED_EDGE('',*,*,#4310,.F.);
#5785=ORIENTED_EDGE('',*,*,#4023,.F.);
#5786=ORIENTED_EDGE('',*,*,#4311,.T.);
#5787=ORIENTED_EDGE('',*,*,#3928,.T.);
#5788=ORIENTED_EDGE('',*,*,#4312,.T.);
#5789=ORIENTED_EDGE('',*,*,#4026,.F.);
#5790=ORIENTED_EDGE('',*,*,#4312,.F.);
#5791=ORIENTED_EDGE('',*,*,#3927,.F.);
#5792=ORIENTED_EDGE('',*,*,#3932,.F.);
#5793=ORIENTED_EDGE('',*,*,#3931,.F.);
#5794=ORIENTED_EDGE('',*,*,#3937,.F.);
#5795=ORIENTED_EDGE('',*,*,#3936,.F.);
#5796=ORIENTED_EDGE('',*,*,#3942,.F.);
#5797=ORIENTED_EDGE('',*,*,#3941,.F.);
#5798=ORIENTED_EDGE('',*,*,#3947,.F.);
#5799=ORIENTED_EDGE('',*,*,#3946,.F.);
#5800=ORIENTED_EDGE('',*,*,#3952,.F.);
#5801=ORIENTED_EDGE('',*,*,#3951,.F.);
#5802=ORIENTED_EDGE('',*,*,#3957,.F.);
#5803=ORIENTED_EDGE('',*,*,#3956,.F.);
#5804=ORIENTED_EDGE('',*,*,#3962,.F.);
#5805=ORIENTED_EDGE('',*,*,#3961,.F.);
#5806=ORIENTED_EDGE('',*,*,#3967,.F.);
#5807=ORIENTED_EDGE('',*,*,#3966,.F.);
#5808=ORIENTED_EDGE('',*,*,#3972,.F.);
#5809=ORIENTED_EDGE('',*,*,#3971,.F.);
#5810=ORIENTED_EDGE('',*,*,#3977,.F.);
#5811=ORIENTED_EDGE('',*,*,#3976,.F.);
#5812=ORIENTED_EDGE('',*,*,#3982,.F.);
#5813=ORIENTED_EDGE('',*,*,#3981,.F.);
#5814=ORIENTED_EDGE('',*,*,#3987,.F.);
#5815=ORIENTED_EDGE('',*,*,#3986,.F.);
#5816=ORIENTED_EDGE('',*,*,#3992,.F.);
#5817=ORIENTED_EDGE('',*,*,#3991,.F.);
#5818=ORIENTED_EDGE('',*,*,#3997,.F.);
#5819=ORIENTED_EDGE('',*,*,#3996,.F.);
#5820=ORIENTED_EDGE('',*,*,#4002,.F.);
#5821=ORIENTED_EDGE('',*,*,#4001,.F.);
#5822=ORIENTED_EDGE('',*,*,#4007,.F.);
#5823=ORIENTED_EDGE('',*,*,#4006,.F.);
#5824=ORIENTED_EDGE('',*,*,#4012,.F.);
#5825=ORIENTED_EDGE('',*,*,#4011,.F.);
#5826=ORIENTED_EDGE('',*,*,#4308,.F.);
#5827=ORIENTED_EDGE('',*,*,#4307,.F.);
#5828=ORIENTED_EDGE('',*,*,#4020,.F.);
#5829=ORIENTED_EDGE('',*,*,#4019,.F.);
#5830=ORIENTED_EDGE('',*,*,#4313,.F.);
#5831=ORIENTED_EDGE('',*,*,#4107,.F.);
#5832=ORIENTED_EDGE('',*,*,#4106,.F.);
#5833=ORIENTED_EDGE('',*,*,#4306,.F.);
#5834=ORIENTED_EDGE('',*,*,#4104,.F.);
#5835=ORIENTED_EDGE('',*,*,#4103,.F.);
#5836=ORIENTED_EDGE('',*,*,#4099,.F.);
#5837=ORIENTED_EDGE('',*,*,#4095,.F.);
#5838=ORIENTED_EDGE('',*,*,#4094,.F.);
#5839=ORIENTED_EDGE('',*,*,#4090,.F.);
#5840=ORIENTED_EDGE('',*,*,#4086,.F.);
#5841=ORIENTED_EDGE('',*,*,#4085,.F.);
#5842=ORIENTED_EDGE('',*,*,#4081,.F.);
#5843=ORIENTED_EDGE('',*,*,#4077,.F.);
#5844=ORIENTED_EDGE('',*,*,#4076,.F.);
#5845=ORIENTED_EDGE('',*,*,#4072,.F.);
#5846=ORIENTED_EDGE('',*,*,#4068,.F.);
#5847=ORIENTED_EDGE('',*,*,#4067,.F.);
#5848=ORIENTED_EDGE('',*,*,#4063,.F.);
#5849=ORIENTED_EDGE('',*,*,#4059,.F.);
#5850=ORIENTED_EDGE('',*,*,#4058,.F.);
#5851=ORIENTED_EDGE('',*,*,#4054,.F.);
#5852=ORIENTED_EDGE('',*,*,#4050,.F.);
#5853=ORIENTED_EDGE('',*,*,#4049,.F.);
#5854=ORIENTED_EDGE('',*,*,#4045,.F.);
#5855=ORIENTED_EDGE('',*,*,#4041,.F.);
#5856=ORIENTED_EDGE('',*,*,#4040,.F.);
#5857=ORIENTED_EDGE('',*,*,#4036,.F.);
#5858=ORIENTED_EDGE('',*,*,#4032,.F.);
#5859=ORIENTED_EDGE('',*,*,#4031,.F.);
#5860=ORIENTED_EDGE('',*,*,#4027,.F.);
#5861=ORIENTED_EDGE('',*,*,#4311,.F.);
#5862=ORIENTED_EDGE('',*,*,#4022,.F.);
#5863=ORIENTED_EDGE('',*,*,#4030,.F.);
#5864=ORIENTED_EDGE('',*,*,#4029,.F.);
#5865=ORIENTED_EDGE('',*,*,#4035,.F.);
#5866=ORIENTED_EDGE('',*,*,#4034,.F.);
#5867=ORIENTED_EDGE('',*,*,#4039,.F.);
#5868=ORIENTED_EDGE('',*,*,#4038,.F.);
#5869=ORIENTED_EDGE('',*,*,#4044,.F.);
#5870=ORIENTED_EDGE('',*,*,#4043,.F.);
#5871=ORIENTED_EDGE('',*,*,#4048,.F.);
#5872=ORIENTED_EDGE('',*,*,#4047,.F.);
#5873=ORIENTED_EDGE('',*,*,#4053,.F.);
#5874=ORIENTED_EDGE('',*,*,#4052,.F.);
#5875=ORIENTED_EDGE('',*,*,#4057,.F.);
#5876=ORIENTED_EDGE('',*,*,#4056,.F.);
#5877=ORIENTED_EDGE('',*,*,#4062,.F.);
#5878=ORIENTED_EDGE('',*,*,#4061,.F.);
#5879=ORIENTED_EDGE('',*,*,#4066,.F.);
#5880=ORIENTED_EDGE('',*,*,#4065,.F.);
#5881=ORIENTED_EDGE('',*,*,#4071,.F.);
#5882=ORIENTED_EDGE('',*,*,#4070,.F.);
#5883=ORIENTED_EDGE('',*,*,#4075,.F.);
#5884=ORIENTED_EDGE('',*,*,#4074,.F.);
#5885=ORIENTED_EDGE('',*,*,#4080,.F.);
#5886=ORIENTED_EDGE('',*,*,#4079,.F.);
#5887=ORIENTED_EDGE('',*,*,#4084,.F.);
#5888=ORIENTED_EDGE('',*,*,#4083,.F.);
#5889=ORIENTED_EDGE('',*,*,#4089,.F.);
#5890=ORIENTED_EDGE('',*,*,#4088,.F.);
#5891=ORIENTED_EDGE('',*,*,#4093,.F.);
#5892=ORIENTED_EDGE('',*,*,#4092,.F.);
#5893=ORIENTED_EDGE('',*,*,#4098,.F.);
#5894=ORIENTED_EDGE('',*,*,#4097,.F.);
#5895=ORIENTED_EDGE('',*,*,#4102,.F.);
#5896=ORIENTED_EDGE('',*,*,#4101,.F.);
#5897=ORIENTED_EDGE('',*,*,#4305,.F.);
#5898=ORIENTED_EDGE('',*,*,#4304,.F.);
#5899=ORIENTED_EDGE('',*,*,#4110,.F.);
#5900=ORIENTED_EDGE('',*,*,#4109,.F.);
#5901=ORIENTED_EDGE('',*,*,#4314,.F.);
#5902=ORIENTED_EDGE('',*,*,#4017,.T.);
#5903=ORIENTED_EDGE('',*,*,#4016,.T.);
#5904=ORIENTED_EDGE('',*,*,#4310,.T.);
#5905=ORIENTED_EDGE('',*,*,#4309,.T.);
#5906=ORIENTED_EDGE('',*,*,#4014,.T.);
#5907=ORIENTED_EDGE('',*,*,#4013,.T.);
#5908=ORIENTED_EDGE('',*,*,#4009,.T.);
#5909=ORIENTED_EDGE('',*,*,#4008,.T.);
#5910=ORIENTED_EDGE('',*,*,#4004,.T.);
#5911=ORIENTED_EDGE('',*,*,#4003,.T.);
#5912=ORIENTED_EDGE('',*,*,#3999,.T.);
#5913=ORIENTED_EDGE('',*,*,#3998,.T.);
#5914=ORIENTED_EDGE('',*,*,#3994,.T.);
#5915=ORIENTED_EDGE('',*,*,#3993,.T.);
#5916=ORIENTED_EDGE('',*,*,#3989,.T.);
#5917=ORIENTED_EDGE('',*,*,#3988,.T.);
#5918=ORIENTED_EDGE('',*,*,#3984,.T.);
#5919=ORIENTED_EDGE('',*,*,#3983,.T.);
#5920=ORIENTED_EDGE('',*,*,#3979,.T.);
#5921=ORIENTED_EDGE('',*,*,#3978,.T.);
#5922=ORIENTED_EDGE('',*,*,#3974,.T.);
#5923=ORIENTED_EDGE('',*,*,#3973,.T.);
#5924=ORIENTED_EDGE('',*,*,#3969,.T.);
#5925=ORIENTED_EDGE('',*,*,#3968,.T.);
#5926=ORIENTED_EDGE('',*,*,#3964,.T.);
#5927=ORIENTED_EDGE('',*,*,#3963,.T.);
#5928=ORIENTED_EDGE('',*,*,#3959,.T.);
#5929=ORIENTED_EDGE('',*,*,#3958,.T.);
#5930=ORIENTED_EDGE('',*,*,#3954,.T.);
#5931=ORIENTED_EDGE('',*,*,#3953,.T.);
#5932=ORIENTED_EDGE('',*,*,#3949,.T.);
#5933=ORIENTED_EDGE('',*,*,#3948,.T.);
#5934=ORIENTED_EDGE('',*,*,#3944,.T.);
#5935=ORIENTED_EDGE('',*,*,#3943,.T.);
#5936=ORIENTED_EDGE('',*,*,#3939,.T.);
#5937=ORIENTED_EDGE('',*,*,#3938,.T.);
#5938=ORIENTED_EDGE('',*,*,#3934,.T.);
#5939=ORIENTED_EDGE('',*,*,#3933,.T.);
#5940=ORIENTED_EDGE('',*,*,#3929,.T.);
#5941=ORIENTED_EDGE('',*,*,#4025,.F.);
#5942=ORIENTED_EDGE('',*,*,#4208,.F.);
#5943=ORIENTED_EDGE('',*,*,#4315,.T.);
#5944=ORIENTED_EDGE('',*,*,#4113,.T.);
#5945=ORIENTED_EDGE('',*,*,#4316,.T.);
#5946=ORIENTED_EDGE('',*,*,#4211,.F.);
#5947=ORIENTED_EDGE('',*,*,#4316,.F.);
#5948=ORIENTED_EDGE('',*,*,#4112,.F.);
#5949=ORIENTED_EDGE('',*,*,#4117,.F.);
#5950=ORIENTED_EDGE('',*,*,#4116,.F.);
#5951=ORIENTED_EDGE('',*,*,#4122,.F.);
#5952=ORIENTED_EDGE('',*,*,#4121,.F.);
#5953=ORIENTED_EDGE('',*,*,#4127,.F.);
#5954=ORIENTED_EDGE('',*,*,#4126,.F.);
#5955=ORIENTED_EDGE('',*,*,#4132,.F.);
#5956=ORIENTED_EDGE('',*,*,#4131,.F.);
#5957=ORIENTED_EDGE('',*,*,#4137,.F.);
#5958=ORIENTED_EDGE('',*,*,#4136,.F.);
#5959=ORIENTED_EDGE('',*,*,#4142,.F.);
#5960=ORIENTED_EDGE('',*,*,#4141,.F.);
#5961=ORIENTED_EDGE('',*,*,#4147,.F.);
#5962=ORIENTED_EDGE('',*,*,#4146,.F.);
#5963=ORIENTED_EDGE('',*,*,#4152,.F.);
#5964=ORIENTED_EDGE('',*,*,#4151,.F.);
#5965=ORIENTED_EDGE('',*,*,#4157,.F.);
#5966=ORIENTED_EDGE('',*,*,#4156,.F.);
#5967=ORIENTED_EDGE('',*,*,#4162,.F.);
#5968=ORIENTED_EDGE('',*,*,#4161,.F.);
#5969=ORIENTED_EDGE('',*,*,#4167,.F.);
#5970=ORIENTED_EDGE('',*,*,#4166,.F.);
#5971=ORIENTED_EDGE('',*,*,#4172,.F.);
#5972=ORIENTED_EDGE('',*,*,#4171,.F.);
#5973=ORIENTED_EDGE('',*,*,#4177,.F.);
#5974=ORIENTED_EDGE('',*,*,#4176,.F.);
#5975=ORIENTED_EDGE('',*,*,#4182,.F.);
#5976=ORIENTED_EDGE('',*,*,#4181,.F.);
#5977=ORIENTED_EDGE('',*,*,#4187,.F.);
#5978=ORIENTED_EDGE('',*,*,#4186,.F.);
#5979=ORIENTED_EDGE('',*,*,#4192,.F.);
#5980=ORIENTED_EDGE('',*,*,#4191,.F.);
#5981=ORIENTED_EDGE('',*,*,#4197,.F.);
#5982=ORIENTED_EDGE('',*,*,#4196,.F.);
#5983=ORIENTED_EDGE('',*,*,#4301,.F.);
#5984=ORIENTED_EDGE('',*,*,#4300,.F.);
#5985=ORIENTED_EDGE('',*,*,#4205,.F.);
#5986=ORIENTED_EDGE('',*,*,#4204,.F.);
#5987=ORIENTED_EDGE('',*,*,#4317,.F.);
#5988=ORIENTED_EDGE('',*,*,#4292,.F.);
#5989=ORIENTED_EDGE('',*,*,#4291,.F.);
#5990=ORIENTED_EDGE('',*,*,#4299,.F.);
#5991=ORIENTED_EDGE('',*,*,#4298,.F.);
#5992=ORIENTED_EDGE('',*,*,#4289,.F.);
#5993=ORIENTED_EDGE('',*,*,#4285,.F.);
#5994=ORIENTED_EDGE('',*,*,#4284,.F.);
#5995=ORIENTED_EDGE('',*,*,#4280,.F.);
#5996=ORIENTED_EDGE('',*,*,#4276,.F.);
#5997=ORIENTED_EDGE('',*,*,#4275,.F.);
#5998=ORIENTED_EDGE('',*,*,#4271,.F.);
#5999=ORIENTED_EDGE('',*,*,#4267,.F.);
#6000=ORIENTED_EDGE('',*,*,#4266,.F.);
#6001=ORIENTED_EDGE('',*,*,#4262,.F.);
#6002=ORIENTED_EDGE('',*,*,#4258,.F.);
#6003=ORIENTED_EDGE('',*,*,#4257,.F.);
#6004=ORIENTED_EDGE('',*,*,#4253,.F.);
#6005=ORIENTED_EDGE('',*,*,#4249,.F.);
#6006=ORIENTED_EDGE('',*,*,#4248,.F.);
#6007=ORIENTED_EDGE('',*,*,#4244,.F.);
#6008=ORIENTED_EDGE('',*,*,#4240,.F.);
#6009=ORIENTED_EDGE('',*,*,#4239,.F.);
#6010=ORIENTED_EDGE('',*,*,#4235,.F.);
#6011=ORIENTED_EDGE('',*,*,#4231,.F.);
#6012=ORIENTED_EDGE('',*,*,#4230,.F.);
#6013=ORIENTED_EDGE('',*,*,#4226,.F.);
#6014=ORIENTED_EDGE('',*,*,#4222,.F.);
#6015=ORIENTED_EDGE('',*,*,#4221,.F.);
#6016=ORIENTED_EDGE('',*,*,#4217,.F.);
#6017=ORIENTED_EDGE('',*,*,#4216,.F.);
#6018=ORIENTED_EDGE('',*,*,#4212,.F.);
#6019=ORIENTED_EDGE('',*,*,#4315,.F.);
#6020=ORIENTED_EDGE('',*,*,#4207,.F.);
#6021=ORIENTED_EDGE('',*,*,#4215,.F.);
#6022=ORIENTED_EDGE('',*,*,#4214,.F.);
#6023=ORIENTED_EDGE('',*,*,#4220,.F.);
#6024=ORIENTED_EDGE('',*,*,#4219,.F.);
#6025=ORIENTED_EDGE('',*,*,#4225,.F.);
#6026=ORIENTED_EDGE('',*,*,#4224,.F.);
#6027=ORIENTED_EDGE('',*,*,#4229,.F.);
#6028=ORIENTED_EDGE('',*,*,#4228,.F.);
#6029=ORIENTED_EDGE('',*,*,#4234,.F.);
#6030=ORIENTED_EDGE('',*,*,#4233,.F.);
#6031=ORIENTED_EDGE('',*,*,#4238,.F.);
#6032=ORIENTED_EDGE('',*,*,#4237,.F.);
#6033=ORIENTED_EDGE('',*,*,#4243,.F.);
#6034=ORIENTED_EDGE('',*,*,#4242,.F.);
#6035=ORIENTED_EDGE('',*,*,#4247,.F.);
#6036=ORIENTED_EDGE('',*,*,#4246,.F.);
#6037=ORIENTED_EDGE('',*,*,#4252,.F.);
#6038=ORIENTED_EDGE('',*,*,#4251,.F.);
#6039=ORIENTED_EDGE('',*,*,#4256,.F.);
#6040=ORIENTED_EDGE('',*,*,#4255,.F.);
#6041=ORIENTED_EDGE('',*,*,#4261,.F.);
#6042=ORIENTED_EDGE('',*,*,#4260,.F.);
#6043=ORIENTED_EDGE('',*,*,#4265,.F.);
#6044=ORIENTED_EDGE('',*,*,#4264,.F.);
#6045=ORIENTED_EDGE('',*,*,#4270,.F.);
#6046=ORIENTED_EDGE('',*,*,#4269,.F.);
#6047=ORIENTED_EDGE('',*,*,#4274,.F.);
#6048=ORIENTED_EDGE('',*,*,#4273,.F.);
#6049=ORIENTED_EDGE('',*,*,#4279,.F.);
#6050=ORIENTED_EDGE('',*,*,#4278,.F.);
#6051=ORIENTED_EDGE('',*,*,#4283,.F.);
#6052=ORIENTED_EDGE('',*,*,#4282,.F.);
#6053=ORIENTED_EDGE('',*,*,#4288,.F.);
#6054=ORIENTED_EDGE('',*,*,#4287,.F.);
#6055=ORIENTED_EDGE('',*,*,#4297,.F.);
#6056=ORIENTED_EDGE('',*,*,#4296,.F.);
#6057=ORIENTED_EDGE('',*,*,#4295,.F.);
#6058=ORIENTED_EDGE('',*,*,#4294,.F.);
#6059=ORIENTED_EDGE('',*,*,#4318,.F.);
#6060=ORIENTED_EDGE('',*,*,#4202,.T.);
#6061=ORIENTED_EDGE('',*,*,#4201,.T.);
#6062=ORIENTED_EDGE('',*,*,#4303,.T.);
#6063=ORIENTED_EDGE('',*,*,#4302,.T.);
#6064=ORIENTED_EDGE('',*,*,#4199,.T.);
#6065=ORIENTED_EDGE('',*,*,#4198,.T.);
#6066=ORIENTED_EDGE('',*,*,#4194,.T.);
#6067=ORIENTED_EDGE('',*,*,#4193,.T.);
#6068=ORIENTED_EDGE('',*,*,#4189,.T.);
#6069=ORIENTED_EDGE('',*,*,#4188,.T.);
#6070=ORIENTED_EDGE('',*,*,#4184,.T.);
#6071=ORIENTED_EDGE('',*,*,#4183,.T.);
#6072=ORIENTED_EDGE('',*,*,#4179,.T.);
#6073=ORIENTED_EDGE('',*,*,#4178,.T.);
#6074=ORIENTED_EDGE('',*,*,#4174,.T.);
#6075=ORIENTED_EDGE('',*,*,#4173,.T.);
#6076=ORIENTED_EDGE('',*,*,#4169,.T.);
#6077=ORIENTED_EDGE('',*,*,#4168,.T.);
#6078=ORIENTED_EDGE('',*,*,#4164,.T.);
#6079=ORIENTED_EDGE('',*,*,#4163,.T.);
#6080=ORIENTED_EDGE('',*,*,#4159,.T.);
#6081=ORIENTED_EDGE('',*,*,#4158,.T.);
#6082=ORIENTED_EDGE('',*,*,#4154,.T.);
#6083=ORIENTED_EDGE('',*,*,#4153,.T.);
#6084=ORIENTED_EDGE('',*,*,#4149,.T.);
#6085=ORIENTED_EDGE('',*,*,#4148,.T.);
#6086=ORIENTED_EDGE('',*,*,#4144,.T.);
#6087=ORIENTED_EDGE('',*,*,#4143,.T.);
#6088=ORIENTED_EDGE('',*,*,#4139,.T.);
#6089=ORIENTED_EDGE('',*,*,#4138,.T.);
#6090=ORIENTED_EDGE('',*,*,#4134,.T.);
#6091=ORIENTED_EDGE('',*,*,#4133,.T.);
#6092=ORIENTED_EDGE('',*,*,#4129,.T.);
#6093=ORIENTED_EDGE('',*,*,#4128,.T.);
#6094=ORIENTED_EDGE('',*,*,#4124,.T.);
#6095=ORIENTED_EDGE('',*,*,#4123,.T.);
#6096=ORIENTED_EDGE('',*,*,#4119,.T.);
#6097=ORIENTED_EDGE('',*,*,#4118,.T.);
#6098=ORIENTED_EDGE('',*,*,#4114,.T.);
#6099=ORIENTED_EDGE('',*,*,#4210,.F.);
#6100=ORIENTED_EDGE('',*,*,#4319,.F.);
#6101=ORIENTED_EDGE('',*,*,#4320,.T.);
#6102=ORIENTED_EDGE('',*,*,#4321,.T.);
#6103=ORIENTED_EDGE('',*,*,#4320,.F.);
#6104=ORIENTED_EDGE('',*,*,#4319,.T.);
#6105=ORIENTED_EDGE('',*,*,#4318,.T.);
#6106=ORIENTED_EDGE('',*,*,#4293,.T.);
#6107=ORIENTED_EDGE('',*,*,#4317,.T.);
#6108=ORIENTED_EDGE('',*,*,#4203,.T.);
#6109=ORIENTED_EDGE('',*,*,#4321,.F.);
#6110=ORIENTED_EDGE('',*,*,#4314,.T.);
#6111=ORIENTED_EDGE('',*,*,#4108,.T.);
#6112=ORIENTED_EDGE('',*,*,#4313,.T.);
#6113=ORIENTED_EDGE('',*,*,#4018,.T.);
#7672=CYLINDRICAL_SURFACE('',#8513,3.0735);
#7673=CYLINDRICAL_SURFACE('',#8515,3.0735);
#7674=CYLINDRICAL_SURFACE('',#8516,3.0735);
#7675=CYLINDRICAL_SURFACE('',#8517,3.0735);
#7676=CYLINDRICAL_SURFACE('',#8518,3.0735);
#7677=CYLINDRICAL_SURFACE('',#8519,3.0735);
#7678=CYLINDRICAL_SURFACE('',#8520,3.0735);
#7679=CYLINDRICAL_SURFACE('',#8521,3.0735);
#7680=CYLINDRICAL_SURFACE('',#8522,3.0735);
#7681=CYLINDRICAL_SURFACE('',#8523,3.0735);
#7682=CYLINDRICAL_SURFACE('',#8524,3.0735);
#7683=CYLINDRICAL_SURFACE('',#8525,3.0735);
#7684=CYLINDRICAL_SURFACE('',#8526,3.0735);
#7685=CYLINDRICAL_SURFACE('',#8527,3.0735);
#7686=CYLINDRICAL_SURFACE('',#8528,3.0735);
#7687=CYLINDRICAL_SURFACE('',#8529,3.0735);
#7688=CYLINDRICAL_SURFACE('',#8530,3.0735);
#7689=CYLINDRICAL_SURFACE('',#8531,3.0735);
#7690=CYLINDRICAL_SURFACE('',#8532,3.0735);
#7691=CYLINDRICAL_SURFACE('',#8534,2.5175);
#7692=CYLINDRICAL_SURFACE('',#8538,2.5175);
#7693=CYLINDRICAL_SURFACE('',#8539,2.5175);
#7694=CYLINDRICAL_SURFACE('',#8540,2.5175);
#7695=CYLINDRICAL_SURFACE('',#8541,2.5175);
#7696=CYLINDRICAL_SURFACE('',#8542,2.5175);
#7697=CYLINDRICAL_SURFACE('',#8543,2.5175);
#7698=CYLINDRICAL_SURFACE('',#8544,2.5175);
#7699=CYLINDRICAL_SURFACE('',#8545,2.5175);
#7700=CYLINDRICAL_SURFACE('',#8546,2.5175);
#7701=CYLINDRICAL_SURFACE('',#8547,2.5175);
#7702=CYLINDRICAL_SURFACE('',#8548,2.5175);
#7703=CYLINDRICAL_SURFACE('',#8549,2.5175);
#7704=CYLINDRICAL_SURFACE('',#8550,2.5175);
#7705=CYLINDRICAL_SURFACE('',#8551,2.5175);
#7706=CYLINDRICAL_SURFACE('',#8552,2.5175);
#7707=CYLINDRICAL_SURFACE('',#8553,2.5175);
#7708=CYLINDRICAL_SURFACE('',#8554,2.5175);
#7709=CYLINDRICAL_SURFACE('',#8555,2.5175);
#7710=CYLINDRICAL_SURFACE('',#8557,3.0735);
#7711=CYLINDRICAL_SURFACE('',#8559,3.0735);
#7712=CYLINDRICAL_SURFACE('',#8560,3.0735);
#7713=CYLINDRICAL_SURFACE('',#8561,3.0735);
#7714=CYLINDRICAL_SURFACE('',#8562,3.0735);
#7715=CYLINDRICAL_SURFACE('',#8563,3.0735);
#7716=CYLINDRICAL_SURFACE('',#8564,3.0735);
#7717=CYLINDRICAL_SURFACE('',#8565,3.0735);
#7718=CYLINDRICAL_SURFACE('',#8566,3.0735);
#7719=CYLINDRICAL_SURFACE('',#8567,3.0735);
#7720=CYLINDRICAL_SURFACE('',#8568,3.0735);
#7721=CYLINDRICAL_SURFACE('',#8569,3.0735);
#7722=CYLINDRICAL_SURFACE('',#8570,3.0735);
#7723=CYLINDRICAL_SURFACE('',#8571,3.0735);
#7724=CYLINDRICAL_SURFACE('',#8572,3.0735);
#7725=CYLINDRICAL_SURFACE('',#8573,3.0735);
#7726=CYLINDRICAL_SURFACE('',#8574,3.0735);
#7727=CYLINDRICAL_SURFACE('',#8575,3.0735);
#7728=CYLINDRICAL_SURFACE('',#8576,3.0735);
#7729=CYLINDRICAL_SURFACE('',#8578,2.5175);
#7730=CYLINDRICAL_SURFACE('',#8582,2.5175);
#7731=CYLINDRICAL_SURFACE('',#8583,2.5175);
#7732=CYLINDRICAL_SURFACE('',#8584,2.5175);
#7733=CYLINDRICAL_SURFACE('',#8585,2.5175);
#7734=CYLINDRICAL_SURFACE('',#8586,2.5175);
#7735=CYLINDRICAL_SURFACE('',#8587,2.5175);
#7736=CYLINDRICAL_SURFACE('',#8588,2.5175);
#7737=CYLINDRICAL_SURFACE('',#8589,2.5175);
#7738=CYLINDRICAL_SURFACE('',#8590,2.5175);
#7739=CYLINDRICAL_SURFACE('',#8591,2.5175);
#7740=CYLINDRICAL_SURFACE('',#8592,2.5175);
#7741=CYLINDRICAL_SURFACE('',#8593,2.5175);
#7742=CYLINDRICAL_SURFACE('',#8594,2.5175);
#7743=CYLINDRICAL_SURFACE('',#8595,2.5175);
#7744=CYLINDRICAL_SURFACE('',#8596,2.5175);
#7745=CYLINDRICAL_SURFACE('',#8597,2.5175);
#7746=CYLINDRICAL_SURFACE('',#8598,2.5175);
#7747=CYLINDRICAL_SURFACE('',#8599,2.5175);
#7748=CYLINDRICAL_SURFACE('',#8601,2.5175);
#7749=CYLINDRICAL_SURFACE('',#8602,3.0735);
#7750=CYLINDRICAL_SURFACE('',#8603,2.5175);
#7751=CYLINDRICAL_SURFACE('',#8604,3.0735);
#7752=CYLINDRICAL_SURFACE('',#8609,8.);
#7941=ADVANCED_FACE('',(#1204),#7672,.F.);
#7942=ADVANCED_FACE('',(#1205),#7673,.F.);
#7943=ADVANCED_FACE('',(#1206),#7674,.F.);
#7944=ADVANCED_FACE('',(#1207),#7675,.F.);
#7945=ADVANCED_FACE('',(#1208),#7676,.F.);
#7946=ADVANCED_FACE('',(#1209),#7677,.F.);
#7947=ADVANCED_FACE('',(#1210),#7678,.F.);
#7948=ADVANCED_FACE('',(#1211),#7679,.F.);
#7949=ADVANCED_FACE('',(#1212),#7680,.F.);
#7950=ADVANCED_FACE('',(#1213),#7681,.F.);
#7951=ADVANCED_FACE('',(#1214),#7682,.F.);
#7952=ADVANCED_FACE('',(#1215),#7683,.F.);
#7953=ADVANCED_FACE('',(#1216),#7684,.F.);
#7954=ADVANCED_FACE('',(#1217),#7685,.F.);
#7955=ADVANCED_FACE('',(#1218),#7686,.F.);
#7956=ADVANCED_FACE('',(#1219),#7687,.F.);
#7957=ADVANCED_FACE('',(#1220),#7688,.F.);
#7958=ADVANCED_FACE('',(#1221),#7689,.F.);
#7959=ADVANCED_FACE('',(#1222),#7690,.F.);
#7960=ADVANCED_FACE('',(#1223),#7691,.F.);
#7961=ADVANCED_FACE('',(#1224),#7692,.F.);
#7962=ADVANCED_FACE('',(#1225),#7693,.F.);
#7963=ADVANCED_FACE('',(#1226),#7694,.F.);
#7964=ADVANCED_FACE('',(#1227),#7695,.F.);
#7965=ADVANCED_FACE('',(#1228),#7696,.F.);
#7966=ADVANCED_FACE('',(#1229),#7697,.F.);
#7967=ADVANCED_FACE('',(#1230),#7698,.F.);
#7968=ADVANCED_FACE('',(#1231),#7699,.F.);
#7969=ADVANCED_FACE('',(#1232),#7700,.F.);
#7970=ADVANCED_FACE('',(#1233),#7701,.F.);
#7971=ADVANCED_FACE('',(#1234),#7702,.F.);
#7972=ADVANCED_FACE('',(#1235),#7703,.F.);
#7973=ADVANCED_FACE('',(#1236),#7704,.F.);
#7974=ADVANCED_FACE('',(#1237),#7705,.F.);
#7975=ADVANCED_FACE('',(#1238),#7706,.F.);
#7976=ADVANCED_FACE('',(#1239),#7707,.F.);
#7977=ADVANCED_FACE('',(#1240),#7708,.F.);
#7978=ADVANCED_FACE('',(#1241),#7709,.F.);
#7979=ADVANCED_FACE('',(#1242),#7710,.F.);
#7980=ADVANCED_FACE('',(#1243),#7711,.F.);
#7981=ADVANCED_FACE('',(#1244),#7712,.F.);
#7982=ADVANCED_FACE('',(#1245),#7713,.F.);
#7983=ADVANCED_FACE('',(#1246),#7714,.F.);
#7984=ADVANCED_FACE('',(#1247),#7715,.F.);
#7985=ADVANCED_FACE('',(#1248),#7716,.F.);
#7986=ADVANCED_FACE('',(#1249),#7717,.F.);
#7987=ADVANCED_FACE('',(#1250),#7718,.F.);
#7988=ADVANCED_FACE('',(#1251),#7719,.F.);
#7989=ADVANCED_FACE('',(#1252),#7720,.F.);
#7990=ADVANCED_FACE('',(#1253),#7721,.F.);
#7991=ADVANCED_FACE('',(#1254),#7722,.F.);
#7992=ADVANCED_FACE('',(#1255),#7723,.F.);
#7993=ADVANCED_FACE('',(#1256),#7724,.F.);
#7994=ADVANCED_FACE('',(#1257),#7725,.F.);
#7995=ADVANCED_FACE('',(#1258),#7726,.F.);
#7996=ADVANCED_FACE('',(#1259),#7727,.F.);
#7997=ADVANCED_FACE('',(#1260),#7728,.F.);
#7998=ADVANCED_FACE('',(#1261),#7729,.F.);
#7999=ADVANCED_FACE('',(#1262),#7730,.F.);
#8000=ADVANCED_FACE('',(#1263),#7731,.F.);
#8001=ADVANCED_FACE('',(#1264),#7732,.F.);
#8002=ADVANCED_FACE('',(#1265),#7733,.F.);
#8003=ADVANCED_FACE('',(#1266),#7734,.F.);
#8004=ADVANCED_FACE('',(#1267),#7735,.F.);
#8005=ADVANCED_FACE('',(#1268),#7736,.F.);
#8006=ADVANCED_FACE('',(#1269),#7737,.F.);
#8007=ADVANCED_FACE('',(#1270),#7738,.F.);
#8008=ADVANCED_FACE('',(#1271),#7739,.F.);
#8009=ADVANCED_FACE('',(#1272),#7740,.F.);
#8010=ADVANCED_FACE('',(#1273),#7741,.F.);
#8011=ADVANCED_FACE('',(#1274),#7742,.F.);
#8012=ADVANCED_FACE('',(#1275),#7743,.F.);
#8013=ADVANCED_FACE('',(#1276),#7744,.F.);
#8014=ADVANCED_FACE('',(#1277),#7745,.F.);
#8015=ADVANCED_FACE('',(#1278),#7746,.F.);
#8016=ADVANCED_FACE('',(#1279),#7747,.F.);
#8017=ADVANCED_FACE('',(#1280),#7748,.F.);
#8018=ADVANCED_FACE('',(#1281),#7749,.F.);
#8019=ADVANCED_FACE('',(#1282),#7750,.F.);
#8020=ADVANCED_FACE('',(#1283),#7751,.F.);
#8021=ADVANCED_FACE('',(#1284),#1090,.F.);
#8022=ADVANCED_FACE('',(#1285),#154,.F.);
#8023=ADVANCED_FACE('',(#1286),#155,.F.);
#8024=ADVANCED_FACE('',(#1287),#1091,.F.);
#8025=ADVANCED_FACE('',(#1288),#1092,.T.);
#8026=ADVANCED_FACE('',(#1289),#156,.F.);
#8027=ADVANCED_FACE('',(#1290),#157,.F.);
#8028=ADVANCED_FACE('',(#1291),#1093,.F.);
#8029=ADVANCED_FACE('',(#1292),#7752,.T.);
#8030=ADVANCED_FACE('',(#1293,#1012),#1094,.T.);
#8031=ADVANCED_FACE('',(#1294,#1013),#1095,.F.);
#8255=CLOSED_SHELL('',(#7941,#7942,#7943,#7944,#7945,#7946,#7947,#7948,
#7949,#7950,#7951,#7952,#7953,#7954,#7955,#7956,#7957,#7958,#7959,#7960,
#7961,#7962,#7963,#7964,#7965,#7966,#7967,#7968,#7969,#7970,#7971,#7972,
#7973,#7974,#7975,#7976,#7977,#7978,#7979,#7980,#7981,#7982,#7983,#7984,
#7985,#7986,#7987,#7988,#7989,#7990,#7991,#7992,#7993,#7994,#7995,#7996,
#7997,#7998,#7999,#8000,#8001,#8002,#8003,#8004,#8005,#8006,#8007,#8008,
#8009,#8010,#8011,#8012,#8013,#8014,#8015,#8016,#8017,#8018,#8019,#8020,
#8021,#8022,#8023,#8024,#8025,#8026,#8027,#8028,#8029,#8030,#8031));
#8512=AXIS2_PLACEMENT_3D('',#10602,#9188,#9189);
#8513=AXIS2_PLACEMENT_3D('',#10603,#9190,#9191);
#8514=AXIS2_PLACEMENT_3D('',#10685,#9193,#9194);
#8515=AXIS2_PLACEMENT_3D('',#10780,#9195,#9196);
#8516=AXIS2_PLACEMENT_3D('',#11082,#9198,#9199);
#8517=AXIS2_PLACEMENT_3D('',#11311,#9201,#9202);
#8518=AXIS2_PLACEMENT_3D('',#11543,#9204,#9205);
#8519=AXIS2_PLACEMENT_3D('',#11773,#9207,#9208);
#8520=AXIS2_PLACEMENT_3D('',#12005,#9210,#9211);
#8521=AXIS2_PLACEMENT_3D('',#12240,#9213,#9214);
#8522=AXIS2_PLACEMENT_3D('',#12472,#9216,#9217);
#8523=AXIS2_PLACEMENT_3D('',#12702,#9219,#9220);
#8524=AXIS2_PLACEMENT_3D('',#12807,#9222,#9223);
#8525=AXIS2_PLACEMENT_3D('',#12841,#9225,#9226);
#8526=AXIS2_PLACEMENT_3D('',#13004,#9228,#9229);
#8527=AXIS2_PLACEMENT_3D('',#13234,#9231,#9232);
#8528=AXIS2_PLACEMENT_3D('',#13466,#9234,#9235);
#8529=AXIS2_PLACEMENT_3D('',#13698,#9237,#9238);
#8530=AXIS2_PLACEMENT_3D('',#13927,#9240,#9241);
#8531=AXIS2_PLACEMENT_3D('',#14160,#9243,#9244);
#8532=AXIS2_PLACEMENT_3D('',#14392,#9246,#9247);
#8533=AXIS2_PLACEMENT_3D('',#14480,#9249,#9250);
#8534=AXIS2_PLACEMENT_3D('',#14553,#9251,#9252);
#8535=AXIS2_PLACEMENT_3D('',#14571,#9254,#9255);
#8536=AXIS2_PLACEMENT_3D('',#14574,#9257,#9258);
#8537=AXIS2_PLACEMENT_3D('',#14576,#9259,#9260);
#8538=AXIS2_PLACEMENT_3D('',#14644,#9261,#9262);
#8539=AXIS2_PLACEMENT_3D('',#15067,#9264,#9265);
#8540=AXIS2_PLACEMENT_3D('',#15535,#9267,#9268);
#8541=AXIS2_PLACEMENT_3D('',#15955,#9270,#9271);
#8542=AXIS2_PLACEMENT_3D('',#16356,#9273,#9274);
#8543=AXIS2_PLACEMENT_3D('',#16773,#9276,#9277);
#8544=AXIS2_PLACEMENT_3D('',#17205,#9279,#9280);
#8545=AXIS2_PLACEMENT_3D('',#17657,#9282,#9283);
#8546=AXIS2_PLACEMENT_3D('',#18120,#9285,#9286);
#8547=AXIS2_PLACEMENT_3D('',#18530,#9288,#9289);
#8548=AXIS2_PLACEMENT_3D('',#18963,#9291,#9292);
#8549=AXIS2_PLACEMENT_3D('',#19389,#9294,#9295);
#8550=AXIS2_PLACEMENT_3D('',#19801,#9297,#9298);
#8551=AXIS2_PLACEMENT_3D('',#20231,#9300,#9301);
#8552=AXIS2_PLACEMENT_3D('',#20712,#9303,#9304);
#8553=AXIS2_PLACEMENT_3D('',#21126,#9306,#9307);
#8554=AXIS2_PLACEMENT_3D('',#21557,#9309,#9310);
#8555=AXIS2_PLACEMENT_3D('',#21972,#9312,#9313);
#8556=AXIS2_PLACEMENT_3D('',#22122,#9315,#9316);
#8557=AXIS2_PLACEMENT_3D('',#22309,#9317,#9318);
#8558=AXIS2_PLACEMENT_3D('',#22321,#9320,#9321);
#8559=AXIS2_PLACEMENT_3D('',#22416,#9322,#9323);
#8560=AXIS2_PLACEMENT_3D('',#22651,#9325,#9326);
#8561=AXIS2_PLACEMENT_3D('',#23008,#9328,#9329);
#8562=AXIS2_PLACEMENT_3D('',#23438,#9331,#9332);
#8563=AXIS2_PLACEMENT_3D('',#23868,#9334,#9335);
#8564=AXIS2_PLACEMENT_3D('',#24295,#9337,#9338);
#8565=AXIS2_PLACEMENT_3D('',#24725,#9340,#9341);
#8566=AXIS2_PLACEMENT_3D('',#25155,#9343,#9344);
#8567=AXIS2_PLACEMENT_3D('',#25585,#9346,#9347);
#8568=AXIS2_PLACEMENT_3D('',#26018,#9349,#9350);
#8569=AXIS2_PLACEMENT_3D('',#26442,#9352,#9353);
#8570=AXIS2_PLACEMENT_3D('',#26872,#9355,#9356);
#8571=AXIS2_PLACEMENT_3D('',#27302,#9358,#9359);
#8572=AXIS2_PLACEMENT_3D('',#27729,#9361,#9362);
#8573=AXIS2_PLACEMENT_3D('',#28159,#9364,#9365);
#8574=AXIS2_PLACEMENT_3D('',#28583,#9367,#9368);
#8575=AXIS2_PLACEMENT_3D('',#29013,#9370,#9371);
#8576=AXIS2_PLACEMENT_3D('',#29312,#9373,#9374);
#8577=AXIS2_PLACEMENT_3D('',#29400,#9376,#9377);
#8578=AXIS2_PLACEMENT_3D('',#29473,#9378,#9379);
#8579=AXIS2_PLACEMENT_3D('',#29491,#9381,#9382);
#8580=AXIS2_PLACEMENT_3D('',#29494,#9384,#9385);
#8581=AXIS2_PLACEMENT_3D('',#29496,#9386,#9387);
#8582=AXIS2_PLACEMENT_3D('',#29564,#9388,#9389);
#8583=AXIS2_PLACEMENT_3D('',#29797,#9391,#9392);
#8584=AXIS2_PLACEMENT_3D('',#30200,#9394,#9395);
#8585=AXIS2_PLACEMENT_3D('',#30625,#9397,#9398);
#8586=AXIS2_PLACEMENT_3D('',#31043,#9400,#9401);
#8587=AXIS2_PLACEMENT_3D('',#31469,#9403,#9404);
#8588=AXIS2_PLACEMENT_3D('',#31910,#9406,#9407);
#8589=AXIS2_PLACEMENT_3D('',#32343,#9409,#9410);
#8590=AXIS2_PLACEMENT_3D('',#32771,#9412,#9413);
#8591=AXIS2_PLACEMENT_3D('',#33192,#9415,#9416);
#8592=AXIS2_PLACEMENT_3D('',#33662,#9418,#9419);
#8593=AXIS2_PLACEMENT_3D('',#34145,#9421,#9422);
#8594=AXIS2_PLACEMENT_3D('',#34558,#9424,#9425);
#8595=AXIS2_PLACEMENT_3D('',#34977,#9427,#9428);
#8596=AXIS2_PLACEMENT_3D('',#35415,#9430,#9431);
#8597=AXIS2_PLACEMENT_3D('',#35828,#9433,#9434);
#8598=AXIS2_PLACEMENT_3D('',#36240,#9436,#9437);
#8599=AXIS2_PLACEMENT_3D('',#36646,#9439,#9440);
#8600=AXIS2_PLACEMENT_3D('',#36787,#9442,#9443);
#8601=AXIS2_PLACEMENT_3D('',#36974,#9444,#9445);
#8602=AXIS2_PLACEMENT_3D('',#37371,#9446,#9447);
#8603=AXIS2_PLACEMENT_3D('',#37600,#9448,#9449);
#8604=AXIS2_PLACEMENT_3D('',#38015,#9450,#9451);
#8605=AXIS2_PLACEMENT_3D('',#38244,#9452,#9453);
#8606=AXIS2_PLACEMENT_3D('',#39606,#9454,#9455);
#8607=AXIS2_PLACEMENT_3D('',#39607,#9456,#9457);
#8608=AXIS2_PLACEMENT_3D('',#40972,#9458,#9459);
#8609=AXIS2_PLACEMENT_3D('',#40973,#9460,#9461);
#8610=AXIS2_PLACEMENT_3D('',#40975,#9462,#9463);
#8611=AXIS2_PLACEMENT_3D('',#40978,#9465,#9466);
#8612=AXIS2_PLACEMENT_3D('',#40979,#9467,#9468);
#8613=AXIS2_PLACEMENT_3D('',#40980,#9469,#9470);
#9188=DIRECTION('axis',(0.,0.,1.));
#9189=DIRECTION('refdir',(1.,0.,0.));
#9190=DIRECTION('center_axis',(0.,0.,1.));
#9191=DIRECTION('ref_axis',(0.60921024449365,-0.793008750269496,0.));
#9192=DIRECTION('',(0.,0.,1.));
#9193=DIRECTION('center_axis',(0.,0.,-1.));
#9194=DIRECTION('ref_axis',(-1.,-8.91852360097567E-14,0.));
#9195=DIRECTION('center_axis',(0.,0.,1.));
#9196=DIRECTION('ref_axis',(0.60921024449365,-0.793008750269496,0.));
#9197=DIRECTION('',(0.,0.,1.));
#9198=DIRECTION('center_axis',(0.,0.,1.));
#9199=DIRECTION('ref_axis',(0.60921024449365,-0.793008750269496,0.));
#9200=DIRECTION('',(0.,0.,1.));
#9201=DIRECTION('center_axis',(0.,0.,1.));
#9202=DIRECTION('ref_axis',(0.60921024449365,-0.793008750269496,0.));
#9203=DIRECTION('',(0.,0.,1.));
#9204=DIRECTION('center_axis',(0.,0.,1.));
#9205=DIRECTION('ref_axis',(0.60921024449365,-0.793008750269496,0.));
#9206=DIRECTION('',(0.,0.,1.));
#9207=DIRECTION('center_axis',(0.,0.,1.));
#9208=DIRECTION('ref_axis',(0.60921024449365,-0.793008750269496,0.));
#9209=DIRECTION('',(0.,0.,1.));
#9210=DIRECTION('center_axis',(0.,0.,1.));
#9211=DIRECTION('ref_axis',(0.60921024449365,-0.793008750269496,0.));
#9212=DIRECTION('',(0.,0.,1.));
#9213=DIRECTION('center_axis',(0.,0.,1.));
#9214=DIRECTION('ref_axis',(0.60921024449365,-0.793008750269496,0.));
#9215=DIRECTION('',(0.,0.,1.));
#9216=DIRECTION('center_axis',(0.,0.,1.));
#9217=DIRECTION('ref_axis',(0.60921024449365,-0.793008750269496,0.));
#9218=DIRECTION('',(0.,0.,1.));
#9219=DIRECTION('center_axis',(0.,0.,1.));
#9220=DIRECTION('ref_axis',(0.60921024449365,-0.793008750269496,0.));
#9221=DIRECTION('',(0.,0.,1.));
#9222=DIRECTION('center_axis',(0.,0.,1.));
#9223=DIRECTION('ref_axis',(0.60921024449365,-0.793008750269496,0.));
#9224=DIRECTION('',(0.,0.,1.));
#9225=DIRECTION('center_axis',(0.,0.,1.));
#9226=DIRECTION('ref_axis',(0.60921024449365,-0.793008750269496,0.));
#9227=DIRECTION('',(0.,0.,1.));
#9228=DIRECTION('center_axis',(0.,0.,1.));
#9229=DIRECTION('ref_axis',(0.60921024449365,-0.793008750269496,0.));
#9230=DIRECTION('',(0.,0.,1.));
#9231=DIRECTION('center_axis',(0.,0.,1.));
#9232=DIRECTION('ref_axis',(0.60921024449365,-0.793008750269496,0.));
#9233=DIRECTION('',(0.,0.,1.));
#9234=DIRECTION('center_axis',(0.,0.,1.));
#9235=DIRECTION('ref_axis',(0.60921024449365,-0.793008750269496,0.));
#9236=DIRECTION('',(0.,0.,1.));
#9237=DIRECTION('center_axis',(0.,0.,1.));
#9238=DIRECTION('ref_axis',(0.60921024449365,-0.793008750269496,0.));
#9239=DIRECTION('',(0.,0.,1.));
#9240=DIRECTION('center_axis',(0.,0.,1.));
#9241=DIRECTION('ref_axis',(0.60921024449365,-0.793008750269496,0.));
#9242=DIRECTION('',(0.,0.,1.));
#9243=DIRECTION('center_axis',(0.,0.,1.));
#9244=DIRECTION('ref_axis',(0.60921024449365,-0.793008750269496,0.));
#9245=DIRECTION('',(0.,0.,1.));
#9246=DIRECTION('center_axis',(0.,0.,1.));
#9247=DIRECTION('ref_axis',(0.60921024449365,-0.793008750269496,0.));
#9248=DIRECTION('',(0.,0.,1.));
#9249=DIRECTION('center_axis',(0.,0.,1.));
#9250=DIRECTION('ref_axis',(-1.,-8.91852360097567E-14,0.));
#9251=DIRECTION('center_axis',(0.,0.,1.));
#9252=DIRECTION('ref_axis',(-0.938002783430529,-0.346627722890971,0.));
#9253=DIRECTION('',(0.,0.,1.));
#9254=DIRECTION('center_axis',(0.,0.,-1.));
#9255=DIRECTION('ref_axis',(-1.,0.,0.));
#9256=DIRECTION('',(0.,0.,1.));
#9257=DIRECTION('center_axis',(0.,0.,-1.));
#9258=DIRECTION('ref_axis',(-1.,0.,0.));
#9259=DIRECTION('center_axis',(0.,0.,-1.));
#9260=DIRECTION('ref_axis',(-1.,0.,0.));
#9261=DIRECTION('center_axis',(0.,0.,1.));
#9262=DIRECTION('ref_axis',(-0.938002783430529,-0.346627722890971,0.));
#9263=DIRECTION('',(0.,0.,1.));
#9264=DIRECTION('center_axis',(0.,0.,1.));
#9265=DIRECTION('ref_axis',(-0.938002783430529,-0.346627722890971,0.));
#9266=DIRECTION('',(0.,0.,1.));
#9267=DIRECTION('center_axis',(0.,0.,1.));
#9268=DIRECTION('ref_axis',(-0.938002783430529,-0.346627722890971,0.));
#9269=DIRECTION('',(0.,0.,1.));
#9270=DIRECTION('center_axis',(0.,0.,1.));
#9271=DIRECTION('ref_axis',(-0.938002783430529,-0.346627722890971,0.));
#9272=DIRECTION('',(0.,0.,1.));
#9273=DIRECTION('center_axis',(0.,0.,1.));
#9274=DIRECTION('ref_axis',(-0.938002783430529,-0.346627722890971,0.));
#9275=DIRECTION('',(0.,0.,1.));
#9276=DIRECTION('center_axis',(0.,0.,1.));
#9277=DIRECTION('ref_axis',(-0.938002783430529,-0.346627722890971,0.));
#9278=DIRECTION('',(0.,0.,1.));
#9279=DIRECTION('center_axis',(0.,0.,1.));
#9280=DIRECTION('ref_axis',(-0.938002783430529,-0.346627722890971,0.));
#9281=DIRECTION('',(0.,0.,1.));
#9282=DIRECTION('center_axis',(0.,0.,1.));
#9283=DIRECTION('ref_axis',(-0.938002783430529,-0.346627722890971,0.));
#9284=DIRECTION('',(0.,0.,1.));
#9285=DIRECTION('center_axis',(0.,0.,1.));
#9286=DIRECTION('ref_axis',(-0.938002783430529,-0.346627722890971,0.));
#9287=DIRECTION('',(0.,0.,1.));
#9288=DIRECTION('center_axis',(0.,0.,1.));
#9289=DIRECTION('ref_axis',(-0.938002783430529,-0.346627722890971,0.));
#9290=DIRECTION('',(0.,0.,1.));
#9291=DIRECTION('center_axis',(0.,0.,1.));
#9292=DIRECTION('ref_axis',(-0.938002783430529,-0.346627722890971,0.));
#9293=DIRECTION('',(0.,0.,1.));
#9294=DIRECTION('center_axis',(0.,0.,1.));
#9295=DIRECTION('ref_axis',(-0.938002783430529,-0.346627722890971,0.));
#9296=DIRECTION('',(0.,0.,1.));
#9297=DIRECTION('center_axis',(0.,0.,1.));
#9298=DIRECTION('ref_axis',(-0.938002783430529,-0.346627722890971,0.));
#9299=DIRECTION('',(0.,0.,1.));
#9300=DIRECTION('center_axis',(0.,0.,1.));
#9301=DIRECTION('ref_axis',(-0.938002783430529,-0.346627722890971,0.));
#9302=DIRECTION('',(0.,0.,1.));
#9303=DIRECTION('center_axis',(0.,0.,1.));
#9304=DIRECTION('ref_axis',(-0.938002783430529,-0.346627722890971,0.));
#9305=DIRECTION('',(0.,0.,1.));
#9306=DIRECTION('center_axis',(0.,0.,1.));
#9307=DIRECTION('ref_axis',(-0.938002783430529,-0.346627722890971,0.));
#9308=DIRECTION('',(0.,0.,1.));
#9309=DIRECTION('center_axis',(0.,0.,1.));
#9310=DIRECTION('ref_axis',(-0.938002783430529,-0.346627722890971,0.));
#9311=DIRECTION('',(0.,0.,1.));
#9312=DIRECTION('center_axis',(0.,0.,1.));
#9313=DIRECTION('ref_axis',(-0.938002783430529,-0.346627722890971,0.));
#9314=DIRECTION('',(0.,0.,1.));
#9315=DIRECTION('center_axis',(0.,0.,-1.));
#9316=DIRECTION('ref_axis',(-1.,0.,0.));
#9317=DIRECTION('center_axis',(0.,0.,-1.));
#9318=DIRECTION('ref_axis',(-0.609201867263802,-0.793015185808126,0.));
#9319=DIRECTION('',(0.,0.,-1.));
#9320=DIRECTION('center_axis',(0.,0.,1.));
#9321=DIRECTION('ref_axis',(1.,-1.05172447564359E-13,0.));
#9322=DIRECTION('center_axis',(0.,0.,-1.));
#9323=DIRECTION('ref_axis',(-0.609201867263802,-0.793015185808126,0.));
#9324=DIRECTION('',(0.,0.,-1.));
#9325=DIRECTION('center_axis',(0.,0.,-1.));
#9326=DIRECTION('ref_axis',(-0.609201867263802,-0.793015185808126,0.));
#9327=DIRECTION('',(0.,0.,-1.));
#9328=DIRECTION('center_axis',(0.,0.,-1.));
#9329=DIRECTION('ref_axis',(-0.609201867263802,-0.793015185808126,0.));
#9330=DIRECTION('',(0.,0.,-1.));
#9331=DIRECTION('center_axis',(0.,0.,-1.));
#9332=DIRECTION('ref_axis',(-0.609201867263802,-0.793015185808126,0.));
#9333=DIRECTION('',(0.,0.,-1.));
#9334=DIRECTION('center_axis',(0.,0.,-1.));
#9335=DIRECTION('ref_axis',(-0.609201867263802,-0.793015185808126,0.));
#9336=DIRECTION('',(0.,0.,-1.));
#9337=DIRECTION('center_axis',(0.,0.,-1.));
#9338=DIRECTION('ref_axis',(-0.609201867263802,-0.793015185808126,0.));
#9339=DIRECTION('',(0.,0.,-1.));
#9340=DIRECTION('center_axis',(0.,0.,-1.));
#9341=DIRECTION('ref_axis',(-0.609201867263802,-0.793015185808126,0.));
#9342=DIRECTION('',(0.,0.,-1.));
#9343=DIRECTION('center_axis',(0.,0.,-1.));
#9344=DIRECTION('ref_axis',(-0.609201867263802,-0.793015185808126,0.));
#9345=DIRECTION('',(0.,0.,-1.));
#9346=DIRECTION('center_axis',(0.,0.,-1.));
#9347=DIRECTION('ref_axis',(-0.609201867263802,-0.793015185808126,0.));
#9348=DIRECTION('',(0.,0.,-1.));
#9349=DIRECTION('center_axis',(0.,0.,-1.));
#9350=DIRECTION('ref_axis',(-0.609201867263802,-0.793015185808126,0.));
#9351=DIRECTION('',(0.,0.,-1.));
#9352=DIRECTION('center_axis',(0.,0.,-1.));
#9353=DIRECTION('ref_axis',(-0.609201867263802,-0.793015185808126,0.));
#9354=DIRECTION('',(0.,0.,-1.));
#9355=DIRECTION('center_axis',(0.,0.,-1.));
#9356=DIRECTION('ref_axis',(-0.609201867263802,-0.793015185808126,0.));
#9357=DIRECTION('',(0.,0.,-1.));
#9358=DIRECTION('center_axis',(0.,0.,-1.));
#9359=DIRECTION('ref_axis',(-0.609201867263802,-0.793015185808126,0.));
#9360=DIRECTION('',(0.,0.,-1.));
#9361=DIRECTION('center_axis',(0.,0.,-1.));
#9362=DIRECTION('ref_axis',(-0.609201867263802,-0.793015185808126,0.));
#9363=DIRECTION('',(0.,0.,-1.));
#9364=DIRECTION('center_axis',(0.,0.,-1.));
#9365=DIRECTION('ref_axis',(-0.609201867263802,-0.793015185808126,0.));
#9366=DIRECTION('',(0.,0.,-1.));
#9367=DIRECTION('center_axis',(0.,0.,-1.));
#9368=DIRECTION('ref_axis',(-0.609201867263802,-0.793015185808126,0.));
#9369=DIRECTION('',(0.,0.,-1.));
#9370=DIRECTION('center_axis',(0.,0.,-1.));
#9371=DIRECTION('ref_axis',(-0.609201867263802,-0.793015185808126,0.));
#9372=DIRECTION('',(0.,0.,-1.));
#9373=DIRECTION('center_axis',(0.,0.,-1.));
#9374=DIRECTION('ref_axis',(-0.609201867263802,-0.793015185808126,0.));
#9375=DIRECTION('',(0.,0.,-1.));
#9376=DIRECTION('center_axis',(0.,0.,-1.));
#9377=DIRECTION('ref_axis',(1.,-1.05172447564359E-13,0.));
#9378=DIRECTION('center_axis',(0.,0.,-1.));
#9379=DIRECTION('ref_axis',(0.938006403579049,-0.346617926317579,0.));
#9380=DIRECTION('',(0.,0.,-1.));
#9381=DIRECTION('center_axis',(0.,0.,1.));
#9382=DIRECTION('ref_axis',(1.,0.,0.));
#9383=DIRECTION('',(0.,0.,-1.));
#9384=DIRECTION('center_axis',(0.,0.,1.));
#9385=DIRECTION('ref_axis',(1.,0.,0.));
#9386=DIRECTION('center_axis',(0.,0.,1.));
#9387=DIRECTION('ref_axis',(1.,0.,0.));
#9388=DIRECTION('center_axis',(0.,0.,-1.));
#9389=DIRECTION('ref_axis',(0.938006403579049,-0.346617926317579,0.));
#9390=DIRECTION('',(0.,0.,-1.));
#9391=DIRECTION('center_axis',(0.,0.,-1.));
#9392=DIRECTION('ref_axis',(0.938006403579049,-0.346617926317579,0.));
#9393=DIRECTION('',(0.,0.,-1.));
#9394=DIRECTION('center_axis',(0.,0.,-1.));
#9395=DIRECTION('ref_axis',(0.938006403579049,-0.346617926317579,0.));
#9396=DIRECTION('',(0.,0.,-1.));
#9397=DIRECTION('center_axis',(0.,0.,-1.));
#9398=DIRECTION('ref_axis',(0.938006403579049,-0.346617926317579,0.));
#9399=DIRECTION('',(0.,0.,-1.));
#9400=DIRECTION('center_axis',(0.,0.,-1.));
#9401=DIRECTION('ref_axis',(0.938006403579049,-0.346617926317579,0.));
#9402=DIRECTION('',(0.,0.,-1.));
#9403=DIRECTION('center_axis',(0.,0.,-1.));
#9404=DIRECTION('ref_axis',(0.938006403579049,-0.346617926317579,0.));
#9405=DIRECTION('',(0.,0.,-1.));
#9406=DIRECTION('center_axis',(0.,0.,-1.));
#9407=DIRECTION('ref_axis',(0.938006403579049,-0.346617926317579,0.));
#9408=DIRECTION('',(0.,0.,-1.));
#9409=DIRECTION('center_axis',(0.,0.,-1.));
#9410=DIRECTION('ref_axis',(0.938006403579049,-0.346617926317579,0.));
#9411=DIRECTION('',(0.,0.,-1.));
#9412=DIRECTION('center_axis',(0.,0.,-1.));
#9413=DIRECTION('ref_axis',(0.938006403579049,-0.346617926317579,0.));
#9414=DIRECTION('',(0.,0.,-1.));
#9415=DIRECTION('center_axis',(0.,0.,-1.));
#9416=DIRECTION('ref_axis',(0.938006403579049,-0.346617926317579,0.));
#9417=DIRECTION('',(0.,0.,-1.));
#9418=DIRECTION('center_axis',(0.,0.,-1.));
#9419=DIRECTION('ref_axis',(0.938006403579049,-0.346617926317579,0.));
#9420=DIRECTION('',(0.,0.,-1.));
#9421=DIRECTION('center_axis',(0.,0.,-1.));
#9422=DIRECTION('ref_axis',(0.938006403579049,-0.346617926317579,0.));
#9423=DIRECTION('',(0.,0.,-1.));
#9424=DIRECTION('center_axis',(0.,0.,-1.));
#9425=DIRECTION('ref_axis',(0.938006403579049,-0.346617926317579,0.));
#9426=DIRECTION('',(0.,0.,-1.));
#9427=DIRECTION('center_axis',(0.,0.,-1.));
#9428=DIRECTION('ref_axis',(0.938006403579049,-0.346617926317579,0.));
#9429=DIRECTION('',(0.,0.,-1.));
#9430=DIRECTION('center_axis',(0.,0.,-1.));
#9431=DIRECTION('ref_axis',(0.938006403579049,-0.346617926317579,0.));
#9432=DIRECTION('',(0.,0.,-1.));
#9433=DIRECTION('center_axis',(0.,0.,-1.));
#9434=DIRECTION('ref_axis',(0.938006403579049,-0.346617926317579,0.));
#9435=DIRECTION('',(0.,0.,-1.));
#9436=DIRECTION('center_axis',(0.,0.,-1.));
#9437=DIRECTION('ref_axis',(0.938006403579049,-0.346617926317579,0.));
#9438=DIRECTION('',(0.,0.,-1.));
#9439=DIRECTION('center_axis',(0.,0.,-1.));
#9440=DIRECTION('ref_axis',(0.938006403579049,-0.346617926317579,0.));
#9441=DIRECTION('',(0.,0.,-1.));
#9442=DIRECTION('center_axis',(0.,0.,-1.));
#9443=DIRECTION('ref_axis',(1.,0.,0.));
#9444=DIRECTION('center_axis',(0.,0.,-1.));
#9445=DIRECTION('ref_axis',(0.938006403579049,-0.346617926317579,0.));
#9446=DIRECTION('center_axis',(0.,0.,-1.));
#9447=DIRECTION('ref_axis',(-0.609201867263802,-0.793015185808126,0.));
#9448=DIRECTION('center_axis',(0.,0.,1.));
#9449=DIRECTION('ref_axis',(-0.938002783430529,-0.346627722890971,0.));
#9450=DIRECTION('center_axis',(0.,0.,1.));
#9451=DIRECTION('ref_axis',(0.60921024449365,-0.793008750269496,0.));
#9452=DIRECTION('center_axis',(0.,0.,1.));
#9453=DIRECTION('ref_axis',(1.,0.,0.));
#9454=DIRECTION('center_axis',(0.,0.,1.));
#9455=DIRECTION('ref_axis',(-1.,0.,0.));
#9456=DIRECTION('center_axis',(0.,0.,1.));
#9457=DIRECTION('ref_axis',(1.,0.,0.));
#9458=DIRECTION('center_axis',(0.,0.,-1.));
#9459=DIRECTION('ref_axis',(1.,0.,0.));
#9460=DIRECTION('center_axis',(0.,0.,1.));
#9461=DIRECTION('ref_axis',(1.,0.,0.));
#9462=DIRECTION('center_axis',(0.,0.,1.));
#9463=DIRECTION('ref_axis',(1.,0.,0.));
#9464=DIRECTION('',(0.,0.,-1.));
#9465=DIRECTION('center_axis',(0.,0.,1.));
#9466=DIRECTION('ref_axis',(1.,0.,0.));
#9467=DIRECTION('center_axis',(0.,0.,1.));
#9468=DIRECTION('ref_axis',(1.,0.,0.));
#9469=DIRECTION('center_axis',(0.,0.,1.));
#9470=DIRECTION('ref_axis',(1.,0.,0.));
#10602=CARTESIAN_POINT('',(0.,0.,0.));
#10603=CARTESIAN_POINT('Origin',(0.,0.,-2.20842344717744));
#10604=CARTESIAN_POINT('',(-1.87240768645123,2.4373123939533,18.5627733953368));
#10605=CARTESIAN_POINT('',(-1.87240768645124,2.43731239395329,18.6457505235039));
#10606=CARTESIAN_POINT('',(-1.87240768645123,2.4373123939533,-2.20842344717744));
#10607=CARTESIAN_POINT('',(-0.793799282532847,-2.9692229537457,19.));
#10608=CARTESIAN_POINT('Ctrl Pts',(-1.87240768645124,2.43731239395329,18.6457505235039));
#10609=CARTESIAN_POINT('Ctrl Pts',(-1.94899259408632,2.37847784731174,18.6507492320743));
#10610=CARTESIAN_POINT('Ctrl Pts',(-2.02273224209293,2.31608369066104,18.6557479406448));
#10611=CARTESIAN_POINT('Ctrl Pts',(-2.09329518872703,2.25044828930866,18.6607466492152));
#10612=CARTESIAN_POINT('Ctrl Pts',(-2.16397015698635,2.18470868901501,18.6657532934443));
#10613=CARTESIAN_POINT('Ctrl Pts',(-2.23145804949518,2.11571788291669,18.6707599376733));
#10614=CARTESIAN_POINT('Ctrl Pts',(-2.29546581565982,2.04382947897744,18.6757665819024));
#10615=CARTESIAN_POINT('Ctrl Pts',(-2.32740848703842,2.00795402509804,18.6782651160788));
#10616=CARTESIAN_POINT('Ctrl Pts',(-2.35848510104462,1.97135743377959,18.6807636502553));
#10617=CARTESIAN_POINT('Ctrl Pts',(-2.38866325982295,1.93408636859164,18.6832621844317));
#10618=CARTESIAN_POINT('Ctrl Pts',(-2.44839709830004,1.86031302131227,18.6882077160004));
#10619=CARTESIAN_POINT('Ctrl Pts',(-2.5048278901498,1.78362392824008,18.6931532475691));
#10620=CARTESIAN_POINT('Ctrl Pts',(-2.55765354176341,1.7043504951462,18.6980987791378));
#10621=CARTESIAN_POINT('Ctrl Pts',(-2.61040637785506,1.62518633351858,18.7030374937256));
#10622=CARTESIAN_POINT('Ctrl Pts',(-2.65956369759587,1.5434452776277,18.7079762083133));
#10623=CARTESIAN_POINT('Ctrl Pts',(-2.70486310812873,1.45949231456839,18.712914922901));
#10624=CARTESIAN_POINT('Ctrl Pts',(-2.75011446193948,1.37562841457122,18.7178483981616));
#10625=CARTESIAN_POINT('Ctrl Pts',(-2.79151582599366,1.28955766248506,18.7227818734221));
#10626=CARTESIAN_POINT('Ctrl Pts',(-2.8288483148355,1.20167360861939,18.7277153486826));
#10627=CARTESIAN_POINT('Ctrl Pts',(-2.86615566208602,1.11384874033268,18.7326455014907));
#10628=CARTESIAN_POINT('Ctrl Pts',(-2.89939940145408,1.02421340789372,18.7375756542988));
#10629=CARTESIAN_POINT('Ctrl Pts',(-2.92840727959673,0.933184362709153,
18.7425058071068));
#10630=CARTESIAN_POINT('Ctrl Pts',(-2.95740541870615,0.842185879390947,
18.7474343046776));
#10631=CARTESIAN_POINT('Ctrl Pts',(-2.98217038382058,0.749795039982814,
18.7523628022484));
#10632=CARTESIAN_POINT('Ctrl Pts',(-3.00257903406844,0.656446032947613,
18.7572912998191));
#10633=CARTESIAN_POINT('Ctrl Pts',(-3.02298669367368,0.563101557104024,
18.762219558159));
#10634=CARTESIAN_POINT('Ctrl Pts',(-3.03903836267948,0.46879944501066,18.7671478164989));
#10635=CARTESIAN_POINT('Ctrl Pts',(-3.05066178046823,0.373985228572495,
18.7720760748388));
#10636=CARTESIAN_POINT('Ctrl Pts',(-3.06228797249442,0.279148382202736,
18.7770055094384));
#10637=CARTESIAN_POINT('Ctrl Pts',(-3.06948376034883,0.183799634724477,
18.7819349440381));
#10638=CARTESIAN_POINT('Ctrl Pts',(-3.07222875606254,0.0883895945368608,
18.7868643786377));
#10639=CARTESIAN_POINT('Ctrl Pts',(-3.07497714791223,-0.00713848790058853,
18.7917999119828));
#10640=CARTESIAN_POINT('Ctrl Pts',(-3.07326374320136,-0.10272756458361,
18.796735445328));
#10641=CARTESIAN_POINT('Ctrl Pts',(-3.06712031399051,-0.197927333905002,
18.8016709786731));
#10642=CARTESIAN_POINT('Ctrl Pts',(-3.06097281995468,-0.293190092541926,
18.806609777634));
#10643=CARTESIAN_POINT('Ctrl Pts',(-3.05038952050478,-0.388062585579013,
18.8115485765948));
#10644=CARTESIAN_POINT('Ctrl Pts',(-3.03545377308445,-0.482102314314468,
18.8164873755557));
#10645=CARTESIAN_POINT('Ctrl Pts',(-3.02049049731446,-0.576315369396592,
18.8214352773074));
#10646=CARTESIAN_POINT('Ctrl Pts',(-3.00115884957716,-0.669692156824441,
18.8263831790592));
#10647=CARTESIAN_POINT('Ctrl Pts',(-2.97759271814336,-0.761803028912078,
18.8313310808109));
#10648=CARTESIAN_POINT('Ctrl Pts',(-2.96124023617427,-0.825718541697934,
18.8347644179459));
#10649=CARTESIAN_POINT('Ctrl Pts',(-2.94284992820392,-0.889024842653302,
18.8381977550809));
#10650=CARTESIAN_POINT('Ctrl Pts',(-2.92248003136601,-0.95158431905266,
18.8416310922159));
#10651=CARTESIAN_POINT('Ctrl Pts',(-2.89199283230741,-1.04521578047666,
18.8467696961815));
#10652=CARTESIAN_POINT('Ctrl Pts',(-2.85695819522448,-1.13751478481036,
18.851908300147));
#10653=CARTESIAN_POINT('Ctrl Pts',(-2.8175101424337,-1.22802233175267,18.8570469041126));
#10654=CARTESIAN_POINT('Ctrl Pts',(-2.77812125277038,-1.31839413791291,
18.8621778013383));
#10655=CARTESIAN_POINT('Ctrl Pts',(-2.73433228100744,-1.40697946042347,
18.867308698564));
#10656=CARTESIAN_POINT('Ctrl Pts',(-2.68632654671846,-1.49333584112739,
18.8724395957898));
#10657=CARTESIAN_POINT('Ctrl Pts',(-2.63659815126665,-1.58279107627869,
18.8777546126318));
#10658=CARTESIAN_POINT('Ctrl Pts',(-2.5823447794107,-1.66985396060582,18.8830696294739));
#10659=CARTESIAN_POINT('Ctrl Pts',(-2.5238245897669,-1.75405578306049,18.888384646316));
#10660=CARTESIAN_POINT('Ctrl Pts',(-2.46747194348866,-1.83513883398108,
18.8935027989722));
#10661=CARTESIAN_POINT('Ctrl Pts',(-2.40716320133204,-1.91356862756652,
18.8986209516284));
#10662=CARTESIAN_POINT('Ctrl Pts',(-2.34317480499982,-1.98895301181654,
18.9037391042846));
#10663=CARTESIAN_POINT('Ctrl Pts',(-2.27923049055607,-2.06428546343174,
18.9088537310228));
#10664=CARTESIAN_POINT('Ctrl Pts',(-2.21161183051787,-2.1365763693934,18.913968357761));
#10665=CARTESIAN_POINT('Ctrl Pts',(-2.14063640845943,-2.20546548755085,
18.9190829844993));
#10666=CARTESIAN_POINT('Ctrl Pts',(-2.06969460595462,-2.27432197439262,
18.9241951885472));
#10667=CARTESIAN_POINT('Ctrl Pts',(-1.99539949979887,-2.33977959626579,
18.9293073925951));
#10668=CARTESIAN_POINT('Ctrl Pts',(-1.91810601416181,-2.40151443227732,
18.934419596643));
#10669=CARTESIAN_POINT('Ctrl Pts',(-1.84083251662006,-2.46323330366033,
18.939530478675));
#10670=CARTESIAN_POINT('Ctrl Pts',(-1.7605625036411,-2.52123105148741,18.9446413607069));
#10671=CARTESIAN_POINT('Ctrl Pts',(-1.67768396001371,-2.57522402526707,
18.9497522427389));
#10672=CARTESIAN_POINT('Ctrl Pts',(-1.59478764470598,-2.62922857678238,
18.9548642206994));
#10673=CARTESIAN_POINT('Ctrl Pts',(-1.50928202221776,-2.67922641180854,
18.9599761986599));
#10674=CARTESIAN_POINT('Ctrl Pts',(-1.4215837615457,-2.72497740521084,18.9650881766204));
#10675=CARTESIAN_POINT('Ctrl Pts',(-1.33387548538877,-2.77073362355578,
18.9702007383888));
#10676=CARTESIAN_POINT('Ctrl Pts',(-1.24397443858875,-2.81224185129505,
18.9753133001572));
#10677=CARTESIAN_POINT('Ctrl Pts',(-1.15232053332067,-2.84930862464696,
18.9804258619256));
#10678=CARTESIAN_POINT('Ctrl Pts',(-1.06060824867288,-2.88639900785194,
18.9855416801639));
#10679=CARTESIAN_POINT('Ctrl Pts',(-0.967141258677279,-2.91904214160113,
18.9906574984022));
#10680=CARTESIAN_POINT('Ctrl Pts',(-0.872377774838882,-2.94709335922145,
18.9957733166406));
#10681=CARTESIAN_POINT('Ctrl Pts',(-0.846279946393651,-2.95481865419249,
18.9971822110937));
#10682=CARTESIAN_POINT('Ctrl Pts',(-0.820083868285662,-2.96219596869362,
18.9985911055469));
#10683=CARTESIAN_POINT('Ctrl Pts',(-0.793799282532847,-2.9692229537457,
19.));
#10684=CARTESIAN_POINT('',(0.793800071764984,-2.96922274275035,18.9999843185276));
#10685=CARTESIAN_POINT('Origin',(0.,0.,19.));
#10686=CARTESIAN_POINT('Ctrl Pts',(-1.87240768645123,2.4373123939533,18.5627733953368));
#10687=CARTESIAN_POINT('Ctrl Pts',(-1.95202497174946,2.37614829478545,18.5679716338033));
#10688=CARTESIAN_POINT('Ctrl Pts',(-2.02872648937363,2.31101413800602,18.5731698722698));
#10689=CARTESIAN_POINT('Ctrl Pts',(-2.10209926441082,2.24222677991399,18.5783681107363));
#10690=CARTESIAN_POINT('Ctrl Pts',(-2.17233753654655,2.17637803458964,18.5833442791837));
#10691=CARTESIAN_POINT('Ctrl Pts',(-2.23952528158551,2.10718214798762,18.5883204476311));
#10692=CARTESIAN_POINT('Ctrl Pts',(-2.30333394996718,2.03495822191233,18.5932966160784));
#10693=CARTESIAN_POINT('Ctrl Pts',(-2.36712461846038,1.9627546695989,18.5982713807906));
#10694=CARTESIAN_POINT('Ctrl Pts',(-2.42753781287959,1.88752510479804,18.6032461455027));
#10695=CARTESIAN_POINT('Ctrl Pts',(-2.48428317614486,1.8096240909989,18.6082209102148));
#10696=CARTESIAN_POINT('Ctrl Pts',(-2.54102813984596,1.73172362572836,18.6131956398978));
#10697=CARTESIAN_POINT('Ctrl Pts',(-2.59410506502922,1.65115210523789,18.6181703695809));
#10698=CARTESIAN_POINT('Ctrl Pts',(-2.64326574704364,1.5682947556202,18.6231450992639));
#10699=CARTESIAN_POINT('Ctrl Pts',(-2.69243960448518,1.48541519961873,18.6281211622114));
#10700=CARTESIAN_POINT('Ctrl Pts',(-2.7376949094152,1.40024897630273,18.6330972251589));
#10701=CARTESIAN_POINT('Ctrl Pts',(-2.77882895177474,1.31320672659657,18.6380732881063));
#10702=CARTESIAN_POINT('Ctrl Pts',(-2.82000986965535,1.22606528530661,18.6430550216743));
#10703=CARTESIAN_POINT('Ctrl Pts',(-2.85705996437771,1.13704394986257,18.6480367552422));
#10704=CARTESIAN_POINT('Ctrl Pts',(-2.88982443219444,1.04657393484267,18.6530184888102));
#10705=CARTESIAN_POINT('Ctrl Pts',(-2.92261088577821,0.95604321220851,18.6580035652444));
#10706=CARTESIAN_POINT('Ctrl Pts',(-2.9511058585197,0.864062295027149,18.6629886416786));
#10707=CARTESIAN_POINT('Ctrl Pts',(-2.975204841963,0.771076130067551,18.6679737181128));
#10708=CARTESIAN_POINT('Ctrl Pts',(-2.99934142645839,0.677944881078109,
18.6729665726394));
#10709=CARTESIAN_POINT('Ctrl Pts',(-3.01906824474975,0.583805684132802,
18.6779594271659));
#10710=CARTESIAN_POINT('Ctrl Pts',(-3.03433217735862,0.489111937542002,
18.6829522816925));
#10711=CARTESIAN_POINT('Ctrl Pts',(-3.03899824941449,0.46016475491518,18.6844785606392));
#10712=CARTESIAN_POINT('Ctrl Pts',(-3.04324764171201,0.431165770154121,
18.686004839586));
#10713=CARTESIAN_POINT('Ctrl Pts',(-3.04707980808541,0.402127956200752,
18.6875311185327));
#10714=CARTESIAN_POINT('Ctrl Pts',(-3.05965639508212,0.30683026873236,18.6925401338219));
#10715=CARTESIAN_POINT('Ctrl Pts',(-3.06777977856026,0.210777340040537,
18.697549149111));
#10716=CARTESIAN_POINT('Ctrl Pts',(-3.07136944940218,0.114420082498388,
18.7025581644002));
#10717=CARTESIAN_POINT('Ctrl Pts',(-3.07495424103575,0.018193797169766,
18.7075603712575));
#10718=CARTESIAN_POINT('Ctrl Pts',(-3.07401755234348,-0.0783355616180718,
18.7125625781148));
#10719=CARTESIAN_POINT('Ctrl Pts',(-3.06853038122612,-0.174709900956579,
18.7175647849721));
#10720=CARTESIAN_POINT('Ctrl Pts',(-3.0630490308355,-0.270982007526868,
18.7225616855471));
#10721=CARTESIAN_POINT('Ctrl Pts',(-3.05302681956203,-0.367098987402478,
18.7275585861221));
#10722=CARTESIAN_POINT('Ctrl Pts',(-3.03848678339903,-0.462601682994587,
18.732555486697));
#10723=CARTESIAN_POINT('Ctrl Pts',(-3.02395741303011,-0.558034322909119,
18.7375487218126));
#10724=CARTESIAN_POINT('Ctrl Pts',(-3.00491687262805,-0.652853143524043,
18.7425419569282));
#10725=CARTESIAN_POINT('Ctrl Pts',(-2.98144003620813,-0.746604018536794,
18.7475351920437));
#10726=CARTESIAN_POINT('Ctrl Pts',(-2.95797203227419,-0.840319622473202,
18.7525265485979));
#10727=CARTESIAN_POINT('Ctrl Pts',(-2.93007115499145,-0.932967655586887,
18.757517905152));
#10728=CARTESIAN_POINT('Ctrl Pts',(-2.89786320815082,-1.02410501260654,
18.7625092617061));
#10729=CARTESIAN_POINT('Ctrl Pts',(-2.86565867477284,-1.11523271070675,
18.7675000892663));
#10730=CARTESIAN_POINT('Ctrl Pts',(-2.82914812531306,-1.20484963895358,
18.7724909168265));
#10731=CARTESIAN_POINT('Ctrl Pts',(-2.78850664465149,-1.29252966802874,
18.7774817443867));
#10732=CARTESIAN_POINT('Ctrl Pts',(-2.74785848859646,-1.38022409861397,
18.782473391694));
#10733=CARTESIAN_POINT('Ctrl Pts',(-2.70307823772816,-1.4659806016047,18.7874650390013));
#10734=CARTESIAN_POINT('Ctrl Pts',(-2.65438789732525,-1.54939573399866,
18.7924566863087));
#10735=CARTESIAN_POINT('Ctrl Pts',(-2.60564698570869,-1.6328975037923,18.7974535180871));
#10736=CARTESIAN_POINT('Ctrl Pts',(-2.55298809732327,-1.71405266973642,
18.8024503498655));
#10737=CARTESIAN_POINT('Ctrl Pts',(-2.49667761527606,-1.79248518414503,
18.8074471816439));
#10738=CARTESIAN_POINT('Ctrl Pts',(-2.44033496820012,-1.87096249987637,
18.8124468676554));
#10739=CARTESIAN_POINT('Ctrl Pts',(-2.38033684479047,-1.94671372420204,
18.8174465536668));
#10740=CARTESIAN_POINT('Ctrl Pts',(-2.31698981315392,-2.01939606212871,
18.8224462396782));
#10741=CARTESIAN_POINT('Ctrl Pts',(-2.25354352263576,-2.09219228648999,
18.8274537597307));
#10742=CARTESIAN_POINT('Ctrl Pts',(-2.18673814776625,-2.16190970667863,
18.8324612797831));
#10743=CARTESIAN_POINT('Ctrl Pts',(-2.11691691042164,-2.2282425910055,18.8374687998355));
#10744=CARTESIAN_POINT('Ctrl Pts',(-2.07773060268851,-2.26547110366031,
18.8402792086627));
#10745=CARTESIAN_POINT('Ctrl Pts',(-2.03759494160999,-2.30163425068253,
18.8430896174898));
#10746=CARTESIAN_POINT('Ctrl Pts',(-1.99657483514119,-2.33668379925075,
18.8459000263169));
#10747=CARTESIAN_POINT('Ctrl Pts',(-1.92384403406119,-2.39882848789992,
18.8508830286286));
#10748=CARTESIAN_POINT('Ctrl Pts',(-1.84807908471453,-2.45768521307757,
18.8558660309403));
#10749=CARTESIAN_POINT('Ctrl Pts',(-1.76961069950184,-2.51294254256013,
18.860849033252));
#10750=CARTESIAN_POINT('Ctrl Pts',(-1.69124716159385,-2.56812603871422,
18.8658253774126));
#10751=CARTESIAN_POINT('Ctrl Pts',(-1.61018772438855,-2.61971944386175,
18.8708017215732));
#10752=CARTESIAN_POINT('Ctrl Pts',(-1.52679728102083,-2.6674505267516,18.8757780657338));
#10753=CARTESIAN_POINT('Ctrl Pts',(-1.44007352228023,-2.7170895351295,18.8809533262669));
#10754=CARTESIAN_POINT('Ctrl Pts',(-1.35082886036575,-2.76255065514993,
18.8861285868));
#10755=CARTESIAN_POINT('Ctrl Pts',(-1.25950866889961,-2.80357631659399,
18.8913038473331));
#10756=CARTESIAN_POINT('Ctrl Pts',(-1.1718498128674,-2.84295712047113,18.8962716141622));
#10757=CARTESIAN_POINT('Ctrl Pts',(-1.08227910453418,-2.87825109438257,
18.9012393809914));
#10758=CARTESIAN_POINT('Ctrl Pts',(-0.991215645650244,-2.90927719439351,
18.9062071478205));
#10759=CARTESIAN_POINT('Ctrl Pts',(-0.900181330555704,-2.94029336486591,
18.9111733247743));
#10760=CARTESIAN_POINT('Ctrl Pts',(-0.807655632238675,-2.96704423262761,
18.9161395017281));
#10761=CARTESIAN_POINT('Ctrl Pts',(-0.71407584706654,-2.98939758724667,
18.9211056786819));
#10762=CARTESIAN_POINT('Ctrl Pts',(-0.620500023152401,-3.01174999564209,
18.9260716454161));
#10763=CARTESIAN_POINT('Ctrl Pts',(-0.525870631315329,-3.02970515889201,
18.9310376121502));
#10764=CARTESIAN_POINT('Ctrl Pts',(-0.43063719198603,-3.04318153564298,
18.9360035788844));
#10765=CARTESIAN_POINT('Ctrl Pts',(-0.335381336785275,-3.05666108443869,
18.9409707144986));
#10766=CARTESIAN_POINT('Ctrl Pts',(-0.239521589473096,-3.06565969150054,
18.9459378501129));
#10767=CARTESIAN_POINT('Ctrl Pts',(-0.143513543742,-3.07014757182169,18.9509049857271));
#10768=CARTESIAN_POINT('Ctrl Pts',(-0.047400527061884,-3.0746403589926,
18.9558775521877));
#10769=CARTESIAN_POINT('Ctrl Pts',(0.0488606694604206,-3.07461255735108,
18.9608501186482));
#10770=CARTESIAN_POINT('Ctrl Pts',(0.144813823536495,-3.07008651449967,
18.9658226851088));
#10771=CARTESIAN_POINT('Ctrl Pts',(0.240829127043579,-3.06555754010328,
18.9707984723303));
#10772=CARTESIAN_POINT('Ctrl Pts',(0.336535551564223,-3.05652456728976,
18.9757742595519));
#10773=CARTESIAN_POINT('Ctrl Pts',(0.431483474223454,-3.04306165916369,
18.9807500467734));
#10774=CARTESIAN_POINT('Ctrl Pts',(0.526575733441245,-3.02957828518883,
18.9857333980152));
#10775=CARTESIAN_POINT('Ctrl Pts',(0.620906757112716,-3.01165162134643,
18.9907167492569));
#10776=CARTESIAN_POINT('Ctrl Pts',(0.714038869693054,-2.9894064197709,18.9957001004986));
#10777=CARTESIAN_POINT('Ctrl Pts',(0.740727621661937,-2.98303164042897,
18.997128173175));
#10778=CARTESIAN_POINT('Ctrl Pts',(0.767318026974863,-2.97630252452361,
18.9985562458513));
#10779=CARTESIAN_POINT('Ctrl Pts',(0.793800071764984,-2.96922274275035,
18.9999843185276));
#10780=CARTESIAN_POINT('Origin',(0.,0.,-2.20842344717744));
#10781=CARTESIAN_POINT('',(-1.8746299318936,2.44024828799233,17.5625875311804));
#10782=CARTESIAN_POINT('',(-1.87240768645122,2.4373123939533,17.6458577700207));
#10783=CARTESIAN_POINT('',(-1.87240768645123,2.4373123939533,-2.20842344717744));
#10784=CARTESIAN_POINT('',(3.07349994772162,0.000566881991104972,18.2915765528661));
#10785=CARTESIAN_POINT('Ctrl Pts',(-1.87240768645122,2.4373123939533,17.6458577700207));
#10786=CARTESIAN_POINT('Ctrl Pts',(-1.94892700937515,2.37852823121723,17.6508396670982));
#10787=CARTESIAN_POINT('Ctrl Pts',(-2.0226886447178,2.31612696413998,17.6558215641758));
#10788=CARTESIAN_POINT('Ctrl Pts',(-2.09334166204538,2.25040506041581,17.6608034612533));
#10789=CARTESIAN_POINT('Ctrl Pts',(-2.16400280134918,2.18467560157567,17.665785931029));
#10790=CARTESIAN_POINT('Ctrl Pts',(-2.23155429177968,2.11562504719635,17.6707684008046));
#10791=CARTESIAN_POINT('Ctrl Pts',(-2.29568115259007,2.04358760410282,17.6757508705803));
#10792=CARTESIAN_POINT('Ctrl Pts',(-2.35987470346979,1.97147524416458,17.6807385219795));
#10793=CARTESIAN_POINT('Ctrl Pts',(-2.4206362195532,1.89637012043201,17.6857261733787));
#10794=CARTESIAN_POINT('Ctrl Pts',(-2.47769035766569,1.81864035519133,17.690713824778));
#10795=CARTESIAN_POINT('Ctrl Pts',(-2.53477476925467,1.74086934578681,17.6957041226732));
#10796=CARTESIAN_POINT('Ctrl Pts',(-2.5881476418964,1.66047128685132,17.7006944205684));
#10797=CARTESIAN_POINT('Ctrl Pts',(-2.63757762074887,1.57784236998654,17.7056847184636));
#10798=CARTESIAN_POINT('Ctrl Pts',(-2.68709107450033,1.49507391350127,17.7106834437267));
#10799=CARTESIAN_POINT('Ctrl Pts',(-2.73264812472186,1.41006746009895,17.7156821689897));
#10800=CARTESIAN_POINT('Ctrl Pts',(-2.77406388216768,1.32324292087764,17.7206808942527));
#10801=CARTESIAN_POINT('Ctrl Pts',(-2.80822083075527,1.25163584412182,17.724803508744));
#10802=CARTESIAN_POINT('Ctrl Pts',(-2.83956177706021,1.17879263909227,17.7289261232353));
#10803=CARTESIAN_POINT('Ctrl Pts',(-2.86800843670303,1.1049569480302,17.7330487377265));
#10804=CARTESIAN_POINT('Ctrl Pts',(-2.90249867852821,1.01543463250934,17.7380472146142));
#10805=CARTESIAN_POINT('Ctrl Pts',(-2.9328540880347,0.924138278697285,17.7430456915019));
#10806=CARTESIAN_POINT('Ctrl Pts',(-2.95889064443608,0.831485660891783,
17.7480441683895));
#10807=CARTESIAN_POINT('Ctrl Pts',(-2.98489186615198,0.738958783643437,
17.7530358617531));
#10808=CARTESIAN_POINT('Ctrl Pts',(-3.00658576558368,0.645079719611513,
17.7580275551166));
#10809=CARTESIAN_POINT('Ctrl Pts',(-3.02383667694098,0.550285381585332,
17.7630192484801));
#10810=CARTESIAN_POINT('Ctrl Pts',(-3.04106938408581,0.45559107631888,17.7680056743047));
#10811=CARTESIAN_POINT('Ctrl Pts',(-3.05386834532723,0.359983846857202,
17.7729921001294));
#10812=CARTESIAN_POINT('Ctrl Pts',(-3.06214821691609,0.263913901940749,
17.777978525954));
#10813=CARTESIAN_POINT('Ctrl Pts',(-3.07042216901413,0.167912639871801,
17.782961386856));
#10814=CARTESIAN_POINT('Ctrl Pts',(-3.07418341646149,0.0714497562502933,
17.7879442477579));
#10815=CARTESIAN_POINT('Ctrl Pts',(-3.07339818251466,-0.0250172283751209,
17.7929271086599));
#10816=CARTESIAN_POINT('Ctrl Pts',(-3.0726132341693,-0.121449126499266,
17.79790815722));
#10817=CARTESIAN_POINT('Ctrl Pts',(-3.0672850935275,-0.217884683964007,
17.8028892057801));
#10818=CARTESIAN_POINT('Ctrl Pts',(-3.05743207966062,-0.313865143432855,
17.8078702543401));
#10819=CARTESIAN_POINT('Ctrl Pts',(-3.04757995664121,-0.409836924952933,
17.8128508525452));
#10820=CARTESIAN_POINT('Ctrl Pts',(-3.03320381880281,-0.505353253435056,
17.8178314507502));
#10821=CARTESIAN_POINT('Ctrl Pts',(-3.01437387261111,-0.599960337121987,
17.8228120489553));
#10822=CARTESIAN_POINT('Ctrl Pts',(-2.99554048271711,-0.694584722963035,
17.8277935580337));
#10823=CARTESIAN_POINT('Ctrl Pts',(-2.97225175257638,-0.78829910306216,
17.8327750671122));
#10824=CARTESIAN_POINT('Ctrl Pts',(-2.94462881146846,-0.880660781839319,
17.8377565761907));
#10825=CARTESIAN_POINT('Ctrl Pts',(-2.91697601330841,-0.973122292399328,
17.8427434696768));
#10826=CARTESIAN_POINT('Ctrl Pts',(-2.88497977756987,-1.06422776123953,
17.847730363163));
#10827=CARTESIAN_POINT('Ctrl Pts',(-2.8488107845463,-1.15355076344854,17.8527172566491));
#10828=CARTESIAN_POINT('Ctrl Pts',(-2.81262037533797,-1.2429266551012,17.8577071029471));
#10829=CARTESIAN_POINT('Ctrl Pts',(-2.77225247299561,-1.33051757998906,
17.8626969492451));
#10830=CARTESIAN_POINT('Ctrl Pts',(-2.72792457571076,-1.41592011046997,
17.8676867955432));
#10831=CARTESIAN_POINT('Ctrl Pts',(-2.6835248520789,-1.50146102224493,17.872684727098));
#10832=CARTESIAN_POINT('Ctrl Pts',(-2.63515254142937,-1.58480607960722,
17.8776826586528));
#10833=CARTESIAN_POINT('Ctrl Pts',(-2.58306941612667,-1.66557937111116,
17.8826805902075));
#10834=CARTESIAN_POINT('Ctrl Pts',(-2.55271998449031,-1.71264689008769,
17.8855929419753));
#10835=CARTESIAN_POINT('Ctrl Pts',(-2.52111132603805,-1.75884173985027,
17.888505293743));
#10836=CARTESIAN_POINT('Ctrl Pts',(-2.48830142754434,-1.80409485772806,
17.8914176455108));
#10837=CARTESIAN_POINT('Ctrl Pts',(-2.43196544577463,-1.88179637284473,
17.8964182765285));
#10838=CARTESIAN_POINT('Ctrl Pts',(-2.37188764610327,-1.95699282588048,
17.9014189075462));
#10839=CARTESIAN_POINT('Ctrl Pts',(-2.30831858452725,-2.02930223533265,
17.9064195385639));
#10840=CARTESIAN_POINT('Ctrl Pts',(-2.24483579656334,-2.10151350909133,
17.9114133829075));
#10841=CARTESIAN_POINT('Ctrl Pts',(-2.17787145089707,-2.17084519978337,
17.9164072272512));
#10842=CARTESIAN_POINT('Ctrl Pts',(-2.10771847124951,-2.23694548345587,
17.9214010715948));
#10843=CARTESIAN_POINT('Ctrl Pts',(-2.03763957282423,-2.30297596553431,
17.9263896424619));
#10844=CARTESIAN_POINT('Ctrl Pts',(-1.96437905187812,-2.36578152492138,
17.931378213329));
#10845=CARTESIAN_POINT('Ctrl Pts',(-1.88826837164119,-2.42504532053724,
17.9363667841961));
#10846=CARTESIAN_POINT('Ctrl Pts',(-1.81221234866321,-2.4842665571244,17.9413517726276));
#10847=CARTESIAN_POINT('Ctrl Pts',(-1.73331058057633,-2.53995081750557,
17.9463367610591));
#10848=CARTESIAN_POINT('Ctrl Pts',(-1.65192872920764,-2.59182054232511,
17.9513217494906));
#10849=CARTESIAN_POINT('Ctrl Pts',(-1.57057665405401,-2.64367128890743,
17.9563049140009));
#10850=CARTESIAN_POINT('Ctrl Pts',(-1.48674666820128,-2.69171003744208,
17.9612880785111));
#10851=CARTESIAN_POINT('Ctrl Pts',(-1.40083382973748,-2.73570225563072,
17.9662712430214));
#10852=CARTESIAN_POINT('Ctrl Pts',(-1.31492899828999,-2.77969037377547,
17.9712539431042));
#10853=CARTESIAN_POINT('Ctrl Pts',(-1.22694209079712,-2.81963251158411,
17.976236643187));
#10854=CARTESIAN_POINT('Ctrl Pts',(-1.13729225024013,-2.85534036281907,
17.9812193432699));
#10855=CARTESIAN_POINT('Ctrl Pts',(-1.0476263193209,-2.8910546229027,17.9862029376482));
#10856=CARTESIAN_POINT('Ctrl Pts',(-0.956297270211579,-2.92253292479704,
17.9911865320265));
#10857=CARTESIAN_POINT('Ctrl Pts',(-0.863742668553909,-2.94963571522305,
17.9961701264049));
#10858=CARTESIAN_POINT('Ctrl Pts',(-0.771088770415735,-2.97676758266578,
18.0011590673934));
#10859=CARTESIAN_POINT('Ctrl Pts',(-0.677207116561666,-2.99951444348679,
18.006148008382));
#10860=CARTESIAN_POINT('Ctrl Pts',(-0.582548608831353,-3.01778716418979,
18.0111369493706));
#10861=CARTESIAN_POINT('Ctrl Pts',(-0.487834422514082,-3.0360706329945,
18.0161288248781));
#10862=CARTESIAN_POINT('Ctrl Pts',(-0.392342906487234,-3.0498746586468,
18.0211207003856));
#10863=CARTESIAN_POINT('Ctrl Pts',(-0.296531179966286,-3.05916189655072,
18.0261125758932));
#10864=CARTESIAN_POINT('Ctrl Pts',(-0.200565204604544,-3.06846408612843,
18.0311124879014));
#10865=CARTESIAN_POINT('Ctrl Pts',(-0.104278427312059,-3.0732349463007,
18.0361123999097));
#10866=CARTESIAN_POINT('Ctrl Pts',(-0.00812900767658515,-3.07348924989729,
18.0411123119179));
#10867=CARTESIAN_POINT('Ctrl Pts',(0.0474735224485313,-3.07363631187066,
18.0440037257103));
#10868=CARTESIAN_POINT('Ctrl Pts',(0.103030173947787,-3.07227390587906,
18.0468951395027));
#10869=CARTESIAN_POINT('Ctrl Pts',(0.158453394787989,-3.06941277310175,
18.049786553295));
#10870=CARTESIAN_POINT('Ctrl Pts',(0.254312618482903,-3.06446419806834,
18.0547875019464));
#10871=CARTESIAN_POINT('Ctrl Pts',(0.350107281262537,-3.05501208153653,
18.0597884505978));
#10872=CARTESIAN_POINT('Ctrl Pts',(0.4453804778901,-3.0410587761361,18.0647893992492));
#10873=CARTESIAN_POINT('Ctrl Pts',(0.540524788304321,-3.02712434685991,
18.0697835825841));
#10874=CARTESIAN_POINT('Ctrl Pts',(0.635148604263144,-3.00870089391408,
18.0747777659189));
#10875=CARTESIAN_POINT('Ctrl Pts',(0.728797270700946,-2.9858427266383,18.0797719492538));
#10876=CARTESIAN_POINT('Ctrl Pts',(0.822347437359301,-2.96300860161023,
18.0847608797006));
#10877=CARTESIAN_POINT('Ctrl Pts',(0.914924069585438,-2.93574913850191,
18.0897498101474));
#10878=CARTESIAN_POINT('Ctrl Pts',(1.00608089271511,-2.90417001694349,18.0947387405942));
#10879=CARTESIAN_POINT('Ctrl Pts',(1.09717278551479,-2.87261338895948,18.0997241174629));
#10880=CARTESIAN_POINT('Ctrl Pts',(1.18684646638078,-2.83674336243439,18.1047094943315));
#10881=CARTESIAN_POINT('Ctrl Pts',(1.27467000622693,-2.79671568544703,18.1096948712001));
#10882=CARTESIAN_POINT('Ctrl Pts',(1.36246172633447,-2.75670251106593,18.1146784417946));
#10883=CARTESIAN_POINT('Ctrl Pts',(1.44840423857149,-2.71253486102905,18.1196620123891));
#10884=CARTESIAN_POINT('Ctrl Pts',(1.53208571652399,-2.66441656037925,18.1246455829836));
#10885=CARTESIAN_POINT('Ctrl Pts',(1.61575968197491,-2.6163025795481,18.1296287061782));
#10886=CARTESIAN_POINT('Ctrl Pts',(1.6971726365371,-2.56423887209535,18.1346118293728));
#10887=CARTESIAN_POINT('Ctrl Pts',(1.77593842944867,-2.50847462510733,18.1395949525674));
#10888=CARTESIAN_POINT('Ctrl Pts',(1.85471861763025,-2.45270018662168,18.1445789864798));
#10889=CARTESIAN_POINT('Ctrl Pts',(1.93085032532406,-2.39322411890687,18.1495630203921));
#10890=CARTESIAN_POINT('Ctrl Pts',(2.00397827758716,-2.33033759634925,18.1545470543045));
#10891=CARTESIAN_POINT('Ctrl Pts',(2.07718500189069,-2.26738333362465,18.1595364569234));
#10892=CARTESIAN_POINT('Ctrl Pts',(2.14738117805299,-2.2010115683744,18.1645258595424));
#10893=CARTESIAN_POINT('Ctrl Pts',(2.21424657112028,-2.1315521040505,18.1695152621613));
#10894=CARTESIAN_POINT('Ctrl Pts',(2.28115146719131,-2.06205160418707,18.1745076124395));
#10895=CARTESIAN_POINT('Ctrl Pts',(2.34472137306829,-1.98946010282752,18.1794999627176));
#10896=CARTESIAN_POINT('Ctrl Pts',(2.40467611751276,-1.91414080460758,18.1844923129958));
#10897=CARTESIAN_POINT('Ctrl Pts',(2.46472756467901,-1.83870002173771,18.1894927155784));
#10898=CARTESIAN_POINT('Ctrl Pts',(2.5211519506014,-1.76052301211704,18.1944931181611));
#10899=CARTESIAN_POINT('Ctrl Pts',(2.57371225948025,-1.68000221886791,18.1994935207438));
#10900=CARTESIAN_POINT('Ctrl Pts',(2.6040614331707,-1.63350820861306,18.2023808341889));
#10901=CARTESIAN_POINT('Ctrl Pts',(2.63312313152376,-1.58623323858147,18.205268147634));
#10902=CARTESIAN_POINT('Ctrl Pts',(2.6608588761498,-1.53825625017903,18.208155461079));
#10903=CARTESIAN_POINT('Ctrl Pts',(2.71072399288484,-1.45200011537753,18.2133464600564));
#10904=CARTESIAN_POINT('Ctrl Pts',(2.75646487212837,-1.36318966043797,18.2185374590337));
#10905=CARTESIAN_POINT('Ctrl Pts',(2.79782224151893,-1.27223934653115,18.2237284580111));
#10906=CARTESIAN_POINT('Ctrl Pts',(2.83910707630913,-1.1814485457841,18.2289103527576));
#10907=CARTESIAN_POINT('Ctrl Pts',(2.87602354093142,-1.08852570938133,18.2340922475042));
#10908=CARTESIAN_POINT('Ctrl Pts',(2.90835739213462,-0.993911228237162,
18.2392741422507));
#10909=CARTESIAN_POINT('Ctrl Pts',(2.94062389796345,-0.899493811389925,
18.2444452440782));
#10910=CARTESIAN_POINT('Ctrl Pts',(2.96832668061917,-0.803392138253361,
18.2496163459056));
#10911=CARTESIAN_POINT('Ctrl Pts',(2.99129936445153,-0.706066825613475,
18.254787447733));
#10912=CARTESIAN_POINT('Ctrl Pts',(3.01424339712983,-0.608862895505413,
18.2599521002471));
#10913=CARTESIAN_POINT('Ctrl Pts',(3.0324689794172,-0.510438741737216,18.2651167527612));
#10914=CARTESIAN_POINT('Ctrl Pts',(3.0458592447649,-0.411270848809141,18.2702814052753));
#10915=CARTESIAN_POINT('Ctrl Pts',(3.05923091965564,-0.312240636232969,
18.2754388874125));
#10916=CARTESIAN_POINT('Ctrl Pts',(3.06778059797625,-0.212469128371478,
18.2805963695496));
#10917=CARTESIAN_POINT('Ctrl Pts',(3.0714424736794,-0.112442789356175,18.2857538516868));
#10918=CARTESIAN_POINT('Ctrl Pts',(3.07282053680199,-0.0748001656682735,
18.2876947520654));
#10919=CARTESIAN_POINT('Ctrl Pts',(3.07350689903397,-0.0371215440459636,
18.289635652444));
#10920=CARTESIAN_POINT('Ctrl Pts',(3.07349994772178,0.000566881145854129,
18.2915765528226));
#10921=CARTESIAN_POINT('Ctrl Pts',(3.07349994772162,0.000566881991102313,
18.2915765528661));
#10922=CARTESIAN_POINT('Ctrl Pts',(3.07348108465619,0.102837956996753,18.2968433680007));
#10923=CARTESIAN_POINT('Ctrl Pts',(3.06835333742015,0.204987653606154,18.3021101831354));
#10924=CARTESIAN_POINT('Ctrl Pts',(3.05817840423343,0.306507908348619,18.30737699827));
#10925=CARTESIAN_POINT('Ctrl Pts',(3.04797107142034,0.408351429913868,18.3126605843101));
#10926=CARTESIAN_POINT('Ctrl Pts',(3.03268444834494,0.509561143595813,18.3179441703501));
#10927=CARTESIAN_POINT('Ctrl Pts',(3.01243181314503,0.609636630421547,18.3232277563902));
#10928=CARTESIAN_POINT('Ctrl Pts',(2.99214601482956,0.709875988017733,18.3285199941525));
#10929=CARTESIAN_POINT('Ctrl Pts',(2.96687806690077,0.808977066377082,18.3338122319149));
#10930=CARTESIAN_POINT('Ctrl Pts',(2.93679113505847,0.906454675668872,18.3391044696772));
#10931=CARTESIAN_POINT('Ctrl Pts',(2.90661691184847,1.0042150972421,18.3444120618357));
#10932=CARTESIAN_POINT('Ctrl Pts',(2.87159586571238,1.10034229232758,18.3497196539942));
#10933=CARTESIAN_POINT('Ctrl Pts',(2.83193989422544,1.19436957659444,18.3550272461528));
#10934=CARTESIAN_POINT('Ctrl Pts',(2.80330609589967,1.26226246116806,18.3588596203896));
#10935=CARTESIAN_POINT('Ctrl Pts',(2.77225681532059,1.32906099180651,18.3626919946264));
#10936=CARTESIAN_POINT('Ctrl Pts',(2.73888628269538,1.3945982147067,18.3665243688633));
#10937=CARTESIAN_POINT('Ctrl Pts',(2.69527008178349,1.48025716157833,18.3715333870459));
#10938=CARTESIAN_POINT('Ctrl Pts',(2.64755618379696,1.56401602255294,18.3765424052285));
#10939=CARTESIAN_POINT('Ctrl Pts',(2.59593365674044,1.64545759586876,18.3815514234111));
#10940=CARTESIAN_POINT('Ctrl Pts',(2.54438129710067,1.72678847051985,18.3865536331346));
#10941=CARTESIAN_POINT('Ctrl Pts',(2.48893110021215,1.8058079518594,18.3915558428581));
#10942=CARTESIAN_POINT('Ctrl Pts',(2.42981864846207,1.88212209635452,18.3965580525815));
#10943=CARTESIAN_POINT('Ctrl Pts',(2.37076890283357,1.95835528727927,18.401554955992));
#10944=CARTESIAN_POINT('Ctrl Pts',(2.30806489226961,2.03188850305573,18.4065518594025));
#10945=CARTESIAN_POINT('Ctrl Pts',(2.24198568692741,2.10235639928453,18.411548762813));
#10946=CARTESIAN_POINT('Ctrl Pts',(2.17595495448098,2.17277260326051,18.4165420007075));
#10947=CARTESIAN_POINT('Ctrl Pts',(2.10655424822711,2.24012764054148,18.4215352386021));
#10948=CARTESIAN_POINT('Ctrl Pts',(2.03410250820549,2.30408967623054,18.4265284764967));
#10949=CARTESIAN_POINT('Ctrl Pts',(1.96167802657922,2.36802764759131,18.4315198357938));
#10950=CARTESIAN_POINT('Ctrl Pts',(1.88620511956672,2.42857486500866,18.4365111950909));
#10951=CARTESIAN_POINT('Ctrl Pts',(1.80803845577153,2.4854374247708,18.4415025543881));
#10952=CARTESIAN_POINT('Ctrl Pts',(1.72988007684324,2.54229395768317,18.4464933846522));
#10953=CARTESIAN_POINT('Ctrl Pts',(1.64902886245486,2.59546635246374,18.4514842149163));
#10954=CARTESIAN_POINT('Ctrl Pts',(1.56587047797939,2.64470261016104,18.4564750451804));
#10955=CARTESIAN_POINT('Ctrl Pts',(1.48269843538775,2.69394695452971,18.4614666951494));
#10956=CARTESIAN_POINT('Ctrl Pts',(1.39721884635418,2.73925365523797,18.4664583451185));
#10957=CARTESIAN_POINT('Ctrl Pts',(1.30984319299196,2.78041598682151,18.4714499950875));
#10958=CARTESIAN_POINT('Ctrl Pts',(1.22237679015729,2.82162107012973,18.4764468294482));
#10959=CARTESIAN_POINT('Ctrl Pts',(1.13301078749947,2.85867300405083,18.4814436638088));
#10960=CARTESIAN_POINT('Ctrl Pts',(1.04217772116053,2.89141277708954,18.4864404981694));
#10961=CARTESIAN_POINT('Ctrl Pts',(0.951292770975532,2.92417125108609,18.4914401867218));
#10962=CARTESIAN_POINT('Ctrl Pts',(0.858939505900463,2.95261253015875,18.4964398752741));
#10963=CARTESIAN_POINT('Ctrl Pts',(0.765564742944816,2.97662776886191,18.5014395638265));
#10964=CARTESIAN_POINT('Ctrl Pts',(0.672043672190903,3.0006806367551,18.5064470863309));
#10965=CARTESIAN_POINT('Ctrl Pts',(0.577498335266228,3.02029352699308,18.5114546088354));
#10966=CARTESIAN_POINT('Ctrl Pts',(0.482384761461372,3.03540890028178,18.5164621313399));
#10967=CARTESIAN_POINT('Ctrl Pts',(0.429003982127228,3.0438921311583,18.5192725131091));
#10968=CARTESIAN_POINT('Ctrl Pts',(0.37544430968187,3.05095966618729,18.5220828948782));
#10969=CARTESIAN_POINT('Ctrl Pts',(0.321786553589066,3.05660852317226,18.5248932766474));
#10970=CARTESIAN_POINT('Ctrl Pts',(0.225641124389739,3.0667302990133,18.5299289952664));
#10971=CARTESIAN_POINT('Ctrl Pts',(0.128852929442827,3.0723286581662,18.5349647138855));
#10972=CARTESIAN_POINT('Ctrl Pts',(0.0318828348761874,3.073334627866,18.5400004325045));
#10973=CARTESIAN_POINT('Ctrl Pts',(-0.0643820208470067,3.07433328140395,
18.5449995276223));
#10974=CARTESIAN_POINT('Ctrl Pts',(-0.16082569776443,3.07080608065001,18.5499986227401));
#10975=CARTESIAN_POINT('Ctrl Pts',(-0.256989783873565,3.06273709302392,
18.5549977178579));
#10976=CARTESIAN_POINT('Ctrl Pts',(-0.353062715945296,3.05467575399961,
18.5599920743283));
#10977=CARTESIAN_POINT('Ctrl Pts',(-0.448856150415055,3.04208121920463,
18.5649864307986));
#10978=CARTESIAN_POINT('Ctrl Pts',(-0.543911997377421,3.02498958495875,
18.569980787269));
#10979=CARTESIAN_POINT('Ctrl Pts',(-0.638903467979729,3.00790952598399,
18.5749717613226));
#10980=CARTESIAN_POINT('Ctrl Pts',(-0.733157914833171,2.98633849890491,
18.5799627353762));
#10981=CARTESIAN_POINT('Ctrl Pts',(-0.826223737422982,2.96036426571441,
18.5849537094297));
#10982=CARTESIAN_POINT('Ctrl Pts',(-0.92069603634875,2.93399749159631,18.5900201106026));
#10983=CARTESIAN_POINT('Ctrl Pts',(-1.01394303112386,2.90309338515365,18.5950865117754));
#10984=CARTESIAN_POINT('Ctrl Pts',(-1.1055050498395,2.86779720949361,18.6001529129483));
#10985=CARTESIAN_POINT('Ctrl Pts',(-1.19567576894536,2.83303736490308,18.60514232934));
#10986=CARTESIAN_POINT('Ctrl Pts',(-1.28421195811642,2.79401819649673,18.6101317457316));
#10987=CARTESIAN_POINT('Ctrl Pts',(-1.37069309330137,2.75092760609507,18.6151211621233));
#10988=CARTESIAN_POINT('Ctrl Pts',(-1.45917578460393,2.70683970877039,18.6202260556867));
#10989=CARTESIAN_POINT('Ctrl Pts',(-1.54550667851344,2.65848978448217,18.6253309492502));
#10990=CARTESIAN_POINT('Ctrl Pts',(-1.62926181217111,2.60612896791408,18.6304358428136));
#10991=CARTESIAN_POINT('Ctrl Pts',(-1.71301694582878,2.55376815134599,18.635540736377));
#10992=CARTESIAN_POINT('Ctrl Pts',(-1.79419592504642,2.49739673258324,18.6406456299405));
#10993=CARTESIAN_POINT('Ctrl Pts',(-1.87240768645124,2.43731239395329,18.6457505235039));
#10994=CARTESIAN_POINT('',(3.07396038371946,0.000496328078016796,18.2084233953208));
#10995=CARTESIAN_POINT('Ctrl Pts',(3.07349995977581,0.000497250552599549,
18.2084234471775));
#10996=CARTESIAN_POINT('Ctrl Pts',(3.07349581818499,0.0260963758433496,
18.2097570965117));
#10997=CARTESIAN_POINT('Ctrl Pts',(3.07317186094799,0.0516926665754111,
18.2110907458459));
#10998=CARTESIAN_POINT('Ctrl Pts',(3.07252826222747,0.0772808372976627,
18.2124243951801));
#10999=CARTESIAN_POINT('Ctrl Pts',(3.07011503473139,0.173225834067707,18.21742502545));
#11000=CARTESIAN_POINT('Ctrl Pts',(3.06319919775923,0.269225925428171,18.2224256557198));
#11001=CARTESIAN_POINT('Ctrl Pts',(3.05177086479431,0.364824394459287,18.2274262859897));
#11002=CARTESIAN_POINT('Ctrl Pts',(3.04035804193262,0.460293120847487,18.2324201295924));
#11003=CARTESIAN_POINT('Ctrl Pts',(3.02444494626311,0.555360876268122,18.2374139731951));
#11004=CARTESIAN_POINT('Ctrl Pts',(3.00407368908106,0.64957179785678,18.2424078167978));
#11005=CARTESIAN_POINT('Ctrl Pts',(2.9837239438239,0.743683233279711,18.2473963869318));
#11006=CARTESIAN_POINT('Ctrl Pts',(2.95892548819042,0.836939207032645,18.2523849570657));
#11007=CARTESIAN_POINT('Ctrl Pts',(2.92977200971182,0.928890855326471,18.2573735271997));
#11008=CARTESIAN_POINT('Ctrl Pts',(2.90063946710002,1.02077647076384,18.2623585149124));
#11009=CARTESIAN_POINT('Ctrl Pts',(2.86715825122914,1.11135920580007,18.2673435026252));
#11010=CARTESIAN_POINT('Ctrl Pts',(2.82947248356031,1.2002031972858,18.2723284903379));
#11011=CARTESIAN_POINT('Ctrl Pts',(2.79180050439657,1.28901468244607,18.2773116541385));
#11012=CARTESIAN_POINT('Ctrl Pts',(2.74992720120223,1.37608828457834,18.2822948179391));
#11013=CARTESIAN_POINT('Ctrl Pts',(2.70404529326473,1.46100694795502,18.2872779817398));
#11014=CARTESIAN_POINT('Ctrl Pts',(2.6581676613985,1.54591769713911,18.2922606811228));
#11015=CARTESIAN_POINT('Ctrl Pts',(2.60828237629102,1.6286735209441,18.2972433805059));
#11016=CARTESIAN_POINT('Ctrl Pts',(2.55462818999486,1.7088818159497,18.3022260798889));
#11017=CARTESIAN_POINT('Ctrl Pts',(2.50096437372331,1.78910450692254,18.3072096735782));
#11018=CARTESIAN_POINT('Ctrl Pts',(2.44353055681198,1.86677839636644,18.3121932672675));
#11019=CARTESIAN_POINT('Ctrl Pts',(2.38260828915974,1.94154062291452,18.3171768609568));
#11020=CARTESIAN_POINT('Ctrl Pts',(2.32162066127232,2.01638305784778,18.3221658012766));
#11021=CARTESIAN_POINT('Ctrl Pts',(2.25713738853279,2.08830725285345,18.3271547415964));
#11022=CARTESIAN_POINT('Ctrl Pts',(2.18947957108095,2.15698434343395,18.3321436819162));
#11023=CARTESIAN_POINT('Ctrl Pts',(2.12178195683039,2.22570183035671,18.3371355567654));
#11024=CARTESIAN_POINT('Ctrl Pts',(2.05090640186082,2.291168112132,18.3421274316146));
#11025=CARTESIAN_POINT('Ctrl Pts',(1.97720846543889,2.35309348182277,18.3471193064637));
#11026=CARTESIAN_POINT('Ctrl Pts',(1.90339188117032,2.41511854645919,18.3521192178365));
#11027=CARTESIAN_POINT('Ctrl Pts',(1.82674419102255,2.47359105018672,18.3571191292092));
#11028=CARTESIAN_POINT('Ctrl Pts',(1.74765133310118,2.52826364683545,18.362119040582));
#11029=CARTESIAN_POINT('Ctrl Pts',(1.7019123755448,2.5598805038227,18.3650104613761));
#11030=CARTESIAN_POINT('Ctrl Pts',(1.65535619738727,2.59022741164452,18.3679018821703));
#11031=CARTESIAN_POINT('Ctrl Pts',(1.60806103526927,2.61926362874162,18.3707933029644));
#11032=CARTESIAN_POINT('Ctrl Pts',(1.52626023406071,2.66948411041971,18.3757942486638));
#11033=CARTESIAN_POINT('Ctrl Pts',(1.44196164653047,2.71595665020612,18.3807951943631));
#11034=CARTESIAN_POINT('Ctrl Pts',(1.355543141196,2.75842437676955,18.3857961400624));
#11035=CARTESIAN_POINT('Ctrl Pts',(1.26924154378735,2.80083465251492,18.3907903204262));
#11036=CARTESIAN_POINT('Ctrl Pts',(1.18082611868765,2.83925069083241,18.39578450079));
#11037=CARTESIAN_POINT('Ctrl Pts',(1.09070231052193,2.87345971258031,18.4007786811537));
#11038=CARTESIAN_POINT('Ctrl Pts',(1.00067329500927,2.9076327531153,18.4057676086146));
#11039=CARTESIAN_POINT('Ctrl Pts',(0.908939876541152,2.9376074189381,18.4107565360755));
#11040=CARTESIAN_POINT('Ctrl Pts',(0.815929691739153,2.96321801225263,18.4157454635365));
#11041=CARTESIAN_POINT('Ctrl Pts',(0.722985757623182,2.98881036327058,18.4207308374095));
#11042=CARTESIAN_POINT('Ctrl Pts',(0.628767286827081,3.01004470529546,18.4257162112825));
#11043=CARTESIAN_POINT('Ctrl Pts',(0.533718454632727,3.02680472795727,18.4307015851556));
#11044=CARTESIAN_POINT('Ctrl Pts',(0.438704060118033,3.04355867820052,18.4356851527496));
#11045=CARTESIAN_POINT('Ctrl Pts',(0.342860333539901,3.05584145402598,18.4406687203437));
#11046=CARTESIAN_POINT('Ctrl Pts',(0.246642116342153,3.06358775236589,18.4456522879377));
#11047=CARTESIAN_POINT('Ctrl Pts',(0.150432537159386,3.07133335527989,18.4506354081307));
#11048=CARTESIAN_POINT('Ctrl Pts',(0.0538489714644777,3.07454325542527,
18.4556185283237));
#11049=CARTESIAN_POINT('Ctrl Pts',(-0.0426492036916367,3.07320407643626,
18.4606016485167));
#11050=CARTESIAN_POINT('Ctrl Pts',(-0.139165014954978,3.0718646526975,18.4655856794299));
#11051=CARTESIAN_POINT('Ctrl Pts',(-0.235594966070892,3.06597450475753,
18.4705697103432));
#11052=CARTESIAN_POINT('Ctrl Pts',(-0.331481341451637,3.05557234741209,
18.4755537412564));
#11053=CARTESIAN_POINT('Ctrl Pts',(-0.427471004300964,3.04515898500758,
18.4805431408984));
#11054=CARTESIAN_POINT('Ctrl Pts',(-0.522915485626964,3.03022395747985,
18.4855325405403));
#11055=CARTESIAN_POINT('Ctrl Pts',(-0.617364065253234,3.01085766201825,
18.4905219401823));
#11056=CARTESIAN_POINT('Ctrl Pts',(-0.711868443774845,2.99147992522108,
18.4955142874915));
#11057=CARTESIAN_POINT('Ctrl Pts',(-0.805375324145514,2.96766581587002,
18.5005066348007));
#11058=CARTESIAN_POINT('Ctrl Pts',(-0.89744808296427,2.93955595088506,18.50549898211));
#11059=CARTESIAN_POINT('Ctrl Pts',(-0.989669349432891,2.91140074643117,
18.5104993817658));
#11060=CARTESIAN_POINT('Ctrl Pts',(-1.08045146271283,2.87893609864151,18.5154997814216));
#11061=CARTESIAN_POINT('Ctrl Pts',(-1.16937680199829,2.84235116495978,18.5205001810775));
#11062=CARTESIAN_POINT('Ctrl Pts',(-1.2207242928934,2.82122620143178,18.5233875243012));
#11063=CARTESIAN_POINT('Ctrl Pts',(-1.27145312842869,2.79872833948767,18.5262748675248));
#11064=CARTESIAN_POINT('Ctrl Pts',(-1.32148688040794,2.77490084055443,18.5291622107485));
#11065=CARTESIAN_POINT('Ctrl Pts',(-1.40800849234638,2.7336967826013,18.5341551920871));
#11066=CARTESIAN_POINT('Ctrl Pts',(-1.49275570937198,2.68836859676869,18.5391481734257));
#11067=CARTESIAN_POINT('Ctrl Pts',(-1.5753080589408,2.63909203504466,18.5441411547643));
#11068=CARTESIAN_POINT('Ctrl Pts',(-1.65773786070718,2.5898886236838,18.5491267240923));
#11069=CARTESIAN_POINT('Ctrl Pts',(-1.73797889834575,2.53674871403438,18.5541122934203));
#11070=CARTESIAN_POINT('Ctrl Pts',(-1.81563271272675,2.47989517973573,18.5590978627483));
#11071=CARTESIAN_POINT('Ctrl Pts',(-1.83471573057289,2.465923721691,18.5603230402778));
#11072=CARTESIAN_POINT('Ctrl Pts',(-1.85364261641151,2.45172821585054,18.5615482178073));
#11073=CARTESIAN_POINT('Ctrl Pts',(-1.87240768645123,2.4373123939533,18.5627733953368));
#11074=CARTESIAN_POINT('Ctrl Pts',(-1.8746299318936,2.44024828799233,17.5625875311804));
#11075=CARTESIAN_POINT('Ctrl Pts',(-1.95834209400996,2.37692452213389,17.5680412754681));
#11076=CARTESIAN_POINT('Ctrl Pts',(-2.81517875351248,1.65341120062326,17.6262846556839));
#11077=CARTESIAN_POINT('Ctrl Pts',(-3.56999562230916,-0.655354264402703,
17.7373176718277));
#11078=CARTESIAN_POINT('Ctrl Pts',(-1.39399312869632,-3.35125860275677,
17.8956865796119));
#11079=CARTESIAN_POINT('Ctrl Pts',(2.02304254293428,-2.99694469112536,18.0527216541862));
#11080=CARTESIAN_POINT('Ctrl Pts',(3.07627241680049,-0.988770447851309,
18.1569670928325));
#11081=CARTESIAN_POINT('Ctrl Pts',(3.0783977291544,0.000487437709835295,
18.2084228955508));
#11082=CARTESIAN_POINT('Origin',(0.,0.,-2.20842344717744));
#11083=CARTESIAN_POINT('',(-1.86972588535603,2.43378780274861,16.5626129315945));
#11084=CARTESIAN_POINT('',(-1.87240768645125,2.43731239395329,16.6459160952886));
#11085=CARTESIAN_POINT('',(-1.87240768645123,2.4373123939533,-2.20842344717744));
#11086=CARTESIAN_POINT('',(3.07349878900434,-0.00272836743798955,17.2915765528552));
#11087=CARTESIAN_POINT('Ctrl Pts',(-1.87240768645125,2.43731239395329,16.6459160952886));
#11088=CARTESIAN_POINT('Ctrl Pts',(-1.94869008435301,2.3787102432702,16.650906378381));
#11089=CARTESIAN_POINT('Ctrl Pts',(-2.02231571227431,2.31644890824351,16.6558966614733));
#11090=CARTESIAN_POINT('Ctrl Pts',(-2.09291629670881,2.25080066309095,16.6608869445657));
#11091=CARTESIAN_POINT('Ctrl Pts',(-2.16480287083741,2.18395663510773,16.665968125668));
#11092=CARTESIAN_POINT('Ctrl Pts',(-2.23355271443631,2.11360133218143,16.6710493067703));
#11093=CARTESIAN_POINT('Ctrl Pts',(-2.29881105051213,2.04006617638824,16.6761304878727));
#11094=CARTESIAN_POINT('Ctrl Pts',(-2.36280734971843,1.96795312363041,16.6811134035536));
#11095=CARTESIAN_POINT('Ctrl Pts',(-2.42344567718209,1.89278245461709,16.6860963192346));
#11096=CARTESIAN_POINT('Ctrl Pts',(-2.4804285996563,1.81490391261,16.6910792349156));
#11097=CARTESIAN_POINT('Ctrl Pts',(-2.53739776626703,1.73704417073715,16.6960609477044));
#11098=CARTESIAN_POINT('Ctrl Pts',(-2.59071302240877,1.65647820902671,16.7010426604933));
#11099=CARTESIAN_POINT('Ctrl Pts',(-2.64011835287779,1.57358740869322,16.7060243732821));
#11100=CARTESIAN_POINT('Ctrl Pts',(-2.68952524410106,1.4906939897725,16.7110062434473));
#11101=CARTESIAN_POINT('Ctrl Pts',(-2.7350217401748,1.40547596383643,16.7159881136125));
#11102=CARTESIAN_POINT('Ctrl Pts',(-2.77639671341757,1.31834120762575,16.7209699837777));
#11103=CARTESIAN_POINT('Ctrl Pts',(-2.81921322186053,1.22817061094453,16.726125426048));
#11104=CARTESIAN_POINT('Ctrl Pts',(-2.8576155186533,1.13594772403954,16.7312808683183));
#11105=CARTESIAN_POINT('Ctrl Pts',(-2.8914236036249,1.04214768358462,16.7364363105887));
#11106=CARTESIAN_POINT('Ctrl Pts',(-2.92414138435231,0.951372676410906,
16.7414254908364));
#11107=CARTESIAN_POINT('Ctrl Pts',(-2.95255666769649,0.859121130163589,
16.7464146710841));
#11108=CARTESIAN_POINT('Ctrl Pts',(-2.97655742563126,0.765838195651939,
16.7514038513318));
#11109=CARTESIAN_POINT('Ctrl Pts',(-3.00175790406929,0.6678923480172,16.7566424246134));
#11110=CARTESIAN_POINT('Ctrl Pts',(-3.02209094743006,0.56880986948559,16.761880997895));
#11111=CARTESIAN_POINT('Ctrl Pts',(-3.03748798446673,0.469115118302798,
16.7671195711767));
#11112=CARTESIAN_POINT('Ctrl Pts',(-3.0528850215034,0.369420367120006,16.7723581444583));
#11113=CARTESIAN_POINT('Ctrl Pts',(-3.06334606838429,0.269113900212103,
16.7775967177399));
#11114=CARTESIAN_POINT('Ctrl Pts',(-3.0688654966124,0.168721112199794,16.7828352910216));
#11115=CARTESIAN_POINT('Ctrl Pts',(-3.07413302261529,0.0729101695618671,
16.7878347800698));
#11116=CARTESIAN_POINT('Ctrl Pts',(-3.07491862900344,-0.02331598262082,
16.7928342691181));
#11117=CARTESIAN_POINT('Ctrl Pts',(-3.07117587759827,-0.119503049578297,
16.7978337581663));
#11118=CARTESIAN_POINT('Ctrl Pts',(-3.06743820323802,-0.215559638711458,
16.8028264654041));
#11119=CARTESIAN_POINT('Ctrl Pts',(-3.05918439625417,-0.311576813109383,
16.8078191726419));
#11120=CARTESIAN_POINT('Ctrl Pts',(-3.04641991747264,-0.407096961946395,
16.8128118798798));
#11121=CARTESIAN_POINT('Ctrl Pts',(-3.03366890489975,-0.502516339394628,
16.8177993199352));
#11122=CARTESIAN_POINT('Ctrl Pts',(-3.01641673826346,-0.597439300872269,
16.8227867599907));
#11123=CARTESIAN_POINT('Ctrl Pts',(-2.99472084953958,-0.69141108129167,
16.8277742000462));
#11124=CARTESIAN_POINT('Ctrl Pts',(-2.97304048430665,-0.785315624544578,
16.8327580715693));
#11125=CARTESIAN_POINT('Ctrl Pts',(-2.9469228161462,-0.878269913198738,
16.8377419430925));
#11126=CARTESIAN_POINT('Ctrl Pts',(-2.91647659018144,-0.9698281027706,16.8427258146156));
#11127=CARTESIAN_POINT('Ctrl Pts',(-2.8860414515551,-1.06135295038955,16.8477078712054));
#11128=CARTESIAN_POINT('Ctrl Pts',(-2.85128102541957,-1.15148229295804,
16.8526899277952));
#11129=CARTESIAN_POINT('Ctrl Pts',(-2.812354003565,-1.23978514615714,16.857671984385));
#11130=CARTESIAN_POINT('Ctrl Pts',(-2.77343053018542,-1.32807994992298,
16.8626535868249));
#11131=CARTESIAN_POINT('Ctrl Pts',(-2.73034139346628,-1.41454819375258,
16.8676351892648));
#11132=CARTESIAN_POINT('Ctrl Pts',(-2.68329312531964,-1.49877958806903,
16.8726167917047));
#11133=CARTESIAN_POINT('Ctrl Pts',(-2.63623630175471,-1.58302629931083,
16.8775993000163));
#11134=CARTESIAN_POINT('Ctrl Pts',(-2.58521913104524,-1.66503497000622,
16.8825818083278));
#11135=CARTESIAN_POINT('Ctrl Pts',(-2.53049318192716,-1.74442153914131,
16.8875643166394));
#11136=CARTESIAN_POINT('Ctrl Pts',(-2.47570824264697,-1.82389368059919,
16.8925521956933));
#11137=CARTESIAN_POINT('Ctrl Pts',(-2.41720679334826,-1.90073771581067,
16.8975400747472));
#11138=CARTESIAN_POINT('Ctrl Pts',(-2.35528254233724,-1.97460031291435,
16.9025279538011));
#11139=CARTESIAN_POINT('Ctrl Pts',(-2.29332170985965,-2.04850654400765,
16.9075187794217));
#11140=CARTESIAN_POINT('Ctrl Pts',(-2.22793434694105,-2.11942750743609,
16.9125096050422));
#11141=CARTESIAN_POINT('Ctrl Pts',(-2.15945163440285,-2.18704615604584,
16.9175004306627));
#11142=CARTESIAN_POINT('Ctrl Pts',(-2.09085824583123,-2.25477408426114,
16.9224993220383));
#11143=CARTESIAN_POINT('Ctrl Pts',(-2.01915984518205,-2.31918874783033,
16.9274982134139));
#11144=CARTESIAN_POINT('Ctrl Pts',(-1.94472127489543,-2.3800129018493,16.9324971047894));
#11145=CARTESIAN_POINT('Ctrl Pts',(-1.90150211680463,-2.41532750714279,
16.9353994694615));
#11146=CARTESIAN_POINT('Ctrl Pts',(-1.857359822824,-2.44943255052934,16.9383018341336));
#11147=CARTESIAN_POINT('Ctrl Pts',(-1.81237000627372,-2.48228064697757,
16.9412041988057));
#11148=CARTESIAN_POINT('Ctrl Pts',(-1.73487197768212,-2.5388637342831,16.946203719977));
#11149=CARTESIAN_POINT('Ctrl Pts',(-1.65458546237634,-2.59191343652079,
16.9512032411484));
#11150=CARTESIAN_POINT('Ctrl Pts',(-1.57186624083407,-2.64114345898253,
16.9562027623198));
#11151=CARTESIAN_POINT('Ctrl Pts',(-1.48925922945181,-2.69030670000465,
16.9611955015478));
#11152=CARTESIAN_POINT('Ctrl Pts',(-1.40422644437154,-2.73566033649841,
16.9661882407759));
#11153=CARTESIAN_POINT('Ctrl Pts',(-1.31715470384538,-2.77695980095823,
16.971180980004));
#11154=CARTESIAN_POINT('Ctrl Pts',(-1.23017482427609,-2.8182156943547,16.9761684518766));
#11155=CARTESIAN_POINT('Ctrl Pts',(-1.14116066002593,-2.85542573134479,
16.9811559237493));
#11156=CARTESIAN_POINT('Ctrl Pts',(-1.05052493798665,-2.88839048687468,
16.986143395622));
#11157=CARTESIAN_POINT('Ctrl Pts',(-0.959954072733928,-2.92133165360244,
16.9911272985773));
#11158=CARTESIAN_POINT('Ctrl Pts',(-0.86776436775069,-2.95003342831423,
16.9961112015327));
#11159=CARTESIAN_POINT('Ctrl Pts',(-0.774389004784814,-2.97434428391677,
17.001095104488));
#11160=CARTESIAN_POINT('Ctrl Pts',(-0.681047649964934,-2.99864628528732,
17.0060771922611));
#11161=CARTESIAN_POINT('Ctrl Pts',(-0.586521919521054,-3.01856043452411,
17.0110592800342));
#11162=CARTESIAN_POINT('Ctrl Pts',(-0.491259724133798,-3.03398519005021,
17.0160413678073));
#11163=CARTESIAN_POINT('Ctrl Pts',(-0.396006217970347,-3.04940853862623,
17.0210230011454));
#11164=CARTESIAN_POINT('Ctrl Pts',(-0.300016813767278,-3.06034323766132,
17.0260046344836));
#11165=CARTESIAN_POINT('Ctrl Pts',(-0.203748110307505,-3.06673914077251,
17.0309862678217));
#11166=CARTESIAN_POINT('Ctrl Pts',(-0.107461907339179,-3.0731362065166,
17.0359688067099));
#11167=CARTESIAN_POINT('Ctrl Pts',(-0.0108967422766421,-3.07499280871843,
17.0409513455981));
#11168=CARTESIAN_POINT('Ctrl Pts',(0.0854882658993729,-3.0723108577085,
17.0459338844863));
#11169=CARTESIAN_POINT('Ctrl Pts',(0.181977155694252,-3.06962601615139,
17.0509217934442));
#11170=CARTESIAN_POINT('Ctrl Pts',(0.2782850614439,-3.06239286808041,17.0559097024021));
#11171=CARTESIAN_POINT('Ctrl Pts',(0.373955696445788,-3.05066540071109,
17.0608976113599));
#11172=CARTESIAN_POINT('Ctrl Pts',(0.469682841667079,-3.03893100622402,
17.0658884665492));
#11173=CARTESIAN_POINT('Ctrl Pts',(0.564771534129519,-3.02269708037209,
17.0708793217385));
#11174=CARTESIAN_POINT('Ctrl Pts',(0.658775520175408,-3.00206879734919,
17.0758701769277));
#11175=CARTESIAN_POINT('Ctrl Pts',(0.752931411299467,-2.98140718019785,
17.0808690970542));
#11176=CARTESIAN_POINT('Ctrl Pts',(0.845998672439075,-2.95633714078435,
17.0858680171808));
#11177=CARTESIAN_POINT('Ctrl Pts',(0.937546108359654,-2.92701375888459,
17.0908669373073));
#11178=CARTESIAN_POINT('Ctrl Pts',(0.990692751657682,-2.90999046049892,
17.0937689937348));
#11179=CARTESIAN_POINT('Ctrl Pts',(1.04332753340845,-2.89153459877591,17.0966710501624));
#11180=CARTESIAN_POINT('Ctrl Pts',(1.09536956551501,-2.87168378568105,17.0995731065899));
#11181=CARTESIAN_POINT('Ctrl Pts',(1.18502573068125,-2.83748550968229,17.1045726663661));
#11182=CARTESIAN_POINT('Ctrl Pts',(1.27323626739536,-2.79902445047461,17.1095722261422));
#11183=CARTESIAN_POINT('Ctrl Pts',(1.35956732428756,-2.75644316842005,17.1145717859184));
#11184=CARTESIAN_POINT('Ctrl Pts',(1.44578128034576,-2.71391964430129,17.1195645642113));
#11185=CARTESIAN_POINT('Ctrl Pts',(1.53012043295859,-2.66728719709655,17.1245573425042));
#11186=CARTESIAN_POINT('Ctrl Pts',(1.61216903342187,-2.61673713958349,17.129550120797));
#11187=CARTESIAN_POINT('Ctrl Pts',(1.69413107963522,-2.5662404080539,17.1345376321362));
#11188=CARTESIAN_POINT('Ctrl Pts',(1.77380700550127,-2.5118345108883,17.1395251434754));
#11189=CARTESIAN_POINT('Ctrl Pts',(1.8508048220962,-2.45375707039337,17.1445126548146));
#11190=CARTESIAN_POINT('Ctrl Pts',(1.92774754795333,-2.39572118340201,17.1494965976671));
#11191=CARTESIAN_POINT('Ctrl Pts',(2.00201562431126,-2.33401923887228,17.1544805405196));
#11192=CARTESIAN_POINT('Ctrl Pts',(2.07324610249455,-2.26893209428823,17.1594644833722));
#11193=CARTESIAN_POINT('Ctrl Pts',(2.1444506416915,-2.20386865156042,17.1644466112934));
#11194=CARTESIAN_POINT('Ctrl Pts',(2.21261945681859,-2.13542275389542,17.1694287392146));
#11195=CARTESIAN_POINT('Ctrl Pts',(2.27742350786363,-2.06391482765887,17.1744108671358));
#11196=CARTESIAN_POINT('Ctrl Pts',(2.34222165054095,-1.99241342100119,17.1793925408224));
#11197=CARTESIAN_POINT('Ctrl Pts',(2.40365534443321,-1.91785086620241,17.184374214509));
#11198=CARTESIAN_POINT('Ctrl Pts',(2.46143392943952,-1.84058285904328,17.1893558881956));
#11199=CARTESIAN_POINT('Ctrl Pts',(2.51922301896186,-1.76330080406661,17.1943384675824));
#11200=CARTESIAN_POINT('Ctrl Pts',(2.57335541701767,-1.68331267143298,17.1993210469691));
#11201=CARTESIAN_POINT('Ctrl Pts',(2.62358275631767,-1.60100461297042,17.2043036263558));
#11202=CARTESIAN_POINT('Ctrl Pts',(2.6738642288716,-1.51860784578685,17.2092915757907));
#11203=CARTESIAN_POINT('Ctrl Pts',(2.72023201128706,-1.43388653640455,17.2142795252257));
#11204=CARTESIAN_POINT('Ctrl Pts',(2.76248296010173,-1.34725281411753,17.2192674746606));
#11205=CARTESIAN_POINT('Ctrl Pts',(2.80475886568258,-1.26056791907319,17.2242583703747));
#11206=CARTESIAN_POINT('Ctrl Pts',(2.84291292215504,-1.17196876482895,17.2292492660888));
#11207=CARTESIAN_POINT('Ctrl Pts',(2.87679038382587,-1.08188693379992,17.2342401618028));
#11208=CARTESIAN_POINT('Ctrl Pts',(2.91072258686855,-0.9916595427801,17.2392391221258));
#11209=CARTESIAN_POINT('Ctrl Pts',(2.94036426167294,-0.899945108481694,
17.2442380824487));
#11210=CARTESIAN_POINT('Ctrl Pts',(2.96561072154697,-0.807189753555912,
17.2492370427717));
#11211=CARTESIAN_POINT('Ctrl Pts',(2.98026508312541,-0.753349709597235,
17.2521386999725));
#11212=CARTESIAN_POINT('Ctrl Pts',(2.99343954445976,-0.699159152140327,
17.2550403571733));
#11213=CARTESIAN_POINT('Ctrl Pts',(3.00512161925494,-0.644706369975154,
17.2579420143741));
#11214=CARTESIAN_POINT('Ctrl Pts',(3.03303837637569,-0.514580076409504,
17.2648761301663));
#11215=CARTESIAN_POINT('Ctrl Pts',(3.05251132490793,-0.382583461353266,
17.2718102459585));
#11216=CARTESIAN_POINT('Ctrl Pts',(3.06334550588529,-0.249632853551782,
17.2787443617507));
#11217=CARTESIAN_POINT('Ctrl Pts',(3.07002870744382,-0.167620589669179,
17.2830217587747));
#11218=CARTESIAN_POINT('Ctrl Pts',(3.073425537775,-0.0852456668693086,17.2872991557986));
#11219=CARTESIAN_POINT('Ctrl Pts',(3.07349878900378,-0.0027283680658539,
17.2915765528226));
#11220=CARTESIAN_POINT('Ctrl Pts',(3.07349878900434,-0.00272836743798955,
17.2915765528551));
#11221=CARTESIAN_POINT('Ctrl Pts',(3.07358305061729,0.0921921193577995,
17.2964968860897));
#11222=CARTESIAN_POINT('Ctrl Pts',(3.06926587962942,0.187247177514582,17.3014172193243));
#11223=CARTESIAN_POINT('Ctrl Pts',(3.06053658859495,0.281989432198457,17.3063375525589));
#11224=CARTESIAN_POINT('Ctrl Pts',(3.05181483583495,0.376649871174996,17.311253636786));
#11225=CARTESIAN_POINT('Ctrl Pts',(3.03868857510245,0.470997594766093,17.3161697210132));
#11226=CARTESIAN_POINT('Ctrl Pts',(3.02119917645395,0.564586385058986,17.3210858052403));
#11227=CARTESIAN_POINT('Ctrl Pts',(3.00371759034355,0.658133369112316,17.325999693446));
#11228=CARTESIAN_POINT('Ctrl Pts',(2.9818768187115,0.7509216489512,17.3309135816516));
#11229=CARTESIAN_POINT('Ctrl Pts',(2.95576980972152,0.842512363077729,17.3358274698573));
#11230=CARTESIAN_POINT('Ctrl Pts',(2.92966686320602,0.934088824903684,17.3407405934198));
#11231=CARTESIAN_POINT('Ctrl Pts',(2.89929912243473,1.02446765630521,17.3456537169823));
#11232=CARTESIAN_POINT('Ctrl Pts',(2.8648098432871,1.11322361266969,17.3505668405448));
#11233=CARTESIAN_POINT('Ctrl Pts',(2.8303158911327,1.2019915947185,17.3554806297942));
#11234=CARTESIAN_POINT('Ctrl Pts',(2.79169945727649,1.28913584410698,17.3603944190435));
#11235=CARTESIAN_POINT('Ctrl Pts',(2.74915205689293,1.37425078427534,17.3653082082929));
#11236=CARTESIAN_POINT('Ctrl Pts',(2.70656102219928,1.45945301371776,17.3702270368584));
#11237=CARTESIAN_POINT('Ctrl Pts',(2.66003117857506,1.54262137562882,17.375145865424));
#11238=CARTESIAN_POINT('Ctrl Pts',(2.60979994620126,1.62337503085637,17.3800646939895));
#11239=CARTESIAN_POINT('Ctrl Pts',(2.55953947560667,1.70417569056875,17.3849863856701));
#11240=CARTESIAN_POINT('Ctrl Pts',(2.50557358689705,1.78255847568588,17.3899080773507));
#11241=CARTESIAN_POINT('Ctrl Pts',(2.44818165604469,1.85817351961713,17.3948297690312));
#11242=CARTESIAN_POINT('Ctrl Pts',(2.39070006538224,1.93390669218384,17.3997591495617));
#11243=CARTESIAN_POINT('Ctrl Pts',(2.32978204222512,2.00686314975054,17.4046885300922));
#11244=CARTESIAN_POINT('Ctrl Pts',(2.26574540435209,2.07672819903265,17.4096179106226));
#11245=CARTESIAN_POINT('Ctrl Pts',(2.23676286091777,2.10834864152643,17.4118489144678));
#11246=CARTESIAN_POINT('Ctrl Pts',(2.20714197249847,2.13933636676563,17.414079918313));
#11247=CARTESIAN_POINT('Ctrl Pts',(2.17691441210261,2.16966492629161,17.4163109221582));
#11248=CARTESIAN_POINT('Ctrl Pts',(2.10917509258733,2.2376305827079,17.421310554293));
#11249=CARTESIAN_POINT('Ctrl Pts',(2.03813081623026,2.30254021499092,17.4263101864277));
#11250=CARTESIAN_POINT('Ctrl Pts',(1.96408843828732,2.36405559507091,17.4313098185624));
#11251=CARTESIAN_POINT('Ctrl Pts',(1.89014650846582,2.42548752153231,17.4363026680455));
#11252=CARTESIAN_POINT('Ctrl Pts',(1.81321489532017,2.48353406932517,17.4412955175286));
#11253=CARTESIAN_POINT('Ctrl Pts',(1.73363761247245,2.53789339386445,17.4462883670117));
#11254=CARTESIAN_POINT('Ctrl Pts',(1.65414429548935,2.59219536123443,17.4512759482963));
#11255=CARTESIAN_POINT('Ctrl Pts',(1.57201121881274,2.6428175933025,17.4562635295809));
#11256=CARTESIAN_POINT('Ctrl Pts',(1.48761502005967,2.68949880128117,17.4612511108654));
#11257=CARTESIAN_POINT('Ctrl Pts',(1.40327924050138,2.73614659020735,17.4662351215432));
#11258=CARTESIAN_POINT('Ctrl Pts',(1.31668394268969,2.77885875197917,17.4712191322209));
#11259=CARTESIAN_POINT('Ctrl Pts',(1.22823343028284,2.81741812493915,17.4762031428986));
#11260=CARTESIAN_POINT('Ctrl Pts',(1.13981515084028,2.85596344616718,17.4811853373129));
#11261=CARTESIAN_POINT('Ctrl Pts',(1.049543402046,2.89035881022278,17.4861675317271));
#11262=CARTESIAN_POINT('Ctrl Pts',(0.957844823162484,2.920434136347,17.4911497261413));
#11263=CARTESIAN_POINT('Ctrl Pts',(0.866154630424322,2.95050671198086,17.496131464917));
#11264=CARTESIAN_POINT('Ctrl Pts',(0.773038284169241,2.9762598985608,17.5011132036927));
#11265=CARTESIAN_POINT('Ctrl Pts',(0.678939012032467,2.99757302962586,17.5060949424683));
#11266=CARTESIAN_POINT('Ctrl Pts',(0.584822660166249,3.01889002918538,17.5110775854673));
#11267=CARTESIAN_POINT('Ctrl Pts',(0.489723456199211,3.0357652757786,17.5160602284662));
#11268=CARTESIAN_POINT('Ctrl Pts',(0.394095226857328,3.04812913147857,17.5210428714652));
#11269=CARTESIAN_POINT('Ctrl Pts',(0.298363984376298,3.06050630583554,17.5260308818927));
#11270=CARTESIAN_POINT('Ctrl Pts',(0.202103014846611,3.06836233080819,17.5310188923203));
#11271=CARTESIAN_POINT('Ctrl Pts',(0.105771460058256,3.07167945076259,17.5360069027479));
#11272=CARTESIAN_POINT('Ctrl Pts',(0.0093830316901561,3.07499852912497,
17.5409978580673));
#11273=CARTESIAN_POINT('Ctrl Pts',(-0.0870756262138116,3.07377337222112,
17.5459888133867));
#11274=CARTESIAN_POINT('Ctrl Pts',(-0.183147307629121,3.06803834945201,
17.5509797687061));
#11275=CARTESIAN_POINT('Ctrl Pts',(-0.2793741728314,3.06229406294837,17.5559787858741));
#11276=CARTESIAN_POINT('Ctrl Pts',(-0.375212377248489,3.0520254112681,17.5609778030421));
#11277=CARTESIAN_POINT('Ctrl Pts',(-0.470211814422976,3.0373184060248,17.5659768202101));
#11278=CARTESIAN_POINT('Ctrl Pts',(-0.525341386131542,3.02878371440669,
17.5688778234542));
#11279=CARTESIAN_POINT('Ctrl Pts',(-0.580188698312286,3.01875529372928,
17.5717788266983));
#11280=CARTESIAN_POINT('Ctrl Pts',(-0.63466808551724,3.00725766625108,17.5746798299425));
#11281=CARTESIAN_POINT('Ctrl Pts',(-0.72856816399157,2.98744048074548,17.5796799675404));
#11282=CARTESIAN_POINT('Ctrl Pts',(-0.821703970702003,2.96318632888084,
17.5846801051384));
#11283=CARTESIAN_POINT('Ctrl Pts',(-0.91362461730408,2.93456850467935,17.5896802427364));
#11284=CARTESIAN_POINT('Ctrl Pts',(-1.00539778619647,2.90599659498482,17.5946723581014));
#11285=CARTESIAN_POINT('Ctrl Pts',(-1.09595925769914,2.87307506905623,17.5996644734665));
#11286=CARTESIAN_POINT('Ctrl Pts',(-1.18486876550315,2.8359281123708,17.6046565888315));
#11287=CARTESIAN_POINT('Ctrl Pts',(-1.27369537056722,2.79881579297632,17.6096440493508));
#11288=CARTESIAN_POINT('Ctrl Pts',(-1.36087266910783,2.75748603727323,17.6146315098701));
#11289=CARTESIAN_POINT('Ctrl Pts',(-1.44597648784965,2.71211250625522,17.6196189703894));
#11290=CARTESIAN_POINT('Ctrl Pts',(-1.53102237885595,2.66676985970214,17.6246030360869));
#11291=CARTESIAN_POINT('Ctrl Pts',(-1.61399720877885,2.61738911376037,17.6295871017845));
#11292=CARTESIAN_POINT('Ctrl Pts',(-1.6944987107767,2.56419117250959,17.6345711674821));
#11293=CARTESIAN_POINT('Ctrl Pts',(-1.75526492802091,2.52403493225613,17.6383333683283));
#11294=CARTESIAN_POINT('Ctrl Pts',(-1.81462225713076,2.48170468535302,17.6420955691745));
#11295=CARTESIAN_POINT('Ctrl Pts',(-1.87240768645122,2.4373123939533,17.6458577700207));
#11296=CARTESIAN_POINT('',(3.07052265917054,0.00228167610776854,17.2084234471775));
#11297=CARTESIAN_POINT('Ctrl Pts',(3.07052265917054,0.00228167610776854,
17.2084234471775));
#11298=CARTESIAN_POINT('Ctrl Pts',(3.07292892970749,0.349269622054914,17.2263526142767));
#11299=CARTESIAN_POINT('Ctrl Pts',(2.85875296905493,1.71502694578071,17.297071417304));
#11300=CARTESIAN_POINT('Ctrl Pts',(0.943423291082137,3.4474838904957,17.4151261119716));
#11301=CARTESIAN_POINT('Ctrl Pts',(-1.14804840810742,2.98986828496906,17.51525163954));
#11302=CARTESIAN_POINT('Ctrl Pts',(-1.8746299318936,2.44024828799233,17.5625875311804));
#11303=CARTESIAN_POINT('Ctrl Pts',(-1.869725885356,2.43378780274863,16.5626129315945));
#11304=CARTESIAN_POINT('Ctrl Pts',(-2.20951416667467,2.1750721455896,16.5846537268424));
#11305=CARTESIAN_POINT('Ctrl Pts',(-3.18623258927536,1.06968771491757,16.6594841580185));
#11306=CARTESIAN_POINT('Ctrl Pts',(-3.19506800687155,-1.72217162700502,
16.7871042251226));
#11307=CARTESIAN_POINT('Ctrl Pts',(-0.295015685898992,-3.61763670826351,
16.9454731329068));
#11308=CARTESIAN_POINT('Ctrl Pts',(2.51507553838982,-2.37564449952294,17.0859128735917));
#11309=CARTESIAN_POINT('Ctrl Pts',(3.06584404144206,-0.672382261526633,
17.1735629783486));
#11310=CARTESIAN_POINT('Ctrl Pts',(3.07052265917054,0.00228167610776854,
17.2084234471775));
#11311=CARTESIAN_POINT('Origin',(0.,0.,-2.20842344717744));
#11312=CARTESIAN_POINT('',(-1.87172893090613,2.4364505825814,15.5628209763329));
#11313=CARTESIAN_POINT('',(-1.87240768645122,2.43731239395331,15.6457416395408));
#11314=CARTESIAN_POINT('',(-1.87240768645123,2.4373123939533,-2.20842344717744));
#11315=CARTESIAN_POINT('',(3.07349950431729,0.00174555474377873,16.2915765527877));
#11316=CARTESIAN_POINT('Ctrl Pts',(-1.87240768645122,2.4373123939533,15.6457416395408));
#11317=CARTESIAN_POINT('Ctrl Pts',(-1.94889871322255,2.37854996906821,15.6507399535145));
#11318=CARTESIAN_POINT('Ctrl Pts',(-2.02253509863369,2.31624920628633,15.6557382674881));
#11319=CARTESIAN_POINT('Ctrl Pts',(-2.09298992423544,2.25073219798557,15.6607365814617));
#11320=CARTESIAN_POINT('Ctrl Pts',(-2.15649750194303,2.19167554061267,15.6652420331519));
#11321=CARTESIAN_POINT('Ctrl Pts',(-2.21742035531678,2.13000631152701,15.6697474848421));
#11322=CARTESIAN_POINT('Ctrl Pts',(-2.27554719717683,2.06598335022833,15.6742529365322));
#11323=CARTESIAN_POINT('Ctrl Pts',(-2.3400481018543,1.9949397705025,15.6792524462372));
#11324=CARTESIAN_POINT('Ctrl Pts',(-2.40133209132135,1.92074789302041,15.6842519559421));
#11325=CARTESIAN_POINT('Ctrl Pts',(-2.45907667225312,1.84373104599899,15.689251465647));
#11326=CARTESIAN_POINT('Ctrl Pts',(-2.51674292303881,1.76681867182645,15.6942441935498));
#11327=CARTESIAN_POINT('Ctrl Pts',(-2.57087904625347,1.68708929227079,15.6992369214525));
#11328=CARTESIAN_POINT('Ctrl Pts',(-2.62120073979498,1.60490153333414,15.7042296493553));
#11329=CARTESIAN_POINT('Ctrl Pts',(-2.67146934522459,1.52280048040112,15.7092171100566));
#11330=CARTESIAN_POINT('Ctrl Pts',(-2.71793129270596,1.43824657623757,15.7142045707578));
#11331=CARTESIAN_POINT('Ctrl Pts',(-2.7603444125331,1.35162900760427,15.7191920314591));
#11332=CARTESIAN_POINT('Ctrl Pts',(-2.8027271847805,1.26507341586823,15.7241759235156));
#11333=CARTESIAN_POINT('Ctrl Pts',(-2.84106669604593,1.17645748818041,15.729159815572));
#11334=CARTESIAN_POINT('Ctrl Pts',(-2.87516622868607,1.0861958421128,15.7341437076285));
#11335=CARTESIAN_POINT('Ctrl Pts',(-2.9092533431198,0.995967067104246,15.7391257846747));
#11336=CARTESIAN_POINT('Ctrl Pts',(-2.9391033919043,0.904094174735669,15.7441078617209));
#11337=CARTESIAN_POINT('Ctrl Pts',(-2.96456779391088,0.811011741780841,
15.7490899387671));
#11338=CARTESIAN_POINT('Ctrl Pts',(-2.99002987414817,0.717937795808494,
15.7540715615622));
#11339=CARTESIAN_POINT('Ctrl Pts',(-3.0111069869707,0.623654951964332,15.7590531843573));
#11340=CARTESIAN_POINT('Ctrl Pts',(-3.0277007316326,0.528611889453358,15.7640348071524));
#11341=CARTESIAN_POINT('Ctrl Pts',(-3.04429749332698,0.433551546454296,
15.7690173356935));
#11342=CARTESIAN_POINT('Ctrl Pts',(-3.05640919250096,0.337731142704052,
15.7739998642346));
#11343=CARTESIAN_POINT('Ctrl Pts',(-3.06398892224302,0.241607397179938,
15.7789823927757));
#11344=CARTESIAN_POINT('Ctrl Pts',(-3.07157682181259,0.145380044476267,
15.7839702917455));
#11345=CARTESIAN_POINT('Ctrl Pts',(-3.0746229653488,0.0488491355876539,
15.7889581907154));
#11346=CARTESIAN_POINT('Ctrl Pts',(-3.07313252882311,-0.0475258907255083,
15.7939460896852));
#11347=CARTESIAN_POINT('Ctrl Pts',(-3.07164121187647,-0.143957847066444,
15.7989369350743));
#11348=CARTESIAN_POINT('Ctrl Pts',(-3.0656080063516,-0.240233299583437,
15.8039277804633));
#11349=CARTESIAN_POINT('Ctrl Pts',(-3.05509005170745,-0.335897344374959,
15.8089186258524));
#11350=CARTESIAN_POINT('Ctrl Pts',(-3.04455509979157,-0.431715984600633,
15.8139175365696));
#11351=CARTESIAN_POINT('Ctrl Pts',(-3.02952099559556,-0.526920810886396,
15.8189164472867));
#11352=CARTESIAN_POINT('Ctrl Pts',(-3.01009610214631,-0.621066587286403,
15.8239153580039));
#11353=CARTESIAN_POINT('Ctrl Pts',(-2.99881880738429,-0.675723755617151,
15.8268175201081));
#11354=CARTESIAN_POINT('Ctrl Pts',(-2.98606254577936,-0.730024228112748,
15.8297196822123));
#11355=CARTESIAN_POINT('Ctrl Pts',(-2.9718561208065,-0.783883567390549,
15.8326218443165));
#11356=CARTESIAN_POINT('Ctrl Pts',(-2.94738293536546,-0.876666206259633,
15.8376213534465));
#11357=CARTESIAN_POINT('Ctrl Pts',(-2.91851752846084,-0.968464617543111,
15.8426208625764));
#11358=CARTESIAN_POINT('Ctrl Pts',(-2.88535552324197,-1.05883225984905,
15.8476203717064));
#11359=CARTESIAN_POINT('Ctrl Pts',(-2.85223850207296,-1.14907731902107,
15.8526130990339));
#11360=CARTESIAN_POINT('Ctrl Pts',(-2.81483661589741,-1.23789505791854,
15.8576058263614));
#11361=CARTESIAN_POINT('Ctrl Pts',(-2.77329588864699,-1.32485175171175,
15.862598553689));
#11362=CARTESIAN_POINT('Ctrl Pts',(-2.73179898581234,-1.41171670839406,
15.8675860138155));
#11363=CARTESIAN_POINT('Ctrl Pts',(-2.68617211019909,-1.49672412902359,
15.8725734739421));
#11364=CARTESIAN_POINT('Ctrl Pts',(-2.63660985891815,-1.57945899024179,
15.8775609340687));
#11365=CARTESIAN_POINT('Ctrl Pts',(-2.58708307056109,-1.66213465277532,
15.8825448255535));
#11366=CARTESIAN_POINT('Ctrl Pts',(-2.53362672924973,-1.74254061295899,
15.8875287170383));
#11367=CARTESIAN_POINT('Ctrl Pts',(-2.47648150971177,-1.82028612642511,
15.8925126085232));
#11368=CARTESIAN_POINT('Ctrl Pts',(-2.41935710102748,-1.89800332692791,
15.8974946849999));
#11369=CARTESIAN_POINT('Ctrl Pts',(-2.35854674301075,-1.97306165241466,
15.9024767614766));
#11370=CARTESIAN_POINT('Ctrl Pts',(-2.29433406001567,-2.04509986823431,
15.9074588379533));
#11371=CARTESIAN_POINT('Ctrl Pts',(-2.2301272317088,-2.117131515861,15.9124404601817));
#11372=CARTESIAN_POINT('Ctrl Pts',(-2.16251898740404,-2.18614327373474,
15.9174220824101));
#11373=CARTESIAN_POINT('Ctrl Pts',(-2.09183210125438,-2.25180832003119,
15.9224037046385));
#11374=CARTESIAN_POINT('Ctrl Pts',(-2.02113236294399,-2.31748530542661,
15.9273862326164));
#11375=CARTESIAN_POINT('Ctrl Pts',(-1.94735319274614,-2.37981407204683,
15.9323687605942));
#11376=CARTESIAN_POINT('Ctrl Pts',(-1.87085214441084,-2.43850661343236,
15.9373512885721));
#11377=CARTESIAN_POINT('Ctrl Pts',(-1.79426863911818,-2.49726241680564,
15.9423391869874));
#11378=CARTESIAN_POINT('Ctrl Pts',(-1.71495774750215,-2.5523739027431,15.9473270854027));
#11379=CARTESIAN_POINT('Ctrl Pts',(-1.63330766125205,-2.60359527071612,
15.9523149838181));
#11380=CARTESIAN_POINT('Ctrl Pts',(-1.55160934312264,-2.65484689588729,
15.9573058286567));
#11381=CARTESIAN_POINT('Ctrl Pts',(-1.46756946122401,-2.70220361210594,
15.9622966734953));
#11382=CARTESIAN_POINT('Ctrl Pts',(-1.38160069503937,-2.74546567442879,
15.9672875183339));
#11383=CARTESIAN_POINT('Ctrl Pts',(-1.29549300100815,-2.78879764941206,
15.9722864285125));
#11384=CARTESIAN_POINT('Ctrl Pts',(-1.20745059917281,-2.82802157915426,
15.9772853386911));
#11385=CARTESIAN_POINT('Ctrl Pts',(-1.11790594835827,-2.86298594838068,
15.9822842488697));
#11386=CARTESIAN_POINT('Ctrl Pts',(-1.06591989781353,-2.88328486572901,
15.9851864166133));
#11387=CARTESIAN_POINT('Ctrl Pts',(-1.0134278131718,-2.90214902794488,15.988088584357));
#11388=CARTESIAN_POINT('Ctrl Pts',(-0.960516202473417,-2.91955662297994,
15.9909907521007));
#11389=CARTESIAN_POINT('Ctrl Pts',(-0.869366371595686,-2.94954435766598,
15.9959902615755));
#11390=CARTESIAN_POINT('Ctrl Pts',(-0.776650751275227,-2.97531206614178,
16.0009897710503));
#11391=CARTESIAN_POINT('Ctrl Pts',(-0.68279595920373,-2.99669683620066,
16.0059892805251));
#11392=CARTESIAN_POINT('Ctrl Pts',(-0.589068480626812,-3.01805259793991,
16.0109820081936));
#11393=CARTESIAN_POINT('Ctrl Pts',(-0.494205325772783,-3.03503714072928,
16.0159747358621));
#11394=CARTESIAN_POINT('Ctrl Pts',(-0.398649802683796,-3.04753680614692,
16.0209674635306));
#11395=CARTESIAN_POINT('Ctrl Pts',(-0.303195088327821,-3.06002328472414,
16.0259549239939));
#11396=CARTESIAN_POINT('Ctrl Pts',(-0.207049890730401,-3.06803423510474,
16.0309423844572));
#11397=CARTESIAN_POINT('Ctrl Pts',(-0.110668277027359,-3.07150692371998,
16.0359298449204));
#11398=CARTESIAN_POINT('Ctrl Pts',(-0.0143556267159142,-3.07497712754196,
16.0409137367343));
#11399=CARTESIAN_POINT('Ctrl Pts',(0.0821926659962651,-3.07391550919141,
16.0458976285481));
#11400=CARTESIAN_POINT('Ctrl Pts',(0.17851781197312,-3.06831120338344,16.050881520362));
#11401=CARTESIAN_POINT('Ctrl Pts',(0.274807878659714,-3.06270893852821,
16.0558635971629));
#11402=CARTESIAN_POINT('Ctrl Pts',(0.370874522301607,-3.05256729867365,
16.0608456739638));
#11403=CARTESIAN_POINT('Ctrl Pts',(0.466260322292488,-3.03792751096133,
16.0658277507647));
#11404=CARTESIAN_POINT('Ctrl Pts',(0.561637425239996,-3.02328905806896,
16.0708093733121));
#11405=CARTESIAN_POINT('Ctrl Pts',(0.656333374104444,-3.00415333950665,
16.0757909958594));
#11406=CARTESIAN_POINT('Ctrl Pts',(0.749898298321378,-2.98061315708273,
16.0807726184068));
#11407=CARTESIAN_POINT('Ctrl Pts',(0.843480234236463,-2.95706869465238,
16.0857551466981));
#11408=CARTESIAN_POINT('Ctrl Pts',(0.935930311420518,-2.9291182850923,16.0907376749893));
#11409=CARTESIAN_POINT('Ctrl Pts',(1.02681228152849,-2.89690503615535,16.0957202032806));
#11410=CARTESIAN_POINT('Ctrl Pts',(1.11779220893244,-2.86465706610974,16.100708101999));
#11411=CARTESIAN_POINT('Ctrl Pts',(1.20720024053117,-2.82813723066903,16.1056960007174));
#11412=CARTESIAN_POINT('Ctrl Pts',(1.29461884911216,-2.7875373155392,16.1106838994358));
#11413=CARTESIAN_POINT('Ctrl Pts',(1.38208909702406,-2.74691341750132,16.115674744572));
#11414=CARTESIAN_POINT('Ctrl Pts',(1.46756719315786,-2.70220484410954,16.1206655897083));
#11415=CARTESIAN_POINT('Ctrl Pts',(1.55066090894839,-2.65364899628028,16.1256564348446));
#11416=CARTESIAN_POINT('Ctrl Pts',(1.63388890622909,-2.60501468100567,16.1306553453095));
#11417=CARTESIAN_POINT('Ctrl Pts',(1.71472446124332,-2.55252091564937,16.1356542557744));
#11418=CARTESIAN_POINT('Ctrl Pts',(1.79280503120254,-2.49644795060799,16.1406531662393));
#11419=CARTESIAN_POINT('Ctrl Pts',(1.8381354414299,-2.46389426267619,16.1435553307878));
#11420=CARTESIAN_POINT('Ctrl Pts',(1.88253790320472,-2.43013496521521,16.1464574953363));
#11421=CARTESIAN_POINT('Ctrl Pts',(1.925947021523,-2.39523074468551,16.1493596598848));
#11422=CARTESIAN_POINT('Ctrl Pts',(1.99978833044786,-2.33585673685569,16.1542964021472));
#11423=CARTESIAN_POINT('Ctrl Pts',(2.07102705737978,-2.27294757807149,16.1592331444097));
#11424=CARTESIAN_POINT('Ctrl Pts',(2.13929911914238,-2.20676268067879,16.1641698866721));
#11425=CARTESIAN_POINT('Ctrl Pts',(2.20747815032313,-2.1406679698039,16.1690999019075));
#11426=CARTESIAN_POINT('Ctrl Pts',(2.27269822491405,-2.07130669737316,16.1740299171429));
#11427=CARTESIAN_POINT('Ctrl Pts',(2.3346270297246,-1.99897946014443,16.1789599323783));
#11428=CARTESIAN_POINT('Ctrl Pts',(2.39648619491134,-1.9267335556914,16.1838844037573));
#11429=CARTESIAN_POINT('Ctrl Pts',(2.45506115559679,-1.85152865704026,16.1888088751362));
#11430=CARTESIAN_POINT('Ctrl Pts',(2.51005623275266,-1.77370233083783,16.1937333465151));
#11431=CARTESIAN_POINT('Ctrl Pts',(2.56501765545072,-1.69592363076753,16.198654804344));
#11432=CARTESIAN_POINT('Ctrl Pts',(2.61640328445328,-1.61552705540436,16.203576262173));
#11433=CARTESIAN_POINT('Ctrl Pts',(2.66395815262426,-1.53288264751961,16.2084977200019));
#11434=CARTESIAN_POINT('Ctrl Pts',(2.71149769214496,-1.4502648789102,16.2134175914673));
#11435=CARTESIAN_POINT('Ctrl Pts',(2.75520869880651,-1.36540110770887,16.2183374629328));
#11436=CARTESIAN_POINT('Ctrl Pts',(2.79488060015965,-1.27868865673049,16.2232573343982));
#11437=CARTESIAN_POINT('Ctrl Pts',(2.83455120284155,-1.19197904430946,16.2281770448103));
#11438=CARTESIAN_POINT('Ctrl Pts',(2.87018277699916,-1.10342128335657,16.2330967552223));
#11439=CARTESIAN_POINT('Ctrl Pts',(2.90161214691215,-1.01343435845241,16.2380164656343));
#11440=CARTESIAN_POINT('Ctrl Pts',(2.93306700840162,-0.923374447402365,
16.2429401663005));
#11441=CARTESIAN_POINT('Ctrl Pts',(2.96031271082498,-0.831883484354772,
16.2478638669667));
#11442=CARTESIAN_POINT('Ctrl Pts',(2.98323557337827,-0.739396891885824,
16.2527875676329));
#11443=CARTESIAN_POINT('Ctrl Pts',(3.00616837220371,-0.646870209661507,
16.2577134025539));
#11444=CARTESIAN_POINT('Ctrl Pts',(3.02477451242689,-0.553347481295938,
16.2626392374749));
#11445=CARTESIAN_POINT('Ctrl Pts',(3.03899162259589,-0.459273521762331,
16.2675650723959));
#11446=CARTESIAN_POINT('Ctrl Pts',(3.05322927646138,-0.365063625540591,
16.2724980251388));
#11447=CARTESIAN_POINT('Ctrl Pts',(3.06306519115917,-0.270301356403268,
16.2774309778817));
#11448=CARTESIAN_POINT('Ctrl Pts',(3.06848897953641,-0.175435550740501,
16.2823639306246));
#11449=CARTESIAN_POINT('Ctrl Pts',(3.07186540981505,-0.116379452609501,
16.2854348046789));
#11450=CARTESIAN_POINT('Ctrl Pts',(3.07353302896985,-0.0572832459287992,
16.2885056787333));
#11451=CARTESIAN_POINT('Ctrl Pts',(3.07349950431729,0.00174555474379678,
16.2915765527877));
#11452=CARTESIAN_POINT('Ctrl Pts',(3.07349950431691,0.00174555541427581,
16.2915765528226));
#11453=CARTESIAN_POINT('Ctrl Pts',(3.07344072725167,0.105237704331132,16.2969605577714));
#11454=CARTESIAN_POINT('Ctrl Pts',(3.06815507646861,0.208578371493949,16.3023445627202));
#11455=CARTESIAN_POINT('Ctrl Pts',(3.05768593610749,0.311382347172158,16.3077285676691));
#11456=CARTESIAN_POINT('Ctrl Pts',(3.04796444844869,0.406844586320621,16.3127280743964));
#11457=CARTESIAN_POINT('Ctrl Pts',(3.03375104390199,0.502018799209545,16.3177275811238));
#11458=CARTESIAN_POINT('Ctrl Pts',(3.01507061941287,0.596449000295305,16.3227270878511));
#11459=CARTESIAN_POINT('Ctrl Pts',(2.99641553481127,0.690751107360806,16.3277198127766));
#11460=CARTESIAN_POINT('Ctrl Pts',(2.97330555755281,0.784310781501738,16.3327125377021));
#11461=CARTESIAN_POINT('Ctrl Pts',(2.94581736658922,0.876676846221759,16.3377052626275));
#11462=CARTESIAN_POINT('Ctrl Pts',(2.91835817496481,0.968945467103353,16.3426927203558));
#11463=CARTESIAN_POINT('Ctrl Pts',(2.88653007627914,1.06002256334226,16.347680178084));
#11464=CARTESIAN_POINT('Ctrl Pts',(2.85046064290332,1.14946786525731,16.3526676358122));
#11465=CARTESIAN_POINT('Ctrl Pts',(2.8144170179336,1.23884916725721,16.357651524914));
#11466=CARTESIAN_POINT('Ctrl Pts',(2.77413825493212,1.32660059008976,16.3626354140157));
#11467=CARTESIAN_POINT('Ctrl Pts',(2.72980122341365,1.41229866906733,16.3676193031175));
#11468=CARTESIAN_POINT('Ctrl Pts',(2.68548033824461,1.49796553911905,16.3726013772215));
#11469=CARTESIAN_POINT('Ctrl Pts',(2.63710432250965,1.58158016158151,16.3775834513254));
#11470=CARTESIAN_POINT('Ctrl Pts',(2.58489706785975,1.6627415308971,16.3825655254294));
#11471=CARTESIAN_POINT('Ctrl Pts',(2.53269457314998,1.74389550041242,16.3875471452981));
#11472=CARTESIAN_POINT('Ctrl Pts',(2.47666177164626,1.82259629240314,16.3925287651669));
#11473=CARTESIAN_POINT('Ctrl Pts',(2.41706658745815,1.89847079561246,16.3975103850356));
#11474=CARTESIAN_POINT('Ctrl Pts',(2.35746056758654,1.97435909443486,16.4024929106697));
#11475=CARTESIAN_POINT('Ctrl Pts',(2.2942911498305,2.04741973872511,16.4074754363039));
#11476=CARTESIAN_POINT('Ctrl Pts',(2.22786665969213,2.11731254108416,16.412457961938));
#11477=CARTESIAN_POINT('Ctrl Pts',(2.1613705731089,2.18728067825058,16.417445858048));
#11478=CARTESIAN_POINT('Ctrl Pts',(2.09161271260839,2.25407383804249,16.422433754158));
#11479=CARTESIAN_POINT('Ctrl Pts',(2.01893824213935,2.31738875125156,16.4274216502681));
#11480=CARTESIAN_POINT('Ctrl Pts',(1.94622084153036,2.38074106573879,16.4324124928196));
#11481=CARTESIAN_POINT('Ctrl Pts',(1.87058374441533,2.44061077016044,16.4374033353712));
#11482=CARTESIAN_POINT('Ctrl Pts',(1.79240347777767,2.49673627418887,16.4423941779227));
#11483=CARTESIAN_POINT('Ctrl Pts',(1.71409686885811,2.5529524791647,16.4473930858655));
#11484=CARTESIAN_POINT('Ctrl Pts',(1.63323925193748,2.60541216294122,16.4523919938082));
#11485=CARTESIAN_POINT('Ctrl Pts',(1.55023420471965,2.65389829505903,16.457390901751));
#11486=CARTESIAN_POINT('Ctrl Pts',(1.5020443754255,2.68204764872133,16.4602930929851));
#11487=CARTESIAN_POINT('Ctrl Pts',(1.45313118248957,2.70885856575204,16.4631952842192));
#11488=CARTESIAN_POINT('Ctrl Pts',(1.40357668229841,2.73429602400841,16.4660974754532));
#11489=CARTESIAN_POINT('Ctrl Pts',(1.31821075943991,2.77811630452486,16.4710969857309));
#11490=CARTESIAN_POINT('Ctrl Pts',(1.23064079775987,2.81801197819068,16.4760964960085));
#11491=CARTESIAN_POINT('Ctrl Pts',(1.14126283010773,2.85375566624308,16.4810960062861));
#11492=CARTESIAN_POINT('Ctrl Pts',(1.05200610348146,2.88945086805752,16.4860887347386));
#11493=CARTESIAN_POINT('Ctrl Pts',(0.960946649267999,2.92100511620065,16.491081463191));
#11494=CARTESIAN_POINT('Ctrl Pts',(0.868504659300871,2.94823708455963,16.4960741916434));
#11495=CARTESIAN_POINT('Ctrl Pts',(0.776160193714096,2.97544032375732,16.5010616528709));
#11496=CARTESIAN_POINT('Ctrl Pts',(0.682436510708975,2.99833022462567,16.5060491140985));
#11497=CARTESIAN_POINT('Ctrl Pts',(0.587772362556805,3.01677408829604,16.511036575326));
#11498=CARTESIAN_POINT('Ctrl Pts',(0.493175949506328,3.03520475481621,16.5160204678721));
#11499=CARTESIAN_POINT('Ctrl Pts',(0.397640838690288,3.04919562465904,16.5210043604181));
#11500=CARTESIAN_POINT('Ctrl Pts',(0.301618526377949,3.05866449852637,16.5259882529642));
#11501=CARTESIAN_POINT('Ctrl Pts',(0.205631183452242,3.06812992402111,16.5309703304772));
#11502=CARTESIAN_POINT('Ctrl Pts',(0.109157427959209,3.07307658255847,16.5359524079903));
#11503=CARTESIAN_POINT('Ctrl Pts',(0.0126555189035832,3.0734739445522,16.5409344855033));
#11504=CARTESIAN_POINT('Ctrl Pts',(-0.0838375909435241,3.07387127031379,
16.545916108742));
#11505=CARTESIAN_POINT('Ctrl Pts',(-0.180358410290221,3.06972012263184,
16.5508977319808));
#11506=CARTESIAN_POINT('Ctrl Pts',(-0.276448104101494,3.06104209310141,
16.5558793552195));
#11507=CARTESIAN_POINT('Ctrl Pts',(-0.372555268239498,3.052362485795,16.5608618841806));
#11508=CARTESIAN_POINT('Ctrl Pts',(-0.468230713995893,3.03915440158997,
16.5658444131417));
#11509=CARTESIAN_POINT('Ctrl Pts',(-0.563021225989915,3.02149124590571,
16.5708269421029));
#11510=CARTESIAN_POINT('Ctrl Pts',(-0.65791390739893,3.0038090520894,16.5758148414545));
#11511=CARTESIAN_POINT('Ctrl Pts',(-0.751919318580594,2.98166228084182,
16.5808027408062));
#11512=CARTESIAN_POINT('Ctrl Pts',(-0.844595154077178,2.95517533755771,
16.5857906401578));
#11513=CARTESIAN_POINT('Ctrl Pts',(-0.937325734045256,2.92867274819172,
16.5907814859077));
#11514=CARTESIAN_POINT('Ctrl Pts',(-1.0287247587648,2.89782502219214,16.5957723316575));
#11515=CARTESIAN_POINT('Ctrl Pts',(-1.11836780700864,2.86280556417069,16.6007631774073));
#11516=CARTESIAN_POINT('Ctrl Pts',(-1.20815571994477,2.82772951410882,16.6057620884489));
#11517=CARTESIAN_POINT('Ctrl Pts',(-1.29618158954533,2.78846844924509,16.6107609994904));
#11518=CARTESIAN_POINT('Ctrl Pts',(-1.38204364321624,2.74524272483247,16.615759910532));
#11519=CARTESIAN_POINT('Ctrl Pts',(-1.43189154145502,2.72014768669051,16.6186620681004));
#11520=CARTESIAN_POINT('Ctrl Pts',(-1.48101062256676,2.69371721369591,16.6215642256689));
#11521=CARTESIAN_POINT('Ctrl Pts',(-1.52932683708478,2.66600106439819,16.6244663832373));
#11522=CARTESIAN_POINT('Ctrl Pts',(-1.61255627029755,2.6182572703137,16.6294656351847));
#11523=CARTESIAN_POINT('Ctrl Pts',(-1.69369397800676,2.5665284006922,16.634464887132));
#11524=CARTESIAN_POINT('Ctrl Pts',(-1.77233367960811,2.51102281513466,16.6394641390793));
#11525=CARTESIAN_POINT('Ctrl Pts',(-1.80616406839357,2.4871446022099,16.6416147911491));
#11526=CARTESIAN_POINT('Ctrl Pts',(-1.83953241787483,2.46256804264623,16.6437654432188));
#11527=CARTESIAN_POINT('Ctrl Pts',(-1.87240768645125,2.43731239395329,16.6459160952886));
#11528=CARTESIAN_POINT('',(3.07037524043715,-0.00221840733777449,16.2084234471775));
#11529=CARTESIAN_POINT('Ctrl Pts',(3.07037524043715,-0.00221840733777449,
16.2084234471775));
#11530=CARTESIAN_POINT('Ctrl Pts',(3.06588334332531,0.666027613145282,16.2429481320417));
#11531=CARTESIAN_POINT('Ctrl Pts',(2.52336161388572,2.36268932502765,16.3302624528339));
#11532=CARTESIAN_POINT('Ctrl Pts',(0.167664259077209,3.42172443700271,16.4483256143063));
#11533=CARTESIAN_POINT('Ctrl Pts',(-1.39569145920811,2.79471881426235,16.5318640909144));
#11534=CARTESIAN_POINT('Ctrl Pts',(-1.869725885356,2.43378780274863,16.5626129315945));
#11535=CARTESIAN_POINT('Ctrl Pts',(-1.87172893090644,2.43645058258115,15.5628209763329));
#11536=CARTESIAN_POINT('Ctrl Pts',(-2.45835653554609,1.9767821845083,15.6013879410997));
#11537=CARTESIAN_POINT('Ctrl Pts',(-3.47096169057706,0.381579628323511,
15.6927445417946));
#11538=CARTESIAN_POINT('Ctrl Pts',(-2.51002850343834,-2.62184868499999,
15.8368907784176));
#11539=CARTESIAN_POINT('Ctrl Pts',(0.832597508902196,-3.53286213886185,
15.9952596862017));
#11540=CARTESIAN_POINT('Ctrl Pts',(2.85331955098111,-1.72819282485178,16.1191039091217));
#11541=CARTESIAN_POINT('Ctrl Pts',(3.07275163521828,-0.355747510086772,
16.1901584961136));
#11542=CARTESIAN_POINT('Ctrl Pts',(3.07037524043715,-0.00221840733777449,
16.2084234471775));
#11543=CARTESIAN_POINT('Origin',(0.,0.,-2.20842344717744));
#11544=CARTESIAN_POINT('',(-1.87525415797411,2.44104769786763,14.562635342152));
#11545=CARTESIAN_POINT('',(-1.87240768645123,2.43731239395329,14.6458302897736));
#11546=CARTESIAN_POINT('',(-1.87240768645123,2.4373123939533,-2.20842344717744));
#11547=CARTESIAN_POINT('',(3.07349970959544,0.00133608261959707,15.2915765528521));
#11548=CARTESIAN_POINT('Ctrl Pts',(-1.87240768645123,2.43731239395329,14.6458302897736));
#11549=CARTESIAN_POINT('Ctrl Pts',(-1.94893277448196,2.37852380231007,14.6508120790211));
#11550=CARTESIAN_POINT('Ctrl Pts',(-2.02268470075316,2.31612913500427,14.6557938682687));
#11551=CARTESIAN_POINT('Ctrl Pts',(-2.09331608143157,2.25042885540067,14.6607756575162));
#11552=CARTESIAN_POINT('Ctrl Pts',(-2.16396717155315,2.18471024236065,14.6657588369149));
#11553=CARTESIAN_POINT('Ctrl Pts',(-2.23149566505041,2.11568448362781,14.6707420163135));
#11554=CARTESIAN_POINT('Ctrl Pts',(-2.29559068105625,2.04368923152413,14.6757251957122));
#11555=CARTESIAN_POINT('Ctrl Pts',(-2.35975808405306,1.97161267013951,14.6807140029644));
#11556=CARTESIAN_POINT('Ctrl Pts',(-2.42048397971851,1.89656025150382,14.6857028102166));
#11557=CARTESIAN_POINT('Ctrl Pts',(-2.47749766809196,1.81890284363924,14.6906916174688));
#11558=CARTESIAN_POINT('Ctrl Pts',(-2.53455000648345,1.74119279122033,14.6956838066718));
#11559=CARTESIAN_POINT('Ctrl Pts',(-2.5878848860152,1.66087459943201,14.7006759958748));
#11560=CARTESIAN_POINT('Ctrl Pts',(-2.63727597990184,1.57834649422514,14.7056681850778));
#11561=CARTESIAN_POINT('Ctrl Pts',(-2.68674191146347,1.49569334194947,14.7106679384751));
#11562=CARTESIAN_POINT('Ctrl Pts',(-2.7322519277768,1.41082398076427,14.7156676918725));
#11563=CARTESIAN_POINT('Ctrl Pts',(-2.77362663010867,1.32415919237531,14.7206674452698));
#11564=CARTESIAN_POINT('Ctrl Pts',(-2.78292824485698,1.30467572957304,14.7217914601223));
#11565=CARTESIAN_POINT('Ctrl Pts',(-2.79202105216519,1.2851015921285,14.7229154749748));
#11566=CARTESIAN_POINT('Ctrl Pts',(-2.8009033586599,1.26544167208436,14.7240394898273));
#11567=CARTESIAN_POINT('Ctrl Pts',(-2.84041100002516,1.17799624663823,14.729038999325));
#11568=CARTESIAN_POINT('Ctrl Pts',(-2.87588898212958,1.08854528756348,14.7340385088227));
#11569=CARTESIAN_POINT('Ctrl Pts',(-2.90712996363765,0.997495676441848,
14.7390380183204));
#11570=CARTESIAN_POINT('Ctrl Pts',(-2.9383285669528,0.906569573539159,14.7440307460152));
#11571=CARTESIAN_POINT('Ctrl Pts',(-2.96530145113131,0.814049540111176,
14.7490234737101));
#11572=CARTESIAN_POINT('Ctrl Pts',(-2.98788847522648,0.720364289515247,
14.7540162014049));
#11573=CARTESIAN_POINT('Ctrl Pts',(-3.01045167058067,0.626777874496728,
14.7590036618979));
#11574=CARTESIAN_POINT('Ctrl Pts',(-3.02863810165544,0.532029110500205,
14.7639911223909));
#11575=CARTESIAN_POINT('Ctrl Pts',(-3.04233712002355,0.436562822657639,
14.7689785828838));
#11576=CARTESIAN_POINT('Ctrl Pts',(-3.05602633642372,0.341164843176166,
14.7739624747322));
#11577=CARTESIAN_POINT('Ctrl Pts',(-3.06523446096093,0.245050793739427,
14.7789463665806));
#11578=CARTESIAN_POINT('Ctrl Pts',(-3.06990191759497,0.148675708663856,
14.783930258429));
#11579=CARTESIAN_POINT('Ctrl Pts',(-3.0745676744569,0.0523357210075346,
14.7889123352674));
#11580=CARTESIAN_POINT('Ctrl Pts',(-3.07469602772451,-0.044264675407972,
14.7938944121058));
#11581=CARTESIAN_POINT('Ctrl Pts',(-3.0702793440808,-0.140666269271646,
14.7988764889442));
#11582=CARTESIAN_POINT('Ctrl Pts',(-3.06586306313689,-0.237059073530537,
14.8038581115319));
#11583=CARTESIAN_POINT('Ctrl Pts',(-3.0569025894642,-0.333252672781994,
14.8088397341197));
#11584=CARTESIAN_POINT('Ctrl Pts',(-3.04344237477877,-0.4287898802455,14.8138213567075));
#11585=CARTESIAN_POINT('Ctrl Pts',(-3.02997971278918,-0.524344458056383,
14.818803885042));
#11586=CARTESIAN_POINT('Ctrl Pts',(-3.01201574625005,-0.619241972402748,
14.8237864133764));
#11587=CARTESIAN_POINT('Ctrl Pts',(-2.98964639589013,-0.713033433676944,
14.8287689417109));
#11588=CARTESIAN_POINT('Ctrl Pts',(-2.96725293466763,-0.806925988322121,
14.8337568404766));
#11589=CARTESIAN_POINT('Ctrl Pts',(-2.94044471197877,-0.899709682159225,
14.8387447392422));
#11590=CARTESIAN_POINT('Ctrl Pts',(-2.90936804084717,-0.990948965838843,
14.8437326380079));
#11591=CARTESIAN_POINT('Ctrl Pts',(-2.8782730122995,-1.08224214581533,14.8487234831938));
#11592=CARTESIAN_POINT('Ctrl Pts',(-2.84290467559671,-1.17198869088507,
14.8537143283797));
#11593=CARTESIAN_POINT('Ctrl Pts',(-2.80345738990325,-1.25977335778975,
14.8587051735656));
#11594=CARTESIAN_POINT('Ctrl Pts',(-2.76394635640081,-1.34769988693106,
14.8637040840832));
#11595=CARTESIAN_POINT('Ctrl Pts',(-2.7203434102168,-1.43365781601732,14.8687029946009));
#11596=CARTESIAN_POINT('Ctrl Pts',(-2.67288867297959,-1.51725686416552,
14.8737019051185));
#11597=CARTESIAN_POINT('Ctrl Pts',(-2.64533838230143,-1.56579107193887,
14.8766040692828));
#11598=CARTESIAN_POINT('Ctrl Pts',(-2.61649066707091,-1.61353075410667,
14.8795062334471));
#11599=CARTESIAN_POINT('Ctrl Pts',(-2.58639891791687,-1.66040443488881,
14.8824083976114));
#11600=CARTESIAN_POINT('Ctrl Pts',(-2.53456036679689,-1.74115293790765,
14.8874079070988));
#11601=CARTESIAN_POINT('Ctrl Pts',(-2.47884563527945,-1.81961330975353,
14.8924074165862));
#11602=CARTESIAN_POINT('Ctrl Pts',(-2.41948312518099,-1.8953901068024,14.8974069260736));
#11603=CARTESIAN_POINT('Ctrl Pts',(-2.36020113995041,-1.97106411310741,
14.9023996537582));
#11604=CARTESIAN_POINT('Ctrl Pts',(-2.29728147872303,-2.04406143677695,
14.9073923814427));
#11605=CARTESIAN_POINT('Ctrl Pts',(-2.23099655396568,-2.11401433916453,
14.9123851091273));
#11606=CARTESIAN_POINT('Ctrl Pts',(-2.16478155813299,-2.18389344300352,
14.91737256961));
#11607=CARTESIAN_POINT('Ctrl Pts',(-2.09520865681056,-2.2507341934602,14.9223600300927));
#11608=CARTESIAN_POINT('Ctrl Pts',(-2.02259072317702,-2.3142015937507,14.9273474905754));
#11609=CARTESIAN_POINT('Ctrl Pts',(-1.95002474937136,-2.37762358163368,
14.9323313824136));
#11610=CARTESIAN_POINT('Ctrl Pts',(-1.87441840416002,-2.43767672965214,
14.9373152742519));
#11611=CARTESIAN_POINT('Ctrl Pts',(-1.79612093054769,-2.49406332173995,
14.9422991660901));
#11612=CARTESIAN_POINT('Ctrl Pts',(-1.71785197093536,-2.55042937922794,
14.9472812429184));
#11613=CARTESIAN_POINT('Ctrl Pts',(-1.63689418600184,-2.60313127755666,
14.9522633197467));
#11614=CARTESIAN_POINT('Ctrl Pts',(-1.55362860267938,-2.65191259564423,
14.957245396575));
#11615=CARTESIAN_POINT('Ctrl Pts',(-1.4703706112591,-2.70068946599985,14.9622270191527));
#11616=CARTESIAN_POINT('Ctrl Pts',(-1.38480561864298,-2.74554624509045,
14.9672086417304));
#11617=CARTESIAN_POINT('Ctrl Pts',(-1.29734131138029,-2.78627130261683,
14.9721902643081));
#11618=CARTESIAN_POINT('Ctrl Pts',(-1.20986110156398,-2.8270037646769,14.9771727926327));
#11619=CARTESIAN_POINT('Ctrl Pts',(-1.12048128922809,-2.86360282799463,
14.9821553209572));
#11620=CARTESIAN_POINT('Ctrl Pts',(-1.02963070758082,-2.8959044970452,14.9871378492818));
#11621=CARTESIAN_POINT('Ctrl Pts',(-0.938682202394371,-2.928240982535,14.9921257480376));
#11622=CARTESIAN_POINT('Ctrl Pts',(-0.846260177329899,-2.95627067918442,
14.9971136467935));
#11623=CARTESIAN_POINT('Ctrl Pts',(-0.752809628174246,-2.9798791777064,
15.0021015455494));
#11624=CARTESIAN_POINT('Ctrl Pts',(-0.659303876495205,-3.00350162209283,
15.0070923907256));
#11625=CARTESIAN_POINT('Ctrl Pts',(-0.564768820949472,-3.02269758079422,
15.0120832359017));
#11626=CARTESIAN_POINT('Ctrl Pts',(-0.469658583527638,-3.03740400093876,
15.0170740810779));
#11627=CARTESIAN_POINT('Ctrl Pts',(-0.374394645557665,-3.05213418703005,
15.0220729915861));
#11628=CARTESIAN_POINT('Ctrl Pts',(-0.278554105879261,-3.0623603009767,
15.0270719020943));
#11629=CARTESIAN_POINT('Ctrl Pts',(-0.182595063680014,-3.06807126591279,
15.0320708126024));
#11630=CARTESIAN_POINT('Ctrl Pts',(-0.126885143956322,-3.07138682003716,
15.0349729768668));
#11631=CARTESIAN_POINT('Ctrl Pts',(-0.0711352813546049,-3.07318152364552,
15.0378751411312));
#11632=CARTESIAN_POINT('Ctrl Pts',(-0.0154344978284385,-3.0734612452863,
15.0407773053956));
#11633=CARTESIAN_POINT('Ctrl Pts',(0.0805203035956334,-3.07394311704455,
15.0457768148829));
#11634=CARTESIAN_POINT('Ctrl Pts',(0.176666230714479,-3.06992790200305,
15.0507763243702));
#11635=CARTESIAN_POINT('Ctrl Pts',(0.272547234741744,-3.06139188194433,
15.0557758338575));
#11636=CARTESIAN_POINT('Ctrl Pts',(0.368298176794052,-3.05286744094277,
15.0607685615419));
#11637=CARTESIAN_POINT('Ctrl Pts',(0.463784476478959,-3.039834421342,15.0657612892262));
#11638=CARTESIAN_POINT('Ctrl Pts',(0.558549362064147,-3.02232110473684,
15.0707540169105));
#11639=CARTESIAN_POINT('Ctrl Pts',(0.653214273082363,-3.00482626423951,
15.075741477393));
#11640=CARTESIAN_POINT('Ctrl Pts',(0.747158853611802,-2.98286060228277,
15.0807289378754));
#11641=CARTESIAN_POINT('Ctrl Pts',(0.839931766644163,-2.95650416495259,
15.0857163983578));
#11642=CARTESIAN_POINT('Ctrl Pts',(0.932638298487297,-2.93016658626979,
15.0907002901956));
#11643=CARTESIAN_POINT('Ctrl Pts',(1.0241744084024,-2.89944459738611,15.0956841820333));
#11644=CARTESIAN_POINT('Ctrl Pts',(1.11410022855096,-2.86446904866202,15.1006680738711));
#11645=CARTESIAN_POINT('Ctrl Pts',(1.20399329994227,-2.82950623716682,15.1056501506989));
#11646=CARTESIAN_POINT('Ctrl Pts',(1.29227683804504,-2.79029310256283,15.1106322275266));
#11647=CARTESIAN_POINT('Ctrl Pts',(1.37852830812589,-2.74700963844242,15.1156143043544));
#11648=CARTESIAN_POINT('Ctrl Pts',(1.4647719140591,-2.7037301207771,15.1205959269315));
#11649=CARTESIAN_POINT('Ctrl Pts',(1.54898342808684,-2.65638120849873,15.1255775495086));
#11650=CARTESIAN_POINT('Ctrl Pts',(1.63076337076852,-2.60518964349233,15.1305591720857));
#11651=CARTESIAN_POINT('Ctrl Pts',(1.7125581824843,-2.55398877095769,15.1355417004095));
#11652=CARTESIAN_POINT('Ctrl Pts',(1.79192017278298,-2.4989440910873,15.1405242287334));
#11653=CARTESIAN_POINT('Ctrl Pts',(1.86847830457372,-2.44032601824784,15.1455067570572));
#11654=CARTESIAN_POINT('Ctrl Pts',(1.94511895474752,-2.38164476376488,15.1504946558123));
#11655=CARTESIAN_POINT('Ctrl Pts',(2.01894936386824,-2.31938269426886,15.1554825545673));
#11656=CARTESIAN_POINT('Ctrl Pts',(2.0896312876575,-2.25385077847733,15.1604704533224));
#11657=CARTESIAN_POINT('Ctrl Pts',(2.16035496422921,-2.18828015208375,15.1654612984977));
#11658=CARTESIAN_POINT('Ctrl Pts',(2.22792614485703,-2.1194361465061,15.170452143673));
#11659=CARTESIAN_POINT('Ctrl Pts',(2.29204469385155,-2.04766534653174,15.1754429888483));
#11660=CARTESIAN_POINT('Ctrl Pts',(2.35626686004106,-1.97577856313149,15.1804418993555));
#11661=CARTESIAN_POINT('Ctrl Pts',(2.41702497696603,-1.90095588155568,15.1854408098626));
#11662=CARTESIAN_POINT('Ctrl Pts',(2.47406034061865,-1.82357552105141,15.1904397203698));
#11663=CARTESIAN_POINT('Ctrl Pts',(2.50717275466987,-1.77865162870884,15.1933418846398));
#11664=CARTESIAN_POINT('Ctrl Pts',(2.53903123799888,-1.73286620314677,15.1962440489098));
#11665=CARTESIAN_POINT('Ctrl Pts',(2.56959224495687,-1.68629711043384,15.1991462131798));
#11666=CARTESIAN_POINT('Ctrl Pts',(2.62325694598382,-1.60452243458724,15.2042423730706));
#11667=CARTESIAN_POINT('Ctrl Pts',(2.67310143634579,-1.52005111486671,15.2093385329613));
#11668=CARTESIAN_POINT('Ctrl Pts',(2.71885041980543,-1.43326712259921,15.2144346928521));
#11669=CARTESIAN_POINT('Ctrl Pts',(2.76453038840025,-1.34661404877059,15.2195231649046));
#11670=CARTESIAN_POINT('Ctrl Pts',(2.80612694416417,-1.25765560565154,15.2246116369571));
#11671=CARTESIAN_POINT('Ctrl Pts',(2.84340806580197,-1.16680453432968,15.2297001090096));
#11672=CARTESIAN_POINT('Ctrl Pts',(2.88118664983322,-1.07474118748064,15.2348564793273));
#11673=CARTESIAN_POINT('Ctrl Pts',(2.91453352909174,-0.98073468158956,15.2400128496451));
#11674=CARTESIAN_POINT('Ctrl Pts',(2.94325508575896,-0.885241068949039,
15.2451692199628));
#11675=CARTESIAN_POINT('Ctrl Pts',(2.97152681557719,-0.79124304345131,15.2502448330347));
#11676=CARTESIAN_POINT('Ctrl Pts',(2.99531692206572,-0.695804568008259,
15.2553204461067));
#11677=CARTESIAN_POINT('Ctrl Pts',(3.0144892537006,-0.599380337785263,15.2603960591786));
#11678=CARTESIAN_POINT('Ctrl Pts',(3.03411915706434,-0.500654822430843,
15.2655928081193));
#11679=CARTESIAN_POINT('Ctrl Pts',(3.0489078940216,-0.400896314881121,15.2707895570599));
#11680=CARTESIAN_POINT('Ctrl Pts',(3.05876400975235,-0.300607688929764,
15.2759863060006));
#11681=CARTESIAN_POINT('Ctrl Pts',(3.06862012548311,-0.200319062978392,
15.2811830549413));
#11682=CARTESIAN_POINT('Ctrl Pts',(3.07354354442197,-0.0995007836552704,
15.2863798038819));
#11683=CARTESIAN_POINT('Ctrl Pts',(3.07349970959569,0.00133608204624416,
15.2915765528226));
#11684=CARTESIAN_POINT('Ctrl Pts',(3.07349970959544,0.00133608261957393,
15.2915765528522));
#11685=CARTESIAN_POINT('Ctrl Pts',(3.07345335999379,0.107957847706477,15.2970714335281));
#11686=CARTESIAN_POINT('Ctrl Pts',(3.06785451556908,0.214401037215095,15.3025663142041));
#11687=CARTESIAN_POINT('Ctrl Pts',(3.05678458082994,0.320109788042046,15.3080611948801));
#11688=CARTESIAN_POINT('Ctrl Pts',(3.04577427243867,0.425249156402119,15.3135264783024));
#11689=CARTESIAN_POINT('Ctrl Pts',(3.0293518421405,0.529661713023204,15.3189917617247));
#11690=CARTESIAN_POINT('Ctrl Pts',(3.00764794714884,0.632815989061115,15.324457045147));
#11691=CARTESIAN_POINT('Ctrl Pts',(2.98576774592482,0.736808213391975,15.3299667244498));
#11692=CARTESIAN_POINT('Ctrl Pts',(2.95852002176638,0.839521339723275,15.3354764037526));
#11693=CARTESIAN_POINT('Ctrl Pts',(2.92608819114021,0.940430830880104,15.3409860830555));
#11694=CARTESIAN_POINT('Ctrl Pts',(2.89365636051403,1.04134032203693,15.3464957623583));
#11695=CARTESIAN_POINT('Ctrl Pts',(2.85604060194039,1.14044592833878,15.3520054416611));
#11696=CARTESIAN_POINT('Ctrl Pts',(2.81347151615592,1.23724705608028,15.3575151209639));
#11697=CARTESIAN_POINT('Ctrl Pts',(2.77484412337439,1.32508486405897,15.3625146304109));
#11698=CARTESIAN_POINT('Ctrl Pts',(2.73203143966757,1.4112662729297,15.367514139858));
#11699=CARTESIAN_POINT('Ctrl Pts',(2.68519747965701,1.49536508761026,15.372513649305));
#11700=CARTESIAN_POINT('Ctrl Pts',(2.63842704961544,1.5793498227834,15.3775063769492));
#11701=CARTESIAN_POINT('Ctrl Pts',(2.58764639613873,1.66125719809427,15.3824991045934));
#11702=CARTESIAN_POINT('Ctrl Pts',(2.53306732292495,1.74068152961126,15.3874918322377));
#11703=CARTESIAN_POINT('Ctrl Pts',(2.47854582925639,1.82002207046238,15.3924792926802));
#11704=CARTESIAN_POINT('Ctrl Pts',(2.42023412928086,1.89688441517076,15.3974667531228));
#11705=CARTESIAN_POINT('Ctrl Pts',(2.35838909377463,1.97088891933687,15.4024542135653));
#11706=CARTESIAN_POINT('Ctrl Pts',(2.29658830983209,2.04484047155619,15.4074381053637));
#11707=CARTESIAN_POINT('Ctrl Pts',(2.23125949694744,2.11593791243814,15.4124219971621));
#11708=CARTESIAN_POINT('Ctrl Pts',(2.16270125905387,2.18383275781064,15.4174058889605));
#11709=CARTESIAN_POINT('Ctrl Pts',(2.0941679883689,2.25170287756562,15.4223879657492));
#11710=CARTESIAN_POINT('Ctrl Pts',(2.022407940991,2.31637241056922,15.4273700425379));
#11711=CARTESIAN_POINT('Ctrl Pts',(1.94775754940253,2.37752871249654,15.4323521193266));
#11712=CARTESIAN_POINT('Ctrl Pts',(1.87311396420502,2.43867943838209,15.437333741865));
#11713=CARTESIAN_POINT('Ctrl Pts',(1.79558089842724,2.49631729201769,15.4423153644034));
#11714=CARTESIAN_POINT('Ctrl Pts',(1.71552809589033,2.55016972027567,15.4472969869419));
#11715=CARTESIAN_POINT('Ctrl Pts',(1.63546073833702,2.60403193985828,15.4522795152274));
#11716=CARTESIAN_POINT('Ctrl Pts',(1.55287309840775,2.65410712220057,15.457262043513));
#11717=CARTESIAN_POINT('Ctrl Pts',(1.46816322861558,2.70016647341254,15.4622445717985));
#11718=CARTESIAN_POINT('Ctrl Pts',(1.38336205405292,2.74627546982525,15.4672324705162));
#11719=CARTESIAN_POINT('Ctrl Pts',(1.29643446922358,2.78835978367424,15.4722203692338));
#11720=CARTESIAN_POINT('Ctrl Pts',(1.20780221607635,2.82623708432981,15.4772082679515));
#11721=CARTESIAN_POINT('Ctrl Pts',(1.11911760663284,2.8641367596301,15.4821991130898));
#11722=CARTESIAN_POINT('Ctrl Pts',(1.02872673496034,2.89782432019123,15.4871899582281));
#11723=CARTESIAN_POINT('Ctrl Pts',(0.937068357705508,2.92716674328387,15.4921808033664));
#11724=CARTESIAN_POINT('Ctrl Pts',(0.845261858177207,2.95655658447999,15.4971797138376));
#11725=CARTESIAN_POINT('Ctrl Pts',(0.752184186637816,2.98158715319984,15.5021786243089));
#11726=CARTESIAN_POINT('Ctrl Pts',(0.658286124793895,3.00217614871344,15.5071775347801));
#11727=CARTESIAN_POINT('Ctrl Pts',(0.6037727187388,3.01412928438694,15.5100796994361));
#11728=CARTESIAN_POINT('Ctrl Pts',(0.548982951197105,3.02458635612461,15.5129818640921));
#11729=CARTESIAN_POINT('Ctrl Pts',(0.494005671626,3.03353929369661,15.5158840287482));
#11730=CARTESIAN_POINT('Ctrl Pts',(0.39928521003126,3.04896432720255,15.5208841738624));
#11731=CARTESIAN_POINT('Ctrl Pts',(0.303675208612645,3.05997581872414,15.5258843189766));
#11732=CARTESIAN_POINT('Ctrl Pts',(0.207622625814003,3.06647926705042,15.5308844640909));
#11733=CARTESIAN_POINT('Ctrl Pts',(0.111730390356419,3.0729718587124,15.5358762621107));
#11734=CARTESIAN_POINT('Ctrl Pts',(0.0153974777927567,3.07497135057233,
15.5408680601306));
#11735=CARTESIAN_POINT('Ctrl Pts',(-0.0809207646067817,3.07243455257479,
15.5458598581505));
#11736=CARTESIAN_POINT('Ctrl Pts',(-0.177147004766832,3.06990017770179,
15.5508468880539));
#11737=CARTESIAN_POINT('Ctrl Pts',(-0.273358166450199,3.0628381328422,15.5558339179573));
#11738=CARTESIAN_POINT('Ctrl Pts',(-0.369096071907349,3.05125717364213,
15.5608209478607));
#11739=CARTESIAN_POINT('Ctrl Pts',(-0.464768669155436,3.03968411446558,
15.5658045758305));
#11740=CARTESIAN_POINT('Ctrl Pts',(-0.559968217377031,3.02359831967842,
15.5707882038004));
#11741=CARTESIAN_POINT('Ctrl Pts',(-0.65423990659825,3.00306050465426,15.5757718317703));
#11742=CARTESIAN_POINT('Ctrl Pts',(-0.74847302501317,2.98253109257792,15.5807534207128));
#11743=CARTESIAN_POINT('Ctrl Pts',(-0.84177861100914,2.95755337559329,15.5857350096554));
#11744=CARTESIAN_POINT('Ctrl Pts',(-0.93371137753408,2.92823928555427,15.5907165985979));
#11745=CARTESIAN_POINT('Ctrl Pts',(-1.02566263012013,2.89891930096775,15.5956991892503));
#11746=CARTESIAN_POINT('Ctrl Pts',(-1.11624009047942,2.86526132574961,15.6006817799027));
#11747=CARTESIAN_POINT('Ctrl Pts',(-1.20501358122756,2.82742719076144,15.6056643705551));
#11748=CARTESIAN_POINT('Ctrl Pts',(-1.29379445198079,2.78958991050877,15.6106473754252));
#11749=CARTESIAN_POINT('Ctrl Pts',(-1.38077065412379,2.74757595989212,15.6156303802952));
#11750=CARTESIAN_POINT('Ctrl Pts',(-1.46553343822706,2.70159471265369,15.6206133851652));
#11751=CARTESIAN_POINT('Ctrl Pts',(-1.55037167699749,2.65557253354,15.6256008258378));
#11752=CARTESIAN_POINT('Ctrl Pts',(-1.63299218083952,2.60557622236346,15.6305882665103));
#11753=CARTESIAN_POINT('Ctrl Pts',(-1.7130124979475,2.55186019050333,15.6355757071829));
#11754=CARTESIAN_POINT('Ctrl Pts',(-1.76738114006162,2.51536361291474,15.6389643513022));
#11755=CARTESIAN_POINT('Ctrl Pts',(-1.82055002616516,2.47715081678408,15.6423529954215));
#11756=CARTESIAN_POINT('Ctrl Pts',(-1.87240768645122,2.4373123939533,15.6457416395408));
#11757=CARTESIAN_POINT('',(3.07834638629682,-0.000587882647548141,15.2084234471775));
#11758=CARTESIAN_POINT('Ctrl Pts',(3.07834638629682,-0.000587882647548141,
15.2084234471775));
#11759=CARTESIAN_POINT('Ctrl Pts',(3.07575445609013,0.982278794615726,15.2595436498067));
#11760=CARTESIAN_POINT('Ctrl Pts',(2.03467585423313,2.98483364549918,15.3634534883639));
#11761=CARTESIAN_POINT('Ctrl Pts',(-0.534116492601284,3.26769481122963,
15.4815859980824));
#11762=CARTESIAN_POINT('Ctrl Pts',(-1.65539322584549,2.60596644955508,15.5485983051717));
#11763=CARTESIAN_POINT('Ctrl Pts',(-1.87172893090644,2.43645058258115,15.5628209763329));
#11764=CARTESIAN_POINT('Ctrl Pts',(-1.87525415797411,2.44104769786763,14.562635342152));
#11765=CARTESIAN_POINT('Ctrl Pts',(-1.91249396820152,2.41267325486651,14.5650700668161));
#11766=CARTESIAN_POINT('Ctrl Pts',(-2.74116781123522,1.74852114079692,14.6202944274082));
#11767=CARTESIAN_POINT('Ctrl Pts',(-3.60135346758601,-0.452312705771215,
14.7283084239283));
#11768=CARTESIAN_POINT('Ctrl Pts',(-1.58136610914474,-3.26704986372211,
14.8866773317125));
#11769=CARTESIAN_POINT('Ctrl Pts',(1.87939897421738,-3.10518809039125,15.0450462394967));
#11770=CARTESIAN_POINT('Ctrl Pts',(3.06346382418965,-1.07966618593221,15.1522949446517));
#11771=CARTESIAN_POINT('Ctrl Pts',(3.07843103100426,-0.0326853759081321,
15.2067540138786));
#11772=CARTESIAN_POINT('Ctrl Pts',(3.07834638629682,-0.000587882647548141,
15.2084234471775));
#11773=CARTESIAN_POINT('Origin',(0.,0.,-2.20842344717744));
#11774=CARTESIAN_POINT('',(-1.87032611617503,2.43456032588387,13.5625747566432));
#11775=CARTESIAN_POINT('',(-1.87240768645124,2.43731239395329,13.6459260020382));
#11776=CARTESIAN_POINT('',(-1.87240768645123,2.4373123939533,-2.20842344717744));
#11777=CARTESIAN_POINT('',(3.07349878502588,-0.00273284548775181,14.2915765527908));
#11778=CARTESIAN_POINT('Ctrl Pts',(-1.87240768645124,2.43731239395329,13.6459260020382));
#11779=CARTESIAN_POINT('Ctrl Pts',(-1.9487521347337,2.37866257453064,13.6509133149982));
#11780=CARTESIAN_POINT('Ctrl Pts',(-2.02242004960628,2.31635947729713,13.6559006279582));
#11781=CARTESIAN_POINT('Ctrl Pts',(-2.09304608808842,2.25067996906218,13.6608879409183));
#11782=CARTESIAN_POINT('Ctrl Pts',(-2.1636225280082,2.18504658558881,13.665871751437));
#11783=CARTESIAN_POINT('Ctrl Pts',(-2.2311610176019,2.11604180284899,13.6708555619558));
#11784=CARTESIAN_POINT('Ctrl Pts',(-2.29532957011213,2.0439824888117,13.6758393724745));
#11785=CARTESIAN_POINT('Ctrl Pts',(-2.35947532998472,1.97194877020658,13.6808214127463));
#11786=CARTESIAN_POINT('Ctrl Pts',(-2.42025323946719,1.89686300354484,13.685803453018));
#11787=CARTESIAN_POINT('Ctrl Pts',(-2.47736913516805,1.81907790325668,13.6907854932898));
#11788=CARTESIAN_POINT('Ctrl Pts',(-2.53448033586542,1.74129919700844,13.6957671240311));
#11789=CARTESIAN_POINT('Ctrl Pts',(-2.58792986166185,1.66082195226451,13.7007487547725));
#11790=CARTESIAN_POINT('Ctrl Pts',(-2.63746537424263,1.57802999010512,13.7057303855138));
#11791=CARTESIAN_POINT('Ctrl Pts',(-2.68701033785819,1.49522223180933,13.710712966716));
#11792=CARTESIAN_POINT('Ctrl Pts',(-2.73263957979876,1.41009925568748,13.7156955479182));
#11793=CARTESIAN_POINT('Ctrl Pts',(-2.77414597988313,1.32307079640443,13.7206781291204));
#11794=CARTESIAN_POINT('Ctrl Pts',(-2.81569732138376,1.23594810629897,13.7256661052558));
#11795=CARTESIAN_POINT('Ctrl Pts',(-2.85311672012191,1.14691621111724,13.7306540813912));
#11796=CARTESIAN_POINT('Ctrl Pts',(-2.88624472676201,1.05640599545746,13.7356420575266));
#11797=CARTESIAN_POINT('Ctrl Pts',(-2.91939256922463,0.965841585635226,
13.7406330202772));
#11798=CARTESIAN_POINT('Ctrl Pts',(-2.94824377220229,0.873797511510271,
13.7456239830279));
#11799=CARTESIAN_POINT('Ctrl Pts',(-2.97268903577202,0.780718993364979,
13.7506149457785));
#11800=CARTESIAN_POINT('Ctrl Pts',(-2.9971735686465,0.687490952238094,13.7556139261001));
#11801=CARTESIAN_POINT('Ctrl Pts',(-3.01723793901163,0.593225578119903,
13.7606129064218));
#11802=CARTESIAN_POINT('Ctrl Pts',(-3.03282414139059,0.498377344387172,
13.7656118867435));
#11803=CARTESIAN_POINT('Ctrl Pts',(-3.04136104928331,0.446426868223962,
13.7683499388697));
#11804=CARTESIAN_POINT('Ctrl Pts',(-3.04855542185305,0.394301620162721,
13.7710879909959));
#11805=CARTESIAN_POINT('Ctrl Pts',(-3.05440435245989,0.34207645588974,13.7738260431222));
#11806=CARTESIAN_POINT('Ctrl Pts',(-3.06508412871873,0.246716618851419,
13.7788255526152));
#11807=CARTESIAN_POINT('Ctrl Pts',(-3.07131261933319,0.150688668848877,
13.7838250621083));
#11808=CARTESIAN_POINT('Ctrl Pts',(-3.07301775946229,0.054443549014884,
13.7888245716014));
#11809=CARTESIAN_POINT('Ctrl Pts',(-3.07472058657965,-0.0416710149252134,
13.7938172992916));
#11810=CARTESIAN_POINT('Ctrl Pts',(-3.07191225019003,-0.138001728080463,
13.7988100269818));
#11811=CARTESIAN_POINT('Ctrl Pts',(-3.06457231374823,-0.23409140054223,
13.803802754672));
#11812=CARTESIAN_POINT('Ctrl Pts',(-3.05724012075436,-0.330079700821654,
13.8087902151603));
#11813=CARTESIAN_POINT('Ctrl Pts',(-3.04538586475401,-0.425827030564542,
13.8137776756486));
#11814=CARTESIAN_POINT('Ctrl Pts',(-3.02904115811137,-0.520876100879417,
13.8187651361369));
#11815=CARTESIAN_POINT('Ctrl Pts',(-3.01270814648839,-0.615857161362664,
13.8237490279807));
#11816=CARTESIAN_POINT('Ctrl Pts',(-2.99189114573891,-0.710140524268516,
13.8287329198245));
#11817=CARTESIAN_POINT('Ctrl Pts',(-2.96667350386284,-0.803274904051028,
13.8337168116682));
#11818=CARTESIAN_POINT('Ctrl Pts',(-2.94146504562736,-0.89637536659911,
13.838698888502));
#11819=CARTESIAN_POINT('Ctrl Pts',(-2.91185924507421,-0.988327254129027,
13.8436809653358));
#11820=CARTESIAN_POINT('Ctrl Pts',(-2.87799015758435,-1.07869129172697,
13.8486630421696));
#11821=CARTESIAN_POINT('Ctrl Pts',(-2.84412415817497,-1.16904709020655,
13.8536446647528));
#11822=CARTESIAN_POINT('Ctrl Pts',(-2.80599579889547,-1.25781491561944,
13.8586262873359));
#11823=CARTESIAN_POINT('Ctrl Pts',(-2.76378806944643,-1.34457344804423,
13.8636079099191));
#11824=CARTESIAN_POINT('Ctrl Pts',(-2.72157266588854,-1.4313477546988,13.868590438249));
#11825=CARTESIAN_POINT('Ctrl Pts',(-2.67527661120517,-1.51611164812035,
13.8735729665789));
#11826=CARTESIAN_POINT('Ctrl Pts',(-2.62512934371512,-1.59846744688962,
13.8785554949088));
#11827=CARTESIAN_POINT('Ctrl Pts',(-2.57492802486133,-1.68091201307252,
13.88354339367));
#11828=CARTESIAN_POINT('Ctrl Pts',(-2.52086743470754,-1.76094292723813,
13.8885312924311));
#11829=CARTESIAN_POINT('Ctrl Pts',(-2.46322082221231,-1.83819080375779,
13.8935191911923));
#11830=CARTESIAN_POINT('Ctrl Pts',(-2.40554015707186,-1.91548431165837,
13.8985100363737));
#11831=CARTESIAN_POINT('Ctrl Pts',(-2.34426953036604,-1.98999116959674,
13.9035008815551));
#11832=CARTESIAN_POINT('Ctrl Pts',(-2.27972165649791,-2.0613760983611,13.9084917267365));
#11833=CARTESIAN_POINT('Ctrl Pts',(-2.21506947163559,-2.13287638697302,
13.9134906372497));
#11834=CARTESIAN_POINT('Ctrl Pts',(-2.1471297736494,-2.20124436127135,13.918489547763));
#11835=CARTESIAN_POINT('Ctrl Pts',(-2.07625113660596,-2.26618257599481,
13.9234884582762));
#11836=CARTESIAN_POINT('Ctrl Pts',(-2.035101881555,-2.30388306335847,13.9263906224863));
#11837=CARTESIAN_POINT('Ctrl Pts',(-1.99296267410306,-2.34042831230664,
13.9292927866964));
#11838=CARTESIAN_POINT('Ctrl Pts',(-1.9499063098848,-2.3757667462677,13.9321949509065));
#11839=CARTESIAN_POINT('Ctrl Pts',(-1.87573383511858,-2.43664367233532,
13.9371944603994));
#11840=CARTESIAN_POINT('Ctrl Pts',(-1.79857744293475,-2.49415064949183,
13.9421939698923));
#11841=CARTESIAN_POINT('Ctrl Pts',(-1.71877614513896,-2.54798171361202,
13.9471934793852));
#11842=CARTESIAN_POINT('Ctrl Pts',(-1.6390830972969,-2.60173975623556,13.9521862070752));
#11843=CARTESIAN_POINT('Ctrl Pts',(-1.55675263514735,-2.6518315524901,13.9571789347653));
#11844=CARTESIAN_POINT('Ctrl Pts',(-1.47215711934958,-2.69799104259972,
13.9621716624553));
#11845=CARTESIAN_POINT('Ctrl Pts',(-1.38765084968853,-2.74410183561085,
13.9671591229435));
#11846=CARTESIAN_POINT('Ctrl Pts',(-1.30088465999158,-2.78628836027448,
13.9721465834316));
#11847=CARTESIAN_POINT('Ctrl Pts',(-1.21225933205399,-2.824328161147,13.9771340439198));
#11848=CARTESIAN_POINT('Ctrl Pts',(-1.12369741761024,-2.86234074365278,
13.9821179357634));
#11849=CARTESIAN_POINT('Ctrl Pts',(-1.03327941163226,-2.8962123281375,13.987101827607));
#11850=CARTESIAN_POINT('Ctrl Pts',(-0.941429227903033,-2.92576712314051,
13.9920857194506));
#11851=CARTESIAN_POINT('Ctrl Pts',(-0.849612493735829,-2.95531115501917,
13.9970677962843));
#11852=CARTESIAN_POINT('Ctrl Pts',(-0.756365035543576,-2.9805413866251,
14.0020498731179));
#11853=CARTESIAN_POINT('Ctrl Pts',(-0.66212830039646,-3.00133109866507,
14.0070319499515));
#11854=CARTESIAN_POINT('Ctrl Pts',(-0.56790015746843,-3.02211891516229,
14.0120135725345));
#11855=CARTESIAN_POINT('Ctrl Pts',(-0.472683345612832,-3.03846692266898,
14.0169951951176));
#11856=CARTESIAN_POINT('Ctrl Pts',(-0.376930893757469,-3.05029922324535,
14.0219768177006));
#11857=CARTESIAN_POINT('Ctrl Pts',(-0.281161032419288,-3.06213367514244,
14.0269593460303));
#11858=CARTESIAN_POINT('Ctrl Pts',(-0.184855773315668,-3.06945073573416,
14.0319418743601));
#11859=CARTESIAN_POINT('Ctrl Pts',(-0.0884736066038495,-3.07222633784272,
14.0369244026899));
#11860=CARTESIAN_POINT('Ctrl Pts',(0.00801244587907222,-3.07500493164129,
14.0419123014509));
#11861=CARTESIAN_POINT('Ctrl Pts',(0.10457513195456,-3.07323228183864,14.0469002002119));
#11862=CARTESIAN_POINT('Ctrl Pts',(0.200755842985021,-3.06693647497097,
14.0518880989729));
#11863=CARTESIAN_POINT('Ctrl Pts',(0.296993369281649,-3.06063694908377,
14.0568789441541));
#11864=CARTESIAN_POINT('Ctrl Pts',(0.392848035266852,-3.0498089952097,14.0618697893354));
#11865=CARTESIAN_POINT('Ctrl Pts',(0.487868353479512,-3.03453237248727,
14.0668606345166));
#11866=CARTESIAN_POINT('Ctrl Pts',(0.583042226926029,-3.01923106235672,
14.0718595450297));
#11867=CARTESIAN_POINT('Ctrl Pts',(0.677378630943842,-2.99946681816297,
14.0768584555428));
#11868=CARTESIAN_POINT('Ctrl Pts',(0.770438289047837,-2.97537007660712,
14.0818573660559));
#11869=CARTESIAN_POINT('Ctrl Pts',(0.824464943171497,-2.96138048812087,
14.0847595302675));
#11870=CARTESIAN_POINT('Ctrl Pts',(0.878061573354344,-2.94593156383784,
14.087661694479));
#11871=CARTESIAN_POINT('Ctrl Pts',(0.931145283868948,-2.92905628322991,
14.0905638586905));
#11872=CARTESIAN_POINT('Ctrl Pts',(1.02259169946942,-2.89998552105282,14.0955633681833));
#11873=CARTESIAN_POINT('Ctrl Pts',(1.11283602641801,-2.86657709802122,14.100562877676));
#11874=CARTESIAN_POINT('Ctrl Pts',(1.20143704886018,-2.82894879197665,14.1055623871688));
#11875=CARTESIAN_POINT('Ctrl Pts',(1.28991788457799,-2.7913715284903,14.1105551148587));
#11876=CARTESIAN_POINT('Ctrl Pts',(1.37675944546292,-2.7495859286715,14.1155478425485));
#11877=CARTESIAN_POINT('Ctrl Pts',(1.46153583028535,-2.70375946910817,14.1205405702384));
#11878=CARTESIAN_POINT('Ctrl Pts',(1.54622277815864,-2.6579813553046,14.1255280307264));
#11879=CARTESIAN_POINT('Ctrl Pts',(1.62884849700867,-2.60817106398228,14.1305154912144));
#11880=CARTESIAN_POINT('Ctrl Pts',(1.70900818665148,-2.55454365160555,14.1355029517024));
#11881=CARTESIAN_POINT('Ctrl Pts',(1.78911052016263,-2.50095461089591,14.1404868435459));
#11882=CARTESIAN_POINT('Ctrl Pts',(1.86674996841423,-2.44355412209013,14.1454707353893));
#11883=CARTESIAN_POINT('Ctrl Pts',(1.94154827836441,-2.38260205086376,14.1504546272328));
#11884=CARTESIAN_POINT('Ctrl Pts',(2.01631934862266,-2.32167217687211,14.1554367040662));
#11885=CARTESIAN_POINT('Ctrl Pts',(2.08825099642142,-2.25719356731368,14.1604187808997));
#11886=CARTESIAN_POINT('Ctrl Pts',(2.1569965840487,-2.18946751206823,14.1654008577332));
#11887=CARTESIAN_POINT('Ctrl Pts',(2.22573590366212,-2.12174763187877,14.170382480316));
#11888=CARTESIAN_POINT('Ctrl Pts',(2.29128942808784,-2.05078120288479,14.1753641028989));
#11889=CARTESIAN_POINT('Ctrl Pts',(2.35334684241256,-1.97690689950408,14.1803457254817));
#11890=CARTESIAN_POINT('Ctrl Pts',(2.41541553986862,-1.9030191644734,14.1853282538113));
#11891=CARTESIAN_POINT('Ctrl Pts',(2.47398658249804,-1.82622284117964,14.1903107821409));
#11892=CARTESIAN_POINT('Ctrl Pts',(2.52879015725592,-1.74688940421699,14.1952933104705));
#11893=CARTESIAN_POINT('Ctrl Pts',(2.58365280219058,-1.66747045750125,14.2002812092313));
#11894=CARTESIAN_POINT('Ctrl Pts',(2.63473962238392,-1.58550929943602,14.2052691079922));
#11895=CARTESIAN_POINT('Ctrl Pts',(2.68182448641721,-1.50140589916687,14.210257006753));
#11896=CARTESIAN_POINT('Ctrl Pts',(2.72893716412597,-1.41725281786477,14.2152478519341));
#11897=CARTESIAN_POINT('Ctrl Pts',(2.77204298248141,-1.33095536715174,14.2202386971152));
#11898=CARTESIAN_POINT('Ctrl Pts',(2.81096302978059,-1.24293567621448,14.2252295422963));
#11899=CARTESIAN_POINT('Ctrl Pts',(2.84994597285909,-1.1547737432338,14.2302284528092));
#11900=CARTESIAN_POINT('Ctrl Pts',(2.88472947973862,-1.0648844217315,14.2352273633222));
#11901=CARTESIAN_POINT('Ctrl Pts',(2.9151837949497,-0.973707189899856,14.2402262738351));
#11902=CARTESIAN_POINT('Ctrl Pts',(2.93286433224172,-0.920773395906811,
14.2431284380483));
#11903=CARTESIAN_POINT('Ctrl Pts',(2.94908666271836,-0.867405765024594,
14.2460306022615));
#11904=CARTESIAN_POINT('Ctrl Pts',(2.96383331659796,-0.813691785274952,
14.2489327664748));
#11905=CARTESIAN_POINT('Ctrl Pts',(2.99602294044835,-0.696442623684468,
14.2552677340639));
#11906=CARTESIAN_POINT('Ctrl Pts',(3.0212702832211,-0.577211563723087,14.261602701653));
#11907=CARTESIAN_POINT('Ctrl Pts',(3.03937583013342,-0.456724001121871,
14.2679376692422));
#11908=CARTESIAN_POINT('Ctrl Pts',(3.0571635192287,-0.338351697110416,14.2741614212476));
#11909=CARTESIAN_POINT('Ctrl Pts',(3.06805797242532,-0.218766467335917,
14.280385173253));
#11910=CARTESIAN_POINT('Ctrl Pts',(3.07191552615637,-0.0986775058431663,
14.2866089252584));
#11911=CARTESIAN_POINT('Ctrl Pts',(3.07294185722405,-0.0667269380329351,
14.2882648011025));
#11912=CARTESIAN_POINT('Ctrl Pts',(3.07347032466018,-0.0347408385475268,
14.2899206769466));
#11913=CARTESIAN_POINT('Ctrl Pts',(3.07349878502588,-0.00273284548777434,
14.2915765527908));
#11914=CARTESIAN_POINT('Ctrl Pts',(3.07349878502642,-0.00273284487212046,
14.2915765528226));
#11915=CARTESIAN_POINT('Ctrl Pts',(3.07358364945225,0.092710080672881,14.2965141205922));
#11916=CARTESIAN_POINT('Ctrl Pts',(3.069218504179,0.188253195776559,14.3014516883618));
#11917=CARTESIAN_POINT('Ctrl Pts',(3.06040211108299,0.283445177201534,14.3063892561314));
#11918=CARTESIAN_POINT('Ctrl Pts',(3.05159013460488,0.378589471709134,14.3113243504008));
#11919=CARTESIAN_POINT('Ctrl Pts',(3.03833137922742,0.473382536333788,14.3162594446702));
#11920=CARTESIAN_POINT('Ctrl Pts',(3.02067664916565,0.567375388244305,14.3211945389396));
#11921=CARTESIAN_POINT('Ctrl Pts',(3.00302571336008,0.661348039734878,14.326128572586));
#11922=CARTESIAN_POINT('Ctrl Pts',(2.98098076245997,0.75452037973125,14.3310626062324));
#11923=CARTESIAN_POINT('Ctrl Pts',(2.95464399796869,0.846452063183483,14.3359966398788));
#11924=CARTESIAN_POINT('Ctrl Pts',(2.9283053601704,0.938390285641968,14.340931024478));
#11925=CARTESIAN_POINT('Ctrl Pts',(2.89767442723464,1.02908724567049,14.3458654090772));
#11926=CARTESIAN_POINT('Ctrl Pts',(2.86290337237835,1.11811740457999,14.3507997936764));
#11927=CARTESIAN_POINT('Ctrl Pts',(2.82809727590647,1.20723728641037,14.3557391510556));
#11928=CARTESIAN_POINT('Ctrl Pts',(2.78914288932616,1.29468659443031,14.3606785084349));
#11929=CARTESIAN_POINT('Ctrl Pts',(2.74624057947654,1.38005975582087,14.3656178658141));
#11930=CARTESIAN_POINT('Ctrl Pts',(2.70331618390134,1.46547686655169,14.3705597659304));
#11931=CARTESIAN_POINT('Ctrl Pts',(2.6564400393954,1.54881531245498,14.3755016660467));
#11932=CARTESIAN_POINT('Ctrl Pts',(2.60585741194769,1.62969610621038,14.3804435661629));
#11933=CARTESIAN_POINT('Ctrl Pts',(2.55518929437882,1.71071359727091,14.3853938186259));
#11934=CARTESIAN_POINT('Ctrl Pts',(2.50080243806243,1.78926477176493,14.3903440710888));
#11935=CARTESIAN_POINT('Ctrl Pts',(2.44298415864097,1.8650015149134,14.3952943235517));
#11936=CARTESIAN_POINT('Ctrl Pts',(2.39623608107655,1.92623728980343,14.3992967737875));
#11937=CARTESIAN_POINT('Ctrl Pts',(2.34724563426181,1.98563375217512,14.4032992240232));
#11938=CARTESIAN_POINT('Ctrl Pts',(2.29618206790021,2.04302475781708,14.407301674259));
#11939=CARTESIAN_POINT('Ctrl Pts',(2.2323979432512,2.11471256418133,14.4123011837513));
#11940=CARTESIAN_POINT('Ctrl Pts',(2.165141381716,2.18353636969329,14.4173006932437));
#11941=CARTESIAN_POINT('Ctrl Pts',(2.09469959610768,2.24914113653775,14.422300202736));
#11942=CARTESIAN_POINT('Ctrl Pts',(2.02435336433424,2.31465691093257,14.4272929304255));
#11943=CARTESIAN_POINT('Ctrl Pts',(1.95083081414323,2.37696202838997,14.432285658115));
#11944=CARTESIAN_POINT('Ctrl Pts',(1.87445831609767,2.43573567351063,14.4372783858044));
#11945=CARTESIAN_POINT('Ctrl Pts',(1.79816638911234,2.49444731391726,14.4422658462921));
#11946=CARTESIAN_POINT('Ctrl Pts',(1.71903083728364,2.54963462199363,14.4472533067797));
#11947=CARTESIAN_POINT('Ctrl Pts',(1.63741289771372,2.60101542717469,14.4522407672673));
#11948=CARTESIAN_POINT('Ctrl Pts',(1.55585335768723,2.65235946818872,14.4572246591103));
#11949=CARTESIAN_POINT('Ctrl Pts',(1.47181533135017,2.69990218759118,14.4622085509534));
#11950=CARTESIAN_POINT('Ctrl Pts',(1.38569017436835,2.74340390585474,14.4671924427965));
#11951=CARTESIAN_POINT('Ctrl Pts',(1.29959638203551,2.78688978186998,14.4721745196296));
#11952=CARTESIAN_POINT('Ctrl Pts',(1.21141736067392,2.82633738301604,14.4771565964627));
#11953=CARTESIAN_POINT('Ctrl Pts',(1.12156942928375,2.86155277171261,14.4821386732958));
#11954=CARTESIAN_POINT('Ctrl Pts',(1.03172968995484,2.89676494957709,14.4871202958782));
#11955=CARTESIAN_POINT('Ctrl Pts',(0.940221751890307,2.92774552217978,14.4921019184607));
#11956=CARTESIAN_POINT('Ctrl Pts',(0.847481291118539,2.95434894878788,14.4970835410432));
#11957=CARTESIAN_POINT('Ctrl Pts',(0.754723968496831,2.98095721236771,14.5020660693724));
#11958=CARTESIAN_POINT('Ctrl Pts',(0.660734100066584,3.00318662840565,14.5070485977017));
#11959=CARTESIAN_POINT('Ctrl Pts',(0.56596083020831,3.02094200352637,14.5120311260309));
#11960=CARTESIAN_POINT('Ctrl Pts',(0.471085408732499,3.03871651632474,14.5170190247914));
#11961=CARTESIAN_POINT('Ctrl Pts',(0.375425332250775,3.05200727985058,14.5220069235519));
#11962=CARTESIAN_POINT('Ctrl Pts',(0.279437986272481,3.06077059934716,14.5269948223123));
#11963=CARTESIAN_POINT('Ctrl Pts',(0.183393939251215,3.06953909545687,14.5319856674931));
#11964=CARTESIAN_POINT('Ctrl Pts',(0.0870226761306488,3.07377480305766,
14.5369765126738));
#11965=CARTESIAN_POINT('Ctrl Pts',(-0.0092174026773135,3.07348617850933,
14.5419673578546));
#11966=CARTESIAN_POINT('Ctrl Pts',(-0.105613007883394,3.07319708753644,
14.5469662683672));
#11967=CARTESIAN_POINT('Ctrl Pts',(-0.201876567349512,3.06836908706779,
14.5519651788798));
#11968=CARTESIAN_POINT('Ctrl Pts',(-0.297553848429102,3.0590625945353,14.5569640893924));
#11969=CARTESIAN_POINT('Ctrl Pts',(-0.353100188140001,3.053659623319,14.5598662536093));
#11970=CARTESIAN_POINT('Ctrl Pts',(-0.408449077039367,3.04674814464449,
14.5627684178262));
#11971=CARTESIAN_POINT('Ctrl Pts',(-0.463513494023612,3.03834782256048,
14.5656705820431));
#11972=CARTESIAN_POINT('Ctrl Pts',(-0.558371273141645,3.02387684583167,
14.5706700511617));
#11973=CARTESIAN_POINT('Ctrl Pts',(-0.652717332392701,3.00493397839403,
14.5756695202804));
#11974=CARTESIAN_POINT('Ctrl Pts',(-0.746097506323219,2.98156682988295,
14.580668989399));
#11975=CARTESIAN_POINT('Ctrl Pts',(-0.839355656886615,2.95823021609912,
14.5856619255243));
#11976=CARTESIAN_POINT('Ctrl Pts',(-0.931650007815505,2.9304809143819,14.5906548616496));
#11977=CARTESIAN_POINT('Ctrl Pts',(-1.02253371283178,2.89841802646245,14.5956477977749));
#11978=CARTESIAN_POINT('Ctrl Pts',(-1.11330986408678,2.86639308246476,14.6006348251506));
#11979=CARTESIAN_POINT('Ctrl Pts',(-1.20267827845999,2.83006485205293,14.6056218525262));
#11980=CARTESIAN_POINT('Ctrl Pts',(-1.29020571006753,2.78958267052782,14.6106088799019));
#11981=CARTESIAN_POINT('Ctrl Pts',(-1.37767341338736,2.74912811384376,14.6155925041547));
#11982=CARTESIAN_POINT('Ctrl Pts',(-1.46330223346942,2.70452542312112,14.6205761284074));
#11983=CARTESIAN_POINT('Ctrl Pts',(-1.54667811974368,2.65597233492861,14.6255597526602));
#11984=CARTESIAN_POINT('Ctrl Pts',(-1.63002245760475,2.60743761862943,14.6305414911706));
#11985=CARTESIAN_POINT('Ctrl Pts',(-1.71111517708098,2.55495569623841,14.6355232296811));
#11986=CARTESIAN_POINT('Ctrl Pts',(-1.78956701475662,2.4987701274217,14.6405049681915));
#11987=CARTESIAN_POINT('Ctrl Pts',(-1.81752119604303,2.47874992620123,14.6422800753855));
#11988=CARTESIAN_POINT('Ctrl Pts',(-1.8451403277701,2.45825989830704,14.6440551825796));
#11989=CARTESIAN_POINT('Ctrl Pts',(-1.87240768645123,2.43731239395329,14.6458302897736));
#11990=CARTESIAN_POINT('',(3.07201600109834,0.00268254658689539,14.2084234471775));
#11991=CARTESIAN_POINT('Ctrl Pts',(3.07201600109834,0.00268254658689539,
14.2084234471775));
#11992=CARTESIAN_POINT('Ctrl Pts',(3.07445542476385,0.291196008346456,14.2233495316436));
#11993=CARTESIAN_POINT('Ctrl Pts',(2.90505334785583,1.59729724456565,14.2910652520378));
#11994=CARTESIAN_POINT('Ctrl Pts',(1.09056355056046,3.43559442656078,14.4091358836959));
#11995=CARTESIAN_POINT('Ctrl Pts',(-1.10506138538983,3.0278871793826,14.512280430888));
#11996=CARTESIAN_POINT('Ctrl Pts',(-1.87525415797411,2.44104769786763,14.562635342152));
#11997=CARTESIAN_POINT('Ctrl Pts',(-1.87032611617489,2.43456032588397,13.5625747566432));
#11998=CARTESIAN_POINT('Ctrl Pts',(-2.16435218332819,2.21187124699417,13.5816251942419));
#11999=CARTESIAN_POINT('Ctrl Pts',(-3.12451768131251,1.18293877132523,13.6534652677685));
#12000=CARTESIAN_POINT('Ctrl Pts',(-3.28738484392744,-1.53864696090213,
13.7780949772233));
#12001=CARTESIAN_POINT('Ctrl Pts',(-0.499216609585515,-3.59515178526775,
13.9364638850075));
#12002=CARTESIAN_POINT('Ctrl Pts',(2.43813708336016,-2.49101688819496,14.0799067083255));
#12003=CARTESIAN_POINT('Ctrl Pts',(3.0658278247078,-0.729200240998579,14.1705598957155));
#12004=CARTESIAN_POINT('Ctrl Pts',(3.07201600109834,0.00268254658689539,
14.2084234471775));
#12005=CARTESIAN_POINT('Origin',(0.,0.,-2.20842344717744));
#12006=CARTESIAN_POINT('',(-1.87077372492537,2.43522501013495,12.5628034348477));
#12007=CARTESIAN_POINT('',(-1.87240768645123,2.43731239395329,12.6457543573089));
#12008=CARTESIAN_POINT('',(-1.87240768645123,2.4373123939533,-2.20842344717744));
#12009=CARTESIAN_POINT('',(3.0734998880982,0.000829373473843992,13.2915765527763));
#12010=CARTESIAN_POINT('Ctrl Pts',(-1.87240768645123,2.43731239395329,12.6457543573089));
#12011=CARTESIAN_POINT('Ctrl Pts',(-1.94880608375446,2.37862112946951,12.6507539181684));
#12012=CARTESIAN_POINT('Ctrl Pts',(-2.02234126144047,2.31641200752082,12.6557534790279));
#12013=CARTESIAN_POINT('Ctrl Pts',(-2.09269109792243,2.25101004410825,12.6607530398874));
#12014=CARTESIAN_POINT('Ctrl Pts',(-2.11375404150425,2.23142850796846,12.6622499228026));
#12015=CARTESIAN_POINT('Ctrl Pts',(-2.1345317118694,2.21156099226433,12.6637468057178));
#12016=CARTESIAN_POINT('Ctrl Pts',(-2.15501616577206,2.19141679633544,12.665243688633));
#12017=CARTESIAN_POINT('Ctrl Pts',(-2.22343315463912,2.12413625104231,12.670243198126));
#12018=CARTESIAN_POINT('Ctrl Pts',(-2.28881650109085,2.05353044898989,12.675242707619));
#12019=CARTESIAN_POINT('Ctrl Pts',(-2.35082593556614,1.97990395491033,12.6802422171119));
#12020=CARTESIAN_POINT('Ctrl Pts',(-2.41275125463733,1.90637733470246,12.685234944802));
#12021=CARTESIAN_POINT('Ctrl Pts',(-2.47131147724655,1.82983849895282,12.6902276724921));
#12022=CARTESIAN_POINT('Ctrl Pts',(-2.52620246685423,1.75062941437062,12.6952204001822));
#12023=CARTESIAN_POINT('Ctrl Pts',(-2.5810355478515,1.67150389337603,12.7002078606704));
#12024=CARTESIAN_POINT('Ctrl Pts',(-2.63220684236038,1.58971408254247,12.7051953211587));
#12025=CARTESIAN_POINT('Ctrl Pts',(-2.67945254972863,1.50563484409492,12.7101827816469));
#12026=CARTESIAN_POINT('Ctrl Pts',(-2.72666445168885,1.4216157663079,12.7151666734906));
#12027=CARTESIAN_POINT('Ctrl Pts',(-2.7699561359476,1.33531089903631,12.7201505653342));
#12028=CARTESIAN_POINT('Ctrl Pts',(-2.80910774232458,1.24712306610539,12.7251344571779));
#12029=CARTESIAN_POINT('Ctrl Pts',(-2.84824509065619,1.15896734899905,12.7301165340116));
#12030=CARTESIAN_POINT('Ctrl Pts',(-2.88324517883553,1.06893042949471,12.7350986108453));
#12031=CARTESIAN_POINT('Ctrl Pts',(-2.91393507687166,0.977437782049056,
12.740080687679));
#12032=CARTESIAN_POINT('Ctrl Pts',(-2.94462217669613,0.885953476624977,
12.7450623102621));
#12033=CARTESIAN_POINT('Ctrl Pts',(-2.97099972828891,0.793014123380326,
12.7500439328451));
#12034=CARTESIAN_POINT('Ctrl Pts',(-2.99294410379904,0.699062115648202,
12.7550255554282));
#12035=CARTESIAN_POINT('Ctrl Pts',(-3.01489246918329,0.605093025785723,
12.760008083758));
#12036=CARTESIAN_POINT('Ctrl Pts',(-3.03240595790341,0.510111343237154,
12.7649906120879));
#12037=CARTESIAN_POINT('Ctrl Pts',(-3.04541189860072,0.414570401573901,
12.7699731404177));
#12038=CARTESIAN_POINT('Ctrl Pts',(-3.05843185778531,0.318926480856186,
12.7749610391787));
#12039=CARTESIAN_POINT('Ctrl Pts',(-3.06693451014778,0.2227225332634,12.7799489379398));
#12040=CARTESIAN_POINT('Ctrl Pts',(-3.07089902991347,0.126417554463398,
12.7849368367008));
#12041=CARTESIAN_POINT('Ctrl Pts',(-3.07486589157541,0.0300556869905675,
12.7899276818821));
#12042=CARTESIAN_POINT('Ctrl Pts',(-3.07428928547725,-0.0664068917736713,
12.7949185270634));
#12043=CARTESIAN_POINT('Ctrl Pts',(-3.06920052266675,-0.162512773842922,
12.7999093722448));
#12044=CARTESIAN_POINT('Ctrl Pts',(-3.06410353628705,-0.258773965444591,
12.8049082827579));
#12045=CARTESIAN_POINT('Ctrl Pts',(-3.05447987696272,-0.354676872871751,
12.8099071932711));
#12046=CARTESIAN_POINT('Ctrl Pts',(-3.04041254424232,-0.449770842556444,
12.8149061037842));
#12047=CARTESIAN_POINT('Ctrl Pts',(-3.0322456227786,-0.504978535267283,
12.8178082679952));
#12048=CARTESIAN_POINT('Ctrl Pts',(-3.02258192059223,-0.559913777938567,
12.8207104322062));
#12049=CARTESIAN_POINT('Ctrl Pts',(-3.01144541790488,-0.614490638642867,
12.8236125964172));
#12050=CARTESIAN_POINT('Ctrl Pts',(-2.99226075196033,-0.708509278992453,
12.8286121059102));
#12051=CARTESIAN_POINT('Ctrl Pts',(-2.96863521495116,-0.801793764721497,
12.8336116154031));
#12052=CARTESIAN_POINT('Ctrl Pts',(-2.94063901313134,-0.893892859603408,
12.8386111248961));
#12053=CARTESIAN_POINT('Ctrl Pts',(-2.91268078798151,-0.985867022647913,
12.8436038525862));
#12054=CARTESIAN_POINT('Ctrl Pts',(-2.88036380765218,-1.07665857419513,
12.8485965802763));
#12055=CARTESIAN_POINT('Ctrl Pts',(-2.84380932356707,-1.16582622255336,
12.8535893079664));
#12056=CARTESIAN_POINT('Ctrl Pts',(-2.80729340354125,-1.25489980129017,
12.8585767684546));
#12057=CARTESIAN_POINT('Ctrl Pts',(-2.76654903238322,-1.34235247853241,
12.8635642289429));
#12058=CARTESIAN_POINT('Ctrl Pts',(-2.72174701495838,-1.42775888600462,
12.8685516894311));
#12059=CARTESIAN_POINT('Ctrl Pts',(-2.67697705442427,-1.51310418319588,
12.8735355812748));
#12060=CARTESIAN_POINT('Ctrl Pts',(-2.62815542265776,-1.59640573367598,
12.8785194731184));
#12061=CARTESIAN_POINT('Ctrl Pts',(-2.57550030195739,-1.6772598023614,12.8835033649621));
#12062=CARTESIAN_POINT('Ctrl Pts',(-2.52286435694783,-1.75808442599756,
12.8884854417958));
#12063=CARTESIAN_POINT('Ctrl Pts',(-2.46639793613164,-1.83646297131842,
12.8934675186295));
#12064=CARTESIAN_POINT('Ctrl Pts',(-2.40636377219709,-1.91201873574957,
12.8984495954632));
#12065=CARTESIAN_POINT('Ctrl Pts',(-2.34633508199521,-1.98756761123568,
12.9034312180463));
#12066=CARTESIAN_POINT('Ctrl Pts',(-2.28273956864474,-2.0602938739697,12.9084128406293));
#12067=CARTESIAN_POINT('Ctrl Pts',(-2.21588099888406,-2.12985296412324,
12.9133944632124));
#12068=CARTESIAN_POINT('Ctrl Pts',(-2.14901027305742,-2.19942470134495,
12.9183769915422));
#12069=CARTESIAN_POINT('Ctrl Pts',(-2.07887561677486,-2.26582780590368,
12.923359519872));
#12070=CARTESIAN_POINT('Ctrl Pts',(-2.005817716704,-2.3287545034538,12.9283420482019));
#12071=CARTESIAN_POINT('Ctrl Pts',(-1.93268107098398,-2.39174902670988,
12.9333299469629));
#12072=CARTESIAN_POINT('Ctrl Pts',(-1.85661522429066,-2.4512593753601,12.938317845724));
#12073=CARTESIAN_POINT('Ctrl Pts',(-1.77799384002364,-2.5070181799975,12.943305744485));
#12074=CARTESIAN_POINT('Ctrl Pts',(-1.6993260130258,-2.56280992212613,12.9482965896663));
#12075=CARTESIAN_POINT('Ctrl Pts',(-1.61810001205918,-2.61484547096943,
12.9532874348476));
#12076=CARTESIAN_POINT('Ctrl Pts',(-1.53471655476278,-2.66290205350048,
12.958278280029));
#12077=CARTESIAN_POINT('Ctrl Pts',(-1.4511983476937,-2.71103629668247,12.9632771905421));
#12078=CARTESIAN_POINT('Ctrl Pts',(-1.36551611247509,-2.75517853314285,
12.9682761010553));
#12079=CARTESIAN_POINT('Ctrl Pts',(-1.27809304307681,-2.79515302322407,
12.9732750115684));
#12080=CARTESIAN_POINT('Ctrl Pts',(-1.22733876320876,-2.81836058698418,
12.9761771757794));
#12081=CARTESIAN_POINT('Ctrl Pts',(-1.17599808773102,-2.8401643267722,12.9790793399904));
#12082=CARTESIAN_POINT('Ctrl Pts',(-1.12415615175048,-2.86053757124103,
12.9819815042013));
#12083=CARTESIAN_POINT('Ctrl Pts',(-1.03484892024039,-2.89563421695799,
12.9869810136943));
#12084=CARTESIAN_POINT('Ctrl Pts',(-0.943739652778633,-2.92660618265725,
12.9919805231873));
#12085=CARTESIAN_POINT('Ctrl Pts',(-0.851245066735443,-2.95326668053506,
12.9969800326802));
#12086=CARTESIAN_POINT('Ctrl Pts',(-0.75887594901092,-2.97989101361678,
13.0019727603703));
#12087=CARTESIAN_POINT('Ctrl Pts',(-0.665125665625023,-3.00221538180513,
13.0069654880604));
#12088=CARTESIAN_POINT('Ctrl Pts',(-0.570430384171196,-3.02010122790848,
13.0119582157505));
#12089=CARTESIAN_POINT('Ctrl Pts',(-0.47583500385242,-3.03796820489502,
13.0169456762387));
#12090=CARTESIAN_POINT('Ctrl Pts',(-0.380297036382623,-3.05140588734459,
13.021933136727));
#12091=CARTESIAN_POINT('Ctrl Pts',(-0.284266272365235,-3.06032595263896,
13.0269205972152));
#12092=CARTESIAN_POINT('Ctrl Pts',(-0.188304220604123,-3.06923963541812,
13.0319044890589));
#12093=CARTESIAN_POINT('Ctrl Pts',(-0.0918505090899103,-3.0736420865382,
13.0368883809025));
#12094=CARTESIAN_POINT('Ctrl Pts',(0.00463742261106573,-3.07349650143148,
13.0418722727462));
#12095=CARTESIAN_POINT('Ctrl Pts',(0.101090215797046,-3.07335096934325,
13.0468543495799));
#12096=CARTESIAN_POINT('Ctrl Pts',(0.197576765895643,-3.06866069254264,
13.0518364264136));
#12097=CARTESIAN_POINT('Ctrl Pts',(0.293638052471368,-3.05944095287698,
13.0568185032473));
#12098=CARTESIAN_POINT('Ctrl Pts',(0.389690580470852,-3.05022205383917,
13.0618001258304));
#12099=CARTESIAN_POINT('Ctrl Pts',(0.485317485101032,-3.03647455514263,
13.0667817484134));
#12100=CARTESIAN_POINT('Ctrl Pts',(0.580064365961156,-3.01826565784758,
13.0717633709965));
#12101=CARTESIAN_POINT('Ctrl Pts',(0.674828473473575,-3.00005344985418,
13.0767458993263));
#12102=CARTESIAN_POINT('Ctrl Pts',(0.768711808385569,-2.97737831517527,
13.0817284276561));
#12103=CARTESIAN_POINT('Ctrl Pts',(0.861270724562416,-2.95035845093638,
13.086710955986));
#12104=CARTESIAN_POINT('Ctrl Pts',(0.953929405609807,-2.92330946326597,
13.091698854747));
#12105=CARTESIAN_POINT('Ctrl Pts',(1.04526039592009,-2.89190652011431,13.0966867535081));
#12106=CARTESIAN_POINT('Ctrl Pts',(1.13483598647618,-2.85631747776725,13.1016746522691));
#12107=CARTESIAN_POINT('Ctrl Pts',(1.22446449056301,-2.82070741248442,13.1066654974504));
#12108=CARTESIAN_POINT('Ctrl Pts',(1.31233513051117,-2.78090650531467,13.1116563426317));
#12109=CARTESIAN_POINT('Ctrl Pts',(1.39804287468024,-2.73712958599987,13.116647187813));
#12110=CARTESIAN_POINT('Ctrl Pts',(1.48388912472832,-2.69328192207792,13.1216460983262));
#12111=CARTESIAN_POINT('Ctrl Pts',(1.56756511884007,-2.64544563374796,13.1266450088394));
#12112=CARTESIAN_POINT('Ctrl Pts',(1.64869303932901,-2.59388001111618,13.1316439193525));
#12113=CARTESIAN_POINT('Ctrl Pts',(1.6957926116729,-2.56394310703967,13.1345460835635));
#12114=CARTESIAN_POINT('Ctrl Pts',(1.74203393130432,-2.53275002469665,13.1374482477745));
#12115=CARTESIAN_POINT('Ctrl Pts',(1.78734827456124,-2.50035765350139,13.1403504119855));
#12116=CARTESIAN_POINT('Ctrl Pts',(1.86486694926461,-2.44494443320335,13.1453151076478));
#12117=CARTESIAN_POINT('Ctrl Pts',(1.93995177014087,-2.38581864905354,13.1502798033101));
#12118=CARTESIAN_POINT('Ctrl Pts',(2.01222215380273,-2.32322281620715,13.1552444989724));
#12119=CARTESIAN_POINT('Ctrl Pts',(2.08439421967946,-2.26071213973233,13.1602024405834));
#12120=CARTESIAN_POINT('Ctrl Pts',(2.1537591213376,-2.19474108272853,13.1651603821943));
#12121=CARTESIAN_POINT('Ctrl Pts',(2.21996586382998,-2.12559493164375,13.1701183238053));
#12122=CARTESIAN_POINT('Ctrl Pts',(2.2875456035691,-2.05501482577601,13.1751790833458));
#12123=CARTESIAN_POINT('Ctrl Pts',(2.35183433745504,-1.98112672110611,13.1802398428862));
#12124=CARTESIAN_POINT('Ctrl Pts',(2.41249487126627,-1.90427696150374,13.1853006024267));
#12125=CARTESIAN_POINT('Ctrl Pts',(2.47181879393753,-1.82912053096289,13.1902498517783));
#12126=CARTESIAN_POINT('Ctrl Pts',(2.52767247112209,-1.75113198889143,13.19519910113));
#12127=CARTESIAN_POINT('Ctrl Pts',(2.57977928200115,-1.67067085512306,13.2001483504816));
#12128=CARTESIAN_POINT('Ctrl Pts',(2.63186879451725,-1.59023643275524,13.2050959567868));
#12129=CARTESIAN_POINT('Ctrl Pts',(2.68021366949812,-1.50733142313621,13.210043563092));
#12130=CARTESIAN_POINT('Ctrl Pts',(2.72458015982682,-1.42234496613096,13.2149911693972));
#12131=CARTESIAN_POINT('Ctrl Pts',(2.76894446929367,-1.33736268668675,13.2199385324997));
#12132=CARTESIAN_POINT('Ctrl Pts',(2.80933057728359,-1.25029955885806,13.2248858956023));
#12133=CARTESIAN_POINT('Ctrl Pts',(2.84555087825037,-1.16156896019503,13.2298332587049));
#12134=CARTESIAN_POINT('Ctrl Pts',(2.88322011483118,-1.06928883485702,13.2349785332108));
#12135=CARTESIAN_POINT('Ctrl Pts',(2.91638305279126,-0.975205509233901,
13.2401238077168));
#12136=CARTESIAN_POINT('Ctrl Pts',(2.94488468889668,-0.879804761922721,
13.2452690822227));
#12137=CARTESIAN_POINT('Ctrl Pts',(2.97232631723561,-0.787952075245871,
13.2502229982075));
#12138=CARTESIAN_POINT('Ctrl Pts',(2.99544715264295,-0.694878677984494,
13.2551769141922));
#12139=CARTESIAN_POINT('Ctrl Pts',(3.01416077415891,-0.601030013827718,
13.260130830177));
#12140=CARTESIAN_POINT('Ctrl Pts',(3.03288686416896,-0.50711882027153,13.2650880468522));
#12141=CARTESIAN_POINT('Ctrl Pts',(3.04719983161365,-0.412431771857661,
13.2700452635274));
#12142=CARTESIAN_POINT('Ctrl Pts',(3.05706504618851,-0.317420152750973,
13.2750024802026));
#12143=CARTESIAN_POINT('Ctrl Pts',(3.06694455849492,-0.222270832572119,
13.2799668814102));
#12144=CARTESIAN_POINT('Ctrl Pts',(3.0723634378255,-0.12679644661346,13.2849312826177));
#12145=CARTESIAN_POINT('Ctrl Pts',(3.0733391029767,-0.0314484993978609,
13.2898956838253));
#12146=CARTESIAN_POINT('Ctrl Pts',(3.07344921798625,-0.0206873892918313,
13.2904559734756));
#12147=CARTESIAN_POINT('Ctrl Pts',(3.07350279090741,-0.00992788374214916,
13.291016263126));
#12148=CARTESIAN_POINT('Ctrl Pts',(3.0734998880982,0.000829373473862042,
13.2915765527763));
#12149=CARTESIAN_POINT('Ctrl Pts',(3.07349988809796,0.000829374363056769,
13.2915765528226));
#12150=CARTESIAN_POINT('Ctrl Pts',(3.07348755274492,0.0465417906928214,
13.2939574751383));
#12151=CARTESIAN_POINT('Ctrl Pts',(3.07245544142313,0.0922390841768832,
13.296338397454));
#12152=CARTESIAN_POINT('Ctrl Pts',(3.07040526815993,0.137890316033319,13.2987193197697));
#12153=CARTESIAN_POINT('Ctrl Pts',(3.06610027230851,0.233749708642161,13.3037188292627));
#12154=CARTESIAN_POINT('Ctrl Pts',(3.05729425420337,0.329575672356923,13.3087183387557));
#12155=CARTESIAN_POINT('Ctrl Pts',(3.04398627306693,0.424911543006448,13.3137178482487));
#12156=CARTESIAN_POINT('Ctrl Pts',(3.03069634412241,0.520118091152705,13.3187105759387));
#12157=CARTESIAN_POINT('Ctrl Pts',(3.01291664934233,0.614835436467569,13.3237033036288));
#12158=CARTESIAN_POINT('Ctrl Pts',(2.99069821909271,0.708608786507531,13.3286960313189));
#12159=CARTESIAN_POINT('Ctrl Pts',(2.96850322872691,0.802283208027114,13.3336834918072));
#12160=CARTESIAN_POINT('Ctrl Pts',(2.94187891259022,0.895015189178195,13.3386709522954));
#12161=CARTESIAN_POINT('Ctrl Pts',(2.91092773001671,0.986357947511824,13.3436584127837));
#12162=CARTESIAN_POINT('Ctrl Pts',(2.87999869373785,1.07763534796666,13.3486423046273));
#12163=CARTESIAN_POINT('Ctrl Pts',(2.84474908614169,1.16752508712019,13.353626196471));
#12164=CARTESIAN_POINT('Ctrl Pts',(2.80533153550818,1.25559437155609,13.3586100883147));
#12165=CARTESIAN_POINT('Ctrl Pts',(2.76592833977033,1.34363158333984,13.3635921651484));
#12166=CARTESIAN_POINT('Ctrl Pts',(2.72236039596414,1.42984925739188,13.3685742419821));
#12167=CARTESIAN_POINT('Ctrl Pts',(2.6748285498448,1.51383436311082,13.3735563188158));
#12168=CARTESIAN_POINT('Ctrl Pts',(2.62730103753478,1.597811811323,13.3785379413989));
#12169=CARTESIAN_POINT('Ctrl Pts',(2.57581055784248,1.67955671398161,13.383519563982));
#12170=CARTESIAN_POINT('Ctrl Pts',(2.52060349661509,1.75868139890425,13.3885011865651));
#12171=CARTESIAN_POINT('Ctrl Pts',(2.46538639777125,1.83782047008873,13.3934837148949));
#12172=CARTESIAN_POINT('Ctrl Pts',(2.40645162657592,1.91433801742991,13.3984662432247));
#12173=CARTESIAN_POINT('Ctrl Pts',(2.34408776827732,1.98787695409264,13.4034487715546));
#12174=CARTESIAN_POINT('Ctrl Pts',(2.28165669093055,2.06149515489106,13.4084366703156));
#12175=CARTESIAN_POINT('Ctrl Pts',(2.21578943203965,2.13212800019607,13.4134245690767));
#12176=CARTESIAN_POINT('Ctrl Pts',(2.14681344500153,2.19945317803327,13.4184124678378));
#12177=CARTESIAN_POINT('Ctrl Pts',(2.07779671290118,2.26681812577705,13.4234033130191));
#12178=CARTESIAN_POINT('Ctrl Pts',(2.00566792421392,2.33087122421097,13.4283941582004));
#12179=CARTESIAN_POINT('Ctrl Pts',(1.93078820319821,2.39132999905714,13.4333850033817));
#12180=CARTESIAN_POINT('Ctrl Pts',(1.85578747466234,2.45188647681028,13.4383839138949));
#12181=CARTESIAN_POINT('Ctrl Pts',(1.77802729086811,2.50883677345668,13.4433828244081));
#12182=CARTESIAN_POINT('Ctrl Pts',(1.69789830452451,2.56194137276652,13.4483817349212));
#12183=CARTESIAN_POINT('Ctrl Pts',(1.65137867273552,2.59277174413303,13.4512838991321));
#12184=CARTESIAN_POINT('Ctrl Pts',(1.60406112681724,2.6223067720711,13.454186063343));
#12185=CARTESIAN_POINT('Ctrl Pts',(1.55602560798144,2.65050684913395,13.4570882275538));
#12186=CARTESIAN_POINT('Ctrl Pts',(1.47327562728747,2.69908664777204,13.4620877370468));
#12187=CARTESIAN_POINT('Ctrl Pts',(1.38810309789964,2.74387282325471,13.4670872465398));
#12188=CARTESIAN_POINT('Ctrl Pts',(1.30089055399384,2.78461595494416,13.4720867560327));
#12189=CARTESIAN_POINT('Ctrl Pts',(1.21379631335012,2.82530381883416,13.4770794837228));
#12190=CARTESIAN_POINT('Ctrl Pts',(1.12466795224939,2.86195935453381,13.4820722114129));
#12191=CARTESIAN_POINT('Ctrl Pts',(1.03391473064707,2.89437775346464,13.487064939103));
#12192=CARTESIAN_POINT('Ctrl Pts',(0.943257251405859,2.92676195180178,13.4920523995912));
#12193=CARTESIAN_POINT('Ctrl Pts',(0.85097873054469,2.95491775272395,13.4970398600794));
#12194=CARTESIAN_POINT('Ctrl Pts',(0.757509709879273,2.97868784692835,13.5020273205677));
#12195=CARTESIAN_POINT('Ctrl Pts',(0.66410756848307,3.00244093307468,13.5070112124113));
#12196=CARTESIAN_POINT('Ctrl Pts',(0.56951704488257,3.02181444297084,13.511995104255));
#12197=CARTESIAN_POINT('Ctrl Pts',(0.474184261561738,3.03670076498939,13.5169789960987));
#12198=CARTESIAN_POINT('Ctrl Pts',(0.378886196079456,3.05158166577816,13.5219610729324));
#12199=CARTESIAN_POINT('Ctrl Pts',(0.282846841222,3.06197855785909,13.526943149766));
#12200=CARTESIAN_POINT('Ctrl Pts',(0.186521994656292,3.06783503394649,13.5319252265997));
#12201=CARTESIAN_POINT('Ctrl Pts',(0.0902059306974106,3.07369097605819,
13.5369068491828));
#12202=CARTESIAN_POINT('Ctrl Pts',(-0.00639513505244603,3.07500729879151,
13.5418884717659));
#12203=CARTESIAN_POINT('Ctrl Pts',(-0.102821880998386,3.07177959996937,
13.5468700943489));
#12204=CARTESIAN_POINT('Ctrl Pts',(-0.199266159025749,3.0685513142947,13.5518526226787));
#12205=CARTESIAN_POINT('Ctrl Pts',(-0.295535615593142,3.060777380984,13.5568351510086));
#12206=CARTESIAN_POINT('Ctrl Pts',(-0.391173608329201,3.04850544663229,
13.5618176793384));
#12207=CARTESIAN_POINT('Ctrl Pts',(-0.486914684726433,3.03622028494396,
13.5668055780994));
#12208=CARTESIAN_POINT('Ctrl Pts',(-0.582022502372989,3.01942749922731,
13.5717934768605));
#12209=CARTESIAN_POINT('Ctrl Pts',(-0.676048425958196,2.99822627160784,
13.5767813756215));
#12210=CARTESIAN_POINT('Ctrl Pts',(-0.770129891947036,2.97701252013221,
13.5817722208028));
#12211=CARTESIAN_POINT('Ctrl Pts',(-0.863127768351872,2.95138525807377,
13.5867630659841));
#12212=CARTESIAN_POINT('Ctrl Pts',(-0.954608503261393,2.92149360011297,
13.5917539111654));
#12213=CARTESIAN_POINT('Ctrl Pts',(-1.04623707334875,2.89155363647804,13.5967528216786));
#12214=CARTESIAN_POINT('Ctrl Pts',(-1.13634319626783,2.85733567212815,13.6017517321918));
#12215=CARTESIAN_POINT('Ctrl Pts',(-1.22451327617568,2.81903697855659,13.6067506427049));
#12216=CARTESIAN_POINT('Ctrl Pts',(-1.27570123997674,2.79680231411921,13.6096528069159));
#12217=CARTESIAN_POINT('Ctrl Pts',(-1.32623710529655,2.77319311371407,13.612554971127));
#12218=CARTESIAN_POINT('Ctrl Pts',(-1.37604412559677,2.74825486707667,13.615457135338));
#12219=CARTESIAN_POINT('Ctrl Pts',(-1.46319537732426,2.70461846005538,13.620535279788));
#12220=CARTESIAN_POINT('Ctrl Pts',(-1.54842440768503,2.65675455361347,13.6256134242381));
#12221=CARTESIAN_POINT('Ctrl Pts',(-1.63129387777118,2.60485748829879,13.6306915686881));
#12222=CARTESIAN_POINT('Ctrl Pts',(-1.71416334785733,2.55296042298411,13.6357697131381));
#12223=CARTESIAN_POINT('Ctrl Pts',(-1.79467281409763,2.49703037383199,13.6408478575881));
#12224=CARTESIAN_POINT('Ctrl Pts',(-1.87240768645124,2.43731239395329,13.6459260020382));
#12225=CARTESIAN_POINT('',(3.06928040870884,-0.00152685987410479,13.2084234471775));
#12226=CARTESIAN_POINT('Ctrl Pts',(3.06928040870884,-0.00152685987410479,
13.2084234471775));
#12227=CARTESIAN_POINT('Ctrl Pts',(3.06652007425599,0.609139336840024,13.2399450494086));
#12228=CARTESIAN_POINT('Ctrl Pts',(2.59469260810837,2.24642660009674,13.3242562875677));
#12229=CARTESIAN_POINT('Ctrl Pts',(0.302932054135814,3.43691440433902,13.4423067240563));
#12230=CARTESIAN_POINT('Ctrl Pts',(-1.34959247200755,2.82895289348612,13.5288355583138));
#12231=CARTESIAN_POINT('Ctrl Pts',(-1.87032611617489,2.43456032588397,13.5625747566432));
#12232=CARTESIAN_POINT('Ctrl Pts',(-1.87077372492565,2.43522501013474,12.5628034348477));
#12233=CARTESIAN_POINT('Ctrl Pts',(-2.41311427435265,2.01152685162279,12.5983731641431));
#12234=CARTESIAN_POINT('Ctrl Pts',(-3.42739819600353,0.513862713512807,
12.6867325293666));
#12235=CARTESIAN_POINT('Ctrl Pts',(-2.65434324796239,-2.47564042307807,
12.8278815305183));
#12236=CARTESIAN_POINT('Ctrl Pts',(0.631386762879294,-3.57430893153388,
12.9862504383024));
#12237=CARTESIAN_POINT('Ctrl Pts',(2.80237170594808,-1.84593683533756,13.1130977438555));
#12238=CARTESIAN_POINT('Ctrl Pts',(3.07114284215139,-0.413551259969408,
13.1871554134805));
#12239=CARTESIAN_POINT('Ctrl Pts',(3.06928040870884,-0.00152685987410479,
13.2084234471775));
#12240=CARTESIAN_POINT('Origin',(0.,0.,-2.20842344717744));
#12241=CARTESIAN_POINT('',(-1.87543872716782,2.44124936891338,11.5626912125175));
#12242=CARTESIAN_POINT('',(-1.87240768645122,2.43731239395331,11.6458032628636));
#12243=CARTESIAN_POINT('',(-1.87240768645123,2.4373123939533,-2.20842344717744));
#12244=CARTESIAN_POINT('',(3.0734992979985,0.00207730660589298,12.2915765528589));
#12245=CARTESIAN_POINT('Ctrl Pts',(-1.87240768645122,2.43731239395331,11.6458032628637));
#12246=CARTESIAN_POINT('Ctrl Pts',(-1.94893212434008,2.37852430176621,11.6507857245407));
#12247=CARTESIAN_POINT('Ctrl Pts',(-2.02266837301939,2.31614178282391,11.6557681862177));
#12248=CARTESIAN_POINT('Ctrl Pts',(-2.09327268938354,2.25046921727025,11.6607506478947));
#12249=CARTESIAN_POINT('Ctrl Pts',(-2.16395265244197,2.18472628898603,11.665738447868));
#12250=CARTESIAN_POINT('Ctrl Pts',(-2.23149366165016,2.1156865757866,11.6707262478412));
#12251=CARTESIAN_POINT('Ctrl Pts',(-2.29558845112282,2.04369173631239,11.6757140478144));
#12252=CARTESIAN_POINT('Ctrl Pts',(-2.35972043037824,1.97165512320162,11.6807047418638));
#12253=CARTESIAN_POINT('Ctrl Pts',(-2.42040193214456,1.89666031063711,11.6856954359131));
#12254=CARTESIAN_POINT('Ctrl Pts',(-2.47736699806578,1.81908081373383,11.6906861299624));
#12255=CARTESIAN_POINT('Ctrl Pts',(-2.53442483895091,1.74137496860452,11.6956849520013));
#12256=CARTESIAN_POINT('Ctrl Pts',(-2.58775391427102,1.66107639850951,11.7006837740402));
#12257=CARTESIAN_POINT('Ctrl Pts',(-2.63713249157206,1.5785862256763,11.7056825960791));
#12258=CARTESIAN_POINT('Ctrl Pts',(-2.66791130636354,1.52716818387506,11.7087984780287));
#12259=CARTESIAN_POINT('Ctrl Pts',(-2.69715614419527,1.47489912502561,11.7119143599783));
#12260=CARTESIAN_POINT('Ctrl Pts',(-2.72482273064765,1.42188021174286,11.7150302419279));
#12261=CARTESIAN_POINT('Ctrl Pts',(-2.76921445146487,1.33681005679142,11.7200297514209));
#12262=CARTESIAN_POINT('Ctrl Pts',(-2.80969643364756,1.24950959633874,11.7250292609139));
#12263=CARTESIAN_POINT('Ctrl Pts',(-2.84603864801091,1.16037332959193,11.7300287704068));
#12264=CARTESIAN_POINT('Ctrl Pts',(-2.88233156439122,1.071357975625,11.7350214980969));
#12265=CARTESIAN_POINT('Ctrl Pts',(-2.91449570921462,0.980512167588973,
11.740014225787));
#12266=CARTESIAN_POINT('Ctrl Pts',(-2.94234694291603,0.888254871932991,
11.7450069534771));
#12267=CARTESIAN_POINT('Ctrl Pts',(-2.97016879426799,0.79609490539819,11.7499944139653));
#12268=CARTESIAN_POINT('Ctrl Pts',(-2.99368665346054,0.702526829448481,
11.7549818744536));
#12269=CARTESIAN_POINT('Ctrl Pts',(-3.01276488262554,0.607988496616754,
11.7599693349418));
#12270=CARTESIAN_POINT('Ctrl Pts',(-3.03182946087159,0.513517808172177,
11.7649532267855));
#12271=CARTESIAN_POINT('Ctrl Pts',(-3.04646063755331,0.418078672019116,
11.7699371186292));
#12272=CARTESIAN_POINT('Ctrl Pts',(-3.05657318778469,0.322122023021898,
11.7749210104728));
#12273=CARTESIAN_POINT('Ctrl Pts',(-3.06668205527574,0.226200319059687,
11.7799030873065));
#12274=CARTESIAN_POINT('Ctrl Pts',(-3.07227551993004,0.129761912812199,
11.7848851641402));
#12275=CARTESIAN_POINT('Ctrl Pts',(-3.07331998006635,0.033264848187884,
11.7898672409739));
#12276=CARTESIAN_POINT('Ctrl Pts',(-3.07436434497196,-0.0632234181271112,
11.794848863557));
#12277=CARTESIAN_POINT('Ctrl Pts',(-3.0708605254204,-0.15976989324702,11.79983048614));
#12278=CARTESIAN_POINT('Ctrl Pts',(-3.06282703587796,-0.255915607759755,
11.8048121087231));
#12279=CARTESIAN_POINT('Ctrl Pts',(-3.05479208570558,-0.352078803257317,
11.8097946370529));
#12280=CARTESIAN_POINT('Ctrl Pts',(-3.04222586650875,-0.447840656006502,
11.8147771653827));
#12281=CARTESIAN_POINT('Ctrl Pts',(-3.02519874309449,-0.542747468699325,
11.8197596937125));
#12282=CARTESIAN_POINT('Ctrl Pts',(-3.00815326695057,-0.637756576949281,
11.8247475924736));
#12283=CARTESIAN_POINT('Ctrl Pts',(-2.98663736511198,-0.731908372459006,
11.8297354912346));
#12284=CARTESIAN_POINT('Ctrl Pts',(-2.96077247436889,-0.824759725628947,
11.8347233899957));
#12285=CARTESIAN_POINT('Ctrl Pts',(-2.93489230487979,-0.917665927367752,
11.839714235177));
#12286=CARTESIAN_POINT('Ctrl Pts',(-2.90465816868911,-1.00926974052672,
11.8447050803583));
#12287=CARTESIAN_POINT('Ctrl Pts',(-2.87024062061914,-1.09914559078762,
11.8496959255396));
#12288=CARTESIAN_POINT('Ctrl Pts',(-2.83576745292237,-1.18916668269209,
11.8546948360528));
#12289=CARTESIAN_POINT('Ctrl Pts',(-2.79709755011834,-1.27745383401603,
11.859693746566));
#12290=CARTESIAN_POINT('Ctrl Pts',(-2.75444856847886,-1.3636038037512,11.8646926570791));
#12291=CARTESIAN_POINT('Ctrl Pts',(-2.72968830365239,-1.41361897371392,
11.8675948212901));
#12292=CARTESIAN_POINT('Ctrl Pts',(-2.70358774084556,-1.46291429447049,
11.8704969855011));
#12293=CARTESIAN_POINT('Ctrl Pts',(-2.67619614131917,-1.51141538406501,
11.8733991497121));
#12294=CARTESIAN_POINT('Ctrl Pts',(-2.62900909334269,-1.59496739567366,
11.8783986592051));
#12295=CARTESIAN_POINT('Ctrl Pts',(-2.57782261901533,-1.67645424199032,
11.8833981686981));
#12296=CARTESIAN_POINT('Ctrl Pts',(-2.52284238147979,-1.75546819060027,
11.888397678191));
#12297=CARTESIAN_POINT('Ctrl Pts',(-2.46793672428747,-1.83437495729047,
11.8933904058811));
#12298=CARTESIAN_POINT('Ctrl Pts',(-2.40924778022429,-1.91081513582678,
11.8983831335712));
#12299=CARTESIAN_POINT('Ctrl Pts',(-2.34702672004189,-1.98440616442537,
11.9033758612613));
#12300=CARTESIAN_POINT('Ctrl Pts',(-2.28487130150936,-2.05791955634404,
11.9083633217495));
#12301=CARTESIAN_POINT('Ctrl Pts',(-2.21919145641302,-2.12858944021296,
11.9133507822378));
#12302=CARTESIAN_POINT('Ctrl Pts',(-2.15028060383048,-2.19606365453974,
11.918338242726));
#12303=CARTESIAN_POINT('Ctrl Pts',(-2.08141905857388,-2.26348958948883,
11.9233221345697));
#12304=CARTESIAN_POINT('Ctrl Pts',(-2.00933141444839,-2.3277240942753,11.9283060264133));
#12305=CARTESIAN_POINT('Ctrl Pts',(-1.93434951131711,-2.38845017073149,
11.933289918257));
#12306=CARTESIAN_POINT('Ctrl Pts',(-1.85939491473789,-2.44915413225461,
11.9382719950907));
#12307=CARTESIAN_POINT('Ctrl Pts',(-1.78154849414485,-2.5063519280796,11.9432540719244));
#12308=CARTESIAN_POINT('Ctrl Pts',(-1.70117615874688,-2.55976599065446,
11.9482361487581));
#12309=CARTESIAN_POINT('Ctrl Pts',(-1.62081115145419,-2.61317518309744,
11.9532177713412));
#12310=CARTESIAN_POINT('Ctrl Pts',(-1.53792105293739,-2.66280108538084,
11.9581993939242));
#12311=CARTESIAN_POINT('Ctrl Pts',(-1.45290092342857,-2.70840934068328,
11.9631810165073));
#12312=CARTESIAN_POINT('Ctrl Pts',(-1.36786533576198,-2.75402588837023,
11.9681635448371));
#12313=CARTESIAN_POINT('Ctrl Pts',(-1.28069933480257,-2.79562313087148,
11.973146073167));
#12314=CARTESIAN_POINT('Ctrl Pts',(-1.19182178858111,-2.83301307343671,
11.9781286014968));
#12315=CARTESIAN_POINT('Ctrl Pts',(-1.10284844546368,-2.87044331684947,
11.9831165002579));
#12316=CARTESIAN_POINT('Ctrl Pts',(-1.01216027941078,-2.90365703641834,
11.9881043990189));
#12317=CARTESIAN_POINT('Ctrl Pts',(-0.920195100561816,-2.93251482978382,
11.99309229778));
#12318=CARTESIAN_POINT('Ctrl Pts',(-0.828175596619435,-2.96138966984393,
11.9980831429613));
#12319=CARTESIAN_POINT('Ctrl Pts',(-0.734878002202757,-2.98590334872945,
12.0030739881426));
#12320=CARTESIAN_POINT('Ctrl Pts',(-0.640752144605902,-3.00596722190761,
12.0080648333239));
#12321=CARTESIAN_POINT('Ctrl Pts',(-0.546474177246193,-3.0260635188115,
12.0130637438371));
#12322=CARTESIAN_POINT('Ctrl Pts',(-0.451365706887995,-3.04169558002864,
12.0180626543502));
#12323=CARTESIAN_POINT('Ctrl Pts',(-0.355883472275034,-3.05282642876425,
12.0230615648634));
#12324=CARTESIAN_POINT('Ctrl Pts',(-0.300450368732202,-3.05928854701045,
12.0259637290744));
#12325=CARTESIAN_POINT('Ctrl Pts',(-0.244891341822311,-3.0642345106269,
12.0288658932853));
#12326=CARTESIAN_POINT('Ctrl Pts',(-0.189295602926492,-3.06766514220713,
12.0317680574963));
#12327=CARTESIAN_POINT('Ctrl Pts',(-0.0935217582459796,-3.07357503355216,
12.0367675669893));
#12328=CARTESIAN_POINT('Ctrl Pts',(0.00269733563998463,-3.07500585446188,
12.0417670764823));
#12329=CARTESIAN_POINT('Ctrl Pts',(0.098907702308422,-3.07190812304406,
12.0467665859752));
#12330=CARTESIAN_POINT('Ctrl Pts',(0.194987560225207,-3.06881459367924,
12.0517593136653));
#12331=CARTESIAN_POINT('Ctrl Pts',(0.291058279470483,-3.06120473470366,
12.0567520413554));
#12332=CARTESIAN_POINT('Ctrl Pts',(0.386662219863552,-3.04908093984568,
12.0617447690455));
#12333=CARTESIAN_POINT('Ctrl Pts',(0.482165300510072,-3.03696993528557,
12.0667322295338));
#12334=CARTESIAN_POINT('Ctrl Pts',(0.577202148086028,-3.0203545165175,12.071719690022));
#12335=CARTESIAN_POINT('Ctrl Pts',(0.671317619773631,-2.9992890663258,12.0767071505103));
#12336=CARTESIAN_POINT('Ctrl Pts',(0.765365749640577,-2.97823868895627,
12.081691042354));
#12337=CARTESIAN_POINT('Ctrl Pts',(0.858493387073661,-2.95274470561031,
12.0866749341976));
#12338=CARTESIAN_POINT('Ctrl Pts',(0.950253965723925,-2.92291287085776,
12.0916588260413));
#12339=CARTESIAN_POINT('Ctrl Pts',(1.04198112744419,-2.89309190012054,12.096640902875));
#12340=CARTESIAN_POINT('Ctrl Pts',(1.13234180252484,-2.85893635232281,12.1016229797087));
#12341=CARTESIAN_POINT('Ctrl Pts',(1.2209039496047,-2.8206020271991,12.1066050565424));
#12342=CARTESIAN_POINT('Ctrl Pts',(1.30945802185707,-2.78227119728267,12.1115866791254));
#12343=CARTESIAN_POINT('Ctrl Pts',(1.39621348936971,-2.73976252209484,12.1165683017085));
#12344=CARTESIAN_POINT('Ctrl Pts',(1.48075868428879,-2.69327977917322,12.1215499242916));
#12345=CARTESIAN_POINT('Ctrl Pts',(1.56531925101419,-2.6467885848698,12.1265324526214));
#12346=CARTESIAN_POINT('Ctrl Pts',(1.64766836240094,-2.59632209934946,12.1315149809513));
#12347=CARTESIAN_POINT('Ctrl Pts',(1.72742027654962,-2.54212931184966,12.1364975092811));
#12348=CARTESIAN_POINT('Ctrl Pts',(1.8072581515078,-2.48787811251195,12.1414854080421));
#12349=CARTESIAN_POINT('Ctrl Pts',(1.88449287681957,-2.42989283993656,12.1464733068032));
#12350=CARTESIAN_POINT('Ctrl Pts',(1.95876915644739,-2.36846482805855,12.1514612055642));
#12351=CARTESIAN_POINT('Ctrl Pts',(2.03308931209322,-2.30700052981066,12.1564520507456));
#12352=CARTESIAN_POINT('Ctrl Pts',(2.10444721774524,-2.2420897381237,12.1614428959269));
#12353=CARTESIAN_POINT('Ctrl Pts',(2.17252360988074,-2.17406150200742,12.1664337411082));
#12354=CARTESIAN_POINT('Ctrl Pts',(2.24071001518497,-2.10592333054375,12.1714326516213));
#12355=CARTESIAN_POINT('Ctrl Pts',(2.30560402268989,-2.03465797948364,12.1764315621345));
#12356=CARTESIAN_POINT('Ctrl Pts',(2.3669259444233,-1.96062842568802,12.1814304726477));
#12357=CARTESIAN_POINT('Ctrl Pts',(2.40252695911084,-1.91764987645977,12.1843326368586));
#12358=CARTESIAN_POINT('Ctrl Pts',(2.4369247941656,-1.87374023092778,12.1872348010695));
#12359=CARTESIAN_POINT('Ctrl Pts',(2.47007156829696,-1.82897476677263,12.1901369652805));
#12360=CARTESIAN_POINT('Ctrl Pts',(2.52743545420019,-1.75150354836614,12.195159457545));
#12361=CARTESIAN_POINT('Ctrl Pts',(2.58125253037603,-1.67119415335723,12.2001819498095));
#12362=CARTESIAN_POINT('Ctrl Pts',(2.63123135768053,-1.58840290617925,12.205204442074));
#12363=CARTESIAN_POINT('Ctrl Pts',(2.68114177306038,-1.50572498516095,12.2102200594601));
#12364=CARTESIAN_POINT('Ctrl Pts',(2.72722415798716,-1.4205723301429,12.2152356768462));
#12365=CARTESIAN_POINT('Ctrl Pts',(2.7692284194762,-1.33333274570354,12.2202512942323));
#12366=CARTESIAN_POINT('Ctrl Pts',(2.81118629016555,-1.24618951134734,12.2252613722161));
#12367=CARTESIAN_POINT('Ctrl Pts',(2.84907480323787,-1.1569643170881,12.2302714501999));
#12368=CARTESIAN_POINT('Ctrl Pts',(2.88268867979679,-1.06607139787701,12.2352815281837));
#12369=CARTESIAN_POINT('Ctrl Pts',(2.91627301188162,-0.97525836780017,12.2402872026255));
#12370=CARTESIAN_POINT('Ctrl Pts',(2.94559003048152,-0.8827809332977,12.2452928770672));
#12371=CARTESIAN_POINT('Ctrl Pts',(2.97048212200562,-0.789074275873315,
12.250298551509));
#12372=CARTESIAN_POINT('Ctrl Pts',(2.99536106342463,-0.695417122219682,
12.2553015815307));
#12373=CARTESIAN_POINT('Ctrl Pts',(3.01581961525063,-0.6005324551105,12.2603046115525));
#12374=CARTESIAN_POINT('Ctrl Pts',(3.03174994754583,-0.504870781047844,
12.2653076415742));
#12375=CARTESIAN_POINT('Ctrl Pts',(3.04767925349592,-0.409215270189403,
12.2703103492652));
#12376=CARTESIAN_POINT('Ctrl Pts',(3.05908083949576,-0.312783277793277,
12.2753130569563));
#12377=CARTESIAN_POINT('Ctrl Pts',(3.06589809758784,-0.216034962927947,
12.2803157646473));
#12378=CARTESIAN_POINT('Ctrl Pts',(3.07101317419918,-0.14344345533498,12.2840693607057));
#12379=CARTESIAN_POINT('Ctrl Pts',(3.07354846896932,-0.0706741086629879,
12.2878229567642));
#12380=CARTESIAN_POINT('Ctrl Pts',(3.07349929799898,0.00207730590177175,
12.2915765528226));
#12381=CARTESIAN_POINT('Ctrl Pts',(3.0734992979985,0.00207730660587326,
12.2915765528589));
#12382=CARTESIAN_POINT('Ctrl Pts',(3.07342502235092,0.1119725671587,12.297246578924));
#12383=CARTESIAN_POINT('Ctrl Pts',(3.06745263996488,0.221638779441771,12.3029166049891));
#12384=CARTESIAN_POINT('Ctrl Pts',(3.05567972599531,0.330490033346267,12.3085866310542));
#12385=CARTESIAN_POINT('Ctrl Pts',(3.04384899836097,0.439875826951024,12.3142845011167));
#12386=CARTESIAN_POINT('Ctrl Pts',(3.02616075202313,0.548438458326586,12.3199823711792));
#12387=CARTESIAN_POINT('Ctrl Pts',(3.00276350587142,0.6556016914307,12.3256802412417));
#12388=CARTESIAN_POINT('Ctrl Pts',(2.97923000797536,0.76338897991921,12.3314112923346));
#12389=CARTESIAN_POINT('Ctrl Pts',(2.94992093138339,0.869760348844745,12.3371423434275));
#12390=CARTESIAN_POINT('Ctrl Pts',(2.91503564058203,0.974150637292065,12.3428733945204));
#12391=CARTESIAN_POINT('Ctrl Pts',(2.90360721621096,1.00834890507739,12.3447508873685));
#12392=CARTESIAN_POINT('Ctrl Pts',(2.89158071887444,1.04233473933266,12.3466283802165));
#12393=CARTESIAN_POINT('Ctrl Pts',(2.87896424539992,1.07608880846745,12.3485058730646));
#12394=CARTESIAN_POINT('Ctrl Pts',(2.84536828312017,1.16597132878745,12.3535053825576));
#12395=CARTESIAN_POINT('Ctrl Pts',(2.8075000202345,1.25443689238546,12.3585048920505));
#12396=CARTESIAN_POINT('Ctrl Pts',(2.76549909601537,1.34105070744479,12.3635044015435));
#12397=CARTESIAN_POINT('Ctrl Pts',(2.72355514578328,1.4275470314139,12.3684971292336));
#12398=CARTESIAN_POINT('Ctrl Pts',(2.67748986552302,1.51219620745523,12.3734898569237));
#12399=CARTESIAN_POINT('Ctrl Pts',(2.62749176748801,1.59458121830867,12.3784825846138));
#12400=CARTESIAN_POINT('Ctrl Pts',(2.57754641618609,1.67687931505238,12.383470045102));
#12401=CARTESIAN_POINT('Ctrl Pts',(2.52367672164747,1.75691762180739,12.3884575055903));
#12402=CARTESIAN_POINT('Ctrl Pts',(2.4661176642449,1.83430256939777,12.3934449660785));
#12403=CARTESIAN_POINT('Ctrl Pts',(2.40859979169336,1.91163214624927,12.3984288579222));
#12404=CARTESIAN_POINT('Ctrl Pts',(2.34739806535293,1.98631178693987,12.4034127497658));
#12405=CARTESIAN_POINT('Ctrl Pts',(2.28279089484576,2.05797667149297,12.4083966416095));
#12406=CARTESIAN_POINT('Ctrl Pts',(2.21820725266996,2.12961545747004,12.4133787184432));
#12407=CARTESIAN_POINT('Ctrl Pts',(2.15022092405051,2.19824134301797,12.4183607952769));
#12408=CARTESIAN_POINT('Ctrl Pts',(2.07915011426217,2.26352315039268,12.4233428721106));
#12409=CARTESIAN_POINT('Ctrl Pts',(2.00808578449422,2.32879900557064,12.4283244946937));
#12410=CARTESIAN_POINT('Ctrl Pts',(1.93393785610592,2.3907310919662,12.4333061172767));
#12411=CARTESIAN_POINT('Ctrl Pts',(1.85706006057644,2.44902637417645,12.4382877398598));
#12412=CARTESIAN_POINT('Ctrl Pts',(1.78016828730922,2.50733225549611,12.4432702681896));
#12413=CARTESIAN_POINT('Ctrl Pts',(1.70054601096471,2.56199975421922,12.4482527965195));
#12414=CARTESIAN_POINT('Ctrl Pts',(1.61857770211763,2.61277792248167,12.4532353248493));
#12415=CARTESIAN_POINT('Ctrl Pts',(1.53652104351402,2.66361082212586,12.4582232236103));
#12416=CARTESIAN_POINT('Ctrl Pts',(1.4521136779172,2.71054579056773,12.4632111223714));
#12417=CARTESIAN_POINT('Ctrl Pts',(1.36576635612441,2.75337692851499,12.4681990211324));
#12418=CARTESIAN_POINT('Ctrl Pts',(1.27936802778348,2.79623336740332,12.4731898663138));
#12419=CARTESIAN_POINT('Ctrl Pts',(1.19102786326098,2.83498097260127,12.4781807114951));
#12420=CARTESIAN_POINT('Ctrl Pts',(1.10117639047012,2.8694621111057,12.4831715566764));
#12421=CARTESIAN_POINT('Ctrl Pts',(1.01117971543017,2.90399897200073,12.4881704671895));
#12422=CARTESIAN_POINT('Ctrl Pts',(0.919667271856441,2.93425546127061,12.4931693777027));
#12423=CARTESIAN_POINT('Ctrl Pts',(0.827084463137039,2.96012390633185,12.4981682882159));
#12424=CARTESIAN_POINT('Ctrl Pts',(0.773334648390229,2.97514207384115,12.5010704524268));
#12425=CARTESIAN_POINT('Ctrl Pts',(0.719224272795122,2.98868220974375,12.5039726166378));
#12426=CARTESIAN_POINT('Ctrl Pts',(0.664841586868226,3.00073122994555,12.5068747808488));
#12427=CARTESIAN_POINT('Ctrl Pts',(0.571149478699316,3.02148964017917,12.5118747156359));
#12428=CARTESIAN_POINT('Ctrl Pts',(0.476319648394481,3.03789227164926,12.5168746504229));
#12429=CARTESIAN_POINT('Ctrl Pts',(0.38079293596222,3.04981950120352,12.52187458521));
#12430=CARTESIAN_POINT('Ctrl Pts',(0.282176421702118,3.06213251578836,12.5270362423808));
#12431=CARTESIAN_POINT('Ctrl Pts',(0.182817606641743,3.06967548974739,12.5321978995516));
#12432=CARTESIAN_POINT('Ctrl Pts',(0.0832165932657832,3.07237322742619,
12.5373595567224));
#12433=CARTESIAN_POINT('Ctrl Pts',(-0.0130116700547539,3.07497961267195,
12.5423464267206));
#12434=CARTESIAN_POINT('Ctrl Pts',(-0.109465510670845,3.07306357916795,
12.5473332967189));
#12435=CARTESIAN_POINT('Ctrl Pts',(-0.205686907854918,3.06660971529425,
12.5523201667172));
#12436=CARTESIAN_POINT('Ctrl Pts',(-0.30184492868777,3.06016010226657,12.5573037521069));
#12437=CARTESIAN_POINT('Ctrl Pts',(-0.397770373701489,3.04917862723745,
12.5622873374966));
#12438=CARTESIAN_POINT('Ctrl Pts',(-0.49300583624215,3.03370194571437,12.5672709228863));
#12439=CARTESIAN_POINT('Ctrl Pts',(-0.588204571716693,3.01823123269389,
12.5722525863819));
#12440=CARTESIAN_POINT('Ctrl Pts',(-0.682713420992185,2.99826882989282,
12.5772342498776));
#12441=CARTESIAN_POINT('Ctrl Pts',(-0.776081777843846,2.97390304551085,
12.5822159133732));
#12442=CARTESIAN_POINT('Ctrl Pts',(-0.869439616633389,2.94954000596496,
12.5871970156782));
#12443=CARTESIAN_POINT('Ctrl Pts',(-0.96165679443306,2.92077468393078,12.5921781179832));
#12444=CARTESIAN_POINT('Ctrl Pts',(-1.05229559545297,2.88774587347818,12.5971592202883));
#12445=CARTESIAN_POINT('Ctrl Pts',(-1.14298524824181,2.85469853262339,12.6021431171786));
#12446=CARTESIAN_POINT('Ctrl Pts',(-1.23209434306856,2.81738307702337,12.607127014069));
#12447=CARTESIAN_POINT('Ctrl Pts',(-1.31920345658343,2.77598711995181,12.6121109109593));
#12448=CARTESIAN_POINT('Ctrl Pts',(-1.4063423521144,2.73457700988281,12.6170965118103));
#12449=CARTESIAN_POINT('Ctrl Pts',(-1.49147951532831,2.68908382281959,12.6220821126612));
#12450=CARTESIAN_POINT('Ctrl Pts',(-1.57422008596841,2.639741156048,12.6270677135122));
#12451=CARTESIAN_POINT('Ctrl Pts',(-1.65704779881578,2.59034652167621,12.6320585651882));
#12452=CARTESIAN_POINT('Ctrl Pts',(-1.7374735140984,2.53709455552647,12.6370494168642));
#12453=CARTESIAN_POINT('Ctrl Pts',(-1.81513171210194,2.48026190506605,12.6420402685402));
#12454=CARTESIAN_POINT('Ctrl Pts',(-1.83439558793767,2.46616401005907,12.6432782981298));
#12455=CARTESIAN_POINT('Ctrl Pts',(-1.85348932959634,2.45184597482623,12.6445163277194));
#12456=CARTESIAN_POINT('Ctrl Pts',(-1.87240768645123,2.43731239395329,12.6457543573089));
#12457=CARTESIAN_POINT('',(3.07749897857868,-0.00155006825877461,12.2084234471775));
#12458=CARTESIAN_POINT('Ctrl Pts',(3.07749897857868,-0.00155006825877461,
12.2084234471775));
#12459=CARTESIAN_POINT('Ctrl Pts',(3.07177196381206,0.924255192727474,12.2565405671735));
#12460=CARTESIAN_POINT('Ctrl Pts',(2.13549779090968,2.87581154197502,12.3574473230977));
#12461=CARTESIAN_POINT('Ctrl Pts',(-0.413050570340105,3.30353187187741,
12.4755739856545));
#12462=CARTESIAN_POINT('Ctrl Pts',(-1.60821750621956,2.64034444383588,12.5455835282151));
#12463=CARTESIAN_POINT('Ctrl Pts',(-1.87077372492565,2.43522501013474,12.5628034348477));
#12464=CARTESIAN_POINT('Ctrl Pts',(-1.87543872716782,2.44124936891338,11.5626912125175));
#12465=CARTESIAN_POINT('Ctrl Pts',(-2.67063619912824,1.82902599129973,11.6148938670213));
#12466=CARTESIAN_POINT('Ctrl Pts',(-3.61429065672828,-0.258675541093378,
11.7198861574532));
#12467=CARTESIAN_POINT('Ctrl Pts',(-1.76367158133378,-3.17234867812122,
11.8776680838132));
#12468=CARTESIAN_POINT('Ctrl Pts',(1.70070785150167,-3.20654430598149,12.0360369915973));
#12469=CARTESIAN_POINT('Ctrl Pts',(3.03378404611734,-1.1965068427,12.1462887793855));
#12470=CARTESIAN_POINT('Ctrl Pts',(3.07805511260628,-0.0914523698142579,
12.2037509312455));
#12471=CARTESIAN_POINT('Ctrl Pts',(3.07749897857868,-0.00155006825877461,
12.2084234471775));
#12472=CARTESIAN_POINT('Origin',(0.,0.,-2.20842344717744));
#12473=CARTESIAN_POINT('',(-1.87115843792479,2.43565187781327,10.5625482443637));
#12474=CARTESIAN_POINT('',(-1.87240768645123,2.4373123939533,10.6459243044939));
#12475=CARTESIAN_POINT('',(-1.87240768645123,2.4373123939533,-2.20842344717744));
#12476=CARTESIAN_POINT('',(3.07349905914928,-0.00240487182579642,11.2915765527899));
#12477=CARTESIAN_POINT('Ctrl Pts',(-1.87240768645123,2.4373123939533,10.6459243044939));
#12478=CARTESIAN_POINT('Ctrl Pts',(-1.94880420429965,2.37862257331628,10.6509091987637));
#12479=CARTESIAN_POINT('Ctrl Pts',(-2.02250521179709,2.3162862646041,10.6558940930335));
#12480=CARTESIAN_POINT('Ctrl Pts',(-2.09314840489398,2.2505848140183,10.6608789873033));
#12481=CARTESIAN_POINT('Ctrl Pts',(-2.16375882816078,2.18491384089648,10.6658615691898));
#12482=CARTESIAN_POINT('Ctrl Pts',(-2.23131393414587,2.11588112560119,10.6708441510764));
#12483=CARTESIAN_POINT('Ctrl Pts',(-2.2954853084557,2.04380758601783,10.6758267329629));
#12484=CARTESIAN_POINT('Ctrl Pts',(-2.35964443383017,1.97174780372324,10.6808083637817));
#12485=CARTESIAN_POINT('Ctrl Pts',(-2.42042081939891,1.89664867850762,10.6857899946005));
#12486=CARTESIAN_POINT('Ctrl Pts',(-2.47752441800935,1.81886640745478,10.6907716254193));
#12487=CARTESIAN_POINT('Ctrl Pts',(-2.53463270582119,1.74107774912086,10.6957536653168));
#12488=CARTESIAN_POINT('Ctrl Pts',(-2.58806734829466,1.6606058615445,10.7007357052144));
#12489=CARTESIAN_POINT('Ctrl Pts',(-2.63758058586237,1.57783741338641,10.705717745112));
#12490=CARTESIAN_POINT('Ctrl Pts',(-2.6871443911959,1.49498443398558,10.7107048731564));
#12491=CARTESIAN_POINT('Ctrl Pts',(-2.73277856605105,1.40983058652907,10.7156920012009));
#12492=CARTESIAN_POINT('Ctrl Pts',(-2.77428055371357,1.32278859206101,10.7206791292454));
#12493=CARTESIAN_POINT('Ctrl Pts',(-2.81580334639611,1.23570296328675,10.725668757346));
#12494=CARTESIAN_POINT('Ctrl Pts',(-2.85318965513954,1.14672770694656,10.7306583854466));
#12495=CARTESIAN_POINT('Ctrl Pts',(-2.88628533694828,1.05629503630253,10.7356480135472));
#12496=CARTESIAN_POINT('Ctrl Pts',(-2.91943817036192,0.96570620110831,10.7406462580364));
#12497=CARTESIAN_POINT('Ctrl Pts',(-2.94828543995732,0.873655342310838,
10.7456445025256));
#12498=CARTESIAN_POINT('Ctrl Pts',(-2.97272303537711,0.780589523974215,
10.7506427470147));
#12499=CARTESIAN_POINT('Ctrl Pts',(-2.99582312290602,0.692617343708724,
10.7553674297508));
#12500=CARTESIAN_POINT('Ctrl Pts',(-3.0149834079316,0.603738674301219,10.7600921124868));
#12501=CARTESIAN_POINT('Ctrl Pts',(-3.03015849914791,0.51433619359491,10.7648167952229));
#12502=CARTESIAN_POINT('Ctrl Pts',(-3.04621629960373,0.419733322681323,
10.7698163047159));
#12503=CARTESIAN_POINT('Ctrl Pts',(-3.05786774372333,0.324211570568965,
10.7748158142088));
#12504=CARTESIAN_POINT('Ctrl Pts',(-3.06501536928884,0.228217080918975,
10.7798153237018));
#12505=CARTESIAN_POINT('Ctrl Pts',(-3.07215329914568,0.132352807184427,
10.7848080513919));
#12506=CARTESIAN_POINT('Ctrl Pts',(-3.07479952016354,0.0360175043909558,
10.789800779082));
#12507=CARTESIAN_POINT('Ctrl Pts',(-3.07290776230443,-0.0603335260793813,
10.7947935067721));
#12508=CARTESIAN_POINT('Ctrl Pts',(-3.07101800020218,-0.156582908641232,
10.7997809672603));
#12509=CARTESIAN_POINT('Ctrl Pts',(-3.06459978496209,-0.252847549351398,
10.8047684277486));
#12510=CARTESIAN_POINT('Ctrl Pts',(-3.05365880648686,-0.348669103255899,
10.8097558882368));
#12511=CARTESIAN_POINT('Ctrl Pts',(-3.04272565653749,-0.444422094598561,
10.8147397800805));
#12512=CARTESIAN_POINT('Ctrl Pts',(-3.02727622630673,-0.53973219451599,
10.8197236719241));
#12513=CARTESIAN_POINT('Ctrl Pts',(-3.00736819811476,-0.6341441247603,10.8247075637678));
#12514=CARTESIAN_POINT('Ctrl Pts',(-2.98746741993359,-0.728521672517914,
10.8296896406015));
#12515=CARTESIAN_POINT('Ctrl Pts',(-2.9631113604055,-0.822001271418687,
10.8346717174352));
#12516=CARTESIAN_POINT('Ctrl Pts',(-2.93440900753201,-0.914136765760458,
10.8396537942689));
#12517=CARTESIAN_POINT('Ctrl Pts',(-2.90570927165185,-1.0062638594678,10.8446354168519));
#12518=CARTESIAN_POINT('Ctrl Pts',(-2.87266416104143,-1.09704667322843,
10.849617039435));
#12519=CARTESIAN_POINT('Ctrl Pts',(-2.83543253547355,-1.18605420903854,
10.8545986620181));
#12520=CARTESIAN_POINT('Ctrl Pts',(-2.79819414053999,-1.27507792798728,
10.8595811903479));
#12521=CARTESIAN_POINT('Ctrl Pts',(-2.75676788836516,-1.36232532300698,
10.8645637186778));
#12522=CARTESIAN_POINT('Ctrl Pts',(-2.71136035032648,-1.44738636883089,
10.8695462470076));
#12523=CARTESIAN_POINT('Ctrl Pts',(-2.66590386965403,-1.53253909792575,
10.8745341457687));
#12524=CARTESIAN_POINT('Ctrl Pts',(-2.61645774311551,-1.615500385283,10.8795220445297));
#12525=CARTESIAN_POINT('Ctrl Pts',(-2.56327388343319,-1.69588597744935,
10.8845099432908));
#12526=CARTESIAN_POINT('Ctrl Pts',(-2.51005860731485,-1.77631905448852,
10.8895007884721));
#12527=CARTESIAN_POINT('Ctrl Pts',(-2.45310146076598,-1.85417305267419,
10.8944916336534));
#12528=CARTESIAN_POINT('Ctrl Pts',(-2.39269568836348,-1.92909553752187,
10.8994824788347));
#12529=CARTESIAN_POINT('Ctrl Pts',(-2.33219229870749,-2.00413909899692,
10.9044813893479));
#12530=CARTESIAN_POINT('Ctrl Pts',(-2.26822944612432,-2.07624135944133,
10.909480299861));
#12531=CARTESIAN_POINT('Ctrl Pts',(-2.20113831793107,-2.14508562890519,
10.9144792103742));
#12532=CARTESIAN_POINT('Ctrl Pts',(-2.16218793652258,-2.18505381286063,
10.9173813745851));
#12533=CARTESIAN_POINT('Ctrl Pts',(-2.12218382895313,-2.22392461687581,
10.9202835387961));
#12534=CARTESIAN_POINT('Ctrl Pts',(-2.08119575623373,-2.26164242846537,
10.923185703007));
#12535=CARTESIAN_POINT('Ctrl Pts',(-2.01058629248023,-2.32661826835241,
10.9281852125));
#12536=CARTESIAN_POINT('Ctrl Pts',(-1.93680703068045,-2.38839837684194,
10.933184721993));
#12537=CARTESIAN_POINT('Ctrl Pts',(-1.86017912923878,-2.44665809976475,
10.9381842314859));
#12538=CARTESIAN_POINT('Ctrl Pts',(-1.78365517305884,-2.50483879374337,
10.943176959176));
#12539=CARTESIAN_POINT('Ctrl Pts',(-1.70429060344906,-2.559508329507,10.9481696868661));
#12540=CARTESIAN_POINT('Ctrl Pts',(-1.62244213190176,-2.61038000655653,
10.9531624145562));
#12541=CARTESIAN_POINT('Ctrl Pts',(-1.54068000842828,-2.66119801526942,
10.9581498750445));
#12542=CARTESIAN_POINT('Ctrl Pts',(-1.45643956315769,-2.7082258997491,10.9631373355327));
#12543=CARTESIAN_POINT('Ctrl Pts',(-1.37010835017776,-2.75121888601637,
10.968124796021));
#12544=CARTESIAN_POINT('Ctrl Pts',(-1.28383890919933,-2.79418110979671,
10.9731086878647));
#12545=CARTESIAN_POINT('Ctrl Pts',(-1.19548206628226,-2.83311397959144,
10.9780925797083));
#12546=CARTESIAN_POINT('Ctrl Pts',(-1.10545111053776,-2.86781800193297,
10.983076471552));
#12547=CARTESIAN_POINT('Ctrl Pts',(-1.01545294183751,-2.9025093859291,10.9880585483857));
#12548=CARTESIAN_POINT('Ctrl Pts',(-0.923782280826665,-2.93297482464626,
10.9930406252194));
#12549=CARTESIAN_POINT('Ctrl Pts',(-0.83087269815376,-2.95906282621081,
10.9980227020531));
#12550=CARTESIAN_POINT('Ctrl Pts',(-0.737971586694155,-2.98514844915068,
11.0030043246362));
#12551=CARTESIAN_POINT('Ctrl Pts',(-0.643832200827791,-3.0068573099751,
11.0079859472193));
#12552=CARTESIAN_POINT('Ctrl Pts',(-0.54890254980647,-3.02408800149995,
11.0129675698023));
#12553=CARTESIAN_POINT('Ctrl Pts',(-0.45395563890225,-3.04132182586806,
11.0179500981321));
#12554=CARTESIAN_POINT('Ctrl Pts',(-0.358218609393281,-3.05407578555472,
11.022932626462));
#12555=CARTESIAN_POINT('Ctrl Pts',(-0.262147855418949,-3.06229991214108,
11.0279151547918));
#12556=CARTESIAN_POINT('Ctrl Pts',(-0.165973551330405,-3.07053290312386,
11.0329030535528));
#12557=CARTESIAN_POINT('Ctrl Pts',(-0.069465242745026,-3.07422627605858,
11.0378909523139));
#12558=CARTESIAN_POINT('Ctrl Pts',(0.0269176072301352,-3.07338212600077,
11.042878851075));
#12559=CARTESIAN_POINT('Ctrl Pts',(0.123357391877683,-3.07253747729193,
11.0478696962563));
#12560=CARTESIAN_POINT('Ctrl Pts',(0.219671132277135,-3.06714999302599,
11.0528605414376));
#12561=CARTESIAN_POINT('Ctrl Pts',(0.315403551634229,-3.0572737609865,11.0578513866189));
#12562=CARTESIAN_POINT('Ctrl Pts',(0.411290676998466,-3.04738156870663,
11.062850297132));
#12563=CARTESIAN_POINT('Ctrl Pts',(0.506594171740867,-3.03298620967495,
11.0678492076452));
#12564=CARTESIAN_POINT('Ctrl Pts',(0.600868083322849,-3.0141930589204,11.0728481181584));
#12565=CARTESIAN_POINT('Ctrl Pts',(0.655599683638426,-3.00328251963643,
11.0757502823693));
#12566=CARTESIAN_POINT('Ctrl Pts',(0.709984512979423,-2.99089065275642,
11.0786524465803));
#12567=CARTESIAN_POINT('Ctrl Pts',(0.763937942530848,-2.97704569497375,
11.0815546107912));
#12568=CARTESIAN_POINT('Ctrl Pts',(0.85688260851611,-2.9531952189727,11.0865541202842));
#12569=CARTESIAN_POINT('Ctrl Pts',(0.948872521154095,-2.92494601987679,
11.0915536297772));
#12570=CARTESIAN_POINT('Ctrl Pts',(1.03946050783772,-2.89239072440875,11.0965531392701));
#12571=CARTESIAN_POINT('Ctrl Pts',(1.12992561249269,-2.85987958999226,11.1015458669602));
#12572=CARTESIAN_POINT('Ctrl Pts',(1.21899216114105,-2.82307411537443,11.1065385946503));
#12573=CARTESIAN_POINT('Ctrl Pts',(1.30622545948717,-2.78211741286875,11.1115313223404));
#12574=CARTESIAN_POINT('Ctrl Pts',(1.39336672890235,-2.74120391865186,11.1165187828287));
#12575=CARTESIAN_POINT('Ctrl Pts',(1.47867819752203,-2.6961480881761,11.1215062433169));
#12576=CARTESIAN_POINT('Ctrl Pts',(1.5617435463928,-2.64714173124531,11.1264937038051));
#12577=CARTESIAN_POINT('Ctrl Pts',(1.64474946006468,-2.59817043950851,11.1314775956488));
#12578=CARTESIAN_POINT('Ctrl Pts',(1.72551207194317,-2.54525446306206,11.1364614874925));
#12579=CARTESIAN_POINT('Ctrl Pts',(1.80363903254495,-2.48863185109415,11.1414453793361));
#12580=CARTESIAN_POINT('Ctrl Pts',(1.88173754124274,-2.43202985967909,11.1464274561698));
#12581=CARTESIAN_POINT('Ctrl Pts',(1.95720195069225,-2.37172417211289,11.1514095330035));
#12582=CARTESIAN_POINT('Ctrl Pts',(2.02966913246219,-2.3079959841235,11.1563916098372));
#12583=CARTESIAN_POINT('Ctrl Pts',(2.10212970689451,-2.24427360667681,11.1613732324203));
#12584=CARTESIAN_POINT('Ctrl Pts',(2.17159326746409,-2.17712963924476,11.1663548550033));
#12585=CARTESIAN_POINT('Ctrl Pts',(2.23773083527072,-2.10688465723176,11.1713364775864));
#12586=CARTESIAN_POINT('Ctrl Pts',(2.30388042805232,-2.03662690344354,11.1763190059162));
#12587=CARTESIAN_POINT('Ctrl Pts',(2.36670252620823,-1.96326733494622,11.181301534246));
#12588=CARTESIAN_POINT('Ctrl Pts',(2.4259067321126,-1.8871615662393,11.1862840625758));
#12589=CARTESIAN_POINT('Ctrl Pts',(2.48517475142586,-1.81097376672962,11.1912719613369));
#12590=CARTESIAN_POINT('Ctrl Pts',(2.54081682341243,-1.73203420469199,11.1962598600979));
#12591=CARTESIAN_POINT('Ctrl Pts',(2.59258454998284,-1.65072941489217,11.201247758859));
#12592=CARTESIAN_POINT('Ctrl Pts',(2.6443828564599,-1.56937659723704,11.2062386040403));
#12593=CARTESIAN_POINT('Ctrl Pts',(2.69230204253117,-1.48565615061418,11.2112294492216));
#12594=CARTESIAN_POINT('Ctrl Pts',(2.73613960045087,-1.39997940586444,11.2162202944029));
#12595=CARTESIAN_POINT('Ctrl Pts',(2.78004800097113,-1.31416420533171,11.2212192049161));
#12596=CARTESIAN_POINT('Ctrl Pts',(2.81986142135796,-1.22638679349434,11.2262181154292));
#12597=CARTESIAN_POINT('Ctrl Pts',(2.85542544981688,-1.13707860350023,11.2312170259424));
#12598=CARTESIAN_POINT('Ctrl Pts',(2.87607247886868,-1.08522989925399,11.2341191901534));
#12599=CARTESIAN_POINT('Ctrl Pts',(2.89528818176261,-1.03286555270386,11.2370213543644));
#12600=CARTESIAN_POINT('Ctrl Pts',(2.9130501669288,-0.980071923358748,11.2399235185754));
#12601=CARTESIAN_POINT('Ctrl Pts',(2.94920738770405,-0.872602465756003,
11.24583131498));
#12602=CARTESIAN_POINT('Ctrl Pts',(2.97944169451371,-0.763046477916852,
11.2517391113846));
#12603=CARTESIAN_POINT('Ctrl Pts',(3.00354581196166,-0.652008286333519,
11.2576469077892));
#12604=CARTESIAN_POINT('Ctrl Pts',(3.02740835185802,-0.542082947544464,
11.2634954947664));
#12605=CARTESIAN_POINT('Ctrl Pts',(3.04526290787206,-0.430705059009903,
11.2693440817437));
#12606=CARTESIAN_POINT('Ctrl Pts',(3.05695463632113,-0.318481712936139,
11.2751926687209));
#12607=CARTESIAN_POINT('Ctrl Pts',(3.0678721407953,-0.213689774925965,11.2806539634106));
#12608=CARTESIAN_POINT('Ctrl Pts',(3.07341630993048,-0.108160880684027,
11.2861152581002));
#12609=CARTESIAN_POINT('Ctrl Pts',(3.07349905914928,-0.00240487182581181,
11.2915765527899));
#12610=CARTESIAN_POINT('Ctrl Pts',(3.07349905914977,-0.00240487119193424,
11.2915765528226));
#12611=CARTESIAN_POINT('Ctrl Pts',(3.07357440903969,0.0938945965502631,
11.2965495068653));
#12612=CARTESIAN_POINT('Ctrl Pts',(3.06911954638383,0.19025278966347,11.301522460908));
#12613=CARTESIAN_POINT('Ctrl Pts',(3.0601446217697,0.286211711594748,11.3064954149507));
#12614=CARTESIAN_POINT('Ctrl Pts',(3.05117154752427,0.382150849584164,11.3114673437147));
#12615=CARTESIAN_POINT('Ctrl Pts',(3.03768030403397,0.477690441648078,11.3164392724788));
#12616=CARTESIAN_POINT('Ctrl Pts',(3.01973301736176,0.572376409240685,11.3214112012428));
#12617=CARTESIAN_POINT('Ctrl Pts',(3.0017844941583,0.667068900502275,11.3263834725626));
#12618=CARTESIAN_POINT('Ctrl Pts',(2.97937940044349,0.760907217840555,11.3313557438823));
#12619=CARTESIAN_POINT('Ctrl Pts',(2.95263100332818,0.853447366968359,11.3363280152021));
#12620=CARTESIAN_POINT('Ctrl Pts',(2.92485280817899,0.949550259060418,11.3414917161319));
#12621=CARTESIAN_POINT('Ctrl Pts',(2.89239026140698,1.04425251028761,11.3466554170616));
#12622=CARTESIAN_POINT('Ctrl Pts',(2.85542656316388,1.1370758076655,11.3518191179914));
#12623=CARTESIAN_POINT('Ctrl Pts',(2.81977708586466,1.22659883133449,11.3567992267962));
#12624=CARTESIAN_POINT('Ctrl Pts',(2.77994134730084,1.31437386440542,11.3617793356009));
#12625=CARTESIAN_POINT('Ctrl Pts',(2.73613155296547,1.39999513387254,11.3667594444057));
#12626=CARTESIAN_POINT('Ctrl Pts',(2.69228901873109,1.48568038975541,11.3717432749412));
#12627=CARTESIAN_POINT('Ctrl Pts',(2.64446673693219,1.56920829804497,11.3767271054767));
#12628=CARTESIAN_POINT('Ctrl Pts',(2.59292101568734,1.65020085335298,11.3817109360122));
#12629=CARTESIAN_POINT('Ctrl Pts',(2.5412957660873,1.73131836965778,11.3867024559512));
#12630=CARTESIAN_POINT('Ctrl Pts',(2.4859358713261,1.80989237280952,11.3916939758901));
#12631=CARTESIAN_POINT('Ctrl Pts',(2.42713849798068,1.885577089811,11.396685495829));
#12632=CARTESIAN_POINT('Ctrl Pts',(2.42082891055362,1.89369886994575,11.3972211393392));
#12633=CARTESIAN_POINT('Ctrl Pts',(2.41447977355891,1.90178741316436,11.3977567828494));
#12634=CARTESIAN_POINT('Ctrl Pts',(2.40809147900629,1.90984231776796,11.3982924263596));
#12635=CARTESIAN_POINT('Ctrl Pts',(2.34846536825864,1.98502398479978,11.4032919358526));
#12636=CARTESIAN_POINT('Ctrl Pts',(2.28521034726906,2.05754269684224,11.4082914453455));
#12637=CARTESIAN_POINT('Ctrl Pts',(2.21859308199777,2.12702773524739,11.4132909548385));
#12638=CARTESIAN_POINT('Ctrl Pts',(2.15206618262392,2.19641851763906,11.4182836825286));
#12639=CARTESIAN_POINT('Ctrl Pts',(2.08218640456877,2.26278349084693,11.4232764102187));
#12640=CARTESIAN_POINT('Ctrl Pts',(2.00926144500829,2.32578388841337,11.4282691379088));
#12641=CARTESIAN_POINT('Ctrl Pts',(1.93641341944198,2.38871782214838,11.433256598397));
#12642=CARTESIAN_POINT('Ctrl Pts',(1.86052692921064,2.4482939510779,11.4382440588852));
#12643=CARTESIAN_POINT('Ctrl Pts',(1.78194666857371,2.50421011905133,11.4432315193734));
#12644=CARTESIAN_POINT('Ctrl Pts',(1.70342263394998,2.5600862776996,11.4482154112171));
#12645=CARTESIAN_POINT('Ctrl Pts',(1.62220901724139,2.61230742764699,11.4531993030607));
#12646=CARTESIAN_POINT('Ctrl Pts',(1.53868298702528,2.66061213171687,11.4581831949044));
#12647=CARTESIAN_POINT('Ctrl Pts',(1.45518737492063,2.7088992444099,11.4631652717381));
#12648=CARTESIAN_POINT('Ctrl Pts',(1.36938140212152,2.75327252554152,11.4681473485718));
#12649=CARTESIAN_POINT('Ctrl Pts',(1.28166974847641,2.79351479427628,11.4731294254055));
#12650=CARTESIAN_POINT('Ctrl Pts',(1.19396609211332,2.83375339384326,11.4781110479886));
#12651=CARTESIAN_POINT('Ctrl Pts',(1.10435749941049,2.86986154698606,11.4830926705716));
#12652=CARTESIAN_POINT('Ctrl Pts',(1.01327071436631,2.90166929704396,11.4880742931547));
#12653=CARTESIAN_POINT('Ctrl Pts',(0.922167368139779,2.93348283031123,11.4930568214845));
#12654=CARTESIAN_POINT('Ctrl Pts',(0.829585710239929,2.96099426297874,11.4980393498143));
#12655=CARTESIAN_POINT('Ctrl Pts',(0.735968779924244,2.98408314310725,11.5030218781442));
#12656=CARTESIAN_POINT('Ctrl Pts',(0.642250944354815,3.00719690964572,11.5080097769052));
#12657=CARTESIAN_POINT('Ctrl Pts',(0.547496035534339,3.02587850176322,11.5129976756662));
#12658=CARTESIAN_POINT('Ctrl Pts',(0.452158234263065,3.04005841739729,11.5179855744273));
#12659=CARTESIAN_POINT('Ctrl Pts',(0.35676411564386,3.05424670930218,11.5229764196086));
#12660=CARTESIAN_POINT('Ctrl Pts',(0.260786855513396,3.0639279857834,11.5279672647899));
#12661=CARTESIAN_POINT('Ctrl Pts',(0.16468459847902,3.06908475494304,11.5329581099712));
#12662=CARTESIAN_POINT('Ctrl Pts',(0.068427037770403,3.07424985757188,11.5379570204844));
#12663=CARTESIAN_POINT('Ctrl Pts',(-0.0279554845304961,3.074875850145,11.5429559309975));
#12664=CARTESIAN_POINT('Ctrl Pts',(-0.124006045127911,3.0709973544065,11.5479548415107));
#12665=CARTESIAN_POINT('Ctrl Pts',(-0.179769095632414,3.0687456574627,11.5508570057217));
#12666=CARTESIAN_POINT('Ctrl Pts',(-0.235420357734087,3.06497669821172,
11.5537591699327));
#12667=CARTESIAN_POINT('Ctrl Pts',(-0.290871837190708,3.05970518585195,
11.5566613341437));
#12668=CARTESIAN_POINT('Ctrl Pts',(-0.386389650552053,3.05062475484006,
11.5616604501667));
#12669=CARTESIAN_POINT('Ctrl Pts',(-0.481649604251123,3.03705127990046,
11.5666595661897));
#12670=CARTESIAN_POINT('Ctrl Pts',(-0.576195663337729,3.01900659282997,
11.5716586822127));
#12671=CARTESIAN_POINT('Ctrl Pts',(-0.670619513877616,3.00098522999957,
11.5766513364677));
#12672=CARTESIAN_POINT('Ctrl Pts',(-0.764330875845443,2.97850421941971,
11.5816439907226));
#12673=CARTESIAN_POINT('Ctrl Pts',(-0.856878087759706,2.95163720547043,
11.5866366449776));
#12674=CARTESIAN_POINT('Ctrl Pts',(-0.949320804020787,2.92480052723968,
11.5916236619945));
#12675=CARTESIAN_POINT('Ctrl Pts',(-1.04060156506698,2.89358781598924,11.5966106790113));
#12676=CARTESIAN_POINT('Ctrl Pts',(-1.13027937124325,2.85812364899456,11.6015976960282));
#12677=CARTESIAN_POINT('Ctrl Pts',(-1.21989648872633,2.82268348207349,11.6065813381237));
#12678=CARTESIAN_POINT('Ctrl Pts',(-1.30791240017554,2.78299773785967,11.6115649802192));
#12679=CARTESIAN_POINT('Ctrl Pts',(-1.39390252402616,2.73924040630126,11.6165486223146));
#12680=CARTESIAN_POINT('Ctrl Pts',(-1.47987428012675,2.69549242144097,11.6215311998891));
#12681=CARTESIAN_POINT('Ctrl Pts',(-1.56382071308338,2.64767476729304,11.6265137774636));
#12682=CARTESIAN_POINT('Ctrl Pts',(-1.64533919886181,2.59600870004104,11.6314963550381));
#12683=CARTESIAN_POINT('Ctrl Pts',(-1.72336290210065,2.54655761099916,11.6362653243133));
#12684=CARTESIAN_POINT('Ctrl Pts',(-1.79916222732898,2.49358148814015,11.6410342935885));
#12685=CARTESIAN_POINT('Ctrl Pts',(-1.87240768645122,2.43731239395331,11.6458032628637));
#12686=CARTESIAN_POINT('',(3.07371628270923,0.00276101913198965,11.2084234471775));
#12687=CARTESIAN_POINT('Ctrl Pts',(3.07371628270923,0.00276101913198965,
11.2084234471775));
#12688=CARTESIAN_POINT('Ctrl Pts',(3.07581988160793,0.232901496003139,11.2203464490105));
#12689=CARTESIAN_POINT('Ctrl Pts',(2.94733814809347,1.47967347839142,11.2850590867715));
#12690=CARTESIAN_POINT('Ctrl Pts',(1.2479789847658,3.4083547403351,11.4025613604607));
#12691=CARTESIAN_POINT('Ctrl Pts',(-1.04966881457196,3.06922939603839,11.508727613741));
#12692=CARTESIAN_POINT('Ctrl Pts',(-1.86649730169686,2.4481333818731,11.5621042310933));
#12693=CARTESIAN_POINT('Ctrl Pts',(-1.87543872716782,2.44124936891338,11.5626912125175));
#12694=CARTESIAN_POINT('Ctrl Pts',(-1.87115843792448,2.43565187781351,10.5625482443637));
#12695=CARTESIAN_POINT('Ctrl Pts',(-2.11905849301121,2.24865376720641,10.5786044367557));
#12696=CARTESIAN_POINT('Ctrl Pts',(-3.0601924156055,1.29275809429756,10.6474502650758));
#12697=CARTESIAN_POINT('Ctrl Pts',(-3.36917065569085,-1.35019356953496,
10.7690857293239));
#12698=CARTESIAN_POINT('Ctrl Pts',(-0.701818273267178,-3.56114935009612,
10.9274546371081));
#12699=CARTESIAN_POINT('Ctrl Pts',(2.35600370687118,-2.60536866769977,11.0739005430593));
#12700=CARTESIAN_POINT('Ctrl Pts',(3.06650610127338,-0.786055991087847,
11.1675568130824));
#12701=CARTESIAN_POINT('Ctrl Pts',(3.07371628270923,0.00276101913198965,
11.2084234471775));
#12702=CARTESIAN_POINT('Origin',(0.,0.,-2.20842344717744));
#12703=CARTESIAN_POINT('',(-1.87002230068587,2.43424832114153,9.56277191102392));
#12704=CARTESIAN_POINT('',(-1.87507731191802,2.44082532704937,9.64577043858893));
#12705=CARTESIAN_POINT('',(-1.87240768645123,2.4373123939533,-2.20842344717744));
#12706=CARTESIAN_POINT('',(3.0739867692329,-0.000220521378201549,10.2915765528225));
#12707=CARTESIAN_POINT('Ctrl Pts',(-1.87507731191802,2.44082532704937,9.64577043858893));
#12708=CARTESIAN_POINT('Ctrl Pts',(-1.92849728325354,2.40024009778082,9.64925843930383));
#12709=CARTESIAN_POINT('Ctrl Pts',(-2.76718558415343,1.71569386742277,9.70553607594679));
#12710=CARTESIAN_POINT('Ctrl Pts',(-3.59172323438899,-0.523312921182784,
9.81460334851782));
#12711=CARTESIAN_POINT('Ctrl Pts',(-1.51656848075747,-3.29762827636767,
9.97297225630197));
#12712=CARTESIAN_POINT('Ctrl Pts',(1.9403270808479,-3.06748480440487,10.1313411640862));
#12713=CARTESIAN_POINT('Ctrl Pts',(3.07300908756268,-1.0389883880359,10.2375425962597));
#12714=CARTESIAN_POINT('Ctrl Pts',(3.0784786722727,-0.0121816033650862,
10.2909543925051));
#12715=CARTESIAN_POINT('Ctrl Pts',(3.07846623440684,-0.000220842725659706,
10.2915765528225));
#12716=CARTESIAN_POINT('Ctrl Pts',(3.07349999209138,-0.000220486457828013,
10.2915765528225));
#12717=CARTESIAN_POINT('Ctrl Pts',(3.0735068617889,0.0955405661343771,10.2965657840521));
#12718=CARTESIAN_POINT('Ctrl Pts',(3.06903399635637,0.191473368380318,10.3015550152818));
#12719=CARTESIAN_POINT('Ctrl Pts',(3.06005921740527,0.287123381097861,10.3065442465114));
#12720=CARTESIAN_POINT('Ctrl Pts',(3.05109660660792,0.382643709945966,10.3115267132588));
#12721=CARTESIAN_POINT('Ctrl Pts',(3.03764425277441,0.477881575931341,10.3165091800062));
#12722=CARTESIAN_POINT('Ctrl Pts',(3.019731980344,0.572381880292938,10.3214916467536));
#12723=CARTESIAN_POINT('Ctrl Pts',(3.00183853151596,0.666782876419912,10.3264688775392));
#12724=CARTESIAN_POINT('Ctrl Pts',(2.97949456205797,0.760447420636118,10.3314461083249));
#12725=CARTESIAN_POINT('Ctrl Pts',(2.95278164157565,0.852926038513187,10.3364233391106));
#12726=CARTESIAN_POINT('Ctrl Pts',(2.92608756221715,0.945339429486644,10.341397059362));
#12727=CARTESIAN_POINT('Ctrl Pts',(2.8950307790698,1.03656813428827,10.3463707796135));
#12728=CARTESIAN_POINT('Ctrl Pts',(2.8597436192445,1.12617435692275,10.3513444998649));
#12729=CARTESIAN_POINT('Ctrl Pts',(2.82446895324371,1.21574885344421,10.3563164591136));
#12730=CARTESIAN_POINT('Ctrl Pts',(2.78496704774315,1.30370159915195,10.3612884183622));
#12731=CARTESIAN_POINT('Ctrl Pts',(2.74141929078964,1.38961236396573,10.3662603776108));
#12732=CARTESIAN_POINT('Ctrl Pts',(2.69787493067551,1.47551642751427,10.3712319490336));
#12733=CARTESIAN_POINT('Ctrl Pts',(2.65028554620233,1.55937843360771,10.3762035204563));
#12734=CARTESIAN_POINT('Ctrl Pts',(2.59887915089251,1.640801453271,10.3811750918791));
#12735=CARTESIAN_POINT('Ctrl Pts',(2.54746257427934,1.72224059918585,10.3861476479473));
#12736=CARTESIAN_POINT('Ctrl Pts',(2.49222772110145,1.80123942658639,10.3911202040156));
#12737=CARTESIAN_POINT('Ctrl Pts',(2.43344610969157,1.87742970074168,10.3960927600839));
#12738=CARTESIAN_POINT('Ctrl Pts',(2.37460080990357,1.95370252511756,10.4010707037899));
#12739=CARTESIAN_POINT('Ctrl Pts',(2.31220135119068,2.02716037259249,10.406048647496));
#12740=CARTESIAN_POINT('Ctrl Pts',(2.24655957909046,2.09746807069783,10.4110265912021));
#12741=CARTESIAN_POINT('Ctrl Pts',(2.18087770752789,2.16781871860181,10.4160075758508));
#12742=CARTESIAN_POINT('Ctrl Pts',(2.11194989512604,2.23501507871381,10.4209885604995));
#12743=CARTESIAN_POINT('Ctrl Pts',(2.04012333288603,2.29876032604837,10.4259695451483));
#12744=CARTESIAN_POINT('Ctrl Pts',(1.96818290531611,2.36260662755274,10.4309584260605));
#12745=CARTESIAN_POINT('Ctrl Pts',(1.89333489730439,2.42299061854258,10.4359473069727));
#12746=CARTESIAN_POINT('Ctrl Pts',(1.8159577522221,2.47965717230113,10.4409361878849));
#12747=CARTESIAN_POINT('Ctrl Pts',(1.77902970865396,2.50670113940314,10.4433171184748));
#12748=CARTESIAN_POINT('Ctrl Pts',(1.74152601497156,2.53289905876088,10.4456980490646));
#12749=CARTESIAN_POINT('Ctrl Pts',(1.70348979365072,2.5582268806593,10.4480789796545));
#12750=CARTESIAN_POINT('Ctrl Pts',(1.62362083384983,2.61141057553755,10.4530784891475));
#12751=CARTESIAN_POINT('Ctrl Pts',(1.54111857553602,2.66094378308378,10.4580779986405));
#12752=CARTESIAN_POINT('Ctrl Pts',(1.45635082880792,2.70655583970301,10.4630775081334));
#12753=CARTESIAN_POINT('Ctrl Pts',(1.37169806899008,2.75210602385703,10.4680702358235));
#12754=CARTESIAN_POINT('Ctrl Pts',(1.28478631163001,2.79374542205774,10.4730629635136));
#12755=CARTESIAN_POINT('Ctrl Pts',(1.19601257379454,2.83124639926047,10.4780556912037));
#12756=CARTESIAN_POINT('Ctrl Pts',(1.10733249001466,2.86870781387757,10.4830431516919));
#12757=CARTESIAN_POINT('Ctrl Pts',(1.01679473296664,2.90203931679327,10.4880306121802));
#12758=CARTESIAN_POINT('Ctrl Pts',(0.924820254834722,2.93105949210306,10.4930180726684));
#12759=CARTESIAN_POINT('Ctrl Pts',(0.832911586591927,2.96005890279903,10.4980019645121));
#12760=CARTESIAN_POINT('Ctrl Pts',(0.739568658314046,2.98475298673081,10.5029858563557));
#12761=CARTESIAN_POINT('Ctrl Pts',(0.645230789620373,3.00500906456634,10.5079697481994));
#12762=CARTESIAN_POINT('Ctrl Pts',(0.550927276441999,3.02525776564001,10.5129518250331));
#12763=CARTESIAN_POINT('Ctrl Pts',(0.455629971505204,3.04107157979621,10.5179339018668));
#12764=CARTESIAN_POINT('Ctrl Pts',(0.359790751080044,3.05236840264036,10.5229159787005));
#12765=CARTESIAN_POINT('Ctrl Pts',(0.263960268983606,3.06366419547455,10.5278976012836));
#12766=CARTESIAN_POINT('Ctrl Pts',(0.167588405601096,3.070443764618,10.5328792238666));
#12767=CARTESIAN_POINT('Ctrl Pts',(0.0711334977556424,3.0726767281146,10.5378608464497));
#12768=CARTESIAN_POINT('Ctrl Pts',(-0.0253389472913298,3.07491009760331,
10.5428433747795));
#12769=CARTESIAN_POINT('Ctrl Pts',(-0.121894027946735,3.0725952095872,10.5478259031094));
#12770=CARTESIAN_POINT('Ctrl Pts',(-0.218073137579717,3.06575379909512,
10.5528084314392));
#12771=CARTESIAN_POINT('Ctrl Pts',(-0.314355914118239,3.05890501457079,
10.5577963302002));
#12772=CARTESIAN_POINT('Ctrl Pts',(-0.41026147202538,3.04751999844631,10.5627842289613));
#12773=CARTESIAN_POINT('Ctrl Pts',(-0.505336283203386,3.03167239174654,
10.5677721277223));
#12774=CARTESIAN_POINT('Ctrl Pts',(-0.600467256377221,3.01581542364799,
10.5727629729036));
#12775=CARTESIAN_POINT('Ctrl Pts',(-0.694766076783461,2.99549070848603,
10.5777538180849));
#12776=CARTESIAN_POINT('Ctrl Pts',(-0.787791450552504,2.97082259322841,
10.5827446632662));
#12777=CARTESIAN_POINT('Ctrl Pts',(-0.880967155674901,2.94611461367354,
10.5877435737794));
#12778=CARTESIAN_POINT('Ctrl Pts',(-0.972864886698754,2.91704935082506,
10.5927424842926));
#12779=CARTESIAN_POINT('Ctrl Pts',(-1.06306054931225,2.88380036037447,10.5977413948057));
#12780=CARTESIAN_POINT('Ctrl Pts',(-1.11542448408048,2.8644973482715,10.6006435590167));
#12781=CARTESIAN_POINT('Ctrl Pts',(-1.16721513135671,2.84378510836322,10.6035457232277));
#12782=CARTESIAN_POINT('Ctrl Pts',(-1.21835329387807,2.82170471546837,10.6064478874387));
#12783=CARTESIAN_POINT('Ctrl Pts',(-1.30644831667027,2.7836671204625,10.6114474065788));
#12784=CARTESIAN_POINT('Ctrl Pts',(-1.39291503604813,2.74143320524252,10.6164469257189));
#12785=CARTESIAN_POINT('Ctrl Pts',(-1.47732616423593,2.69516412384552,10.6214464448589));
#12786=CARTESIAN_POINT('Ctrl Pts',(-1.56161152410786,2.6489639810419,10.6264385149681));
#12787=CARTESIAN_POINT('Ctrl Pts',(-1.64384700138803,2.59874083633503,10.6314305850773));
#12788=CARTESIAN_POINT('Ctrl Pts',(-1.72362566041007,2.5447036827057,10.6364226551865));
#12789=CARTESIAN_POINT('Ctrl Pts',(-1.77424119155379,2.51041983705109,10.6395898716223));
#12790=CARTESIAN_POINT('Ctrl Pts',(-1.82386818012003,2.47460172337064,10.6427570880581));
#12791=CARTESIAN_POINT('Ctrl Pts',(-1.87240768645123,2.4373123939533,10.6459243044939));
#12792=CARTESIAN_POINT('',(3.06865031396352,-0.000662305851861743,10.2084234471775));
#12793=CARTESIAN_POINT('Ctrl Pts',(3.06865031396352,-0.000662305851861743,
10.2084234471775));
#12794=CARTESIAN_POINT('Ctrl Pts',(3.0675799278391,0.552109147929758,10.2369419667754));
#12795=CARTESIAN_POINT('Ctrl Pts',(2.66113839896666,2.12956437036722,10.3182501223015));
#12796=CARTESIAN_POINT('Ctrl Pts',(0.440568577236155,3.44770654288841,10.4362917213636));
#12797=CARTESIAN_POINT('Ctrl Pts',(-1.30401135511826,2.86346716363096,10.5258148008277));
#12798=CARTESIAN_POINT('Ctrl Pts',(-1.87115843792448,2.43565187781351,10.5625482443637));
#12799=CARTESIAN_POINT('Ctrl Pts',(-1.87002230068597,2.43424832114145,9.56277191102393));
#12800=CARTESIAN_POINT('Ctrl Pts',(-2.36808575988716,2.04690839709662,9.59534906562752));
#12801=CARTESIAN_POINT('Ctrl Pts',(-3.38005807385769,0.642742195174603,
9.68071585615918));
#12802=CARTESIAN_POINT('Ctrl Pts',(-2.79015488039725,-2.32150152396616,
9.81887228261889));
#12803=CARTESIAN_POINT('Ctrl Pts',(0.428153388171217,-3.60430551682002,
9.97724119040307));
#12804=CARTESIAN_POINT('Ctrl Pts',(2.74707663572839,-1.96358325211724,10.1070915785893));
#12805=CARTESIAN_POINT('Ctrl Pts',(3.0695612822224,-0.471106790621865,10.1841523308474));
#12806=CARTESIAN_POINT('Ctrl Pts',(3.06865031396352,-0.000662305851861743,
10.2084234471775));
#12807=CARTESIAN_POINT('Origin',(0.,0.,-2.20842344717744));
#12808=CARTESIAN_POINT('',(-1.87509145403828,2.44076729861451,8.56274498137416));
#12809=CARTESIAN_POINT('',(-1.87008710121024,2.4342504331012,8.6457400628962));
#12810=CARTESIAN_POINT('',(-1.87240768645123,2.4373123939533,-2.20842344717744));
#12811=CARTESIAN_POINT('',(3.07146331992749,0.00257687728019439,9.29157655282255));
#12812=CARTESIAN_POINT('Ctrl Pts',(-1.87008710121014,2.43425043310128,8.64574006289619));
#12813=CARTESIAN_POINT('Ctrl Pts',(-2.18011611706346,2.19903440513027,8.66583370660699));
#12814=CARTESIAN_POINT('Ctrl Pts',(-3.14634585166812,1.14383563916985,8.73871698624584));
#12815=CARTESIAN_POINT('Ctrl Pts',(-3.25637227139195,-1.60323792246698,
8.86438990181277));
#12816=CARTESIAN_POINT('Ctrl Pts',(-0.428153365804491,-3.60430532853098,
9.02275880959692));
#12817=CARTESIAN_POINT('Ctrl Pts',(2.46555070482014,-2.45088718888649,9.16515435993354));
#12818=CARTESIAN_POINT('Ctrl Pts',(3.06576103701022,-0.709387139347176,
9.25476027434207));
#12819=CARTESIAN_POINT('Ctrl Pts',(3.07146331992749,0.00257687728019439,
9.29157655282255));
#12820=CARTESIAN_POINT('Ctrl Pts',(3.07146331992749,0.00257687728019439,
9.29157655282255));
#12821=CARTESIAN_POINT('Ctrl Pts',(3.07393735062978,0.311474359502131,9.30754991027013));
#12822=CARTESIAN_POINT('Ctrl Pts',(2.88937061009456,1.63834518503067,9.37631290364576));
#12823=CARTESIAN_POINT('Ctrl Pts',(1.03904173686729,3.44037562732375,9.49437753223457));
#12824=CARTESIAN_POINT('Ctrl Pts',(-1.1200052362076,3.01448294124964,9.59646880337577));
#12825=CARTESIAN_POINT('Ctrl Pts',(-1.87507731191802,2.44082532704937,9.64577043858893));
#12826=CARTESIAN_POINT('',(3.07611314785335,-0.00227856489099164,9.20842344717746));
#12827=CARTESIAN_POINT('Ctrl Pts',(3.07611314785335,-0.00227856489099164,
9.20842344717746));
#12828=CARTESIAN_POINT('Ctrl Pts',(3.06889864904703,0.866771338679833,9.25353748454042));
#12829=CARTESIAN_POINT('Ctrl Pts',(2.23070911990389,2.7649081202533,9.35144115783146));
#12830=CARTESIAN_POINT('Ctrl Pts',(-0.289334010845272,3.33608061026952,
9.46955731244694));
#12831=CARTESIAN_POINT('Ctrl Pts',(-1.56099904527893,2.67457320759152,9.54255942969946));
#12832=CARTESIAN_POINT('Ctrl Pts',(-1.87002230068597,2.43424832114145,9.56277191102393));
#12833=CARTESIAN_POINT('Ctrl Pts',(-1.87509145403828,2.44076729861451,8.56274498137416));
#12834=CARTESIAN_POINT('Ctrl Pts',(-2.62208853077648,1.86033637000951,8.61192663029266));
#12835=CARTESIAN_POINT('Ctrl Pts',(-3.59091621734738,-0.111479728561327,
8.71389791513923));
#12836=CARTESIAN_POINT('Ctrl Pts',(-1.94032718221066,-3.06748496465039,
8.86865883591383));
#12837=CARTESIAN_POINT('Ctrl Pts',(1.51656855998305,-3.29762844863588,9.02702774369802));
#12838=CARTESIAN_POINT('Ctrl Pts',(3.0005807836722,-1.31362321131185,9.14028261411922));
#12839=CARTESIAN_POINT('Ctrl Pts',(3.07734060608858,-0.150136716870874,
9.20074784861237));
#12840=CARTESIAN_POINT('Ctrl Pts',(3.07611314785335,-0.00227856489099164,
9.20842344717746));
#12841=CARTESIAN_POINT('Origin',(0.,0.,-2.20842344717744));
#12842=CARTESIAN_POINT('',(-1.87240768645123,2.4373123939533,7.56258888046525));
#12843=CARTESIAN_POINT('',(-1.87108789359224,2.43562943220425,7.64596441938478));
#12844=CARTESIAN_POINT('',(-1.87240768645123,2.4373123939533,-2.20842344717744));
#12845=CARTESIAN_POINT('',(3.06961342576491,-0.00179236055451414,8.29157655282255));
#12846=CARTESIAN_POINT('Ctrl Pts',(-1.87108789359255,2.43562943220401,7.6459644193848));
#12847=CARTESIAN_POINT('Ctrl Pts',(-2.4288603418159,1.99933281172997,7.68257879536437));
#12848=CARTESIAN_POINT('Ctrl Pts',(-3.44303055876561,0.468116087731995,
7.77198280727201));
#12849=CARTESIAN_POINT('Ctrl Pts',(-2.60495841071609,-2.52755294392938,
7.9141764551077));
#12850=CARTESIAN_POINT('Ctrl Pts',(0.701818236604134,-3.56114916406156,
8.07254536289188));
#12851=CARTESIAN_POINT('Ctrl Pts',(2.8206242810132,-1.80488084996747,8.19834539546349));
#12852=CARTESIAN_POINT('Ctrl Pts',(3.07170577833404,-0.393421405353705,
8.27135579210705));
#12853=CARTESIAN_POINT('Ctrl Pts',(3.06961342576491,-0.00179236055451414,
8.29157655282255));
#12854=CARTESIAN_POINT('Ctrl Pts',(3.06961342576491,-0.00179236055451414,
8.29157655282255));
#12855=CARTESIAN_POINT('Ctrl Pts',(3.06624334633598,0.628990905670613,8.32414542803511));
#12856=CARTESIAN_POINT('Ctrl Pts',(2.57037956950142,2.28704841286455,8.40950393917573));
#12857=CARTESIAN_POINT('Ctrl Pts',(0.2554864632756,3.43210578860563,8.52755844253362));
#12858=CARTESIAN_POINT('Ctrl Pts',(-1.36561382421955,2.81698944901127,8.61304407067893));
#12859=CARTESIAN_POINT('Ctrl Pts',(-1.87008710121014,2.43425043310128,8.64574006289619));
#12860=CARTESIAN_POINT('',(3.07349899192449,0.00248930494810733,8.20842344717746));
#12861=CARTESIAN_POINT('Ctrl Pts',(3.07544103263855,0.00249087785624028,
8.20842344717746));
#12862=CARTESIAN_POINT('Ctrl Pts',(3.07695265662786,0.174416482836779,8.21734336637735));
#12863=CARTESIAN_POINT('Ctrl Pts',(2.98575884214701,1.36222404473923,8.2790529215053));
#12864=CARTESIAN_POINT('Ctrl Pts',(1.43881299711621,3.33228911436436,8.3935521125613));
#12865=CARTESIAN_POINT('Ctrl Pts',(-0.940162896586096,3.11776444662607,
8.50273937142698));
#12866=CARTESIAN_POINT('Ctrl Pts',(-1.82029142580991,2.48334796226457,8.5591369943646));
#12867=CARTESIAN_POINT('Ctrl Pts',(-1.87509145403828,2.44076729861451,8.56274498137416));
#12868=CARTESIAN_POINT('Ctrl Pts',(-1.87240768645123,2.4373123939533,7.56258888046525));
#12869=CARTESIAN_POINT('Ctrl Pts',(-1.94889060415999,2.37855619866402,7.56757962088293));
#12870=CARTESIAN_POINT('Ctrl Pts',(-2.02253758922204,2.31624850330128,7.57257036130061));
#12871=CARTESIAN_POINT('Ctrl Pts',(-2.09301755323034,2.25070650504895,7.57756110171829));
#12872=CARTESIAN_POINT('Ctrl Pts',(-2.16361202823142,2.18505801867062,7.58255995074737));
#12873=CARTESIAN_POINT('Ctrl Pts',(-2.23102890013812,2.11616504953983,7.58755879977645));
#12874=CARTESIAN_POINT('Ctrl Pts',(-2.29497537334076,2.04438017153353,7.59255764880554));
#12875=CARTESIAN_POINT('Ctrl Pts',(-2.33399138281656,2.00058167350474,7.5956076237505));
#12876=CARTESIAN_POINT('Ctrl Pts',(-2.37171628177913,1.95570725733652,7.59865759869547));
#12877=CARTESIAN_POINT('Ctrl Pts',(-2.4080914790063,1.90984231776795,7.60170757364043));
#12878=CARTESIAN_POINT('Ctrl Pts',(-2.46771758975397,1.83466065073611,7.60670708313341));
#12879=CARTESIAN_POINT('Ctrl Pts',(-2.52392424819064,1.75655192635735,7.61170659262638));
#12880=CARTESIAN_POINT('Ctrl Pts',(-2.57641121104058,1.67586023332031,7.61670610211936));
#12881=CARTESIAN_POINT('Ctrl Pts',(-2.62882697565872,1.59527799805247,7.62169882980945));
#12882=CARTESIAN_POINT('Ctrl Pts',(-2.67753283546951,1.51212012247806,7.62669155749954));
#12883=CARTESIAN_POINT('Ctrl Pts',(-2.722269004492,1.42676337112436,7.63168428518964));
#12884=CARTESIAN_POINT('Ctrl Pts',(-2.7669579779838,1.3414966689918,7.63667174567787));
#12885=CARTESIAN_POINT('Ctrl Pts',(-2.80768538333751,1.25403608935131,7.6416592061661));
#12886=CARTESIAN_POINT('Ctrl Pts',(-2.84423550879916,1.16478608357327,7.64664666665433));
#12887=CARTESIAN_POINT('Ctrl Pts',(-2.88075948179167,1.07559993826063,7.651630558498));
#12888=CARTESIAN_POINT('Ctrl Pts',(-2.91311195088674,0.984627317191547,
7.65661445034167));
#12889=CARTESIAN_POINT('Ctrl Pts',(-2.94112424919369,0.892295018928627,
7.66159834218534));
#12890=CARTESIAN_POINT('Ctrl Pts',(-2.9691263461154,0.799996345801906,7.66658041901903));
#12891=CARTESIAN_POINT('Ctrl Pts',(-2.99279128538638,0.706339398938925,
7.67156249585273));
#12892=CARTESIAN_POINT('Ctrl Pts',(-3.01199975905624,0.611767685845843,
7.67654457268643));
#12893=CARTESIAN_POINT('Ctrl Pts',(-3.03120648135583,0.51720459551419,7.6815261952695));
#12894=CARTESIAN_POINT('Ctrl Pts',(-3.04595745871357,0.421727334993386,
7.68650781785256));
#12895=CARTESIAN_POINT('Ctrl Pts',(-3.05618439138251,0.325790140842137,
7.69148944043563));
#12896=CARTESIAN_POINT('Ctrl Pts',(-3.066413183488,0.229835503618643,7.69647196876546));
#12897=CARTESIAN_POINT('Ctrl Pts',(-3.07211625082295,0.133421203175779,
7.70145449709529));
#12898=CARTESIAN_POINT('Ctrl Pts',(-3.07327720859963,0.0370060684490644,
7.70643702542512));
#12899=CARTESIAN_POINT('Ctrl Pts',(-3.0744394177177,-0.0595129875833837,
7.71142492418617));
#12900=CARTESIAN_POINT('Ctrl Pts',(-3.07104973812129,-0.156032440036607,
7.71641282294722));
#12901=CARTESIAN_POINT('Ctrl Pts',(-3.06314393340569,-0.252094215006905,
7.72140072170827));
#12902=CARTESIAN_POINT('Ctrl Pts',(-3.05523345862272,-0.348212734986198,
7.72639156688958));
#12903=CARTESIAN_POINT('Ctrl Pts',(-3.04280160336488,-0.443872604060398,
7.73138241207089));
#12904=CARTESIAN_POINT('Ctrl Pts',(-3.02593567731295,-0.538623733941082,
7.7363732572522));
#12905=CARTESIAN_POINT('Ctrl Pts',(-3.0090424954986,-0.633527984040422,
7.74137216776536));
#12906=CARTESIAN_POINT('Ctrl Pts',(-2.98770103195924,-0.727520134807251,
7.74637107827852));
#12907=CARTESIAN_POINT('Ctrl Pts',(-2.9620490623146,-0.820163155988626,
7.75136998879168));
#12908=CARTESIAN_POINT('Ctrl Pts',(-2.94715657163131,-0.873947927642711,
7.75427215300265));
#12909=CARTESIAN_POINT('Ctrl Pts',(-2.93081215209485,-0.927278294014041,
7.75717431721363));
#12910=CARTESIAN_POINT('Ctrl Pts',(-2.91305016692879,-0.98007192335876,
7.76007648142461));
#12911=CARTESIAN_POINT('Ctrl Pts',(-2.88245189371052,-1.07101862102636,
7.76507599091758));
#12912=CARTESIAN_POINT('Ctrl Pts',(-2.84753670122274,-1.16069074941773,
7.77007550041056));
#12913=CARTESIAN_POINT('Ctrl Pts',(-2.80842974048275,-1.24864912716583,
7.77507500990354));
#12914=CARTESIAN_POINT('Ctrl Pts',(-2.76937582808669,-1.33648818993301,
7.78006773759363));
#12915=CARTESIAN_POINT('Ctrl Pts',(-2.72614162500842,-1.42261772455461,
7.78506046528372));
#12916=CARTESIAN_POINT('Ctrl Pts',(-2.67890171754387,-1.50661469451898,
7.79005319297381));
#12917=CARTESIAN_POINT('Ctrl Pts',(-2.6317116469909,-1.59052304979738,7.79504065346204));
#12918=CARTESIAN_POINT('Ctrl Pts',(-2.58052448695269,-1.67230293231824,
7.80002811395028));
#12919=CARTESIAN_POINT('Ctrl Pts',(-2.52556204351728,-1.75155320054654,
7.80501557443851));
#12920=CARTESIAN_POINT('Ctrl Pts',(-2.47063892699494,-1.83074676335538,
7.80999946628218));
#12921=CARTESIAN_POINT('Ctrl Pts',(-2.41194614658159,-1.90741395039178,
7.81498335812585));
#12922=CARTESIAN_POINT('Ctrl Pts',(-2.34974986666695,-1.98118091402544,
7.81996724996951));
#12923=CARTESIAN_POINT('Ctrl Pts',(-2.28757623709701,-2.05492101355795,
7.82494932680321));
#12924=CARTESIAN_POINT('Ctrl Pts',(-2.22190192574253,-2.12576265296946,
7.8299314036369));
#12925=CARTESIAN_POINT('Ctrl Pts',(-2.15303398587823,-2.1933642893175,7.8349134804706));
#12926=CARTESIAN_POINT('Ctrl Pts',(-2.08417232518345,-2.26095976195375,
7.83989510305366));
#12927=CARTESIAN_POINT('Ctrl Pts',(-2.01211792829748,-2.32531551149458,
7.84487672563673));
#12928=CARTESIAN_POINT('Ctrl Pts',(-1.93721461943757,-2.38612693883568,
7.8498583482198));
#12929=CARTESIAN_POINT('Ctrl Pts',(-1.86229769183637,-2.44694942276573,
7.85484087654963));
#12930=CARTESIAN_POINT('Ctrl Pts',(-1.78453116435683,-2.50422602803074,
7.85982340487945));
#12931=CARTESIAN_POINT('Ctrl Pts',(-1.70429097844702,-2.55769320106695,
7.86480593320928));
#12932=CARTESIAN_POINT('Ctrl Pts',(-1.62396430544244,-2.61121800383581,
7.86979383197033));
#12933=CARTESIAN_POINT('Ctrl Pts',(-1.54115901700692,-2.66092493329987,
7.87478173073138));
#12934=CARTESIAN_POINT('Ctrl Pts',(-1.45627881354217,-2.70659458863499,
7.87976962949243));
#12935=CARTESIAN_POINT('Ctrl Pts',(-1.37134847017622,-2.75229122166235,
7.88476047467374));
#12936=CARTESIAN_POINT('Ctrl Pts',(-1.28434116699347,-2.79394564242777,
7.88975131985505));
#12937=CARTESIAN_POINT('Ctrl Pts',(-1.19568197046988,-2.83138603434665,
7.89474216503636));
#12938=CARTESIAN_POINT('Ctrl Pts',(-1.10687949844573,-2.86888693088439,
7.89974107554952));
#12939=CARTESIAN_POINT('Ctrl Pts',(-1.0164202143759,-2.90216004912347,7.90473998606268));
#12940=CARTESIAN_POINT('Ctrl Pts',(-0.924745708016164,-2.93108301238735,
7.90973889657584));
#12941=CARTESIAN_POINT('Ctrl Pts',(-0.871523216692048,-2.94787450898226,
7.91264106078682));
#12942=CARTESIAN_POINT('Ctrl Pts',(-0.817891372082817,-2.96320073719094,
7.9155432249978));
#12943=CARTESIAN_POINT('Ctrl Pts',(-0.763937942530774,-2.97704569497377,
7.91844538920878));
#12944=CARTESIAN_POINT('Ctrl Pts',(-0.670993276545539,-3.00089617097481,
7.92344489870176));
#12945=CARTESIAN_POINT('Ctrl Pts',(-0.576767356000975,-3.02043170716473,
7.92844440819473));
#12946=CARTESIAN_POINT('Ctrl Pts',(-0.481696701506282,-3.03551816627046,
7.93344391768771));
#12947=CARTESIAN_POINT('Ctrl Pts',(-0.386755009750755,-3.0505841606902,
7.9384366453778));
#12948=CARTESIAN_POINT('Ctrl Pts',(-0.290971291227511,-3.06121300426838,
7.94342937306789));
#12949=CARTESIAN_POINT('Ctrl Pts',(-0.194795439480239,-3.06732081575399,
7.94842210075799));
#12950=CARTESIAN_POINT('Ctrl Pts',(-0.0987210508323314,-3.07342218365243,
7.95340956124622));
#12951=CARTESIAN_POINT('Ctrl Pts',(-0.00225578710280942,-3.075011973412,
7.95839702173445));
#12952=CARTESIAN_POINT('Ctrl Pts',(0.0941431146125853,-3.07205783213322,
7.96338448222268));
#12953=CARTESIAN_POINT('Ctrl Pts',(0.190473040660504,-3.06910580461157,
7.96836837406634));
#12954=CARTESIAN_POINT('Ctrl Pts',(0.286736261591087,-3.06161632286734,
7.97335226591001));
#12955=CARTESIAN_POINT('Ctrl Pts',(0.382474283278711,-3.04960910161129,
7.97833615775367));
#12956=CARTESIAN_POINT('Ctrl Pts',(0.478177439550023,-3.03760625308784,
7.98331823458737));
#12957=CARTESIAN_POINT('Ctrl Pts',(0.57335534149521,-3.02108898855313,7.98830031142107));
#12958=CARTESIAN_POINT('Ctrl Pts',(0.667554329894348,-3.00012890833699,
7.99328238825476));
#12959=CARTESIAN_POINT('Ctrl Pts',(0.761744729515948,-2.97917073919728,
7.99826401083783));
#12960=CARTESIAN_POINT('Ctrl Pts',(0.854955964602248,-2.95377065527513,
8.0032456334209));
#12961=CARTESIAN_POINT('Ctrl Pts',(0.946745344142695,-2.92405121421362,
8.00822725600397));
#12962=CARTESIAN_POINT('Ctrl Pts',(1.03855141260955,-2.8943263696341,8.0132097843338));
#12963=CARTESIAN_POINT('Ctrl Pts',(1.12893469451006,-2.86028074348634,8.01819231266362));
#12964=CARTESIAN_POINT('Ctrl Pts',(1.21746944123998,-2.82208618040747,8.02317484099344));
#12965=CARTESIAN_POINT('Ctrl Pts',(1.30609961537883,-2.78385044921862,8.02816273975449));
#12966=CARTESIAN_POINT('Ctrl Pts',(1.39287687288442,-2.7414570274477,8.03315063851555));
#12967=CARTESIAN_POINT('Ctrl Pts',(1.47739738672416,-2.69512508275602,8.0381385372766));
#12968=CARTESIAN_POINT('Ctrl Pts',(1.56196782799152,-2.64876576914867,8.04312938245791));
#12969=CARTESIAN_POINT('Ctrl Pts',(1.64427849681297,-2.59846352889428,8.04812022763922));
#12970=CARTESIAN_POINT('Ctrl Pts',(1.7239538466565,-2.5444813586659,8.05311107282053));
#12971=CARTESIAN_POINT('Ctrl Pts',(1.80375795387742,-2.49041195188721,8.05810998333369));
#12972=CARTESIAN_POINT('Ctrl Pts',(1.88091788718259,-2.43265100345217,8.06310889384685));
#12973=CARTESIAN_POINT('Ctrl Pts',(1.95509057372796,-2.37150228726858,8.06810780436));
#12974=CARTESIAN_POINT('Ctrl Pts',(1.99815222001228,-2.33600182868093,8.07100996857099));
#12975=CARTESIAN_POINT('Ctrl Pts',(2.0402076835136,-2.2993602400556,8.07391213278197));
#12976=CARTESIAN_POINT('Ctrl Pts',(2.08119575623356,-2.26164242846552,8.07681429699296));
#12977=CARTESIAN_POINT('Ctrl Pts',(2.15075950934274,-2.19762886649112,8.0817397648488));
#12978=CARTESIAN_POINT('Ctrl Pts',(2.2175068160232,-2.13027396279288,8.08666523270465));
#12979=CARTESIAN_POINT('Ctrl Pts',(2.28109244639392,-2.05985909736676,8.0915907005605));
#12980=CARTESIAN_POINT('Ctrl Pts',(2.3445757885859,-1.98955750609235,8.09650824497305));
#12981=CARTESIAN_POINT('Ctrl Pts',(2.40490726497235,-1.91620607231197,8.1014257893856));
#12982=CARTESIAN_POINT('Ctrl Pts',(2.46177625232316,-1.84012497768432,8.10634333379815));
#12983=CARTESIAN_POINT('Ctrl Pts',(2.51859341366845,-1.76411321749385,8.1112563967403));
#12984=CARTESIAN_POINT('Ctrl Pts',(2.57195407934571,-1.68537709464414,8.11616945968244));
#12985=CARTESIAN_POINT('Ctrl Pts',(2.62158640063749,-1.60427148388063,8.12108252262459));
#12986=CARTESIAN_POINT('Ctrl Pts',(2.67118799605355,-1.52321608315874,8.1259925440374));
#12987=CARTESIAN_POINT('Ctrl Pts',(2.71706559402599,-1.43979449251527,8.1309025654502));
#12988=CARTESIAN_POINT('Ctrl Pts',(2.75899012028254,-1.35439128990973,8.13581258686301));
#12989=CARTESIAN_POINT('Ctrl Pts',(2.800900940989,-1.26901600647168,8.14072100314034));
#12990=CARTESIAN_POINT('Ctrl Pts',(2.83886105818273,-1.18166080472173,8.14562941941766));
#12991=CARTESIAN_POINT('Ctrl Pts',(2.87268751225075,-1.09273450890808,8.15053783569499));
#12992=CARTESIAN_POINT('Ctrl Pts',(2.90652877058616,-1.00376929418623,8.15544840015809));
#12993=CARTESIAN_POINT('Ctrl Pts',(2.9362325826473,-0.913232033076059,8.16035896462118));
#12994=CARTESIAN_POINT('Ctrl Pts',(2.96166455066029,-0.821550570179439,
8.16526952908427));
#12995=CARTESIAN_POINT('Ctrl Pts',(2.98710113918497,-0.729852450480216,
8.17018098570484));
#12996=CARTESIAN_POINT('Ctrl Pts',(3.0082642306464,-0.637010155946488,8.17509244232541));
#12997=CARTESIAN_POINT('Ctrl Pts',(3.02507014949394,-0.543463743630365,
8.18000389894599));
#12998=CARTESIAN_POINT('Ctrl Pts',(3.04189704873931,-0.449800548592386,
8.18492148699649));
#12999=CARTESIAN_POINT('Ctrl Pts',(3.05435584318727,-0.355431929188367,
8.189839075047));
#13000=CARTESIAN_POINT('Ctrl Pts',(3.0624145814086,-0.260804872607883,8.1947566630975));
#13001=CARTESIAN_POINT('Ctrl Pts',(3.0698801000122,-0.173143500330372,8.19931225779082));
#13002=CARTESIAN_POINT('Ctrl Pts',(3.07357006286123,-0.0852606722414295,
8.20386785248414));
#13003=CARTESIAN_POINT('Ctrl Pts',(3.07349899192449,0.00248930494810733,
8.20842344717746));
#13004=CARTESIAN_POINT('Origin',(0.,0.,-2.20842344717744));
#13005=CARTESIAN_POINT('',(-1.87240768645124,2.43731239395329,6.5627091405633));
#13006=CARTESIAN_POINT('',(-1.87543519516197,2.44126013959499,6.6458244875715));
#13007=CARTESIAN_POINT('',(-1.87240768645123,2.4373123939533,-2.20842344717744));
#13008=CARTESIAN_POINT('',(3.07786885453234,-0.00123528292102317,7.29157655282255));
#13009=CARTESIAN_POINT('Ctrl Pts',(-1.87543519516259,2.44126013959451,6.64582448757154));
#13010=CARTESIAN_POINT('Ctrl Pts',(-1.88255777719139,2.43579791465536,6.64629138932579));
#13011=CARTESIAN_POINT('Ctrl Pts',(-2.69199670149138,1.80887592431544,6.6995479270081));
#13012=CARTESIAN_POINT('Ctrl Pts',(-3.61557748169771,-0.319267411063196,
6.80559410061847));
#13013=CARTESIAN_POINT('Ctrl Pts',(-1.70070776265665,-3.20654413847151,
6.96396300840265));
#13014=CARTESIAN_POINT('Ctrl Pts',(1.76367148919952,-3.17234851239761,7.12233191618683));
#13015=CARTESIAN_POINT('Ctrl Pts',(3.0445276197161,-1.15572815572695,7.23153643099346));
#13016=CARTESIAN_POINT('Ctrl Pts',(3.07822572016116,-0.070965146153975,
7.28795130987203));
#13017=CARTESIAN_POINT('Ctrl Pts',(3.07786885453234,-0.00123528292102317,
7.29157655282255));
#13018=CARTESIAN_POINT('Ctrl Pts',(3.07786885453234,-0.00123528292102317,
7.29157655282255));
#13019=CARTESIAN_POINT('Ctrl Pts',(3.0730291562681,0.944418965649178,7.34074094580009));
#13020=CARTESIAN_POINT('Ctrl Pts',(2.10098001424261,2.9140591129136,7.44269497470569));
#13021=CARTESIAN_POINT('Ctrl Pts',(-0.455571413424762,3.29139779091718,
7.56082426355977));
#13022=CARTESIAN_POINT('Ctrl Pts',(-1.62467882336431,2.62837370441962,7.62978915943631));
#13023=CARTESIAN_POINT('Ctrl Pts',(-1.87108789359255,2.43562943220401,7.6459644193848));
#13024=CARTESIAN_POINT('',(3.07349998753216,0.000276838914890879,7.20842344720515));
#13025=CARTESIAN_POINT('Ctrl Pts',(3.07349998753216,0.000276838914890267,
7.20842344720515));
#13026=CARTESIAN_POINT('Ctrl Pts',(3.0734907994524,0.102284040624626,7.21367722612571));
#13027=CARTESIAN_POINT('Ctrl Pts',(3.06839901409326,0.20417997742157,7.21893100504626));
#13028=CARTESIAN_POINT('Ctrl Pts',(3.05828337165217,0.305458783923172,7.22418478396682));
#13029=CARTESIAN_POINT('Ctrl Pts',(3.0481377246032,0.407037999508376,7.22945414643309));
#13030=CARTESIAN_POINT('Ctrl Pts',(3.03293845951892,0.507996061934451,7.23472350889935));
#13031=CARTESIAN_POINT('Ctrl Pts',(3.01279594210165,0.607834567341986,7.23999287136562));
#13032=CARTESIAN_POINT('Ctrl Pts',(2.99262318887218,0.707822939731749,7.24527014364032));
#13033=CARTESIAN_POINT('Ctrl Pts',(2.96749246796263,0.806688050722019,7.25054741591501));
#13034=CARTESIAN_POINT('Ctrl Pts',(2.93756412736932,0.903946484916509,7.25582468818971));
#13035=CARTESIAN_POINT('Ctrl Pts',(2.90755169173929,1.00147820361103,7.26111678896464));
#13036=CARTESIAN_POINT('Ctrl Pts',(2.87271479946082,1.09739387420792,7.26640888973958));
#13037=CARTESIAN_POINT('Ctrl Pts',(2.83326264746001,1.1912283662287,7.27170099051452));
#13038=CARTESIAN_POINT('Ctrl Pts',(2.80029014392393,1.26965141701431,7.2761239130337));
#13039=CARTESIAN_POINT('Ctrl Pts',(2.76409481162759,1.34662108790793,7.28054683555289));
#13040=CARTESIAN_POINT('Ctrl Pts',(2.72482273064765,1.42188021174286,7.28496975807208));
#13041=CARTESIAN_POINT('Ctrl Pts',(2.68043100983039,1.50695036669435,7.28996926756506));
#13042=CARTESIAN_POINT('Ctrl Pts',(2.63197360866318,1.59008905533462,7.29496877705804));
#13043=CARTESIAN_POINT('Ctrl Pts',(2.57964256266099,1.6708819524155,7.29996828655102));
#13044=CARTESIAN_POINT('Ctrl Pts',(2.52738250339041,1.75156525444452,7.30496101424111));
#13045=CARTESIAN_POINT('Ctrl Pts',(2.47125947900092,1.82990872375334,7.30995374193121));
#13046=CARTESIAN_POINT('Ctrl Pts',(2.41151184191219,1.9055216835075,7.31494646962131));
#13047=CARTESIAN_POINT('Ctrl Pts',(2.35182723707454,1.9810548734951,7.31993393010954));
#13048=CARTESIAN_POINT('Ctrl Pts',(2.28852589187282,2.05386293783942,7.32492139059777));
#13049=CARTESIAN_POINT('Ctrl Pts',(2.22188939148064,2.12358418293832,7.32990885108601));
#13050=CARTESIAN_POINT('Ctrl Pts',(2.15530057106218,2.19325554085654,7.33489274292968));
#13051=CARTESIAN_POINT('Ctrl Pts',(2.08538164189108,2.25984415387933,7.33987663477335));
#13052=CARTESIAN_POINT('Ctrl Pts',(2.01245375433213,2.32302219891987,7.34486052661702));
#13053=CARTESIAN_POINT('Ctrl Pts',(1.9395524253036,2.38617723608115,7.34984260345071));
#13054=CARTESIAN_POINT('Ctrl Pts',(1.86364464653801,2.44592388593928,7.35482468028441));
#13055=CARTESIAN_POINT('Ctrl Pts',(1.78508692598543,2.501972605101,7.35980675711811));
#13056=CARTESIAN_POINT('Ctrl Pts',(1.70653636808716,2.55801621391078,7.36478837970118));
#13057=CARTESIAN_POINT('Ctrl Pts',(1.6253367062168,2.61036230757298,7.36977000228424));
#13058=CARTESIAN_POINT('Ctrl Pts',(1.54187501558459,2.6587635634475,7.37475162486731));
#13059=CARTESIAN_POINT('Ctrl Pts',(1.45839815014636,2.70717361952319,7.37973415319714));
#13060=CARTESIAN_POINT('Ctrl Pts',(1.37265881889303,2.75163719318927,7.38471668152697));
#13061=CARTESIAN_POINT('Ctrl Pts',(1.28506942846019,2.79195250927321,7.3896992098568));
#13062=CARTESIAN_POINT('Ctrl Pts',(1.19738562957334,2.83231127932625,7.39468710861785));
#13063=CARTESIAN_POINT('Ctrl Pts',(1.10784818990066,2.86851268159868,7.3996750073789));
#13064=CARTESIAN_POINT('Ctrl Pts',(1.01689005841237,2.90040287875703,7.40466290613995));
#13065=CARTESIAN_POINT('Ctrl Pts',(0.925878196707301,2.93231191389258,7.40965375132126));
#13066=CARTESIAN_POINT('Ctrl Pts',(0.833444392583186,2.95990454753982,7.41464459650257));
#13067=CARTESIAN_POINT('Ctrl Pts',(0.74003528797117,2.9830772739836,7.41963544168388));
#13068=CARTESIAN_POINT('Ctrl Pts',(0.646475231887209,3.0062874481385,7.42463435219704));
#13069=CARTESIAN_POINT('Ctrl Pts',(0.55193715843439,3.02506336728004,7.4296332627102));
#13070=CARTESIAN_POINT('Ctrl Pts',(0.456876329764853,3.03935293595538,7.43463217322336));
#13071=CARTESIAN_POINT('Ctrl Pts',(0.401687877380416,3.04764887857939,7.43753433743433));
#13072=CARTESIAN_POINT('Ctrl Pts',(0.346323316646573,3.05443367349224,7.44043650164529));
#13073=CARTESIAN_POINT('Ctrl Pts',(0.290871837190702,3.05970518585195,7.44333866585626));
#13074=CARTESIAN_POINT('Ctrl Pts',(0.195371922835088,3.06878391528922,7.44833684509896));
#13075=CARTESIAN_POINT('Ctrl Pts',(0.0992788577162925,3.07340316990389,
7.45333502434166));
#13076=CARTESIAN_POINT('Ctrl Pts',(0.00304436661068013,3.07349849224494,
7.45833320358435));
#13077=CARTESIAN_POINT('Ctrl Pts',(-0.0930703017848441,3.07359369589902,
7.4633251595346));
#13078=CARTESIAN_POINT('Ctrl Pts',(-0.189325611690144,3.06917615571992,
7.46831711548484));
#13079=CARTESIAN_POINT('Ctrl Pts',(-0.285264308459432,3.06023308333192,
7.47330907143509));
#13080=CARTESIAN_POINT('Ctrl Pts',(-0.381109750793669,3.05129870379874,
7.47829617509895));
#13081=CARTESIAN_POINT('Ctrl Pts',(-0.476638757002943,3.03784757285239,
7.48328327876281));
#13082=CARTESIAN_POINT('Ctrl Pts',(-0.571394728592988,3.01991892509321,
7.48827038242667));
#13083=CARTESIAN_POINT('Ctrl Pts',(-0.666084468146671,3.00200280900703,
7.49325400023074));
#13084=CARTESIAN_POINT('Ctrl Pts',(-0.760001817139245,2.97961547816257,
7.49823761803481));
#13085=CARTESIAN_POINT('Ctrl Pts',(-0.852697018688738,2.95284778549781,
7.50322123583888));
#13086=CARTESIAN_POINT('Ctrl Pts',(-0.94537387288352,2.92608539101834,7.50820386722508));
#13087=CARTESIAN_POINT('Ctrl Pts',(-1.03682863594406,2.89494446852317,7.51318649861128));
#13088=CARTESIAN_POINT('Ctrl Pts',(-1.12662418623037,2.85956643444435,7.51816912999748));
#13089=CARTESIAN_POINT('Ctrl Pts',(-1.21640461733843,2.82419435708389,7.5231509224413));
#13090=CARTESIAN_POINT('Ctrl Pts',(-1.30452598436501,2.78458675206373,7.52813271488512));
#13091=CARTESIAN_POINT('Ctrl Pts',(-1.39057003939577,2.74093363938911,7.53311450732895));
#13092=CARTESIAN_POINT('Ctrl Pts',(-1.47666863303423,2.69725285740037,7.53809945745779));
#13093=CARTESIAN_POINT('Ctrl Pts',(-1.56068689183067,2.64952164364708,7.54308440758664));
#13094=CARTESIAN_POINT('Ctrl Pts',(-1.64223045413458,2.59797640203158,7.54806935771549));
#13095=CARTESIAN_POINT('Ctrl Pts',(-1.72140032727714,2.54793161462588,7.55290919863207));
#13096=CARTESIAN_POINT('Ctrl Pts',(-1.79823729817869,2.49429204311649,7.55774903954866));
#13097=CARTESIAN_POINT('Ctrl Pts',(-1.87240768645123,2.4373123939533,7.56258888046525));
#13098=CARTESIAN_POINT('Ctrl Pts',(-1.87240768645124,2.43731239395329,6.5627091405633));
#13099=CARTESIAN_POINT('Ctrl Pts',(-1.94892008865579,2.37853354789643,6.56769076779308));
#13100=CARTESIAN_POINT('Ctrl Pts',(-2.02267799124896,2.31613618435552,6.57267239502285));
#13101=CARTESIAN_POINT('Ctrl Pts',(-2.09332988527124,2.25041601519148,6.57765402225263));
#13102=CARTESIAN_POINT('Ctrl Pts',(-2.16398784569987,2.18469020307537,6.58263607722147));
#13103=CARTESIAN_POINT('Ctrl Pts',(-2.23153894679076,2.11564131807246,6.58761813219031));
#13104=CARTESIAN_POINT('Ctrl Pts',(-2.29566752976676,2.04360290731212,6.59260018715915));
#13105=CARTESIAN_POINT('Ctrl Pts',(-2.35986174777179,1.97149076588504,6.59758734121653));
#13106=CARTESIAN_POINT('Ctrl Pts',(-2.42062615831467,1.89638331565215,6.60257449527391));
#13107=CARTESIAN_POINT('Ctrl Pts',(-2.47768464333418,1.81864814029157,6.60756164933129));
#13108=CARTESIAN_POINT('Ctrl Pts',(-2.53477192355408,1.74087373500838,6.61255132021154));
#13109=CARTESIAN_POINT('Ctrl Pts',(-2.58814930967629,1.66046932891588,6.6175409910918));
#13110=CARTESIAN_POINT('Ctrl Pts',(-2.63758460280537,1.57783069847308,6.62253066197205));
#13111=CARTESIAN_POINT('Ctrl Pts',(-2.68710505115045,1.49504971810212,6.62752892785549));
#13112=CARTESIAN_POINT('Ctrl Pts',(-2.73266963029805,1.41002721092648,6.63252719373892));
#13113=CARTESIAN_POINT('Ctrl Pts',(-2.77409252163596,1.32318287904713,6.63752545962236));
#13114=CARTESIAN_POINT('Ctrl Pts',(-2.81268074414734,1.24228151523177,6.64218168206004));
#13115=CARTESIAN_POINT('Ctrl Pts',(-2.84767512121639,1.15979962218973,6.64683790449771));
#13116=CARTESIAN_POINT('Ctrl Pts',(-2.87896424539989,1.07608880846751,6.65149412693539));
#13117=CARTESIAN_POINT('Ctrl Pts',(-2.91256020767968,0.9862062881474,6.65649363642837));
#13118=CARTESIAN_POINT('Ctrl Pts',(-2.9420018871256,0.894591066769512,6.66149314592135));
#13119=CARTESIAN_POINT('Ctrl Pts',(-2.96710950151727,0.801662931665151,
6.66649265541433));
#13120=CARTESIAN_POINT('Ctrl Pts',(-2.99218305758949,0.70886085298577,6.67148538310444));
#13121=CARTESIAN_POINT('Ctrl Pts',(-3.01293411947718,0.614749820260872,
6.67647811079455));
#13122=CARTESIAN_POINT('Ctrl Pts',(-3.02923145456872,0.519768260527229,
6.68147083848466));
#13123=CARTESIAN_POINT('Ctrl Pts',(-3.04551159638247,0.424886903945295,
6.68645829897289));
#13124=CARTESIAN_POINT('Ctrl Pts',(-3.05734727803301,0.329137276385941,
6.69144575946111));
#13125=CARTESIAN_POINT('Ctrl Pts',(-3.0646577226007,0.232970584632222,6.69643321994934));
#13126=CARTESIAN_POINT('Ctrl Pts',(-3.07196293637442,0.136872702394353,
6.70141711179301));
#13127=CARTESIAN_POINT('Ctrl Pts',(-3.07474931670532,0.0403587856497919,
6.70640100363668));
#13128=CARTESIAN_POINT('Ctrl Pts',(-3.07298772560657,-0.0561131737775446,
6.71138489548034));
#13129=CARTESIAN_POINT('Ctrl Pts',(-3.07122677603566,-0.152550000506614,
6.71636697231404));
#13130=CARTESIAN_POINT('Ctrl Pts',(-3.06492115384698,-0.248944461837164,
6.72134904914773));
#13131=CARTESIAN_POINT('Ctrl Pts',(-3.05409382663993,-0.344837857666258,
6.72633112598143));
#13132=CARTESIAN_POINT('Ctrl Pts',(-3.04326748663569,-0.440722510226871,
6.7313127485645));
#13133=CARTESIAN_POINT('Ctrl Pts',(-3.02792031072521,-0.536105751947464,
6.73629437114756));
#13134=CARTESIAN_POINT('Ctrl Pts',(-3.00812710105978,-0.630534371679836,
6.74127599373063));
#13135=CARTESIAN_POINT('Ctrl Pts',(-2.98833029264009,-0.724980160199006,
6.74625852206045));
#13136=CARTESIAN_POINT('Ctrl Pts',(-2.96408593513457,-0.818470552411485,
6.75124105039028));
#13137=CARTESIAN_POINT('Ctrl Pts',(-2.93551963948915,-0.910563944033318,
6.7562235787201));
#13138=CARTESIAN_POINT('Ctrl Pts',(-2.90692255358704,-1.00275659875887,
6.76121147748115));
#13139=CARTESIAN_POINT('Ctrl Pts',(-2.8739943597189,-1.0935488268306,6.7661993762422));
#13140=CARTESIAN_POINT('Ctrl Pts',(-2.83691005410301,-1.18251579056233,
6.77118727500326));
#13141=CARTESIAN_POINT('Ctrl Pts',(-2.79980384227881,-1.2715353083006,6.77617812018457));
#13142=CARTESIAN_POINT('Ctrl Pts',(-2.75853681795526,-1.35872701822717,
6.78116896536588));
#13143=CARTESIAN_POINT('Ctrl Pts',(-2.71333056440624,-1.44368954358578,
6.78615981054719));
#13144=CARTESIAN_POINT('Ctrl Pts',(-2.66805125640985,-1.52878937053099,
6.79115872106035));
#13145=CARTESIAN_POINT('Ctrl Pts',(-2.61882023196557,-1.61165244254711,
6.79615763157351));
#13146=CARTESIAN_POINT('Ctrl Pts',(-2.5659030726829,-1.69190533765825,6.80115654208667));
#13147=CARTESIAN_POINT('Ctrl Pts',(-2.53518152137452,-1.73849690584187,
6.80405870629763));
#13148=CARTESIAN_POINT('Ctrl Pts',(-2.50321834242866,-1.78420930261702,
6.8069608705086));
#13149=CARTESIAN_POINT('Ctrl Pts',(-2.47007156829701,-1.82897476677256,
6.80986303471956));
#13150=CARTESIAN_POINT('Ctrl Pts',(-2.41297017778761,-1.90609147924443,
6.81486254421253));
#13151=CARTESIAN_POINT('Ctrl Pts',(-2.35215360522452,-1.9806669831205,6.81986205370551));
#13152=CARTESIAN_POINT('Ctrl Pts',(-2.28787608227214,-2.05232192459348,
6.82486156319848));
#13153=CARTESIAN_POINT('Ctrl Pts',(-2.22368575137151,-2.12387966659332,
6.82985429088857));
#13154=CARTESIAN_POINT('Ctrl Pts',(-2.15604409120953,-2.19252439589185,
6.83484701857866));
#13155=CARTESIAN_POINT('Ctrl Pts',(-2.08524740120198,-2.25790733330232,
6.83983974626875));
#13156=CARTESIAN_POINT('Ctrl Pts',(-2.01452539991779,-2.32322129336195,
6.84482720675698));
#13157=CARTESIAN_POINT('Ctrl Pts',(-1.94065530636246,-2.38528000601394,
6.84981466724521));
#13158=CARTESIAN_POINT('Ctrl Pts',(-1.86397161018464,-2.44377005596388,
6.85480212773344));
#13159=CARTESIAN_POINT('Ctrl Pts',(-1.78734278298395,-2.50221825491584,
6.85978601957711));
#13160=CARTESIAN_POINT('Ctrl Pts',(-1.70790470332665,-2.55710260187456,
6.86476991142077));
#13161=CARTESIAN_POINT('Ctrl Pts',(-1.62602566699892,-2.608149301758,6.86975380326444));
#13162=CARTESIAN_POINT('Ctrl Pts',(-1.54417644898836,-2.65917741169758,
6.87473588009813));
#13163=CARTESIAN_POINT('Ctrl Pts',(-1.45988841264609,-2.70637041939934,
6.87971795693182));
#13164=CARTESIAN_POINT('Ctrl Pts',(-1.373558816825,-2.74949784992138,6.88470003376551));
#13165=CARTESIAN_POINT('Ctrl Pts',(-1.28723709227403,-2.79262134821541,
6.88968165634858));
#13166=CARTESIAN_POINT('Ctrl Pts',(-1.19887457110102,-2.83167981031415,
6.89466327893165));
#13167=CARTESIAN_POINT('Ctrl Pts',(-1.10889212946868,-2.86648922816787,
6.89964490151472));
#13168=CARTESIAN_POINT('Ctrl Pts',(-1.01889332744293,-2.9013049749871,6.90462742984456));
#13169=CARTESIAN_POINT('Ctrl Pts',(-0.927274429425946,-2.93186998493455,
6.90960995817438));
#13170=CARTESIAN_POINT('Ctrl Pts',(-0.834474238759799,-2.95804918736086,
6.91459248650422));
#13171=CARTESIAN_POINT('Ctrl Pts',(-0.741574023164949,-2.98425660710911,
6.91958038526527));
#13172=CARTESIAN_POINT('Ctrl Pts',(-0.647490396150168,-3.00606866243137,
6.92456828402632));
#13173=CARTESIAN_POINT('Ctrl Pts',(-0.552674985253281,-3.02340083526404,
6.92955618278737));
#13174=CARTESIAN_POINT('Ctrl Pts',(-0.457803565591813,-3.04074324644908,
6.93454702796868));
#13175=CARTESIAN_POINT('Ctrl Pts',(-0.362199936161134,-3.05360044739323,
6.93953787314999));
#13176=CARTESIAN_POINT('Ctrl Pts',(-0.266321410047212,-3.0619397702356,
6.9445287183313));
#13177=CARTESIAN_POINT('Ctrl Pts',(-0.170287941813808,-3.07029256963429,
6.94952762884446));
#13178=CARTESIAN_POINT('Ctrl Pts',(-0.073979128169933,-3.07411289505045,
6.95452653935761));
#13179=CARTESIAN_POINT('Ctrl Pts',(0.0221472110900531,-3.07342020411153,
6.95952544987077));
#13180=CARTESIAN_POINT('Ctrl Pts',(0.0779542556048634,-3.07301805591405,
6.96242761408176));
#13181=CARTESIAN_POINT('Ctrl Pts',(0.133699864030344,-3.07109577378738,
6.96532977829275));
#13182=CARTESIAN_POINT('Ctrl Pts',(0.189295602926454,-3.06766514220713,
6.96823194250373));
#13183=CARTESIAN_POINT('Ctrl Pts',(0.285069447606795,-3.06175525086211,
6.9732314519967));
#13184=CARTESIAN_POINT('Ctrl Pts',(0.380734482790612,-3.05134552848551,
6.97823096148967));
#13185=CARTESIAN_POINT('Ctrl Pts',(0.475834092604456,-3.0364426828635,6.98323047098264));
#13186=CARTESIAN_POINT('Ctrl Pts',(0.5708047004015,-3.02156005285694,6.98822319867273));
#13187=CARTESIAN_POINT('Ctrl Pts',(0.665210977222059,-3.00219648017976,
6.99321592636282));
#13188=CARTESIAN_POINT('Ctrl Pts',(0.758599049095575,-2.97841060512336,
6.99820865405291));
#13189=CARTESIAN_POINT('Ctrl Pts',(0.851888598907804,-2.95464982356544,
7.00319611454117));
#13190=CARTESIAN_POINT('Ctrl Pts',(0.944161656059448,-2.92647612196475,
7.00818357502943));
#13191=CARTESIAN_POINT('Ctrl Pts',(1.03497321680813,-2.89399942821173,7.01317103551769));
#13192=CARTESIAN_POINT('Ctrl Pts',(1.12571979976179,-2.86154597229245,7.01815492736135));
#13193=CARTESIAN_POINT('Ctrl Pts',(1.21500655304333,-2.82479579230441,7.02313881920501));
#13194=CARTESIAN_POINT('Ctrl Pts',(1.30240330023451,-2.78390874375189,7.02812271104868));
#13195=CARTESIAN_POINT('Ctrl Pts',(1.3897682196951,-2.74303658524973,7.03310478788238));
#13196=CARTESIAN_POINT('Ctrl Pts',(1.4752441034335,-2.69803073734582,7.03808686471607));
#13197=CARTESIAN_POINT('Ctrl Pts',(1.55842134264391,-2.6490989352593,7.04306894154977));
#13198=CARTESIAN_POINT('Ctrl Pts',(1.64159099800624,-2.60017159462591,7.04805056413284));
#13199=CARTESIAN_POINT('Ctrl Pts',(1.7224620472756,-2.54731923422812,7.0530321867159));
#13200=CARTESIAN_POINT('Ctrl Pts',(1.80065099923568,-2.49079469827434,7.05801380929897));
#13201=CARTESIAN_POINT('Ctrl Pts',(1.87885416732519,-2.43425988516376,7.06299633762881));
#13202=CARTESIAN_POINT('Ctrl Pts',(1.95437391391174,-2.37405182770905,7.06797886595865));
#13203=CARTESIAN_POINT('Ctrl Pts',(2.02685803561213,-2.31046505134237,7.07296139428849));
#13204=CARTESIAN_POINT('Ctrl Pts',(2.09942028451285,-2.24680973780234,7.07794929304953));
#13205=CARTESIAN_POINT('Ctrl Pts',(2.16894004583742,-2.17976872487001,7.08293719181058));
#13206=CARTESIAN_POINT('Ctrl Pts',(2.23510053716814,-2.10967481824823,7.08792509057163));
#13207=CARTESIAN_POINT('Ctrl Pts',(2.3013001104092,-2.03953950619371,7.09291593575293));
#13208=CARTESIAN_POINT('Ctrl Pts',(2.36413617665463,-1.9663480425164,7.09790678093424));
#13209=CARTESIAN_POINT('Ctrl Pts',(2.42333234953121,-1.89046623183688,7.10289762611554));
#13210=CARTESIAN_POINT('Ctrl Pts',(2.48262418491815,-1.81446179423493,7.10789653662871));
#13211=CARTESIAN_POINT('Ctrl Pts',(2.5382641283343,-1.73575868649176,7.11289544714187));
#13212=CARTESIAN_POINT('Ctrl Pts',(2.59001923998573,-1.65475151805452,7.11789435765503));
#13213=CARTESIAN_POINT('Ctrl Pts',(2.62006615368293,-1.60772204944317,7.12079652186599));
#13214=CARTESIAN_POINT('Ctrl Pts',(2.64880454179316,-1.55991647365887,7.12369868607694));
#13215=CARTESIAN_POINT('Ctrl Pts',(2.67619614131918,-1.511415384065,7.1266008502879));
#13216=CARTESIAN_POINT('Ctrl Pts',(2.72544131435982,-1.42421914174841,7.13181841995284));
#13217=CARTESIAN_POINT('Ctrl Pts',(2.77049117203043,-1.33449006635658,7.13703598961777));
#13218=CARTESIAN_POINT('Ctrl Pts',(2.81108935767531,-1.24264993991252,7.14225355928271));
#13219=CARTESIAN_POINT('Ctrl Pts',(2.8516143832756,-1.15097531415871,7.14746172661541));
#13220=CARTESIAN_POINT('Ctrl Pts',(2.88770355110386,-1.05719755939824,7.15266989394812));
#13221=CARTESIAN_POINT('Ctrl Pts',(2.91914588564439,-0.961763769501352,
7.15787806128082));
#13222=CARTESIAN_POINT('Ctrl Pts',(2.95051943878262,-0.866538744951909,
7.1630748355329));
#13223=CARTESIAN_POINT('Ctrl Pts',(2.97726629363165,-0.769665267033125,
7.16827160978499));
#13224=CARTESIAN_POINT('Ctrl Pts',(2.9992236063298,-0.671610012755951,7.17346838403706));
#13225=CARTESIAN_POINT('Ctrl Pts',(3.021151801193,-0.573684790634829,7.17865826678939));
#13226=CARTESIAN_POINT('Ctrl Pts',(3.03830301001047,-0.474581284233719,
7.18384814954172));
#13227=CARTESIAN_POINT('Ctrl Pts',(3.05056405627979,-0.37478152106769,7.18903803229404));
#13228=CARTESIAN_POINT('Ctrl Pts',(3.06280647431905,-0.275133383864656,
7.194220030048));
#13229=CARTESIAN_POINT('Ctrl Pts',(3.07017348425874,-0.174791477733736,
7.19940202780196));
#13230=CARTESIAN_POINT('Ctrl Pts',(3.07260306387723,-0.0742473019864619,
7.20458402555591));
#13231=CARTESIAN_POINT('Ctrl Pts',(3.07320310147929,-0.049415727973635,
7.2058638327631));
#13232=CARTESIAN_POINT('Ctrl Pts',(3.07350222572077,-0.0245718569918277,
7.20714363997028));
#13233=CARTESIAN_POINT('Ctrl Pts',(3.07349998753221,0.000276838377213211,
7.20842344717746));
#13234=CARTESIAN_POINT('Origin',(0.,0.,-2.20842344717744));
#13235=CARTESIAN_POINT('',(-1.87240768645123,2.4373123939533,5.56275985257814));
#13236=CARTESIAN_POINT('',(-1.87084604423464,2.43524047469653,5.64570902492364));
#13237=CARTESIAN_POINT('',(-1.87240768645123,2.4373123939533,-2.20842344717744));
#13238=CARTESIAN_POINT('',(3.07311034755939,0.00277269570115833,6.29157655282255));
#13239=CARTESIAN_POINT('Ctrl Pts',(-1.87084604423436,2.43524047469674,5.64570902492362));
#13240=CARTESIAN_POINT('Ctrl Pts',(-2.13486897241354,2.23583486155222,5.66280993199216));
#13241=CARTESIAN_POINT('Ctrl Pts',(-3.08290902783559,1.25484794830019,5.73270047498876));
#13242=CARTESIAN_POINT('Ctrl Pts',(-3.34186209072106,-1.41643565774369,
5.85538065391343));
#13243=CARTESIAN_POINT('Ctrl Pts',(-0.631386729895664,-3.57430874481187,
6.01374956169758));
#13244=CARTESIAN_POINT('Ctrl Pts',(2.38524471380796,-2.56562027744576,6.15914819466731));
#13245=CARTESIAN_POINT('Ctrl Pts',(3.06618249768684,-0.76621717896174,6.25175719170896));
#13246=CARTESIAN_POINT('Ctrl Pts',(3.07311034755939,0.00277269570115833,
6.29157655282255));
#13247=CARTESIAN_POINT('Ctrl Pts',(3.07311034755939,0.00277269570115833,
6.29157655282255));
#13248=CARTESIAN_POINT('Ctrl Pts',(3.07536694119141,0.253254112905881,6.30454682763701));
#13249=CARTESIAN_POINT('Ctrl Pts',(2.93303834198825,1.5206760271736,6.37030673837954));
#13250=CARTESIAN_POINT('Ctrl Pts',(1.1873595229057,3.42479583189181,6.48838938329588));
#13251=CARTESIAN_POINT('Ctrl Pts',(-1.07725235962685,3.053377230368,6.59350175339774));
#13252=CARTESIAN_POINT('Ctrl Pts',(-1.87543519516259,2.44126013959451,6.64582448757154));
#13253=CARTESIAN_POINT('',(3.07349882217906,-0.00269073669219618,6.2084234472256));
#13254=CARTESIAN_POINT('Ctrl Pts',(3.07349882217906,-0.00269073669218799,
6.2084234472256));
#13255=CARTESIAN_POINT('Ctrl Pts',(3.07358187200714,0.0921730786858093,
6.21334262298627));
#13256=CARTESIAN_POINT('Ctrl Pts',(3.06926874327925,0.187176666180301,6.21826179874695));
#13257=CARTESIAN_POINT('Ctrl Pts',(3.06054730741738,0.281873072605769,6.22318097450763));
#13258=CARTESIAN_POINT('Ctrl Pts',(3.05183388741538,0.376482443692495,6.22809562906053));
#13259=CARTESIAN_POINT('Ctrl Pts',(3.03872025259062,0.470784745903885,6.23301028361344));
#13260=CARTESIAN_POINT('Ctrl Pts',(3.02124633040207,0.564333997763762,6.23792493816634));
#13261=CARTESIAN_POINT('Ctrl Pts',(3.00378085463484,0.657838030445783,6.24283721710818));
#13262=CARTESIAN_POINT('Ctrl Pts',(2.98195935854854,0.750589291198084,6.24774949605002));
#13263=CARTESIAN_POINT('Ctrl Pts',(2.95587337233148,0.842148951636062,6.25266177499185));
#13264=CARTESIAN_POINT('Ctrl Pts',(2.92979239118119,0.933691044702462,6.25757311142441));
#13265=CARTESIAN_POINT('Ctrl Pts',(2.89944866936247,1.02404155634354,6.26248444785697));
#13266=CARTESIAN_POINT('Ctrl Pts',(2.86498409548813,1.11277508176634,6.26739578428952));
#13267=CARTESIAN_POINT('Ctrl Pts',(2.8305160875989,1.20151744850685,6.27230761008262));
#13268=CARTESIAN_POINT('Ctrl Pts',(2.79192657793376,1.28864208772415,6.27721943587571));
#13269=CARTESIAN_POINT('Ctrl Pts',(2.74940578904599,1.37374308266152,6.28213126166881));
#13270=CARTESIAN_POINT('Ctrl Pts',(2.70684237482433,1.45892938782994,6.2870480113643));
#13271=CARTESIAN_POINT('Ctrl Pts',(2.66034001807517,1.54208759401821,6.2919647610598));
#13272=CARTESIAN_POINT('Ctrl Pts',(2.61013494932703,1.62283634304312,6.2968815107553));
#13273=CARTESIAN_POINT('Ctrl Pts',(2.55990223285614,1.70362956006859,6.30180096808442));
#13274=CARTESIAN_POINT('Ctrl Pts',(2.50596300435945,1.78201030765024,6.30672042541354));
#13275=CARTESIAN_POINT('Ctrl Pts',(2.44859557063384,1.85762805251007,6.31163988274266));
#13276=CARTESIAN_POINT('Ctrl Pts',(2.39113686527861,1.93336610525806,6.31656716693205));
#13277=CARTESIAN_POINT('Ctrl Pts',(2.33023935842095,2.00633203472531,6.32149445112143));
#13278=CARTESIAN_POINT('Ctrl Pts',(2.26621999104809,2.0762102981572,6.32642173531081));
#13279=CARTESIAN_POINT('Ctrl Pts',(2.23012341357383,2.11561034619337,6.32919992732955));
#13280=CARTESIAN_POINT('Ctrl Pts',(2.1930350019566,2.15402947379665,6.33197811934829));
#13281=CARTESIAN_POINT('Ctrl Pts',(2.15501616577207,2.19141679633543,6.33475631136702));
#13282=CARTESIAN_POINT('Ctrl Pts',(2.08659917690504,2.25869734162852,6.33975582085999));
#13283=CARTESIAN_POINT('Ctrl Pts',(2.01490820660427,2.32288897701831,6.34475533035296));
#13284=CARTESIAN_POINT('Ctrl Pts',(1.94025347588063,2.38365658166883,6.34975483984593));
#13285=CARTESIAN_POINT('Ctrl Pts',(1.86570001382517,2.44434175544952,6.35474756753602));
#13286=CARTESIAN_POINT('Ctrl Pts',(1.78819111899676,2.50161185473718,6.35974029522612));
#13287=CARTESIAN_POINT('Ctrl Pts',(1.70807380396387,2.55516851307549,6.36473302291621));
#13288=CARTESIAN_POINT('Ctrl Pts',(1.62804101067879,2.60866867048928,6.36972048340444));
#13289=CARTESIAN_POINT('Ctrl Pts',(1.54540563062918,2.65846293222649,6.37470794389267));
#13290=CARTESIAN_POINT('Ctrl Pts',(1.46054689172026,2.70429381301039,6.3796954043809));
#13291=CARTESIAN_POINT('Ctrl Pts',(1.37574887122264,2.75009190072778,6.38467929622457));
#13292=CARTESIAN_POINT('Ctrl Pts',(1.28873103955486,2.791932037111,6.38966318806824));
#13293=CARTESIAN_POINT('Ctrl Pts',(1.19989984636415,2.82960113950629,6.3946470799119));
#13294=CARTESIAN_POINT('Ctrl Pts',(1.11110100329383,2.86725652374747,6.3996291567456));
#13295=CARTESIAN_POINT('Ctrl Pts',(1.02049051452189,2.90074372086693,6.4046112335793));
#13296=CARTESIAN_POINT('Ctrl Pts',(0.928496691140445,2.92989695118126,6.409593310413));
#13297=CARTESIAN_POINT('Ctrl Pts',(0.836511255476272,2.95904752339264,6.41457493299607));
#13298=CARTESIAN_POINT('Ctrl Pts',(0.743143154476896,2.98386478201134,6.41955655557915));
#13299=CARTESIAN_POINT('Ctrl Pts',(0.648836790001681,3.00423252594407,6.42453817816222));
#13300=CARTESIAN_POINT('Ctrl Pts',(0.554513278968048,3.02460397309147,6.42952070649203));
#13301=CARTESIAN_POINT('Ctrl Pts',(0.459251594733455,3.04052420624505,6.43450323482185));
#13302=CARTESIAN_POINT('Ctrl Pts',(0.363506224417138,3.05192815688869,6.43948576315167));
#13303=CARTESIAN_POINT('Ctrl Pts',(0.267657654702218,3.06334439931046,6.44447366191272));
#13304=CARTESIAN_POINT('Ctrl Pts',(0.171324794697949,3.07023458893296,6.44946156067377));
#13305=CARTESIAN_POINT('Ctrl Pts',(0.074966924490973,3.07258559038351,6.45444945943482));
#13306=CARTESIAN_POINT('Ctrl Pts',(-0.021447865632527,3.07493798060288,
6.45944030461614));
#13307=CARTESIAN_POINT('Ctrl Pts',(-0.11788725673191,3.07274585359341,6.46443114979745));
#13308=CARTESIAN_POINT('Ctrl Pts',(-0.213894429391949,3.06604817690053,
6.46942199497876));
#13309=CARTESIAN_POINT('Ctrl Pts',(-0.310056752067485,3.05933967659299,
6.47442090549192));
#13310=CARTESIAN_POINT('Ctrl Pts',(-0.405785025921967,3.04811113899375,
6.47941981600508));
#13311=CARTESIAN_POINT('Ctrl Pts',(-0.50063005071512,3.03245309977269,6.48441872651824));
#13312=CARTESIAN_POINT('Ctrl Pts',(-0.555693216142961,3.02336267878555,
6.48732089072923));
#13313=CARTESIAN_POINT('Ctrl Pts',(-0.610458900941248,3.01278025014737,
6.49022305494021));
#13314=CARTESIAN_POINT('Ctrl Pts',(-0.664841586868172,3.00073122994556,
6.4931252191512));
#13315=CARTESIAN_POINT('Ctrl Pts',(-0.758533571728651,2.97997284703214,
6.49812514735784));
#13316=CARTESIAN_POINT('Ctrl Pts',(-0.8514169915867,2.95478576948772,6.50312507556447));
#13317=CARTESIAN_POINT('Ctrl Pts',(-0.943041736551915,2.92524777294525,
6.50812500377111));
#13318=CARTESIAN_POINT('Ctrl Pts',(-1.03451892194578,2.89575734667553,6.51311687970689));
#13319=CARTESIAN_POINT('Ctrl Pts',(-1.12474105055002,2.86193007375763,6.51810875564268));
#13320=CARTESIAN_POINT('Ctrl Pts',(-1.21326914801803,2.82389451369339,6.52310063157846));
#13321=CARTESIAN_POINT('Ctrl Pts',(-1.30171457559361,2.78589447224695,6.5280878459677));
#13322=CARTESIAN_POINT('Ctrl Pts',(-1.38846871344482,2.74369412203258,6.53307506035695));
#13323=CARTESIAN_POINT('Ctrl Pts',(-1.47310917413638,2.69747133646962,6.53806227474619));
#13324=CARTESIAN_POINT('Ctrl Pts',(-1.55769019425479,2.65128101184608,6.5430459867575));
#13325=CARTESIAN_POINT('Ctrl Pts',(-1.64016010366088,2.60107407660144,6.54802969876881));
#13326=CARTESIAN_POINT('Ctrl Pts',(-1.72011891763209,2.54707541294015,6.55301341078012));
#13327=CARTESIAN_POINT('Ctrl Pts',(-1.77197177030419,2.51205757547788,6.55624532070785));
#13328=CARTESIAN_POINT('Ctrl Pts',(-1.82276904813623,2.4754461055598,6.55947723063557));
#13329=CARTESIAN_POINT('Ctrl Pts',(-1.87240768645124,2.43731239395329,6.5627091405633));
#13330=CARTESIAN_POINT('Ctrl Pts',(-1.87240768645123,2.4373123939533,5.56275985257814));
#13331=CARTESIAN_POINT('Ctrl Pts',(-1.94867787076473,2.37871962607096,5.56775071013256));
#13332=CARTESIAN_POINT('Ctrl Pts',(-2.02229488902666,2.31646673029867,5.57274156768697));
#13333=CARTESIAN_POINT('Ctrl Pts',(-2.09288995973404,2.25082515234845,5.57773242524139));
#13334=CARTESIAN_POINT('Ctrl Pts',(-2.16570558394975,2.18311883199131,5.58288026919926));
#13335=CARTESIAN_POINT('Ctrl Pts',(-2.23530558256172,2.1118073480244,5.58802811315714));
#13336=CARTESIAN_POINT('Ctrl Pts',(-2.30132069780014,2.03723471791462,5.59317595711501));
#13337=CARTESIAN_POINT('Ctrl Pts',(-2.36522302770871,1.96504875271235,5.59815904654424));
#13338=CARTESIAN_POINT('Ctrl Pts',(-2.42576613994928,1.88980756866498,5.60314213597346));
#13339=CARTESIAN_POINT('Ctrl Pts',(-2.48265241930305,1.81186070516713,5.60812522540269));
#13340=CARTESIAN_POINT('Ctrl Pts',(-2.53952351220385,1.73393465048978,5.61310698453832));
#13341=CARTESIAN_POINT('Ctrl Pts',(-2.5927394535247,1.65330470610248,5.61808874367394));
#13342=CARTESIAN_POINT('Ctrl Pts',(-2.64204400985501,1.57035209427353,5.62307050280957));
#13343=CARTESIAN_POINT('Ctrl Pts',(-2.69134886375604,1.48739898179575,5.62805229201191));
#13344=CARTESIAN_POINT('Ctrl Pts',(-2.73674206215645,1.40212355182324,5.63303408121425));
#13345=CARTESIAN_POINT('Ctrl Pts',(-2.7780122302168,1.31493357199741,5.63801587041658));
#13346=CARTESIAN_POINT('Ctrl Pts',(-2.8192939138382,1.22771926366548,5.64299904968105));
#13347=CARTESIAN_POINT('Ctrl Pts',(-2.85645009413505,1.13858974097728,5.64798222894551));
#13348=CARTESIAN_POINT('Ctrl Pts',(-2.88931707809965,1.04797379366171,5.65296540820997));
#13349=CARTESIAN_POINT('Ctrl Pts',(-2.92222118075134,0.957255508236955,
5.65795421528233));
#13350=CARTESIAN_POINT('Ctrl Pts',(-2.95082627120404,0.865047861450858,
5.66294302235469));
#13351=CARTESIAN_POINT('Ctrl Pts',(-2.97501828281642,0.771795612133184,
5.66793182942705));
#13352=CARTESIAN_POINT('Ctrl Pts',(-2.99922669399225,0.678480147891317,
5.67292401837023));
#13353=CARTESIAN_POINT('Ctrl Pts',(-3.01901598159721,0.584119100388228,
5.67791620731341));
#13354=CARTESIAN_POINT('Ctrl Pts',(-3.03432342957772,0.489166203570661,
5.68290839625659));
#13355=CARTESIAN_POINT('Ctrl Pts',(-3.04965407176638,0.394069431872271,
5.68790814948283));
#13356=CARTESIAN_POINT('Ctrl Pts',(-3.06048927543287,0.298379456239109,
5.69290790270908));
#13357=CARTESIAN_POINT('Ctrl Pts',(-3.06681826942858,0.202553578835506,
5.69790765593532));
#13358=CARTESIAN_POINT('Ctrl Pts',(-3.06824152970727,0.181004314438745,
5.69903199736699));
#13359=CARTESIAN_POINT('Ctrl Pts',(-3.06943711614308,0.159448168233771,
5.70015633879866));
#13360=CARTESIAN_POINT('Ctrl Pts',(-3.07040526815993,0.137890316033282,
5.70128068023033));
#13361=CARTESIAN_POINT('Ctrl Pts',(-3.07471026401133,0.0420309234247481,
5.7062801897233));
#13362=CARTESIAN_POINT('Ctrl Pts',(-3.07452936043882,-0.0541986383043321,
5.71127969921626));
#13363=CARTESIAN_POINT('Ctrl Pts',(-3.06982068590684,-0.150343627661687,
5.71627920870923));
#13364=CARTESIAN_POINT('Ctrl Pts',(-3.06511839866196,-0.246358196951463,
5.72127193639932));
#13365=CARTESIAN_POINT('Ctrl Pts',(-3.05590056835119,-0.342287987185201,
5.72626466408941));
#13366=CARTESIAN_POINT('Ctrl Pts',(-3.04217725314556,-0.437675462464726,
5.7312573917795));
#13367=CARTESIAN_POINT('Ctrl Pts',(-3.02846841569156,-0.532962306362232,
5.73624485226772));
#13368=CARTESIAN_POINT('Ctrl Pts',(-3.01026360454062,-0.627707540484224,
5.74123231275594));
#13369=CARTESIAN_POINT('Ctrl Pts',(-2.98762481780047,-0.721456996682917,
5.74621977324417));
#13370=CARTESIAN_POINT('Ctrl Pts',(-2.96500222964141,-0.815139372954289,
5.75120366508783));
#13371=CARTESIAN_POINT('Ctrl Pts',(-2.93795207564248,-0.907826962249409,
5.75618755693149));
#13372=CARTESIAN_POINT('Ctrl Pts',(-2.90658757484834,-0.999075032085795,
5.76117144877515));
#13373=CARTESIAN_POINT('Ctrl Pts',(-2.87523449622858,-1.09028987163512,
5.76615352560884));
#13374=CARTESIAN_POINT('Ctrl Pts',(-2.83957033511789,-1.18006581862899,
5.77113560244253));
#13375=CARTESIAN_POINT('Ctrl Pts',(-2.79975810543453,-1.26797350171589,
5.77611767927622));
#13376=CARTESIAN_POINT('Ctrl Pts',(-2.75994950570929,-1.35587316964736,
5.78109930185929));
#13377=CARTESIAN_POINT('Ctrl Pts',(-2.71599377062049,-1.44190451255417,
5.78608092444235));
#13378=CARTESIAN_POINT('Ctrl Pts',(-2.66810154393448,-1.52565933328985,
5.79106254702541));
#13379=CARTESIAN_POINT('Ctrl Pts',(-2.62020060959783,-1.60942938212764,
5.79604507535524));
#13380=CARTESIAN_POINT('Ctrl Pts',(-2.56836198016167,-1.69092170572364,
5.80102760368506));
#13381=CARTESIAN_POINT('Ctrl Pts',(-2.51284107053017,-1.76975478647658,
5.80601013201488));
#13382=CARTESIAN_POINT('Ctrl Pts',(-2.45726031754067,-1.84867283767229,
5.81099803077592));
#13383=CARTESIAN_POINT('Ctrl Pts',(-2.39798961388144,-1.92492556429473,
5.81598592953697));
#13384=CARTESIAN_POINT('Ctrl Pts',(-2.33532620329277,-1.99816259954343,
5.82097382829801));
#13385=CARTESIAN_POINT('Ctrl Pts',(-2.27262577656736,-2.0714428969141,5.82596467347932));
#13386=CARTESIAN_POINT('Ctrl Pts',(-2.20652895301908,-2.14170363625871,
5.83095551866062));
#13387=CARTESIAN_POINT('Ctrl Pts',(-2.13737008268281,-2.20863110990778,
5.83594636384193));
#13388=CARTESIAN_POINT('Ctrl Pts',(-2.06809944986559,-2.27566674004441,
5.84094527435508));
#13389=CARTESIAN_POINT('Ctrl Pts',(-1.99575721875399,-2.33935805868011,
5.84594418486824));
#13390=CARTESIAN_POINT('Ctrl Pts',(-1.9207109996448,-2.39943149638482,5.85094309538139));
#13391=CARTESIAN_POINT('Ctrl Pts',(-1.87714221586694,-2.43430769200422,
5.85384525959243));
#13392=CARTESIAN_POINT('Ctrl Pts',(-1.83266261781887,-2.46796528230561,
5.85674742380347));
#13393=CARTESIAN_POINT('Ctrl Pts',(-1.78734827456123,-2.50035765350139,
5.85964958801451));
#13394=CARTESIAN_POINT('Ctrl Pts',(-1.70928601729032,-2.5561594467553,5.86464909750748));
#13395=CARTESIAN_POINT('Ctrl Pts',(-1.62847091007287,-2.60840004133584,
5.86964860700046));
#13396=CARTESIAN_POINT('Ctrl Pts',(-1.54526158954145,-2.65679673100669,
5.87464811649343));
#13397=CARTESIAN_POINT('Ctrl Pts',(-1.46216514192501,-2.70512777087528,
5.87964084418353));
#13398=CARTESIAN_POINT('Ctrl Pts',(-1.37668131185556,-2.74962504996738,
5.88463357187361));
#13399=CARTESIAN_POINT('Ctrl Pts',(-1.2891993531016,-2.79004789886525,5.8896262995637));
#13400=CARTESIAN_POINT('Ctrl Pts',(-1.20180968560897,-2.83042810267648,
5.89461376005193));
#13401=CARTESIAN_POINT('Ctrl Pts',(-1.11242647631994,-2.86674223814857,
5.89960122054016));
#13402=CARTESIAN_POINT('Ctrl Pts',(-1.02146443293957,-2.89879503625894,
5.90458868102839));
#13403=CARTESIAN_POINT('Ctrl Pts',(-0.930567475027476,-2.93082489984302,
5.90957257287206));
#13404=CARTESIAN_POINT('Ctrl Pts',(-0.838094341623338,-2.95859934203635,
5.91455646471573));
#13405=CARTESIAN_POINT('Ctrl Pts',(-0.744479713188049,-2.98197119480578,
5.9195403565594));
#13406=CARTESIAN_POINT('Ctrl Pts',(-0.650899176881863,-3.0053345361253,
5.92452243339309));
#13407=CARTESIAN_POINT('Ctrl Pts',(-0.55617839695845,-3.02429836741265,
5.92950451022679));
#13408=CARTESIAN_POINT('Ctrl Pts',(-0.460766279977206,-3.03876565158223,
5.93448658706048));
#13409=CARTESIAN_POINT('Ctrl Pts',(-0.365362862382894,-3.05323161666879,
5.93946820964355));
#13410=CARTESIAN_POINT('Ctrl Pts',(-0.269268667082945,-3.06320178413059,
5.94444983222662));
#13411=CARTESIAN_POINT('Ctrl Pts',(-0.172940772022078,-3.06863059676013,
5.94943145480969));
#13412=CARTESIAN_POINT('Ctrl Pts',(-0.0765953628526493,-3.07406039644346,
5.95441398313951));
#13413=CARTESIAN_POINT('Ctrl Pts',(0.0199833922000153,-3.07494717679239,
5.95939651146934));
#13414=CARTESIAN_POINT('Ctrl Pts',(0.116336418072036,-3.07129746000451,
5.96437903979916));
#13415=CARTESIAN_POINT('Ctrl Pts',(0.21279329830562,-3.06764380935982,5.96936693856021));
#13416=CARTESIAN_POINT('Ctrl Pts',(0.309023524251918,-3.05944391643605,
5.97435483732126));
#13417=CARTESIAN_POINT('Ctrl Pts',(0.404571376123319,-3.04675634923794,
5.97934273608231));
#13418=CARTESIAN_POINT('Ctrl Pts',(0.500175669422252,-3.03406128731974,
5.98433358126362));
#13419=CARTESIAN_POINT('Ctrl Pts',(0.595096354296386,-3.01687335086815,
5.98932442644493));
#13420=CARTESIAN_POINT('Ctrl Pts',(0.688888257774321,-2.99530219148263,
5.99431527162624));
#13421=CARTESIAN_POINT('Ctrl Pts',(0.782831731336869,-2.9736961725588,5.9993141821394));
#13422=CARTESIAN_POINT('Ctrl Pts',(0.875642358699442,-2.94769290506517,
6.00431309265256));
#13423=CARTESIAN_POINT('Ctrl Pts',(0.966890525934692,-2.91745179237939,
6.00931200316572));
#13424=CARTESIAN_POINT('Ctrl Pts',(1.0198655020962,-2.89989503182007,6.0122141673767));
#13425=CARTESIAN_POINT('Ctrl Pts',(1.07231421576954,-2.88091081571002,6.01511633158769));
#13426=CARTESIAN_POINT('Ctrl Pts',(1.12415615175047,-2.86053757124104,6.01801849579868));
#13427=CARTESIAN_POINT('Ctrl Pts',(1.21346338326062,-2.82544092552406,6.02301800529165));
#13428=CARTESIAN_POINT('Ctrl Pts',(1.30128230224825,-2.78609631033278,6.02801751478463));
#13429=CARTESIAN_POINT('Ctrl Pts',(1.38718051662889,-2.74265062745607,6.03301702427761));
#13430=CARTESIAN_POINT('Ctrl Pts',(1.47296221062716,-2.69926387837233,6.0380097519677));
#13431=CARTESIAN_POINT('Ctrl Pts',(1.55682798976621,-2.65178731426579,6.0430024796578));
#13432=CARTESIAN_POINT('Ctrl Pts',(1.63836405257326,-2.60041640535429,6.0479952073479));
#13433=CARTESIAN_POINT('Ctrl Pts',(1.71981409688929,-2.54909969145681,6.05298266783613));
#13434=CARTESIAN_POINT('Ctrl Pts',(1.79893894139447,-2.49389703282577,6.05797012832436));
#13435=CARTESIAN_POINT('Ctrl Pts',(1.87534900768173,-2.43504996856064,6.06295758881259));
#13436=CARTESIAN_POINT('Ctrl Pts',(1.95170440078042,-2.37624501074557,6.06794148065626));
#13437=CARTESIAN_POINT('Ctrl Pts',(2.02534853045345,-2.3138010982686,6.07292537249993));
#13438=CARTESIAN_POINT('Ctrl Pts',(2.09592129083453,-2.24800271188149,6.0779092643436));
#13439=CARTESIAN_POINT('Ctrl Pts',(2.1664683503642,-2.18222828763702,6.0828913411773));
#13440=CARTESIAN_POINT('Ctrl Pts',(2.23394594223766,-2.11310211573837,6.08787341801099));
#13441=CARTESIAN_POINT('Ctrl Pts',(2.29802826461911,-2.0409479035516,6.09285549484469));
#13442=CARTESIAN_POINT('Ctrl Pts',(2.36210474416911,-1.96880027016666,6.09783711742776));
#13443=CARTESIAN_POINT('Ctrl Pts',(2.42278627835587,-1.89362547373654,6.10281874001084));
#13444=CARTESIAN_POINT('Ctrl Pts',(2.47978579734471,-1.81578210402225,6.10780036259391));
#13445=CARTESIAN_POINT('Ctrl Pts',(2.53679567985041,-1.73792458101177,6.11278289092374));
#13446=CARTESIAN_POINT('Ctrl Pts',(2.59012195831738,-1.6573978753062,6.11776541925357));
#13447=CARTESIAN_POINT('Ctrl Pts',(2.63952015937944,-1.57459060654811,6.1227479475834));
#13448=CARTESIAN_POINT('Ctrl Pts',(2.68897160442201,-1.49169408375831,6.12773584634445));
#13449=CARTESIAN_POINT('Ctrl Pts',(2.73448629423379,-1.40651246813039,6.1327237451055));
#13450=CARTESIAN_POINT('Ctrl Pts',(2.77586523785553,-1.31945990134799,6.13771164386656));
#13451=CARTESIAN_POINT('Ctrl Pts',(2.8172686245872,-1.23235591141961,6.14270248904787));
#13452=CARTESIAN_POINT('Ctrl Pts',(2.85453123114794,-1.14337917441077,6.14769333422918));
#13453=CARTESIAN_POINT('Ctrl Pts',(2.88750265733424,-1.05296279795998,6.15268417941049));
#13454=CARTESIAN_POINT('Ctrl Pts',(2.9205273661779,-0.962400306361512,6.15768308992365));
#13455=CARTESIAN_POINT('Ctrl Pts',(2.94924691696318,-0.870393948567786,
6.16268200043681));
#13456=CARTESIAN_POINT('Ctrl Pts',(2.97356111204012,-0.777390868844463,
6.16768091094997));
#13457=CARTESIAN_POINT('Ctrl Pts',(2.98767694519714,-0.723397061839546,
6.17058307516093));
#13458=CARTESIAN_POINT('Ctrl Pts',(3.0003089152176,-0.669067499346793,6.1734852393719));
#13459=CARTESIAN_POINT('Ctrl Pts',(3.01144541790487,-0.61449063864291,6.17638740358286));
#13460=CARTESIAN_POINT('Ctrl Pts',(3.03868361335526,-0.481003920176007,
6.18348565679818));
#13461=CARTESIAN_POINT('Ctrl Pts',(3.05705350500806,-0.345651342796243,
6.1905839100135));
#13462=CARTESIAN_POINT('Ctrl Pts',(3.06635784075604,-0.209408315102262,
6.19768216322882));
#13463=CARTESIAN_POINT('Ctrl Pts',(3.07105103823204,-0.140686006383418,
6.2012625912117));
#13464=CARTESIAN_POINT('Ctrl Pts',(3.07343837424032,-0.0717374795267619,
6.20484301919458));
#13465=CARTESIAN_POINT('Ctrl Pts',(3.07349882217824,-0.00269073762051493,
6.20842344717746));
#13466=CARTESIAN_POINT('Origin',(0.,0.,-2.20842344717744));
#13467=CARTESIAN_POINT('',(-1.87240768645123,2.4373123939533,4.56258760229939));
#13468=CARTESIAN_POINT('',(-1.87025628839741,2.4345543755422,4.64593736840472));
#13469=CARTESIAN_POINT('',(-1.87240768645123,2.4373123939533,-2.20842344717744));
#13470=CARTESIAN_POINT('',(3.06881272651402,-0.000977486742642815,5.29157655282255));
#13471=CARTESIAN_POINT('Ctrl Pts',(-1.87025628839757,2.43455437554208,4.64593736840473));
#13472=CARTESIAN_POINT('Ctrl Pts',(-2.38377235667202,2.03450370412233,4.67955767874455));
#13473=CARTESIAN_POINT('Ctrl Pts',(-3.39698165770904,0.598186149263013,
4.76596762501243));
#13474=CARTESIAN_POINT('Ctrl Pts',(-2.74378617582191,-2.37612491828059,
4.90516720720836));
#13475=CARTESIAN_POINT('Ctrl Pts',(0.499216583506413,-3.59515159745691,
5.06353611499254));
#13476=CARTESIAN_POINT('Ctrl Pts',(2.76686331140346,-1.92257446296493,5.19233923019727));
#13477=CARTESIAN_POINT('Ctrl Pts',(3.0701031042517,-0.451063181367307,5.26835270947394));
#13478=CARTESIAN_POINT('Ctrl Pts',(3.06881272651402,-0.000977486742642815,
5.29157655282255));
#13479=CARTESIAN_POINT('Ctrl Pts',(3.06881272651402,-0.000977486742642815,
5.29157655282255));
#13480=CARTESIAN_POINT('Ctrl Pts',(3.0671699734189,0.572017262252944,5.32114234540199));
#13481=CARTESIAN_POINT('Ctrl Pts',(2.6385116023052,2.17037498979142,5.4034977739095));
#13482=CARTESIAN_POINT('Ctrl Pts',(0.392306605071205,3.44445527983356,5.52154193127653));
#13483=CARTESIAN_POINT('Ctrl Pts',(-1.31984353549509,2.85138991238784,5.61002029606411));
#13484=CARTESIAN_POINT('Ctrl Pts',(-1.87084604423436,2.43524047469674,5.64570902492362));
#13485=CARTESIAN_POINT('',(3.07349942256352,0.00188401212730468,5.20842344714237));
#13486=CARTESIAN_POINT('Ctrl Pts',(3.07349942256311,0.00188401280199884,
5.20842344717746));
#13487=CARTESIAN_POINT('Ctrl Pts',(3.07342968576285,0.11564970223751,5.21434028374424));
#13488=CARTESIAN_POINT('Ctrl Pts',(3.06704369053517,0.229219670324171,5.22025712031102));
#13489=CARTESIAN_POINT('Ctrl Pts',(3.05440435245992,0.342076455889465,5.22617395687781));
#13490=CARTESIAN_POINT('Ctrl Pts',(3.04372457620137,0.437436292925306,5.23117346637075));
#13491=CARTESIAN_POINT('Ctrl Pts',(3.02855599778435,0.532463002356707,5.23617297586368));
#13492=CARTESIAN_POINT('Ctrl Pts',(3.00892809284608,0.626700871294788,5.24117248535662));
#13493=CARTESIAN_POINT('Ctrl Pts',(2.98932681303621,0.720810907162142,5.24616521304668));
#13494=CARTESIAN_POINT('Ctrl Pts',(2.96527831752864,0.814133803139797,5.25115794073675));
#13495=CARTESIAN_POINT('Ctrl Pts',(2.93686381305271,0.906219175244882,5.25615066842681));
#13496=CARTESIAN_POINT('Ctrl Pts',(2.90847928516275,0.998207399603617,5.26113812891501));
#13497=CARTESIAN_POINT('Ctrl Pts',(2.87573803355213,1.08896027823987,5.26612558940321));
#13498=CARTESIAN_POINT('Ctrl Pts',(2.83877204625539,1.17803884460529,5.27111304989142));
#13499=CARTESIAN_POINT('Ctrl Pts',(2.80183250898673,1.26705367317406,5.27609694173504));
#13500=CARTESIAN_POINT('Ctrl Pts',(2.76067441317566,1.35439616678284,5.28108083357867));
#13501=CARTESIAN_POINT('Ctrl Pts',(2.71547887272697,1.43964465816169,5.2860647254223));
#13502=CARTESIAN_POINT('Ctrl Pts',(2.67029979137473,1.52486210415137,5.29104680225596));
#13503=CARTESIAN_POINT('Ctrl Pts',(2.62108639218778,1.6079866756494,5.29602887908962));
#13504=CARTESIAN_POINT('Ctrl Pts',(2.56806658326335,1.68861963565692,5.30101095592328));
#13505=CARTESIAN_POINT('Ctrl Pts',(2.51505160852398,1.76924524379617,5.30599257850631));
#13506=CARTESIAN_POINT('Ctrl Pts',(2.45823115538501,1.84737932544126,5.31097420108934));
#13507=CARTESIAN_POINT('Ctrl Pts',(2.39787688202416,1.92265147872777,5.31595582367237));
#13508=CARTESIAN_POINT('Ctrl Pts',(2.33751163519306,1.99793731781794,5.32093835200216));
#13509=CARTESIAN_POINT('Ctrl Pts',(2.2736115667338,2.07035985269263,5.32592088033194));
#13510=CARTESIAN_POINT('Ctrl Pts',(2.20648840351205,2.13958200945111,5.33090340866173));
#13511=CARTESIAN_POINT('Ctrl Pts',(2.1392928914128,2.20887877749277,5.33589130742274));
#13512=CARTESIAN_POINT('Ctrl Pts',(2.06886765507404,2.27496796508148,5.34087920618375));
#13513=CARTESIAN_POINT('Ctrl Pts',(1.9955608871673,2.33754978462664,5.34586710494477));
#13514=CARTESIAN_POINT('Ctrl Pts',(1.92221081594657,2.40016857211159,5.35085795012604));
#13515=CARTESIAN_POINT('Ctrl Pts',(1.84597617062353,2.45927559731828,5.35584879530731));
#13516=CARTESIAN_POINT('Ctrl Pts',(1.7672360867378,2.51461306441601,5.36083964048859));
#13517=CARTESIAN_POINT('Ctrl Pts',(1.68836875688804,2.57003995825803,5.36583855100171));
#13518=CARTESIAN_POINT('Ctrl Pts',(1.60698827419281,2.62168489516321,5.37083746151483));
#13519=CARTESIAN_POINT('Ctrl Pts',(1.52350037602741,2.66933490859509,5.37583637202795));
#13520=CARTESIAN_POINT('Ctrl Pts',(1.47503069658438,2.69699856916447,5.37873853623929));
#13521=CARTESIAN_POINT('Ctrl Pts',(1.42585114590227,2.72331662043663,5.38164070045063));
#13522=CARTESIAN_POINT('Ctrl Pts',(1.37604412559674,2.74825486707669,5.38454286466197));
#13523=CARTESIAN_POINT('Ctrl Pts',(1.29024240911866,2.79121556527837,5.38954237415494));
#13524=CARTESIAN_POINT('Ctrl Pts',(1.20227618216278,2.83022971901549,5.39454188364791));
#13525=CARTESIAN_POINT('Ctrl Pts',(1.11254374124125,2.86507393863141,5.39954139314088));
#13526=CARTESIAN_POINT('Ctrl Pts',(1.02293302180603,2.89987089228469,5.40453412083097));
#13527=CARTESIAN_POINT('Ctrl Pts',(0.931561255708756,2.93050899617844,5.40952684852107));
#13528=CARTESIAN_POINT('Ctrl Pts',(0.838850434690195,2.95681115362819,5.41451957621116));
#13529=CARTESIAN_POINT('Ctrl Pts',(0.746237421251002,2.98308556296478,5.41950703669938));
#13530=CARTESIAN_POINT('Ctrl Pts',(0.652288581242648,3.00503300014876,5.4244944971876));
#13531=CARTESIAN_POINT('Ctrl Pts',(0.557443977510773,3.02252517970272,5.42948195767582));
#13532=CARTESIAN_POINT('Ctrl Pts',(0.462667237309793,3.04000484319334,5.43446584951948));
#13533=CARTESIAN_POINT('Ctrl Pts',(0.36699643798775,3.0530355069444,5.43944974136315));
#13534=CARTESIAN_POINT('Ctrl Pts',(0.270883878545778,3.0615395104986,5.44443363320681));
#13535=CARTESIAN_POINT('Ctrl Pts',(0.174806320917514,3.07004041710532,5.4494157100405));
#13536=CARTESIAN_POINT('Ctrl Pts',(0.0782877596238715,3.07401790025223,
5.45439778687419));
#13537=CARTESIAN_POINT('Ctrl Pts',(-0.018213262897366,3.07344603451153,
5.45937986370788));
#13538=CARTESIAN_POINT('Ctrl Pts',(-0.114705486748633,3.0728742209118,5.46436148629095));
#13539=CARTESIAN_POINT('Ctrl Pts',(-0.211179736053418,3.06775388589988,
5.46934310887402));
#13540=CARTESIAN_POINT('Ctrl Pts',(-0.307177415866493,3.05811122838617,
5.47432473145708));
#13541=CARTESIAN_POINT('Ctrl Pts',(-0.40319254974915,3.04846681766743,5.47930725978691));
#13542=CARTESIAN_POINT('Ctrl Pts',(-0.49873050529916,3.03429849538759,5.48428978811673));
#13543=CARTESIAN_POINT('Ctrl Pts',(-0.593338827350413,3.0156842152252,5.48927231644655));
#13544=CARTESIAN_POINT('Ctrl Pts',(-0.688049123229613,2.99704987161215,
5.4942602152076));
#13545=CARTESIAN_POINT('Ctrl Pts',(-0.781827353774678,2.9739600880389,5.49924811396864));
#13546=CARTESIAN_POINT('Ctrl Pts',(-0.874232485423852,2.94654370601042,
5.50423601272969));
#13547=CARTESIAN_POINT('Ctrl Pts',(-0.966692202052608,2.91911112874878,
5.509226857911));
#13548=CARTESIAN_POINT('Ctrl Pts',(-1.05777679044786,2.88734700852964,5.5142177030923));
#13549=CARTESIAN_POINT('Ctrl Pts',(-1.14706359251928,2.85142900397621,5.51920854827361));
#13550=CARTESIAN_POINT('Ctrl Pts',(-1.23649468431763,2.81545295502038,5.52420745878676));
#13551=CARTESIAN_POINT('Ctrl Pts',(-1.32412178980427,2.77530980048819,5.52920636929992));
#13552=CARTESIAN_POINT('Ctrl Pts',(-1.40954536994406,2.73122391979663,5.53420527981307));
#13553=CARTESIAN_POINT('Ctrl Pts',(-1.45913882763995,2.70562944979801,5.5371074440241));
#13554=CARTESIAN_POINT('Ctrl Pts',(-1.50799008914286,2.67870692619843,5.54000960823512));
#13555=CARTESIAN_POINT('Ctrl Pts',(-1.55602560798146,2.65050684913394,5.54291177244615));
#13556=CARTESIAN_POINT('Ctrl Pts',(-1.63877544569276,2.60192713443629,5.54791127330053));
#13557=CARTESIAN_POINT('Ctrl Pts',(-1.71939343083612,2.54938315646748,5.55291077415492));
#13558=CARTESIAN_POINT('Ctrl Pts',(-1.79747533480956,2.49308737727968,5.5579102750093));
#13559=CARTESIAN_POINT('Ctrl Pts',(-1.82272213851202,2.47488484360536,5.55952680086558));
#13560=CARTESIAN_POINT('Ctrl Pts',(-1.8477039709751,2.45629043995846,5.56114332672186));
#13561=CARTESIAN_POINT('Ctrl Pts',(-1.87240768645123,2.4373123939533,5.56275985257814));
#13562=CARTESIAN_POINT('Ctrl Pts',(-1.87240768645123,2.4373123939533,4.56258760229939));
#13563=CARTESIAN_POINT('Ctrl Pts',(-1.94922488799432,2.37829939300283,4.56760605620634));
#13564=CARTESIAN_POINT('Ctrl Pts',(-2.02316578639418,2.315715664159,4.57262451011329));
#13565=CARTESIAN_POINT('Ctrl Pts',(-2.09389869348013,2.24988677747175,4.57764296402024));
#13566=CARTESIAN_POINT('Ctrl Pts',(-2.16463160056609,2.18405789078449,4.5826614179272));
#13567=CARTESIAN_POINT('Ctrl Pts',(-2.23215624896084,2.11498420753435,4.58767987183415));
#13568=CARTESIAN_POINT('Ctrl Pts',(-2.29618206790087,2.04302475781634,4.5926983257411));
#13569=CARTESIAN_POINT('Ctrl Pts',(-2.35996619256591,1.97133695143401,4.59769783523471));
#13570=CARTESIAN_POINT('Ctrl Pts',(-2.42050194477723,1.89653331526934,4.60269734472831));
#13571=CARTESIAN_POINT('Ctrl Pts',(-2.47747009481934,1.81894040014396,4.60769685422192));
#13572=CARTESIAN_POINT('Ctrl Pts',(-2.53436096792775,1.7414527393151,4.61268958191266));
#13573=CARTESIAN_POINT('Ctrl Pts',(-2.58769359935125,1.66118367006765,4.61768230960339));
#13574=CARTESIAN_POINT('Ctrl Pts',(-2.63718730318107,1.5784946556579,4.62267503729413));
#13575=CARTESIAN_POINT('Ctrl Pts',(-2.68662879240102,1.49589287607388,4.62766249778301));
#13576=CARTESIAN_POINT('Ctrl Pts',(-2.73223918088222,1.41087660114449,4.63264995827189));
#13577=CARTESIAN_POINT('Ctrl Pts',(-2.77378021992166,1.32383743018974,4.63763741876078));
#13578=CARTESIAN_POINT('Ctrl Pts',(-2.81529153537671,1.2368605377962,4.6426213106051));
#13579=CARTESIAN_POINT('Ctrl Pts',(-2.85273910121061,1.1478640218185,4.64760520244944));
#13580=CARTESIAN_POINT('Ctrl Pts',(-2.88593037390322,1.05726445461048,4.65258909429376));
#13581=CARTESIAN_POINT('Ctrl Pts',(-2.91910955915642,0.966697881520837,
4.65757117112813));
#13582=CARTESIAN_POINT('Ctrl Pts',(-2.94803538017669,0.8745298288834,4.66255324796249));
#13583=CARTESIAN_POINT('Ctrl Pts',(-2.97256362798983,0.781196343790704,
4.66753532479685));
#13584=CARTESIAN_POINT('Ctrl Pts',(-2.99708963939189,0.687871368561476,
4.67251694738059));
#13585=CARTESIAN_POINT('Ctrl Pts',(-3.01721876336985,0.593381596735652,
4.67749856996433));
#13586=CARTESIAN_POINT('Ctrl Pts',(-3.03285711043859,0.498176673141256,
4.68248019254807));
#13587=CARTESIAN_POINT('Ctrl Pts',(-3.04849830083437,0.402954439614213,
4.68746272087858));
#13588=CARTESIAN_POINT('Ctrl Pts',(-3.0596470216313,0.307017229243321,4.69244524920908));
#13589=CARTESIAN_POINT('Ctrl Pts',(-3.06626095532859,0.210822209046808,
4.69742777753958));
#13590=CARTESIAN_POINT('Ctrl Pts',(-3.07288201787166,0.114523504795564,
4.70241567630131));
#13591=CARTESIAN_POINT('Ctrl Pts',(-3.07495850504973,0.0179668746095363,
4.70740357506304));
#13592=CARTESIAN_POINT('Ctrl Pts',(-3.07250020693417,-0.0783883179400242,
4.71239147382477));
#13593=CARTESIAN_POINT('Ctrl Pts',(-3.07004045666818,-0.174800428824401,
4.71738231900676));
#13594=CARTESIAN_POINT('Ctrl Pts',(-3.06304061909772,-0.271010427539188,
4.72237316418875));
#13595=CARTESIAN_POINT('Ctrl Pts',(-3.05156239961503,-0.366564007038006,
4.72736400937074));
#13596=CARTESIAN_POINT('Ctrl Pts',(-3.0400656310398,-0.462272003534262,
4.73236291988458));
#13597=CARTESIAN_POINT('Ctrl Pts',(-3.02407610227852,-0.557321030063018,
4.73736183039841));
#13598=CARTESIAN_POINT('Ctrl Pts',(-3.00370664260785,-0.651266961509247,
4.74236074091225));
#13599=CARTESIAN_POINT('Ctrl Pts',(-2.99188096248128,-0.705808149760561,
4.74526290511659));
#13600=CARTESIAN_POINT('Ctrl Pts',(-2.97857997043236,-0.759977805689979,
4.74816506932093));
#13601=CARTESIAN_POINT('Ctrl Pts',(-2.96383331659785,-0.813691785275364,
4.75106723352527));
#13602=CARTESIAN_POINT('Ctrl Pts',(-2.93842950391147,-0.90622395503668,
4.75606674301803));
#13603=CARTESIAN_POINT('Ctrl Pts',(-2.90864357578993,-0.997727833434325,
4.76106625251079));
#13604=CARTESIAN_POINT('Ctrl Pts',(-2.87457563542604,-1.08775786194123,
4.76606576200356));
#13605=CARTESIAN_POINT('Ctrl Pts',(-2.84055390800695,-1.17766576528609,
4.77105848969344));
#13606=CARTESIAN_POINT('Ctrl Pts',(-2.80226186642582,-1.2661033851133,4.77605121738332));
#13607=CARTESIAN_POINT('Ctrl Pts',(-2.75984988339205,-1.35263848501397,
4.7810439450732));
#13608=CARTESIAN_POINT('Ctrl Pts',(-2.71748264393132,-1.43908229256549,
4.78603140556121));
#13609=CARTESIAN_POINT('Ctrl Pts',(-2.67100429562576,-1.52362717813468,
4.79101886604923));
#13610=CARTESIAN_POINT('Ctrl Pts',(-2.62061359408541,-1.60586009368648,
4.79600632653724));
#13611=CARTESIAN_POINT('Ctrl Pts',(-2.57025894826994,-1.68803416966495,
4.80099021838069));
#13612=CARTESIAN_POINT('Ctrl Pts',(-2.5159977429492,-1.76789919102667,4.80597411022414));
#13613=CARTESIAN_POINT('Ctrl Pts',(-2.45807456517958,-1.84506685028408,
4.8109580020676));
#13614=CARTESIAN_POINT('Ctrl Pts',(-2.4001724815967,-1.92220640699123,4.81594007890107));
#13615=CARTESIAN_POINT('Ctrl Pts',(-2.33861133852885,-1.99665020263482,
4.82092215573455));
#13616=CARTESIAN_POINT('Ctrl Pts',(-2.27367837411193,-2.06803986931967,
4.82590423256803));
#13617=CARTESIAN_POINT('Ctrl Pts',(-2.20875133008542,-2.13942302691163,
4.83088585515088));
#13618=CARTESIAN_POINT('Ctrl Pts',(-2.14045337143884,-2.20775228458013,
4.83586747773373));
#13619=CARTESIAN_POINT('Ctrl Pts',(-2.06911053850813,-2.27270407872089,
4.84084910031658));
#13620=CARTESIAN_POINT('Ctrl Pts',(-1.99775473419338,-2.33766768224224,
4.84583162864619));
#13621=CARTESIAN_POINT('Ctrl Pts',(-1.92335328073249,-2.39925230718283,
4.8508141569758));
#13622=CARTESIAN_POINT('Ctrl Pts',(-1.84626660646391,-2.45717355265277,
4.85579668530541));
#13623=CARTESIAN_POINT('Ctrl Pts',(-1.76909684412133,-2.51515722868902,
4.86078458406624));
#13624=CARTESIAN_POINT('Ctrl Pts',(-1.68923643434323,-2.56946937814897,
4.86577248282708));
#13625=CARTESIAN_POINT('Ctrl Pts',(-1.60707601796877,-2.61986811165556,
4.87076038158791));
#13626=CARTESIAN_POINT('Ctrl Pts',(-1.52486706830866,-2.67029661638577,
4.875751226769));
#13627=CARTESIAN_POINT('Ctrl Pts',(-1.44035579115729,-2.71680689062622,
4.88074207195009));
#13628=CARTESIAN_POINT('Ctrl Pts',(-1.35395685135728,-2.7592033442033,4.88573291713119));
#13629=CARTESIAN_POINT('Ctrl Pts',(-1.26741828868862,-2.80166831152005,
4.89073182764413));
#13630=CARTESIAN_POINT('Ctrl Pts',(-1.17898637464839,-2.84000600902761,
4.89573073815708));
#13631=CARTESIAN_POINT('Ctrl Pts',(-1.08909506803239,-2.87406927244065,
4.90072964867002));
#13632=CARTESIAN_POINT('Ctrl Pts',(-1.03690782994163,-2.89384501833651,
4.90363181288317));
#13633=CARTESIAN_POINT('Ctrl Pts',(-0.984228994413888,-2.91218100261231,
4.90653397709631));
#13634=CARTESIAN_POINT('Ctrl Pts',(-0.931145283869829,-2.92905628322963,
4.90943614130945));
#13635=CARTESIAN_POINT('Ctrl Pts',(-0.839698868266351,-2.95812704540771,
4.91443565080237));
#13636=CARTESIAN_POINT('Ctrl Pts',(-0.74672912593629,-2.98296226812754,
4.91943516029529));
#13637=CARTESIAN_POINT('Ctrl Pts',(-0.652664289274368,-3.00340333213939,
4.92443466978821));
#13638=CARTESIAN_POINT('Ctrl Pts',(-0.558727050966137,-3.02381666797769,
4.92942739747825));
#13639=CARTESIAN_POINT('Ctrl Pts',(-0.463698095917904,-3.03984759908492,
4.93442012516828));
#13640=CARTESIAN_POINT('Ctrl Pts',(-0.36802185135121,-3.05138692514208,
4.93941285285832));
#13641=CARTESIAN_POINT('Ctrl Pts',(-0.272446542810913,-3.06291407750111,
4.94440031334649));
#13642=CARTESIAN_POINT('Ctrl Pts',(-0.176225735751422,-3.06995899243969,
4.94938777383466));
#13643=CARTESIAN_POINT('Ctrl Pts',(-0.0798141044801399,-3.07246349998271,
4.95437523432283));
#13644=CARTESIAN_POINT('Ctrl Pts',(0.0165285420153408,-3.07496621549205,
4.95935912616644));
#13645=CARTESIAN_POINT('Ctrl Pts',(0.113061303733088,-3.07293497063588,
4.96434301801005));
#13646=CARTESIAN_POINT('Ctrl Pts',(0.209325305543598,-3.06636350853239,
4.96932690985366));
#13647=CARTESIAN_POINT('Ctrl Pts',(0.305554250388853,-3.05979443959265,
4.97430898668729));
#13648=CARTESIAN_POINT('Ctrl Pts',(0.401514192299747,-3.04868846846636,
4.97929106352093));
#13649=CARTESIAN_POINT('Ctrl Pts',(0.496748147799032,-3.03309141432602,
4.98427314035457));
#13650=CARTESIAN_POINT('Ctrl Pts',(0.591973420155595,-3.01749578227769,
4.98925476293758));
#13651=CARTESIAN_POINT('Ctrl Pts',(0.68647240454356,-2.9974099524712,4.99423638552059));
#13652=CARTESIAN_POINT('Ctrl Pts',(0.779796185138011,-2.97293124031556,
4.99921800810359));
#13653=CARTESIAN_POINT('Ctrl Pts',(0.873136933640147,-2.94844807749873,
5.00420053643336));
#13654=CARTESIAN_POINT('Ctrl Pts',(0.965301629408796,-2.91957055751148,
5.00918306476313));
#13655=CARTESIAN_POINT('Ctrl Pts',(1.0558554834001,-2.886446162355,5.0141655930929));
#13656=CARTESIAN_POINT('Ctrl Pts',(1.14650694110024,-2.85328606398241,5.01915349185389));
#13657=CARTESIAN_POINT('Ctrl Pts',(1.23554367782967,-2.81587010292265,5.02414139061488));
#13658=CARTESIAN_POINT('Ctrl Pts',(1.3225501136303,-2.77439424864897,5.02912928937587));
#13659=CARTESIAN_POINT('Ctrl Pts',(1.4096079453268,-2.73289389401888,5.03412013455712));
#13660=CARTESIAN_POINT('Ctrl Pts',(1.49463270131337,-2.68732907814428,5.03911097973837));
#13661=CARTESIAN_POINT('Ctrl Pts',(1.57723455714045,-2.63794112932074,5.04410182491962));
#13662=CARTESIAN_POINT('Ctrl Pts',(1.65996989965248,-2.58847336832471,5.04910073543271));
#13663=CARTESIAN_POINT('Ctrl Pts',(1.74027415819936,-2.53517038031442,5.05409964594581));
#13664=CARTESIAN_POINT('Ctrl Pts',(1.81778762297006,-2.47831604275501,5.0590985564589));
#13665=CARTESIAN_POINT('Ctrl Pts',(1.8627887892808,-2.44530872579961,5.06200072067047));
#13666=CARTESIAN_POINT('Ctrl Pts',(1.9068499456451,-2.41110518024639,5.06490288488204));
#13667=CARTESIAN_POINT('Ctrl Pts',(1.94990630988549,-2.37576674626714,5.06780504909361));
#13668=CARTESIAN_POINT('Ctrl Pts',(2.02310041339419,-2.31569281666009,5.07273861260852));
#13669=CARTESIAN_POINT('Ctrl Pts',(2.0936608174452,-2.25211385751832,5.07767217612343));
#13670=CARTESIAN_POINT('Ctrl Pts',(2.16122630734251,-2.18529245146975,5.08260573963834));
#13671=CARTESIAN_POINT('Ctrl Pts',(2.22869969055807,-2.11856213775234,5.0875325776168));
#13672=CARTESIAN_POINT('Ctrl Pts',(2.29318595058021,-2.04859847115308,5.09245941559526));
#13673=CARTESIAN_POINT('Ctrl Pts',(2.35435603556388,-1.97570491415189,5.09738625357373));
#13674=CARTESIAN_POINT('Ctrl Pts',(2.41545719842112,-1.90289348845643,5.10230754033953));
#13675=CARTESIAN_POINT('Ctrl Pts',(2.47324932477958,-1.82715907853083,5.10722882710534));
#13676=CARTESIAN_POINT('Ctrl Pts',(2.52744035697135,-1.74884175726466,5.11215011387114));
#13677=CARTESIAN_POINT('Ctrl Pts',(2.58159824009642,-1.67057234329976,5.11706839024839));
#13678=CARTESIAN_POINT('Ctrl Pts',(2.63215914616383,-1.58972352520295,5.12198666662564));
#13679=CARTESIAN_POINT('Ctrl Pts',(2.678872048634,-1.50666744739757,5.12690494300289));
#13680=CARTESIAN_POINT('Ctrl Pts',(2.72556993901313,-1.42363806126268,5.13182163879729));
#13681=CARTESIAN_POINT('Ctrl Pts',(2.76842206103465,-1.33840321787111,5.13673833459168));
#13682=CARTESIAN_POINT('Ctrl Pts',(2.8072220542146,-1.25136189343097,5.14165503038608));
#13683=CARTESIAN_POINT('Ctrl Pts',(2.84602084260932,-1.16432327172591,5.14657157351131));
#13684=CARTESIAN_POINT('Ctrl Pts',(2.88076757018275,-1.07547869382835,5.15148811663654));
#13685=CARTESIAN_POINT('Ctrl Pts',(2.91130349058757,-0.985248311692343,
5.15640465976177));
#13686=CARTESIAN_POINT('Ctrl Pts',(2.94186355432602,-0.8949465885851,5.16132509016924));
#13687=CARTESIAN_POINT('Ctrl Pts',(2.96820601883254,-0.803257302184073,
5.16624552057671));
#13688=CARTESIAN_POINT('Ctrl Pts',(2.99022180531888,-0.710616496427913,
5.17116595098418));
#13689=CARTESIAN_POINT('Ctrl Pts',(3.01224721692289,-0.617935188886504,
5.17608853256265));
#13690=CARTESIAN_POINT('Ctrl Pts',(3.02994210090488,-0.52430197766384,5.18101111414113));
#13691=CARTESIAN_POINT('Ctrl Pts',(3.04324877593432,-0.430161757684539,
5.18593369571961));
#13692=CARTESIAN_POINT('Ctrl Pts',(3.05657391129798,-0.335890937091645,
5.19086310638957));
#13693=CARTESIAN_POINT('Ctrl Pts',(3.06549864354479,-0.241112153047857,
5.19579251705953));
#13694=CARTESIAN_POINT('Ctrl Pts',(3.0700173061377,-0.146273681894655,5.2007219277295));
#13695=CARTESIAN_POINT('Ctrl Pts',(3.0723705670046,-0.0968830362660627,
5.20328910086712));
#13696=CARTESIAN_POINT('Ctrl Pts',(3.07352967967375,-0.0474761854391445,
5.20585627400474));
#13697=CARTESIAN_POINT('Ctrl Pts',(3.07349942256352,0.00188401212731454,
5.20842344714237));
#13698=CARTESIAN_POINT('Origin',(0.,0.,-2.20842344717744));
#13699=CARTESIAN_POINT('',(-1.87240768645123,2.4373123939533,3.56268206416256));
#13700=CARTESIAN_POINT('',(-1.87526655020737,2.4410026577968,3.64588021366773));
#13701=CARTESIAN_POINT('',(-1.87240768645123,2.4373123939533,-2.20842344717744));
#13702=CARTESIAN_POINT('',(3.0766413087884,-0.00205726601264529,4.29157655282254));
#13703=CARTESIAN_POINT('Ctrl Pts',(-1.87526655020737,2.4410026577968,3.64588021366773));
#13704=CARTESIAN_POINT('Ctrl Pts',(-2.6388745207397,1.84934209790722,3.69611509335153));
#13705=CARTESIAN_POINT('Ctrl Pts',(-3.59964389029708,-0.162448805822295,
3.7991396089634));
#13706=CARTESIAN_POINT('Ctrl Pts',(-1.87939887603769,-3.10518792817496,
3.9549537605033));
#13707=CARTESIAN_POINT('Ctrl Pts',(1.58136602653418,-3.26704969305195,4.11332266828749));
#13708=CARTESIAN_POINT('Ctrl Pts',(3.01256814619275,-1.2727511792973,4.22553026572723));
#13709=CARTESIAN_POINT('Ctrl Pts',(3.07762631741651,-0.129684115097173,
4.28494822723892));
#13710=CARTESIAN_POINT('Ctrl Pts',(3.0766413087884,-0.00205726601264529,
4.29157655282254));
#13711=CARTESIAN_POINT('Ctrl Pts',(3.0766413087884,-0.00205726601264529,
4.29157655282254));
#13712=CARTESIAN_POINT('Ctrl Pts',(3.06978146335676,0.886767900244137,4.33773786316697));
#13713=CARTESIAN_POINT('Ctrl Pts',(2.19813638014636,2.80377976238209,4.43668880943947));
#13714=CARTESIAN_POINT('Ctrl Pts',(-0.332778404768295,3.3251151002074,4.55480908130019));
#13715=CARTESIAN_POINT('Ctrl Pts',(-1.57746432401505,2.66265166241204,4.62676804281649));
#13716=CARTESIAN_POINT('Ctrl Pts',(-1.87025628839757,2.43455437554208,4.64593736840473));
#13717=CARTESIAN_POINT('',(3.07349977118744,0.00118596406329618,4.20842344720459));
#13718=CARTESIAN_POINT('Ctrl Pts',(3.07349977118744,0.0011859640632942,
4.20842344720459));
#13719=CARTESIAN_POINT('Ctrl Pts',(3.07345762577915,0.110408415858429,4.21405153578527));
#13720=CARTESIAN_POINT('Ctrl Pts',(3.06758844717546,0.219451566274083,4.21967962436595));
#13721=CARTESIAN_POINT('Ctrl Pts',(3.05597865567641,0.32771436656059,4.22530771294663));
#13722=CARTESIAN_POINT('Ctrl Pts',(3.04477419211802,0.432197431621468,4.23073931035393));
#13723=CARTESIAN_POINT('Ctrl Pts',(3.02822341389494,0.535953470165536,4.23617090776124));
#13724=CARTESIAN_POINT('Ctrl Pts',(3.00645543745351,0.638457479090209,4.24160250516854));
#13725=CARTESIAN_POINT('Ctrl Pts',(2.9835062573314,0.74652370060515,4.24732883933591));
#13726=CARTESIAN_POINT('Ctrl Pts',(2.95475800374141,0.853197801579446,4.25305517350328));
#13727=CARTESIAN_POINT('Ctrl Pts',(2.9204200294079,0.957887833638757,4.25878150767065));
#13728=CARTESIAN_POINT('Ctrl Pts',(2.8860820550744,1.06257786569806,4.26450784183801));
#13729=CARTESIAN_POINT('Ctrl Pts',(2.84615458915048,1.16528350102013,4.27023417600538));
#13730=CARTESIAN_POINT('Ctrl Pts',(2.80090335865945,1.26544167208537,4.27596051017275));
#13731=CARTESIAN_POINT('Ctrl Pts',(2.76139571734074,1.3528870974284,4.28096001966454));
#13732=CARTESIAN_POINT('Ctrl Pts',(2.71771963212303,1.43863417231869,4.28595952915634));
#13733=CARTESIAN_POINT('Ctrl Pts',(2.67004338983875,1.52225837044123,4.29095903864814));
#13734=CARTESIAN_POINT('Ctrl Pts',(2.62243182007454,1.60576913286978,4.29595176633705));
#13735=CARTESIAN_POINT('Ctrl Pts',(2.57083109298431,1.68716236360383,4.30094449402595));
#13736=CARTESIAN_POINT('Ctrl Pts',(2.51545707606337,1.76603452641298,4.30593722171486));
#13737=CARTESIAN_POINT('Ctrl Pts',(2.46014147733459,1.84482348107832,4.31092468220189));
#13738=CARTESIAN_POINT('Ctrl Pts',(2.40106075310402,1.92109629771701,4.31591214268892));
#13739=CARTESIAN_POINT('Ctrl Pts',(2.33847557414465,1.99447593094748,4.32089960317596));
#13740=CARTESIAN_POINT('Ctrl Pts',(2.27593517634376,2.06780305933514,4.32588349501843));
#13741=CARTESIAN_POINT('Ctrl Pts',(2.20989559268149,2.13824078662851,4.3308673868609));
#13742=CARTESIAN_POINT('Ctrl Pts',(2.14065891202591,2.20544364524783,4.33585127870338));
#13743=CARTESIAN_POINT('Ctrl Pts',(2.07144744565466,2.27262203025043,4.34083335553588));
#13744=CARTESIAN_POINT('Ctrl Pts',(1.99904151029799,2.33656758183441,4.34581543236837));
#13745=CARTESIAN_POINT('Ctrl Pts',(1.92378066150868,2.39697105038948,4.35079750920087));
#13746=CARTESIAN_POINT('Ctrl Pts',(1.84852667477487,2.45736901153983,4.35577913178275));
#13747=CARTESIAN_POINT('Ctrl Pts',(1.77041863459167,2.51422525714381,4.36076075436462));
#13748=CARTESIAN_POINT('Ctrl Pts',(1.68982900351582,2.56727096132775,4.36574237694649));
#13749=CARTESIAN_POINT('Ctrl Pts',(1.60922471982507,2.62032631015537,4.37072490527512));
#13750=CARTESIAN_POINT('Ctrl Pts',(1.52613831584143,2.66956950030223,4.37570743360376));
#13751=CARTESIAN_POINT('Ctrl Pts',(1.44097012189121,2.71477574724264,4.38068996193239));
#13752=CARTESIAN_POINT('Ctrl Pts',(1.35571012917975,2.76003071985489,4.38567786069225));
#13753=CARTESIAN_POINT('Ctrl Pts',(1.26836425520858,2.80123985628929,4.39066575945211));
#13754=CARTESIAN_POINT('Ctrl Pts',(1.17935605189272,2.83822507086102,4.39565365821197));
#13755=CARTESIAN_POINT('Ctrl Pts',(1.09029527020938,2.87523213310667,4.4006445033921));
#13756=CARTESIAN_POINT('Ctrl Pts',(0.999570616588127,2.9080101561935,4.40563534857222));
#13757=CARTESIAN_POINT('Ctrl Pts',(0.907622161561579,2.93643053073664,4.41062619375235));
#13758=CARTESIAN_POINT('Ctrl Pts',(0.815525115509369,2.96489683332286,4.41562510426434));
#13759=CARTESIAN_POINT('Ctrl Pts',(0.722200743773071,2.98899131624859,4.42062401477633));
#13760=CARTESIAN_POINT('Ctrl Pts',(0.628100631914152,3.00863621034332,4.42562292528832));
#13761=CARTESIAN_POINT('Ctrl Pts',(0.573469932414809,3.02004123723208,4.42852508951118));
#13762=CARTESIAN_POINT('Ctrl Pts',(0.518577911122112,3.02994750045903,4.43142725373405));
#13763=CARTESIAN_POINT('Ctrl Pts',(0.463513494024363,3.03834782256037,4.43432941795692));
#13764=CARTESIAN_POINT('Ctrl Pts',(0.368642164044329,3.05282086653356,4.4393296012723));
#13765=CARTESIAN_POINT('Ctrl Pts',(0.272925653470679,3.06287158941055,4.44432978458769));
#13766=CARTESIAN_POINT('Ctrl Pts',(0.176811857637761,3.06840998189595,4.44932996790308));
#13767=CARTESIAN_POINT('Ctrl Pts',(0.0808588515851836,3.07393910914628,
4.45432178635919));
#13768=CARTESIAN_POINT('Ctrl Pts',(-0.0154896827983501,3.07497089992487,
4.4593136048153));
#13769=CARTESIAN_POINT('Ctrl Pts',(-0.111777981769336,3.0714667396525,4.46430542327141));
#13770=CARTESIAN_POINT('Ctrl Pts',(-0.207974064497727,3.06796593534859,
4.46929246101432));
#13771=CARTESIAN_POINT('Ctrl Pts',(-0.304109590402857,3.05993782645941,
4.47427949875723));
#13772=CARTESIAN_POINT('Ctrl Pts',(-0.399726490619734,3.04739577060428,
4.47926653650014));
#13773=CARTESIAN_POINT('Ctrl Pts',(-0.495277924424917,3.0348623019695,4.48425015974765));
#13774=CARTESIAN_POINT('Ctrl Pts',(-0.590311004409107,3.01782108546238,
4.48923378299516));
#13775=CARTESIAN_POINT('Ctrl Pts',(-0.6843715547045,2.99633740174757,4.49421740624267));
#13776=CARTESIAN_POINT('Ctrl Pts',(-0.778393383831029,2.97486256205229,
4.4991989779211));
#13777=CARTESIAN_POINT('Ctrl Pts',(-0.871443052055211,2.94894898937803,
4.50418054959952));
#13778=CARTESIAN_POINT('Ctrl Pts',(-0.963076423723207,2.91871308149131,
4.50916212127795));
#13779=CARTESIAN_POINT('Ctrl Pts',(-1.05472610266889,2.8884717927555,4.51414457948789));
#13780=CARTESIAN_POINT('Ctrl Pts',(-1.14495856171286,2.85390676117679,4.51912703769784));
#13781=CARTESIAN_POINT('Ctrl Pts',(-1.23334530459458,2.81518411647169,4.52410949590779));
#13782=CARTESIAN_POINT('Ctrl Pts',(-1.32173930652233,2.77645829154464,4.52909236331817));
#13783=CARTESIAN_POINT('Ctrl Pts',(-1.40828689198012,2.7335743583164,4.53407523072855));
#13784=CARTESIAN_POINT('Ctrl Pts',(-1.4925814678542,2.68674576613013,4.53905809813893));
#13785=CARTESIAN_POINT('Ctrl Pts',(-1.57694638082662,2.63987809921979,4.54404512335462));
#13786=CARTESIAN_POINT('Ctrl Pts',(-1.65905415102559,2.58905942264468,4.54903214857031));
#13787=CARTESIAN_POINT('Ctrl Pts',(-1.73852499335928,2.5345479079049,4.554019173786));
#13788=CARTESIAN_POINT('Ctrl Pts',(-1.78403911597311,2.50332836004464,4.5568753166238));
#13789=CARTESIAN_POINT('Ctrl Pts',(-1.82868886306956,2.47089834754116,4.5597314594616));
#13790=CARTESIAN_POINT('Ctrl Pts',(-1.87240768645123,2.4373123939533,4.56258760229939));
#13791=CARTESIAN_POINT('Ctrl Pts',(-1.87240768645123,2.4373123939533,3.56268206416256));
#13792=CARTESIAN_POINT('Ctrl Pts',(-1.94893179304657,2.37852455627463,3.56766378537458));
#13793=CARTESIAN_POINT('Ctrl Pts',(-2.02268548271812,2.31612868029567,3.5726455065866));
#13794=CARTESIAN_POINT('Ctrl Pts',(-2.09332073888429,2.25042452309713,3.57762722779863));
#13795=CARTESIAN_POINT('Ctrl Pts',(-2.16397364935239,2.18470394405639,3.58261019412273));
#13796=CARTESIAN_POINT('Ctrl Pts',(-2.23150625682829,2.1156737403338,3.58759316044683));
#13797=CARTESIAN_POINT('Ctrl Pts',(-2.29560695052068,2.04367095656838,3.59257612677093));
#13798=CARTESIAN_POINT('Ctrl Pts',(-2.35977907302726,1.97158793851585,3.59756464572411));
#13799=CARTESIAN_POINT('Ctrl Pts',(-2.42051135734872,1.89652605799303,3.60255316467729));
#13800=CARTESIAN_POINT('Ctrl Pts',(-2.47753227791021,1.81885570123445,3.60754168363046));
#13801=CARTESIAN_POINT('Ctrl Pts',(-2.53459036481876,1.74113471878608,3.61253345411001));
#13802=CARTESIAN_POINT('Ctrl Pts',(-2.58793202987521,1.66080224067301,3.61752522458955));
#13803=CARTESIAN_POINT('Ctrl Pts',(-2.63733005394467,1.578256137818,3.6225169950691));
#13804=CARTESIAN_POINT('Ctrl Pts',(-2.68680438012126,1.49558253104556,3.62751647603126));
#13805=CARTESIAN_POINT('Ctrl Pts',(-2.73232270149939,1.41068886153324,3.63251595699342));
#13806=CARTESIAN_POINT('Ctrl Pts',(-2.7737046480908,1.32399576100512,3.63751543795558));
#13807=CARTESIAN_POINT('Ctrl Pts',(-2.78741574776541,1.29527169555264,3.63917191831574));
#13808=CARTESIAN_POINT('Ctrl Pts',(-2.80067315699813,1.26635023217343,3.64082839867589));
#13809=CARTESIAN_POINT('Ctrl Pts',(-2.81347151615409,1.23724705608444,3.64248487903604));
#13810=CARTESIAN_POINT('Ctrl Pts',(-2.85209890952511,1.14940924676559,3.64748438855936));
#13811=CARTESIAN_POINT('Ctrl Pts',(-2.88667670430598,1.05960647673055,3.65248389808267));
#13812=CARTESIAN_POINT('Ctrl Pts',(-2.91700165612439,0.968247689471843,
3.65748340760598));
#13813=CARTESIAN_POINT('Ctrl Pts',(-2.94728547234083,0.877012829820052,
3.6624761353268));
#13814=CARTESIAN_POINT('Ctrl Pts',(-2.97332777390544,0.784226560922798,
3.66746886304762));
#13815=CARTESIAN_POINT('Ctrl Pts',(-2.99497273372111,0.690319182890849,
3.67246159076844));
#13816=CARTESIAN_POINT('Ctrl Pts',(-3.01659485865146,0.596510874768349,
3.67744905128776));
#13817=CARTESIAN_POINT('Ctrl Pts',(-3.03382876598409,0.501584234202811,
3.68243651180707));
#13818=CARTESIAN_POINT('Ctrl Pts',(-3.04656828046346,0.405985175189797,
3.68742397232638));
#13819=CARTESIAN_POINT('Ctrl Pts',(-3.05929867952357,0.3104545195297,3.69240786420155));
#13820=CARTESIAN_POINT('Ctrl Pts',(-3.06754102085665,0.214252835756214,
3.69739175607672));
#13821=CARTESIAN_POINT('Ctrl Pts',(-3.07124030155397,0.117835733589989,
3.70237564795189));
#13822=CARTESIAN_POINT('Ctrl Pts',(-3.07493823506507,0.0214537441395582,
3.70735772481733));
#13823=CARTESIAN_POINT('Ctrl Pts',(-3.07409637838022,-0.0751430696406089,
3.71233980168276));
#13824=CARTESIAN_POINT('Ctrl Pts',(-3.06871171064564,-0.171495442931594,
3.7173218785482));
#13825=CARTESIAN_POINT('Ctrl Pts',(-3.06332753386848,-0.267839031109949,
3.72230350116321));
#13826=CARTESIAN_POINT('Ctrl Pts',(-3.0534013942232,-0.363937784842323,
3.72728512377822));
#13827=CARTESIAN_POINT('Ctrl Pts',(-3.03898233292869,-0.459334986853035,
3.73226674639323));
#13828=CARTESIAN_POINT('Ctrl Pts',(-3.02456064999435,-0.554749533758849,
3.73724927475516));
#13829=CARTESIAN_POINT('Ctrl Pts',(-3.0056444886985,-0.649461841596929,
3.74223180311709));
#13830=CARTESIAN_POINT('Ctrl Pts',(-2.98233427434873,-0.743023906778798,
3.74721433147902));
#13831=CARTESIAN_POINT('Ctrl Pts',(-2.95899893502323,-0.836686818078247,
3.75220223027223));
#13832=CARTESIAN_POINT('Ctrl Pts',(-2.93126019367038,-0.929196584942988,
3.75719012906543));
#13833=CARTESIAN_POINT('Ctrl Pts',(-2.89926873036408,-1.02011914947866,
3.76217802785864));
#13834=CARTESIAN_POINT('Ctrl Pts',(-2.86725836926098,-1.11109542322207,
3.76716887307217));
#13835=CARTESIAN_POINT('Ctrl Pts',(-2.83099044908122,-1.20048222119091,
3.77215971828571));
#13836=CARTESIAN_POINT('Ctrl Pts',(-2.79066348967254,-1.28786627310785,
3.77715056349924));
#13837=CARTESIAN_POINT('Ctrl Pts',(-2.75027136088101,-1.3753915398552,3.78214947404443));
#13838=CARTESIAN_POINT('Ctrl Pts',(-2.70580729733472,-1.46090720879924,
3.78714838458962));
#13839=CARTESIAN_POINT('Ctrl Pts',(-2.65751532832826,-1.54402543039301,
3.79214729513482));
#13840=CARTESIAN_POINT('Ctrl Pts',(-2.62947897768579,-1.59228048508068,
3.79504945902995));
#13841=CARTESIAN_POINT('Ctrl Pts',(-2.60015324796666,-1.63972802373726,
3.79795162292508));
#13842=CARTESIAN_POINT('Ctrl Pts',(-2.56959224495613,-1.68629711043497,
3.80085378682021));
#13843=CARTESIAN_POINT('Ctrl Pts',(-2.51694531321621,-1.76652090177191,
3.80585329630727));
#13844=CARTESIAN_POINT('Ctrl Pts',(-2.46044537736041,-1.84441774704064,
3.81085280579432));
#13845=CARTESIAN_POINT('Ctrl Pts',(-2.40032479931129,-1.91959451650894,
3.81585231528138));
#13846=CARTESIAN_POINT('Ctrl Pts',(-2.34028577444489,-1.9946693091664,3.82084504296553));
#13847=CARTESIAN_POINT('Ctrl Pts',(-2.2766361402387,-2.06703101930238,3.82583777064968));
#13848=CARTESIAN_POINT('Ctrl Pts',(-2.20965198879184,-2.13631466278455,
3.83083049833384));
#13849=CARTESIAN_POINT('Ctrl Pts',(-2.14273850393668,-2.20552521376887,
3.8358179588161));
#13850=CARTESIAN_POINT('Ctrl Pts',(-2.07249779856724,-2.27166383959328,
3.84080541929837));
#13851=CARTESIAN_POINT('Ctrl Pts',(-1.99924609461182,-2.33439870270256,
3.84579287978064));
#13852=CARTESIAN_POINT('Ctrl Pts',(-1.92604680396258,-2.39708867755108,
3.85077677161837));
#13853=CARTESIAN_POINT('Ctrl Pts',(-1.8498411300987,-2.4563794465704,3.8557606634561));
#13854=CARTESIAN_POINT('Ctrl Pts',(-1.77098128851237,-2.51197681632197,
3.86074455529383));
#13855=CARTESIAN_POINT('Ctrl Pts',(-1.69215016572705,-2.56755393888859,
3.8657266321216));
#13856=CARTESIAN_POINT('Ctrl Pts',(-1.61066715411105,-2.61944008196891,
3.87070870894937));
#13857=CARTESIAN_POINT('Ctrl Pts',(-1.52691583673615,-2.6673826642468,3.87569078577714));
#13858=CARTESIAN_POINT('Ctrl Pts',(-1.44317215555176,-2.71532087526578,
3.88067240835429));
#13859=CARTESIAN_POINT('Ctrl Pts',(-1.35716096085037,-2.75931602244041,
3.88565403093144));
#13860=CARTESIAN_POINT('Ctrl Pts',(-1.26929204412124,-2.79916058073318,
3.89063565350859));
#13861=CARTESIAN_POINT('Ctrl Pts',(-1.18140715127442,-2.83901238346888,
3.89561818183252));
#13862=CARTESIAN_POINT('Ctrl Pts',(-1.0916642653861,-2.87471191733804,3.90060071015645));
#13863=CARTESIAN_POINT('Ctrl Pts',(-1.00049384511949,-2.9060995020608,3.90558323848038));
#13864=CARTESIAN_POINT('Ctrl Pts',(-0.909225156574733,-2.9375209179746,
3.91057113723562));
#13865=CARTESIAN_POINT('Ctrl Pts',(-0.816526277577877,-2.9646209630174,
3.91555903599086));
#13866=CARTESIAN_POINT('Ctrl Pts',(-0.722843330537677,-2.98728970297445,
3.9205469347461));
#13867=CARTESIAN_POINT('Ctrl Pts',(-0.62910504369396,-3.00997183366755,
3.92553777992164));
#13868=CARTESIAN_POINT('Ctrl Pts',(-0.534381962176159,-3.02821736415241,
3.93052862509718));
#13869=CARTESIAN_POINT('Ctrl Pts',(-0.439128818339874,-3.04196780569805,
3.93551947027272));
#13870=CARTESIAN_POINT('Ctrl Pts',(-0.343721743015635,-3.05574046830478,
3.94051838078021));
#13871=CARTESIAN_POINT('Ctrl Pts',(-0.247783331579856,-3.06500349485755,
3.94551729128769));
#13872=CARTESIAN_POINT('Ctrl Pts',(-0.151771771365071,-3.06975040995464,
3.95051620179518));
#13873=CARTESIAN_POINT('Ctrl Pts',(-0.0960313617058057,-3.07250627593097,
3.95341836606492));
#13874=CARTESIAN_POINT('Ctrl Pts',(-0.0402662857999868,-3.07374096692759,
3.95632053033466));
#13875=CARTESIAN_POINT('Ctrl Pts',(0.015434497828892,-3.07346124528629,
3.9592226946044));
#13876=CARTESIAN_POINT('Ctrl Pts',(0.111389299267059,-3.07297937352795,
3.96422220409244));
#13877=CARTESIAN_POINT('Ctrl Pts',(0.207490050402046,-3.06799872222247,
3.96922171358048));
#13878=CARTESIAN_POINT('Ctrl Pts',(0.303280487235858,-3.0585001546611,3.97422122306852));
#13879=CARTESIAN_POINT('Ctrl Pts',(0.398940984948382,-3.04901447184651,
3.97921395075358));
#13880=CARTESIAN_POINT('Ctrl Pts',(0.494291571865417,-3.03502309575796,
3.98420667843864));
#13881=CARTESIAN_POINT('Ctrl Pts',(0.588875783338042,-3.01655889413716,
3.9891994061237));
#13882=CARTESIAN_POINT('Ctrl Pts',(0.683360210849682,-2.99811417178405,
3.9941868666068));
#13883=CARTESIAN_POINT('Ctrl Pts',(0.777079441640563,-2.9752060880826,3.99917432708989));
#13884=CARTESIAN_POINT('Ctrl Pts',(0.869582965406786,-2.94791921807134,
4.00416178757299));
#13885=CARTESIAN_POINT('Ctrl Pts',(0.96202030073714,-2.92065187245409,4.0091456794114));
#13886=CARTESIAN_POINT('Ctrl Pts',(1.05324323847752,-2.88901209286882,4.01412957124982));
#13887=CARTESIAN_POINT('Ctrl Pts',(1.14281324716655,-2.85313514087585,4.01911346308823));
#13888=CARTESIAN_POINT('Ctrl Pts',(1.23235063667565,-2.81727125438069,4.02409553991661));
#13889=CARTESIAN_POINT('Ctrl Pts',(1.32023588608128,-2.7771734244486,4.02907761674499));
#13890=CARTESIAN_POINT('Ctrl Pts',(1.4060482897216,-2.73302587930868,4.03405969357336));
#13891=CARTESIAN_POINT('Ctrl Pts',(1.49185286924658,-2.68888235940835,4.03904131615105));
#13892=CARTESIAN_POINT('Ctrl Pts',(1.57558458851359,-2.64069005939631,4.04402293872873));
#13893=CARTESIAN_POINT('Ctrl Pts',(1.65684626550578,-2.58867972188132,4.04900456130642));
#13894=CARTESIAN_POINT('Ctrl Pts',(1.73812271730209,-2.53665992797093,4.05398708963083));
#13895=CARTESIAN_POINT('Ctrl Pts',(1.81692786521932,-2.48082095456316,4.05896961795524));
#13896=CARTESIAN_POINT('Ctrl Pts',(1.89289340677911,-2.42143692888586,4.06395214627965));
#13897=CARTESIAN_POINT('Ctrl Pts',(1.96894082799592,-2.36198889598166,4.06894004503521));
#13898=CARTESIAN_POINT('Ctrl Pts',(2.04214218608905,-2.29898845324128,4.07392794379076));
#13899=CARTESIAN_POINT('Ctrl Pts',(2.11216237704504,-2.23274995084435,4.07891584254631));
#13900=CARTESIAN_POINT('Ctrl Pts',(2.18222392988828,-2.16647232045547,4.08390668772208));
#13901=CARTESIAN_POINT('Ctrl Pts',(2.24910026970181,-2.09695313798019,4.08889753289785));
#13902=CARTESIAN_POINT('Ctrl Pts',(2.31249475684799,-2.02454198512912,4.09388837807362));
#13903=CARTESIAN_POINT('Ctrl Pts',(2.37599169108638,-1.95201381402635,4.09888728858123));
#13904=CARTESIAN_POINT('Ctrl Pts',(2.43599526416855,-1.87658468390078,4.10388619908884));
#13905=CARTESIAN_POINT('Ctrl Pts',(2.49225058376852,-1.79863539320938,4.10888510959645));
#13906=CARTESIAN_POINT('Ctrl Pts',(2.52491013587622,-1.75338120321994,4.11178727386049));
#13907=CARTESIAN_POINT('Ctrl Pts',(2.55630716772764,-1.70727811728341,4.11468943812453));
#13908=CARTESIAN_POINT('Ctrl Pts',(2.58639891791606,-1.66040443489008,4.11759160238857));
#13909=CARTESIAN_POINT('Ctrl Pts',(2.6394023618579,-1.57784138749249,4.12270345862544));
#13910=CARTESIAN_POINT('Ctrl Pts',(2.68853322222333,-1.49260657023215,4.12781531486231));
#13911=CARTESIAN_POINT('Ctrl Pts',(2.73351906799659,-1.40508923378519,4.13292717109918));
#13912=CARTESIAN_POINT('Ctrl Pts',(2.77843555063002,-1.317706839277,4.1380311454258));
#13913=CARTESIAN_POINT('Ctrl Pts',(2.81921954333956,-1.22804928936143,4.14313511975242));
#13914=CARTESIAN_POINT('Ctrl Pts',(2.8556422189893,-1.1365341029313,4.14823909407904));
#13915=CARTESIAN_POINT('Ctrl Pts',(2.89200450440251,-1.04517065229916,4.15333460581439));
#13916=CARTESIAN_POINT('Ctrl Pts',(2.924019720944,-0.951956079566954,4.15843011754974));
#13917=CARTESIAN_POINT('Ctrl Pts',(2.95150578656232,-0.857330649101683,
4.1635256292851));
#13918=CARTESIAN_POINT('Ctrl Pts',(2.97896501468297,-0.762797611262038,
4.16861616574366));
#13919=CARTESIAN_POINT('Ctrl Pts',(3.00190377200421,-0.666856849596358,
4.17370670220221));
#13920=CARTESIAN_POINT('Ctrl Pts',(3.02018879138804,-0.569966590577061,
4.17879723866078));
#13921=CARTESIAN_POINT('Ctrl Pts',(3.03845833206675,-0.47315835147345,4.18388346585878));
#13922=CARTESIAN_POINT('Ctrl Pts',(3.05208189916622,-0.375402619071065,
4.1889696930568));
#13923=CARTESIAN_POINT('Ctrl Pts',(3.06097682471455,-0.277169855071588,
4.1940559202548));
#13924=CARTESIAN_POINT('Ctrl Pts',(3.06935225882419,-0.184674191356969,
4.19884509589569));
#13925=CARTESIAN_POINT('Ctrl Pts',(3.07353563445991,-0.0917559825750235,
4.20363427153658));
#13926=CARTESIAN_POINT('Ctrl Pts',(3.07349977118764,0.00118596353673709,
4.20842344717746));
#13927=CARTESIAN_POINT('Origin',(0.,0.,-2.20842344717744));
#13928=CARTESIAN_POINT('',(-1.87240768645123,2.4373123939533,2.56277205249695));
#13929=CARTESIAN_POINT('',(-1.87178979188679,2.43648733431069,2.64569210698702));
#13930=CARTESIAN_POINT('',(-1.87240768645123,2.4373123939533,-2.20842344717744));
#13931=CARTESIAN_POINT('',(3.07484942901424,0.00262471338485415,3.29157655282254));
#13932=CARTESIAN_POINT('Ctrl Pts',(-1.87178979188648,2.43648733431093,2.645692106987));
#13933=CARTESIAN_POINT('Ctrl Pts',(-2.0894887030698,2.27255165391444,2.65979557073464));
#13934=CARTESIAN_POINT('Ctrl Pts',(-3.01698552853461,1.36245345030385,2.72668867041033));
#13935=CARTESIAN_POINT('Ctrl Pts',(-3.41664634935444,-1.2250959035962,2.84637140601408));
#13936=CARTESIAN_POINT('Ctrl Pts',(-0.832597465415741,-3.53286195426117,
3.00474031379826));
#13937=CARTESIAN_POINT('Ctrl Pts',(2.2996550447433,-2.6791845859618,3.15314202940108));
#13938=CARTESIAN_POINT('Ctrl Pts',(3.06738194658167,-0.823160515664817,
3.24875410907584));
#13939=CARTESIAN_POINT('Ctrl Pts',(3.07484942901424,0.00262471338485415,
3.29157655282254));
#13940=CARTESIAN_POINT('Ctrl Pts',(3.07484942901424,0.00262471338485415,
3.29157655282254));
#13941=CARTESIAN_POINT('Ctrl Pts',(3.07658753235455,0.194831401241035,3.3015437450039));
#13942=CARTESIAN_POINT('Ctrl Pts',(2.97278968204648,1.40315899371448,3.36430057311331));
#13943=CARTESIAN_POINT('Ctrl Pts',(1.37275537107956,3.36004090547696,3.47984703715079));
#13944=CARTESIAN_POINT('Ctrl Pts',(-0.978619792012921,3.10112051414917,
3.58798106525116));
#13945=CARTESIAN_POINT('Ctrl Pts',(-1.83643233296303,2.47109227917888,3.64332545742347));
#13946=CARTESIAN_POINT('Ctrl Pts',(-1.87526655020737,2.4410026577968,3.64588021366773));
#13947=CARTESIAN_POINT('',(3.07349876324234,-0.00275723554104452,3.2084234471304));
#13948=CARTESIAN_POINT('Ctrl Pts',(3.07349876324315,-0.00275723463170688,
3.20842344717746));
#13949=CARTESIAN_POINT('Ctrl Pts',(3.0735842794169,0.0925679332825739,3.21335662415332));
#13950=CARTESIAN_POINT('Ctrl Pts',(3.06923075795488,0.187999949967112,3.21828980112919));
#13951=CARTESIAN_POINT('Ctrl Pts',(3.0604351335259,0.283088402235619,3.22322297810505));
#13952=CARTESIAN_POINT('Ctrl Pts',(3.05164431819358,0.378124863930588,3.22815345781648));
#13953=CARTESIAN_POINT('Ctrl Pts',(3.03841626328675,0.472817687881733,3.23308393752792));
#13954=CARTESIAN_POINT('Ctrl Pts',(3.02079995091825,0.566718542604943,3.23801441723935));
#13955=CARTESIAN_POINT('Ctrl Pts',(3.00318820947799,0.660595032747312,3.24294361763259));
#13956=CARTESIAN_POINT('Ctrl Pts',(2.98119055500706,0.75367952049474,3.24787281802583));
#13957=CARTESIAN_POINT('Ctrl Pts',(2.95490740437485,0.845532070101819,3.25280201841907));
#13958=CARTESIAN_POINT('Ctrl Pts',(2.92862352264444,0.937387174700717,3.25773135592409));
#13959=CARTESIAN_POINT('Ctrl Pts',(2.89805403289688,1.0280098414945,3.26266069342911));
#13960=CARTESIAN_POINT('Ctrl Pts',(2.86334938943221,1.11697471951615,3.26759003093413));
#13961=CARTESIAN_POINT('Ctrl Pts',(2.82861088193035,1.20602640753317,3.27252417837961));
#13962=CARTESIAN_POINT('Ctrl Pts',(2.78972932530905,1.29341665643582,3.27745832582509));
#13963=CARTESIAN_POINT('Ctrl Pts',(2.74690346004834,1.37873987074229,3.28239247327057));
#13964=CARTESIAN_POINT('Ctrl Pts',(2.70405710939133,1.46410389869835,3.28732898092442));
#13965=CARTESIAN_POINT('Ctrl Pts',(2.65726291414173,1.54739853173953,3.29226548857827));
#13966=CARTESIAN_POINT('Ctrl Pts',(2.60676462830897,1.62824458316224,3.29720199623213));
#13967=CARTESIAN_POINT('Ctrl Pts',(2.55617955234244,1.70922958266015,3.30214698813752));
#13968=CARTESIAN_POINT('Ctrl Pts',(2.50187792443551,1.7877572238769,3.30709198004292));
#13969=CARTESIAN_POINT('Ctrl Pts',(2.44414572994418,1.86347897782498,3.31203697194832));
#13970=CARTESIAN_POINT('Ctrl Pts',(2.39079116535085,1.93345901665323,3.31660700245478));
#13971=CARTESIAN_POINT('Ctrl Pts',(2.33450719914795,2.00104271688985,3.32117703296123));
#13972=CARTESIAN_POINT('Ctrl Pts',(2.27554719717419,2.06598335023124,3.32574706346769));
#13973=CARTESIAN_POINT('Ctrl Pts',(2.21104629554571,2.13702692659862,3.33074657293629));
#13974=CARTESIAN_POINT('Ctrl Pts',(2.14310189670449,2.20517177128013,3.33574608240488));
#13975=CARTESIAN_POINT('Ctrl Pts',(2.07200476478582,2.27006574898281,3.34074559187347));
#13976=CARTESIAN_POINT('Ctrl Pts',(2.00100407567367,2.33487169841813,3.34573831953932));
#13977=CARTESIAN_POINT('Ctrl Pts',(1.92685947450858,2.39643525162542,3.35073104720517));
#13978=CARTESIAN_POINT('Ctrl Pts',(1.84990053748908,2.45443888728108,3.35572377487102));
#13979=CARTESIAN_POINT('Ctrl Pts',(1.77302279020602,2.51238133056491,3.36071123533518));
#13980=CARTESIAN_POINT('Ctrl Pts',(1.69333695805015,2.56677105944817,3.36569869579933));
#13981=CARTESIAN_POINT('Ctrl Pts',(1.61120709387242,2.61732954567345,3.37068615626349));
#13982=CARTESIAN_POINT('Ctrl Pts',(1.52913599552668,2.66785185612348,3.37567004808345));
#13983=CARTESIAN_POINT('Ctrl Pts',(1.44462471435453,2.71454814412126,3.3806539399034));
#13984=CARTESIAN_POINT('Ctrl Pts',(1.35806699349407,2.75718267279881,3.38563783172335));
#13985=CARTESIAN_POINT('Ctrl Pts',(1.27154079480793,2.79980167503883,3.39061990853357));
#13986=CARTESIAN_POINT('Ctrl Pts',(1.18297003057217,2.83836166318928,3.39560198534378));
#13987=CARTESIAN_POINT('Ctrl Pts',(1.09277294659231,2.8726728907406,3.40058406215399));
#13988=CARTESIAN_POINT('Ctrl Pts',(1.00258408650373,2.90698098990026,3.40556568471384));
#13989=CARTESIAN_POINT('Ctrl Pts',(0.910769611829694,2.93704094276129,3.41054730727369));
#13990=CARTESIAN_POINT('Ctrl Pts',(0.817766638355192,2.96271159163244,3.41552892983354));
#13991=CARTESIAN_POINT('Ctrl Pts',(0.724746755296085,2.98838690788134,3.42051145814043));
#13992=CARTESIAN_POINT('Ctrl Pts',(0.630538367425689,3.00967121844639,3.42549398644732));
#13993=CARTESIAN_POINT('Ctrl Pts',(0.535591552539519,3.02647384572349,3.43047651475421));
#13994=CARTESIAN_POINT('Ctrl Pts',(0.440542398968198,3.04329458375853,3.43546441349292));
#13995=CARTESIAN_POINT('Ctrl Pts',(0.34475366237185,3.05562391804869,3.44045231223163));
#13996=CARTESIAN_POINT('Ctrl Pts',(0.248683144034158,3.06342274978059,3.44544021097033));
#13997=CARTESIAN_POINT('Ctrl Pts',(0.152555875516732,3.07122618838992,3.4504310561296));
#13998=CARTESIAN_POINT('Ctrl Pts',(0.0561469323296408,3.0744937807667,3.45542190128886));
#13999=CARTESIAN_POINT('Ctrl Pts',(-0.0400853931705421,3.07323858677688,
3.46041274644812));
#14000=CARTESIAN_POINT('Ctrl Pts',(-0.13647323255312,3.0719813643617,3.46541165693994));
#14001=CARTESIAN_POINT('Ctrl Pts',(-0.232683446457692,3.06618678761908,
3.47041056743175));
#14002=CARTESIAN_POINT('Ctrl Pts',(-0.328262431952541,3.0559198330075,3.47540947792356));
#14003=CARTESIAN_POINT('Ctrl Pts',(-0.383751709792868,3.04995925606618,
3.47831164236633));
#14004=CARTESIAN_POINT('Ctrl Pts',(-0.439028396098693,3.04249223061018,
3.4812138068091));
#14005=CARTESIAN_POINT('Ctrl Pts',(-0.494005671630389,3.0335392936959,3.48411597125187));
#14006=CARTESIAN_POINT('Ctrl Pts',(-0.588714580362088,3.01811614154995,
3.48911550650851));
#14007=CARTESIAN_POINT('Ctrl Pts',(-0.682866867034428,2.9982263454016,3.49411504176514));
#14008=CARTESIAN_POINT('Ctrl Pts',(-0.77600884927957,2.97392207628912,3.49911457702178));
#14009=CARTESIAN_POINT('Ctrl Pts',(-0.869028885514338,2.94964962750709,
3.50410756664386));
#14010=CARTESIAN_POINT('Ctrl Pts',(-0.96104082446848,2.92097429983823,3.50910055626593));
#14011=CARTESIAN_POINT('Ctrl Pts',(-1.0515988235673,2.88799968218001,3.514093545888));
#14012=CARTESIAN_POINT('Ctrl Pts',(-1.14204897447052,2.85506433496782,3.51908058921128));
#14013=CARTESIAN_POINT('Ctrl Pts',(-1.23104821975664,2.81784003257502,3.52406763253455));
#14014=CARTESIAN_POINT('Ctrl Pts',(-1.31816483149295,2.77648045680411,3.52905467585783));
#14015=CARTESIAN_POINT('Ctrl Pts',(-1.40522190785358,2.73514914611184,3.53403831104238));
#14016=CARTESIAN_POINT('Ctrl Pts',(-1.4903985123169,2.68968836607186,3.53902194622693));
#14017=CARTESIAN_POINT('Ctrl Pts',(-1.5732825990588,2.64030000445003,3.54400558141149));
#14018=CARTESIAN_POINT('Ctrl Pts',(-1.65613360688019,2.5909313536527,3.54898722763436));
#14019=CARTESIAN_POINT('Ctrl Pts',(-1.7366935394388,2.53763846205762,3.55396887385724));
#14020=CARTESIAN_POINT('Ctrl Pts',(-1.81457562117796,2.48066877374361,3.55895052008011));
#14021=CARTESIAN_POINT('Ctrl Pts',(-1.83402169771838,2.46644423204288,3.56019436810759));
#14022=CARTESIAN_POINT('Ctrl Pts',(-1.85330096510086,2.45199068140142,3.56143821613508));
#14023=CARTESIAN_POINT('Ctrl Pts',(-1.87240768645123,2.4373123939533,3.56268206416256));
#14024=CARTESIAN_POINT('Ctrl Pts',(-1.87240768645123,2.4373123939533,2.56277205249695));
#14025=CARTESIAN_POINT('Ctrl Pts',(-1.94874179693929,2.37867051629705,2.56775984818642));
#14026=CARTESIAN_POINT('Ctrl Pts',(-2.02240282813516,2.31637425317476,2.57274764387588));
#14027=CARTESIAN_POINT('Ctrl Pts',(-2.09302490950143,2.25069966415035,2.57773543956535));
#14028=CARTESIAN_POINT('Ctrl Pts',(-2.16359434507864,2.18507403276772,2.58271951706308));
#14029=CARTESIAN_POINT('Ctrl Pts',(-2.23112901408335,2.11607538019443,2.58770359456081));
#14030=CARTESIAN_POINT('Ctrl Pts',(-2.29529630712004,2.04401984151845,2.59268767205853));
#14031=CARTESIAN_POINT('Ctrl Pts',(-2.35943893603888,1.97199199898195,2.59766983381587));
#14032=CARTESIAN_POINT('Ctrl Pts',(-2.42021646901576,1.89690993229495,2.60265199557321));
#14033=CARTESIAN_POINT('Ctrl Pts',(-2.47733402183739,1.81912572249611,2.60763415733055));
#14034=CARTESIAN_POINT('Ctrl Pts',(-2.53444521331875,1.74135017574043,2.61261576421072));
#14035=CARTESIAN_POINT('Ctrl Pts',(-2.5878969753007,1.66087343803078,2.61759737109089));
#14036=CARTESIAN_POINT('Ctrl Pts',(-2.63743616477765,1.57807880878078,2.62257897797106));
#14037=CARTESIAN_POINT('Ctrl Pts',(-2.686983360921,1.49527079802449,2.62756138999287));
#14038=CARTESIAN_POINT('Ctrl Pts',(-2.73261650341584,1.41014452848584,2.63254380201468));
#14039=CARTESIAN_POINT('Ctrl Pts',(-2.77412759930302,1.32310933515915,2.63752621403649));
#14040=CARTESIAN_POINT('Ctrl Pts',(-2.81568297515355,1.23598130122951,2.64251394080649));
#14041=CARTESIAN_POINT('Ctrl Pts',(-2.85310733598039,1.14694067481163,2.6475016675765));
#14042=CARTESIAN_POINT('Ctrl Pts',(-2.88624030085153,1.05641808756783,2.6524893943465));
#14043=CARTESIAN_POINT('Ctrl Pts',(-2.91939223780762,0.965843666682782,
2.65747997711132));
#14044=CARTESIAN_POINT('Ctrl Pts',(-2.94824775430845,0.87378601396475,2.66247055987614));
#14045=CARTESIAN_POINT('Ctrl Pts',(-2.97269658770118,0.780690237847104,
2.66746114264096));
#14046=CARTESIAN_POINT('Ctrl Pts',(-2.99718546494448,0.687441983560535,
2.67245989929888));
#14047=CARTESIAN_POINT('Ctrl Pts',(-3.01725315369669,0.593152639522881,
2.6774586559568));
#14048=CARTESIAN_POINT('Ctrl Pts',(-3.03284066354309,0.498276790107153,
2.68245741261471));
#14049=CARTESIAN_POINT('Ctrl Pts',(-3.04304160879334,0.436187119916245,
2.68572875252014));
#14050=CARTESIAN_POINT('Ctrl Pts',(-3.051324850439,0.373846396131847,2.68900009242556));
#14051=CARTESIAN_POINT('Ctrl Pts',(-3.05768593609462,0.311382347298604,
2.69227143233099));
#14052=CARTESIAN_POINT('Ctrl Pts',(-3.06740743167987,0.215920030353821,
2.69727094313311));
#14053=CARTESIAN_POINT('Ctrl Pts',(-3.07267115330314,0.11983434104367,2.70227045393522));
#14054=CARTESIAN_POINT('Ctrl Pts',(-3.07340956897462,0.02357692378719,2.70726996473734));
#14055=CARTESIAN_POINT('Ctrl Pts',(-3.07414698299245,-0.0725499212228172,
2.71226269375188));
#14056=CARTESIAN_POINT('Ctrl Pts',(-3.07037128764889,-0.168847596017427,
2.71725542276642));
#14057=CARTESIAN_POINT('Ctrl Pts',(-3.06206663938885,-0.264858728272064,
2.72224815178096));
#14058=CARTESIAN_POINT('Ctrl Pts',(-3.05377075229881,-0.360768571486514,
2.72723561360701));
#14059=CARTESIAN_POINT('Ctrl Pts',(-3.04095544813071,-0.456392038100134,
2.73222307543307));
#14060=CARTESIAN_POINT('Ctrl Pts',(-3.02365693060796,-0.551272179586862,
2.73721053725913));
#14061=CARTESIAN_POINT('Ctrl Pts',(-3.0063707905256,-0.646084432406635,
2.74219443045503));
#14062=CARTESIAN_POINT('Ctrl Pts',(-2.98460789261121,-0.740153986815278,
2.74717832365092));
#14063=CARTESIAN_POINT('Ctrl Pts',(-2.95845611331786,-0.833030416954972,
2.75216221684681));
#14064=CARTESIAN_POINT('Ctrl Pts',(-2.93231385780814,-0.925873023964895,
2.75714429504114));
#14065=CARTESIAN_POINT('Ctrl Pts',(-2.90178601544909,-1.017522947919,2.76212637323547));
#14066=CARTESIAN_POINT('Ctrl Pts',(-2.86701104688474,-1.10754228228129,
2.76710845142979));
#14067=CARTESIAN_POINT('Ctrl Pts',(-2.83223924894844,-1.19755340907826,
2.77209007538023));
#14068=CARTESIAN_POINT('Ctrl Pts',(-2.79322125305204,-1.28593383246197,
2.77707169933068));
#14069=CARTESIAN_POINT('Ctrl Pts',(-2.75014427135568,-1.37226409146692,
2.78205332328112));
#14070=CARTESIAN_POINT('Ctrl Pts',(-2.70705945746326,-1.45861004691781,
2.7870358529834));
#14071=CARTESIAN_POINT('Ctrl Pts',(-2.65991438812218,-1.54290470493198,
2.79201838268568));
#14072=CARTESIAN_POINT('Ctrl Pts',(-2.60894248435051,-1.62475270836856,
2.79700091238796));
#14073=CARTESIAN_POINT('Ctrl Pts',(-2.55791564039992,-1.7066889318562,2.80198881252088));
#14074=CARTESIAN_POINT('Ctrl Pts',(-2.50305395974698,-1.78617286274464,
2.80697671265379));
#14075=CARTESIAN_POINT('Ctrl Pts',(-2.4446343876474,-1.86283787827385,2.8119646127867));
#14076=CARTESIAN_POINT('Ctrl Pts',(-2.38618030629432,-1.93954818089368,
2.81695545934158));
#14077=CARTESIAN_POINT('Ctrl Pts',(-2.32416443074657,-2.01343591645363,
2.82194630589645));
#14078=CARTESIAN_POINT('Ctrl Pts',(-2.25890282716458,-2.08416896326278,
2.82693715245132));
#14079=CARTESIAN_POINT('Ctrl Pts',(-2.19353575935452,-2.15501631627606,
2.83193606432716));
#14080=CARTESIAN_POINT('Ctrl Pts',(-2.12491280238239,-2.22269849282685,
2.83693497620299));
#14081=CARTESIAN_POINT('Ctrl Pts',(-2.0533855002772,-2.28692156342349,2.84193388807883));
#14082=CARTESIAN_POINT('Ctrl Pts',(-2.01185986159587,-2.32420668317651,
2.8448360387576));
#14083=CARTESIAN_POINT('Ctrl Pts',(-1.96935593236938,-2.3603266909794,2.84773818943638));
#14084=CARTESIAN_POINT('Ctrl Pts',(-1.9259470215076,-2.39523074469789,2.85064034011516));
#14085=CARTESIAN_POINT('Ctrl Pts',(-1.85116687262225,-2.4553596509974,2.85563984956007));
#14086=CARTESIAN_POINT('Ctrl Pts',(-1.77343680286138,-2.51208880948381,
2.86063935900498));
#14087=CARTESIAN_POINT('Ctrl Pts',(-1.69309887987733,-2.56511567633082,
2.86563886844989));
#14088=CARTESIAN_POINT('Ctrl Pts',(-1.61286993473259,-2.6180706125981,2.87063159609466));
#14089=CARTESIAN_POINT('Ctrl Pts',(-1.53004053020147,-2.6673329986404,2.87562432373944));
#14090=CARTESIAN_POINT('Ctrl Pts',(-1.44498568032854,-2.71264052790735,
2.88061705138421));
#14091=CARTESIAN_POINT('Ctrl Pts',(-1.36002056113136,-2.75790025889797,
2.88560451182993));
#14092=CARTESIAN_POINT('Ctrl Pts',(-1.27283504921582,-2.79921322206013,
2.89059197227564));
#14093=CARTESIAN_POINT('Ctrl Pts',(-1.18383214038874,-2.83636099842432,
2.89557943272135));
#14094=CARTESIAN_POINT('Ctrl Pts',(-1.09489291514546,-2.87348219471871,
2.9005633245269));
#14095=CARTESIAN_POINT('Ctrl Pts',(-1.00413928203352,-2.90644396028856,
2.90554721633245));
#14096=CARTESIAN_POINT('Ctrl Pts',(-0.911996899011164,-2.93507477011984,
2.910531108138));
#14097=CARTESIAN_POINT('Ctrl Pts',(-0.819888071912237,-2.96369515333493,
2.91551318493631));
#14098=CARTESIAN_POINT('Ctrl Pts',(-0.726391918532192,-2.98798758446537,
2.92049526173463));
#14099=CARTESIAN_POINT('Ctrl Pts',(-0.631951136375388,-3.00782978428532,
2.92547733853294));
#14100=CARTESIAN_POINT('Ctrl Pts',(-0.537518964989268,-3.02767017496488,
2.93045896108342));
#14101=CARTESIAN_POINT('Ctrl Pts',(-0.442142765685321,-3.04306105097527,
2.9354405836339));
#14102=CARTESIAN_POINT('Ctrl Pts',(-0.346276306816527,-3.05393106820333,
2.94042220618437));
#14103=CARTESIAN_POINT('Ctrl Pts',(-0.250392417681477,-3.06480306179826,
2.94540473448446));
#14104=CARTESIAN_POINT('Ctrl Pts',(-0.154018528120127,-3.07115251474852,
2.95038726278454));
#14105=CARTESIAN_POINT('Ctrl Pts',(-0.0576133468764672,-3.07295996593865,
2.95536979108463));
#14106=CARTESIAN_POINT('Ctrl Pts',(0.0388957450335715,-3.07476936529646,
2.96035768982051));
#14107=CARTESIAN_POINT('Ctrl Pts',(0.13543575634752,-3.07202698101351,2.96534558855638));
#14108=CARTESIAN_POINT('Ctrl Pts',(0.231548383653232,-3.06476550424785,
2.97033348729226));
#14109=CARTESIAN_POINT('Ctrl Pts',(0.327717786056384,-3.05749973802447,
2.97532433245094));
#14110=CARTESIAN_POINT('Ctrl Pts',(0.423458866290721,-3.04570961754902,
2.98031517760962));
#14111=CARTESIAN_POINT('Ctrl Pts',(0.518320960736258,-3.02947943245394,
2.9853060227683));
#14112=CARTESIAN_POINT('Ctrl Pts',(0.61333635480394,-3.01322301895586,2.99030493326311));
#14113=CARTESIAN_POINT('Ctrl Pts',(0.707469498310246,-2.99251230768777,
2.99530384375791));
#14114=CARTESIAN_POINT('Ctrl Pts',(0.800282446976151,-2.9674821406475,3.00030275425271));
#14115=CARTESIAN_POINT('Ctrl Pts',(0.854165878090701,-2.95295064153141,
3.00320491880159));
#14116=CARTESIAN_POINT('Ctrl Pts',(0.907604650046743,-2.9369641988445,3.00610708335046));
#14117=CARTESIAN_POINT('Ctrl Pts',(0.960516202499753,-2.91955662297128,
3.00900924789933));
#14118=CARTESIAN_POINT('Ctrl Pts',(1.05166602766874,-2.88956889016248,3.0140087570609));
#14119=CARTESIAN_POINT('Ctrl Pts',(1.14157026009048,-2.85525578898929,3.01900826622246));
#14120=CARTESIAN_POINT('Ctrl Pts',(1.22978888909977,-2.8167395226124,3.02400777538403));
#14121=CARTESIAN_POINT('Ctrl Pts',(1.3178878499894,-2.77827550335413,3.02900050273695));
#14122=CARTESIAN_POINT('Ctrl Pts',(1.40430535290841,-2.73561982452741,3.03399323008987));
#14123=CARTESIAN_POINT('Ctrl Pts',(1.48861720018372,-2.68894423172315,3.03898595744279));
#14124=CARTESIAN_POINT('Ctrl Pts',(1.57284010049035,-2.64231788054536,3.04397341758858));
#14125=CARTESIAN_POINT('Ctrl Pts',(1.65496137919667,-2.59168025754403,3.04896087773436));
#14126=CARTESIAN_POINT('Ctrl Pts',(1.73457841647093,-2.53725047386205,3.05394833788015));
#14127=CARTESIAN_POINT('Ctrl Pts',(1.81413848578713,-2.48285963603564,3.05893222937493));
#14128=CARTESIAN_POINT('Ctrl Pts',(1.89119751444243,-2.4246822786342,3.0639161208697));
#14129=CARTESIAN_POINT('Ctrl Pts',(1.9653798784427,-2.36298205312959,3.06890001236448));
#14130=CARTESIAN_POINT('Ctrl Pts',(2.03953522700394,-2.30130429736834,3.07388208884543));
#14131=CARTESIAN_POINT('Ctrl Pts',(2.11081565526192,-2.23610650298653,3.07886416532637));
#14132=CARTESIAN_POINT('Ctrl Pts',(2.17887756899577,-2.16769342604693,3.08384624180731));
#14133=CARTESIAN_POINT('Ctrl Pts',(2.24693327700375,-2.09928658685144,3.0888278640342));
#14134=CARTESIAN_POINT('Ctrl Pts',(2.3117707444701,-2.02766535927851,3.09380948626107));
#14135=CARTESIAN_POINT('Ctrl Pts',(2.37308307360751,-1.95317151723998,3.09879110848796));
#14136=CARTESIAN_POINT('Ctrl Pts',(2.43440655037017,-1.87866413095274,3.10377363645857));
#14137=CARTESIAN_POINT('Ctrl Pts',(2.49220333699067,-1.80128343187748,3.10875616442918));
#14138=CARTESIAN_POINT('Ctrl Pts',(2.54620736493229,-1.72140358567205,3.11373869239979));
#14139=CARTESIAN_POINT('Ctrl Pts',(2.60026960123481,-1.6414376407978,3.11872659079919));
#14140=CARTESIAN_POINT('Ctrl Pts',(2.65053067121611,-1.55896753530423,3.12371448919859));
#14141=CARTESIAN_POINT('Ctrl Pts',(2.6967684719449,-1.47439548925109,3.12870238759799));
#14142=CARTESIAN_POINT('Ctrl Pts',(2.74303358596144,-1.38977348535843,3.13369323241573));
#14143=CARTESIAN_POINT('Ctrl Pts',(2.78527050641838,-1.30304746305312,3.13868407723347));
#14144=CARTESIAN_POINT('Ctrl Pts',(2.82330457028139,-1.21464132707076,3.14367492205122));
#14145=CARTESIAN_POINT('Ctrl Pts',(2.86140009816075,-1.12609232451997,3.14867383220135));
#14146=CARTESIAN_POINT('Ctrl Pts',(2.89527905328596,-1.0358581974992,3.15367274235149));
#14147=CARTESIAN_POINT('Ctrl Pts',(2.92481610062052,-0.9443797051774,3.15867165250163));
#14148=CARTESIAN_POINT('Ctrl Pts',(2.94196413148312,-0.891270943430509,
3.16157382022893));
#14149=CARTESIAN_POINT('Ctrl Pts',(2.9576496683022,-0.837743011043862,3.16447598795622));
#14150=CARTESIAN_POINT('Ctrl Pts',(2.97185612080094,-0.783883567411629,
3.16737815568352));
#14151=CARTESIAN_POINT('Ctrl Pts',(3.0033493354305,-0.664486623080219,3.1738117527504));
#14152=CARTESIAN_POINT('Ctrl Pts',(3.0276611199019,-0.543122418651518,3.18024534981728));
#14153=CARTESIAN_POINT('Ctrl Pts',(3.04459242610206,-0.420546321969373,
3.18667894688416));
#14154=CARTESIAN_POINT('Ctrl Pts',(3.06118864443189,-0.300396131635276,
3.19298521648355));
#14155=CARTESIAN_POINT('Ctrl Pts',(3.0706936399446,-0.179081323696639,3.19929148608295));
#14156=CARTESIAN_POINT('Ctrl Pts',(3.0729651698961,-0.0573351079655099,
3.20559775568234));
#14157=CARTESIAN_POINT('Ctrl Pts',(3.07330444298811,-0.0391512336901752,
3.2065396528317));
#14158=CARTESIAN_POINT('Ctrl Pts',(3.07348243553562,-0.020957779401148,
3.20748154998105));
#14159=CARTESIAN_POINT('Ctrl Pts',(3.07349876324234,-0.00275723554103428,
3.2084234471304));
#14160=CARTESIAN_POINT('Origin',(0.,0.,-2.20842344717744));
#14161=CARTESIAN_POINT('',(-1.87240768645123,2.4373123939533,1.56259812102449));
#14162=CARTESIAN_POINT('',(-1.86967516139564,2.4337884984361,1.64589879171829));
#14163=CARTESIAN_POINT('',(-1.87240768645123,2.4373123939533,-2.20842344717744));
#14164=CARTESIAN_POINT('',(3.06851769484666,-5.29070161844891E-5,2.29157655282254));
#14165=CARTESIAN_POINT('Ctrl Pts',(-1.86967516139566,2.43378849843609,1.64589879171829));
#14166=CARTESIAN_POINT('Ctrl Pts',(-2.33881678074012,2.07024255782115,1.67652887832048));
#14167=CARTESIAN_POINT('Ctrl Pts',(-3.347303037218,0.724834725607579,1.75994860085072));
#14168=CARTESIAN_POINT('Ctrl Pts',(-2.87382423513241,-2.21708609137177,
1.89615795930903));
#14169=CARTESIAN_POINT('Ctrl Pts',(0.295015670113215,-3.61763651773389,
2.0545268670932));
#14170=CARTESIAN_POINT('Ctrl Pts',(2.70865137306433,-2.04009181137399,2.18633306493104));
#14171=CARTESIAN_POINT('Ctrl Pts',(3.06859605637346,-0.508461450263827,
2.26534962684082));
#14172=CARTESIAN_POINT('Ctrl Pts',(3.06851769484666,-5.29070161844891E-5,
2.29157655282254));
#14173=CARTESIAN_POINT('Ctrl Pts',(3.06851769484666,-5.29070161844891E-5,
2.29157655282254));
#14174=CARTESIAN_POINT('Ctrl Pts',(3.06843833005534,0.514864803047814,2.31813926276888));
#14175=CARTESIAN_POINT('Ctrl Pts',(2.70185886612363,2.05321498844667,2.39749160864328));
#14176=CARTESIAN_POINT('Ctrl Pts',(0.531438462838955,3.45227005220736,2.51553012669809));
#14177=CARTESIAN_POINT('Ctrl Pts',(-1.27463594994892,2.88616721946652,2.60700593480658));
#14178=CARTESIAN_POINT('Ctrl Pts',(-1.87178979188648,2.43648733431093,2.645692106987));
#14179=CARTESIAN_POINT('',(3.0734998353151,0.00100614018965784,2.20842344715011));
#14180=CARTESIAN_POINT('Ctrl Pts',(3.07349983531492,0.00100614071472882,
2.20842344717745));
#14181=CARTESIAN_POINT('Ctrl Pts',(3.07348151913187,0.0569573459386727,
2.21133720111112));
#14182=CARTESIAN_POINT('Ctrl Pts',(3.0719354652809,0.112881503038161,2.21425095504479));
#14183=CARTESIAN_POINT('Ctrl Pts',(3.06886549665176,0.168721111483932,2.21716470897846));
#14184=CARTESIAN_POINT('Ctrl Pts',(3.06359794048394,0.264532603198921,2.22216422668006));
#14185=CARTESIAN_POINT('Ctrl Pts',(3.05382990902008,0.360265456024861,2.22716374438167));
#14186=CARTESIAN_POINT('Ctrl Pts',(3.03956504934842,0.455463018015246,2.23216326208327));
#14187=CARTESIAN_POINT('Ctrl Pts',(3.02531953958613,0.550531447000532,2.23715599806976));
#14188=CARTESIAN_POINT('Ctrl Pts',(3.00658938911884,0.64506559784126,2.24214873405625));
#14189=CARTESIAN_POINT('Ctrl Pts',(2.98343019475376,0.738611212365163,2.24714147004275));
#14190=CARTESIAN_POINT('Ctrl Pts',(2.96029543236287,0.832058140207496,2.25212893890315));
#14191=CARTESIAN_POINT('Ctrl Pts',(2.93274101956111,0.924518181053002,2.25711640776356));
#14192=CARTESIAN_POINT('Ctrl Pts',(2.90087389905939,1.01554560299179,2.26210387662396));
#14193=CARTESIAN_POINT('Ctrl Pts',(2.86902957968994,1.10650789421733,2.26708777691791));
#14194=CARTESIAN_POINT('Ctrl Pts',(2.83287883161229,1.19603919116548,2.27207167721187));
#14195=CARTESIAN_POINT('Ctrl Pts',(2.7925786234219,1.28370825424121,2.27705557750582));
#14196=CARTESIAN_POINT('Ctrl Pts',(2.75229309117913,1.3713453912641,2.28203766283497));
#14197=CARTESIAN_POINT('Ctrl Pts',(2.70786128434982,1.45712124341626,2.28701974816412));
#14198=CARTESIAN_POINT('Ctrl Pts',(2.65948818804544,1.54062481728901,2.29200183349326));
#14199=CARTESIAN_POINT('Ctrl Pts',(2.61111950190808,1.62412077815503,2.29698346460653));
#14200=CARTESIAN_POINT('Ctrl Pts',(2.55881046089606,1.70534449288149,2.3019650957198));
#14201=CARTESIAN_POINT('Ctrl Pts',(2.50281133318863,1.78391078265214,2.30694672683307));
#14202=CARTESIAN_POINT('Ctrl Pts',(2.44680202359668,1.86249135751833,2.31192926371746));
#14203=CARTESIAN_POINT('Ctrl Pts',(2.38710154962829,1.93841319040467,2.31691180060185));
#14204=CARTESIAN_POINT('Ctrl Pts',(2.3240020695165,2.01132211017605,2.32189433748624));
#14205=CARTESIAN_POINT('Ctrl Pts',(2.26083457777066,2.08430961466415,2.3268822447869));
#14206=CARTESIAN_POINT('Ctrl Pts',(2.19426105355551,2.15427739031301,2.33187015208757));
#14207=CARTESIAN_POINT('Ctrl Pts',(2.12461217200144,2.2209064294975,2.33685805938824));
#14208=CARTESIAN_POINT('Ctrl Pts',(2.05492214790873,2.28757482735879,2.34184891311338));
#14209=CARTESIAN_POINT('Ctrl Pts',(1.98215348019765,2.35090027368193,2.34683976683852));
#14210=CARTESIAN_POINT('Ctrl Pts',(1.90667011304086,2.41060393470946,2.35183062056366));
#14211=CARTESIAN_POINT('Ctrl Pts',(1.83106476424255,2.47040407726467,2.35682953954281));
#14212=CARTESIAN_POINT('Ctrl Pts',(1.75273631267024,2.52657049209211,2.36182845852196));
#14213=CARTESIAN_POINT('Ctrl Pts',(1.67207779799985,2.57886759788788,2.36682737750111));
#14214=CARTESIAN_POINT('Ctrl Pts',(1.62525218562726,2.60922823636737,2.36972945725495));
#14215=CARTESIAN_POINT('Ctrl Pts',(1.57764175605759,2.6382856582793,2.37263153700879));
#14216=CARTESIAN_POINT('Ctrl Pts',(1.52932683703008,2.66600106442957,2.37553361676263));
#14217=CARTESIAN_POINT('Ctrl Pts',(1.44609310741097,2.71374732310551,2.38053312677789));
#14218=CARTESIAN_POINT('Ctrl Pts',(1.36047505246342,2.75767581755783,2.38553263679314));
#14219=CARTESIAN_POINT('Ctrl Pts',(1.27285769233677,2.79754098183728,2.39053214680839));
#14220=CARTESIAN_POINT('Ctrl Pts',(1.18535918404278,2.83735206952933,2.39552487505201));
#14221=CARTESIAN_POINT('Ctrl Pts',(1.09586715668542,2.87311060126025,2.40051760329563));
#14222=CARTESIAN_POINT('Ctrl Pts',(1.00479290675893,2.90461588932632,2.40551033153924));
#14223=CARTESIAN_POINT('Ctrl Pts',(0.913814737306463,2.93608794030273,2.41049779261133));
#14224=CARTESIAN_POINT('Ctrl Pts',(0.821258076180029,2.96331552483282,2.41548525368342));
#14225=CARTESIAN_POINT('Ctrl Pts',(0.727555023575959,2.9861456658491,2.42047271475551));
#14226=CARTESIAN_POINT('Ctrl Pts',(0.633919016878905,3.008959471565,2.42545660722612));
#14227=CARTESIAN_POINT('Ctrl Pts',(0.539138674605391,3.02738198511897,2.43044049969674));
#14228=CARTESIAN_POINT('Ctrl Pts',(0.443661177673654,3.04131008110407,2.43542439216736));
#14229=CARTESIAN_POINT('Ctrl Pts',(0.348218450770178,3.05523310489617,2.44040646965447));
#14230=CARTESIAN_POINT('Ctrl Pts',(0.252079507566787,3.06466489982751,2.44538854714158));
#14231=CARTESIAN_POINT('Ctrl Pts',(0.155700689380518,3.06955363942812,2.4503706246287));
#14232=CARTESIAN_POINT('Ctrl Pts',(0.0593306582226456,3.07444193331365,
2.45535224789094));
#14233=CARTESIAN_POINT('Ctrl Pts',(-0.0372787660290401,3.07478797331731,
2.46033387115318));
#14234=CARTESIAN_POINT('Ctrl Pts',(-0.133668240644852,3.07059197084909,
2.46531549441542));
#14235=CARTESIAN_POINT('Ctrl Pts',(-0.230075241047957,3.06639520545269,
2.47029802344947));
#14236=CARTESIAN_POINT('Ctrl Pts',(-0.326261773850551,3.05765477657871,
2.47528055248353));
#14237=CARTESIAN_POINT('Ctrl Pts',(-0.42177169818593,3.04442291487391,2.48026308151759));
#14238=CARTESIAN_POINT('Ctrl Pts',(-0.517384568786063,3.03117679108328,
2.48525098101714));
#14239=CARTESIAN_POINT('Ctrl Pts',(-0.612318939430988,3.01342962992525,
2.4902388805167));
#14240=CARTESIAN_POINT('Ctrl Pts',(-0.706127193526199,2.99128511455575,
2.49522678001625));
#14241=CARTESIAN_POINT('Ctrl Pts',(-0.799990861821142,2.9691275180282,2.50021762595652));
#14242=CARTESIAN_POINT('Ctrl Pts',(-0.892726667212065,2.94256751585795,
2.50520847189678));
#14243=CARTESIAN_POINT('Ctrl Pts',(-0.983902577260418,2.91175856974103,
2.51019931783705));
#14244=CARTESIAN_POINT('Ctrl Pts',(-1.07522583031713,2.88089983544209,2.51519822913422));
#14245=CARTESIAN_POINT('Ctrl Pts',(-1.16498374596833,2.84577860631539,2.52019714043138));
#14246=CARTESIAN_POINT('Ctrl Pts',(-1.25276473051643,2.80659629800477,2.52519605172855));
#14247=CARTESIAN_POINT('Ctrl Pts',(-1.3037266773949,2.78384869811191,2.52809820933464));
#14248=CARTESIAN_POINT('Ctrl Pts',(-1.35402275645602,2.75973318744216,2.53100036694073));
#14249=CARTESIAN_POINT('Ctrl Pts',(-1.40357668246183,2.73429602392452,2.53390252454682));
#14250=CARTESIAN_POINT('Ctrl Pts',(-1.48892148252625,2.6904865862149,2.53890079775363));
#14251=CARTESIAN_POINT('Ctrl Pts',(-1.57236306688953,2.64260062643993,2.54389907096044));
#14252=CARTESIAN_POINT('Ctrl Pts',(-1.65348613732799,2.59082725083402,2.54889734416725));
#14253=CARTESIAN_POINT('Ctrl Pts',(-1.72854932379068,2.54292134039566,2.55352224694382));
#14254=CARTESIAN_POINT('Ctrl Pts',(-1.8016273535101,2.49168771316857,2.55814714972038));
#14255=CARTESIAN_POINT('Ctrl Pts',(-1.87240768645123,2.4373123939533,2.56277205249695));
#14256=CARTESIAN_POINT('Ctrl Pts',(-1.87240768645123,2.4373123939533,1.56259812102449));
#14257=CARTESIAN_POINT('Ctrl Pts',(-1.94882482793984,2.37860672969176,1.56759754314901));
#14258=CARTESIAN_POINT('Ctrl Pts',(-2.02238011400756,2.31637935109213,1.57259696527352));
#14259=CARTESIAN_POINT('Ctrl Pts',(-2.09275054956073,2.25095477238288,1.57759638739804));
#14260=CARTESIAN_POINT('Ctrl Pts',(-2.12133687210871,2.22437758702305,1.57962728421261));
#14261=CARTESIAN_POINT('Ctrl Pts',(-2.14939807886449,2.19727319978244,1.58165818102718));
#14262=CARTESIAN_POINT('Ctrl Pts',(-2.17691441706924,2.16966492130838,1.58368907784175));
#14263=CARTESIAN_POINT('Ctrl Pts',(-2.24465021132717,2.1017028016172,1.58868844977007));
#14264=CARTESIAN_POINT('Ctrl Pts',(-2.30931938227318,2.0304461905262,1.59368782169838));
#14265=CARTESIAN_POINT('Ctrl Pts',(-2.37058473659246,1.95620302030103,1.5986871936267));
#14266=CARTESIAN_POINT('Ctrl Pts',(-2.43176695745554,1.88206059365938,1.60367978170349));
#14267=CARTESIAN_POINT('Ctrl Pts',(-2.48955426417674,1.80493999780551,1.60867236978029));
#14268=CARTESIAN_POINT('Ctrl Pts',(-2.54364596787284,1.72518620447888,1.61366495785708));
#14269=CARTESIAN_POINT('Ctrl Pts',(-2.59768058460601,1.64551658121035,1.61865227688759));
#14270=CARTESIAN_POINT('Ctrl Pts',(-2.6480271066488,1.56321964633603,1.62363959591809));
#14271=CARTESIAN_POINT('Ctrl Pts',(-2.69442550748228,1.47867286261325,1.6286269149486));
#14272=CARTESIAN_POINT('Ctrl Pts',(-2.74079068806385,1.39418661255978,1.6336106631665));
#14273=CARTESIAN_POINT('Ctrl Pts',(-2.7832131563224,1.30745409967807,1.63859441138441));
#14274=CARTESIAN_POINT('Ctrl Pts',(-2.82147710351386,1.21888030763773,1.64357815960231));
#14275=CARTESIAN_POINT('Ctrl Pts',(-2.85972710562926,1.13033879580782,1.64856009152176));
#14276=CARTESIAN_POINT('Ctrl Pts',(-2.89382142398838,1.03995774068917,1.65354202344122));
#14277=CARTESIAN_POINT('Ctrl Pts',(-2.92359140418526,0.948164306106309,
1.65852395536067));
#14278=CARTESIAN_POINT('Ctrl Pts',(-2.95335866331643,0.856379261719421,
1.66350543191656));
#14279=CARTESIAN_POINT('Ctrl Pts',(-2.97880223487575,0.763182512169141,
1.66848690847245));
#14280=CARTESIAN_POINT('Ctrl Pts',(-2.99980293344201,0.669017645890376,
1.67346838502835));
#14281=CARTESIAN_POINT('Ctrl Pts',(-3.02080744646165,0.574835676014279,
1.67845076639272));
#14282=CARTESIAN_POINT('Ctrl Pts',(-3.03736738830957,0.479685668652976,
1.68343314775708));
#14283=CARTESIAN_POINT('Ctrl Pts',(-3.04941463707283,0.384021641585425,
1.68841552912145));
#14284=CARTESIAN_POINT('Ctrl Pts',(-3.06147487006335,0.288254510191585,
1.69340328037343));
#14285=CARTESIAN_POINT('Ctrl Pts',(-3.06901264516244,0.191972689359046,
1.69839103162542));
#14286=CARTESIAN_POINT('Ctrl Pts',(-3.07201174019826,0.095635339096251,
1.7033787828774));
#14287=CARTESIAN_POINT('Ctrl Pts',(-3.075012606577,-0.000758910491449369,
1.70836948002397));
#14288=CARTESIAN_POINT('Ctrl Pts',(-3.07346946228496,-0.0972083160843792,
1.71336017717054));
#14289=CARTESIAN_POINT('Ctrl Pts',(-3.06741820345264,-0.193255828184808,
1.71835087431711));
#14290=CARTESIAN_POINT('Ctrl Pts',(-3.06135716458187,-0.289458572177848,
1.7233496374234));
#14291=CARTESIAN_POINT('Ctrl Pts',(-3.05077351079541,-0.385257689649415,
1.72834840052969));
#14292=CARTESIAN_POINT('Ctrl Pts',(-3.03575475640733,-0.480203403726241,
1.73334716363598));
#14293=CARTESIAN_POINT('Ctrl Pts',(-3.02703088524136,-0.535354061095335,
1.73625077096596));
#14294=CARTESIAN_POINT('Ctrl Pts',(-3.01681154598786,-0.59021698782647,
1.73915437829595));
#14295=CARTESIAN_POINT('Ctrl Pts',(-3.00512162006299,-0.644706366208652,
1.74205798562594));
#14296=CARTESIAN_POINT('Ctrl Pts',(-2.98499339097518,-0.738528576715243,
1.7470575445534));
#14297=CARTESIAN_POINT('Ctrl Pts',(-2.96043180028799,-0.831572020007051,
1.75205710348086));
#14298=CARTESIAN_POINT('Ctrl Pts',(-2.93151159147554,-0.923386180882382,
1.75705666240832));
#14299=CARTESIAN_POINT('Ctrl Pts',(-2.90263060966395,-1.01507580620574,
1.76204943999807));
#14300=CARTESIAN_POINT('Ctrl Pts',(-2.86940289013932,-1.10553904783446,
1.76704221758783));
#14301=CARTESIAN_POINT('Ctrl Pts',(-2.8319541189141,-1.19433584822924,1.77203499517759));
#14302=CARTESIAN_POINT('Ctrl Pts',(-2.79454485185385,-1.28303897816871,
1.77702250595877));
#14303=CARTESIAN_POINT('Ctrl Pts',(-2.75292355451497,-1.37007875917954,
1.78201001673995));
#14304=CARTESIAN_POINT('Ctrl Pts',(-2.70726530367091,-1.45503155482609,
1.78699752752113));
#14305=CARTESIAN_POINT('Ctrl Pts',(-2.66163971859919,-1.53992357178246,
1.79198147003395));
#14306=CARTESIAN_POINT('Ctrl Pts',(-2.61198312884155,-1.62273118607782,
1.79696541254677));
#14307=CARTESIAN_POINT('Ctrl Pts',(-2.55851776865546,-1.70305286984119,
1.8019493550596));
#14308=CARTESIAN_POINT('Ctrl Pts',(-2.50507187673896,-1.78334530617803,
1.80693148277614));
#14309=CARTESIAN_POINT('Ctrl Pts',(-2.44782021295935,-1.86115324548523,
1.81191361049269));
#14310=CARTESIAN_POINT('Ctrl Pts',(-2.38702928791256,-1.93610263897544,
1.81689573820924));
#14311=CARTESIAN_POINT('Ctrl Pts',(-2.32624390369737,-2.01104520115048,
1.82187741182625));
#14312=CARTESIAN_POINT('Ctrl Pts',(-2.26192017623445,-2.0831293947229,1.82685908544326));
#14313=CARTESIAN_POINT('Ctrl Pts',(-2.19436532499682,-2.15201372450355,
1.83184075906028));
#14314=CARTESIAN_POINT('Ctrl Pts',(-2.12679819002139,-2.22091057976577,
1.83682333851264));
#14315=CARTESIAN_POINT('Ctrl Pts',(-2.05599907181081,-2.28660610232763,
1.84180591796501));
#14316=CARTESIAN_POINT('Ctrl Pts',(-1.98231173822915,-2.34879595164819,
1.84678849741737));
#14317=CARTESIAN_POINT('Ctrl Pts',(-1.90854498399631,-2.41105282956226,
1.85177644712383));
#14318=CARTESIAN_POINT('Ctrl Pts',(-1.83188413571029,-2.46979620735661,
1.85676439683028));
#14319=CARTESIAN_POINT('Ctrl Pts',(-1.75270553031896,-2.52476247872732,
1.86175234653674));
#14320=CARTESIAN_POINT('Ctrl Pts',(-1.6734801539065,-2.57976121882652,1.86674324263888));
#14321=CARTESIAN_POINT('Ctrl Pts',(-1.59173443083607,-2.63097817697288,
1.87173413874102));
#14322=CARTESIAN_POINT('Ctrl Pts',(-1.50787130299238,-2.6781946127218,1.87672503484316));
#14323=CARTESIAN_POINT('Ctrl Pts',(-1.42387266072209,-2.72548734550829,
1.88172399573421));
#14324=CARTESIAN_POINT('Ctrl Pts',(-1.33775017361861,-2.76876645086329,
1.88672295662526));
#14325=CARTESIAN_POINT('Ctrl Pts',(-1.24992878636426,-2.80786044507521,
1.89172191751631));
#14326=CARTESIAN_POINT('Ctrl Pts',(-1.19895265514617,-2.83055264615619,
1.89462357614757));
#14327=CARTESIAN_POINT('Ctrl Pts',(-1.1474044639194,-2.85183569365316,1.89752523477884));
#14328=CARTESIAN_POINT('Ctrl Pts',(-1.09536956545426,-2.87168378570422,
1.90042689341011));
#14329=CARTESIAN_POINT('Ctrl Pts',(-1.00571413125093,-2.90588178288372,
1.90542641242849));
#14330=CARTESIAN_POINT('Ctrl Pts',(-0.914298179497828,-2.93593718597948,
1.91042593144687));
#14331=CARTESIAN_POINT('Ctrl Pts',(-0.821540285226743,-2.96166740363424,
1.91542545046525));
#14332=CARTESIAN_POINT('Ctrl Pts',(-0.72890821070842,-2.98736272000485,
1.9204181879773));
#14333=CARTESIAN_POINT('Ctrl Pts',(-0.634938230676253,-3.00874439452058,
1.92541092548935));
#14334=CARTESIAN_POINT('Ctrl Pts',(-0.540067884674282,-3.02567825948885,
1.93040366300141));
#14335=CARTESIAN_POINT('Ctrl Pts',(-0.445297618949502,-3.04259426064643,
1.93539113359313));
#14336=CARTESIAN_POINT('Ctrl Pts',(-0.34962930525442,-3.05507170308052,
1.94037860418486));
#14337=CARTESIAN_POINT('Ctrl Pts',(-0.253513600610845,-3.06302678804893,
1.94536607477658));
#14338=CARTESIAN_POINT('Ctrl Pts',(-0.157466661538478,-3.0709761815857,
1.95034997710373));
#14339=CARTESIAN_POINT('Ctrl Pts',(-0.0609734040397047,-3.07440961357692,
1.95533387943087));
#14340=CARTESIAN_POINT('Ctrl Pts',(0.0355083839726203,-3.0732948775976,
1.96031778175802));
#14341=CARTESIAN_POINT('Ctrl Pts',(0.13195504026161,-3.0721805475249,1.96529986930663));
#14342=CARTESIAN_POINT('Ctrl Pts',(0.228389796879552,-3.06652134506973,
1.97028195685525));
#14343=CARTESIAN_POINT('Ctrl Pts',(0.324353808531808,-3.05633716348359,
1.97526404440386));
#14344=CARTESIAN_POINT('Ctrl Pts',(0.42030907471396,-3.04615391001054,1.98024567792084));
#14345=CARTESIAN_POINT('Ctrl Pts',(0.515793244734481,-3.03144654378952,
1.98522731143781));
#14346=CARTESIAN_POINT('Ctrl Pts',(0.610352614800831,-3.01228682824292,
1.99020894495478));
#14347=CARTESIAN_POINT('Ctrl Pts',(0.704929181312647,-2.99312362833508,
1.99519148442522));
#14348=CARTESIAN_POINT('Ctrl Pts',(0.798580183652301,-2.96950655824357,
2.00017402389566));
#14349=CARTESIAN_POINT('Ctrl Pts',(0.890863184148258,-2.94155826682546,
2.0051565633661));
#14350=CARTESIAN_POINT('Ctrl Pts',(0.983245656525631,-2.91357984993338,
2.01014447351774));
#14351=CARTESIAN_POINT('Ctrl Pts',(1.07425676240429,-2.88126101868106,2.01513238366937));
#14352=CARTESIAN_POINT('Ctrl Pts',(1.16347049934951,-2.84477391845879,2.020120293821));
#14353=CARTESIAN_POINT('Ctrl Pts',(1.25273693878055,-2.80826526369854,2.02511115055097));
#14354=CARTESIAN_POINT('Ctrl Pts',(1.34020349726109,-2.76758362200166,2.03010200728093));
#14355=CARTESIAN_POINT('Ctrl Pts',(1.42546732052527,-2.72294788200482,2.0350928640109));
#14356=CARTESIAN_POINT('Ctrl Pts',(1.51086893430869,-2.67824000846346,2.04009178621006));
#14357=CARTESIAN_POINT('Ctrl Pts',(1.59406032626629,-2.62956549869764,2.04509070840922));
#14358=CARTESIAN_POINT('Ctrl Pts',(1.67466630137768,-2.57718742605772,2.05008963060838));
#14359=CARTESIAN_POINT('Ctrl Pts',(1.72146101309108,-2.54678004241276,2.05299168747035));
#14360=CARTESIAN_POINT('Ctrl Pts',(1.7673849620253,-2.51512525908508,2.05589374433232));
#14361=CARTESIAN_POINT('Ctrl Pts',(1.81237000721957,-2.48228064628699,2.05879580119428));
#14362=CARTESIAN_POINT('Ctrl Pts',(1.8892313844923,-2.4261623926596,2.06375425097179));
#14363=CARTESIAN_POINT('Ctrl Pts',(1.96362979729519,-2.36636412933964,2.0687127007493));
#14364=CARTESIAN_POINT('Ctrl Pts',(2.0351876424133,-2.30313124032657,2.0736711505268));
#14365=CARTESIAN_POINT('Ctrl Pts',(2.10664810430205,-2.23998440509172,2.07862285233906));
#14366=CARTESIAN_POINT('Ctrl Pts',(2.1752753464389,-2.17341252342043,2.08357455415132));
#14367=CARTESIAN_POINT('Ctrl Pts',(2.24072173531615,-2.10370348549451,2.08852625596358));
#14368=CARTESIAN_POINT('Ctrl Pts',(2.30674986141293,-2.03337482068628,2.09352197226302));
#14369=CARTESIAN_POINT('Ctrl Pts',(2.36953992237088,-1.95985320948171,2.09851768856246));
#14370=CARTESIAN_POINT('Ctrl Pts',(2.42876994344176,-1.88347519543899,2.1035134048619));
#14371=CARTESIAN_POINT('Ctrl Pts',(2.48737572225326,-1.8079021512948,2.10845646986773));
#14372=CARTESIAN_POINT('Ctrl Pts',(2.54249586388351,-1.72953298782537,2.11339953487355));
#14373=CARTESIAN_POINT('Ctrl Pts',(2.59385731432301,-1.64872874753035,2.11834259987938));
#14374=CARTESIAN_POINT('Ctrl Pts',(2.6452017517199,-1.56795127295109,2.12328402753707));
#14375=CARTESIAN_POINT('Ctrl Pts',(2.69278973145011,-1.48474070068797,2.12822545519475));
#14376=CARTESIAN_POINT('Ctrl Pts',(2.73639132183341,-1.39948732891541,2.13316688285244));
#14377=CARTESIAN_POINT('Ctrl Pts',(2.77999087058241,-1.31423794911211,2.13810807912892));
#14378=CARTESIAN_POINT('Ctrl Pts',(2.81960419835934,-1.2269463583883,2.14304927540541));
#14379=CARTESIAN_POINT('Ctrl Pts',(2.85504772508441,-1.13802668575493,2.1479904716819));
#14380=CARTESIAN_POINT('Ctrl Pts',(2.89117186826129,-1.04739950267674,2.15302655297091));
#14381=CARTESIAN_POINT('Ctrl Pts',(2.92296420655424,-0.955081501042653,
2.15806263425993));
#14382=CARTESIAN_POINT('Ctrl Pts',(2.95028273665268,-0.861530048117416,
2.16309871554895));
#14383=CARTESIAN_POINT('Ctrl Pts',(2.97712156033067,-0.769621334843533,
2.16804636453508));
#14384=CARTESIAN_POINT('Ctrl Pts',(2.99964237774386,-0.676522593922476,
2.1729940135212));
#14385=CARTESIAN_POINT('Ctrl Pts',(3.0177620145246,-0.582678876991815,2.17794166250733));
#14386=CARTESIAN_POINT('Ctrl Pts',(3.0363674460371,-0.486319172359758,2.18302195994779));
#14387=CARTESIAN_POINT('Ctrl Pts',(3.05033226418924,-0.389174478221524,
2.18810225738826));
#14388=CARTESIAN_POINT('Ctrl Pts',(3.05962333423175,-0.291731559185131,
2.19318255482872));
#14389=CARTESIAN_POINT('Ctrl Pts',(3.06891440427426,-0.194288640148734,
2.19826285226918));
#14390=CARTESIAN_POINT('Ctrl Pts',(3.07353177061625,-0.0965480017052525,
2.20334314970964));
#14391=CARTESIAN_POINT('Ctrl Pts',(3.0734998353151,0.00100614018966156,
2.2084234471501));
#14392=CARTESIAN_POINT('Origin',(0.,0.,-2.20842344717744));
#14393=CARTESIAN_POINT('',(-1.87240768645124,2.43731239395329,0.562647869306095));
#14394=CARTESIAN_POINT('',(-1.87460960294492,2.44013607231272,0.645925936011554));
#14395=CARTESIAN_POINT('',(-1.87240768645123,2.4373123939533,-2.20842344717744));
#14396=CARTESIAN_POINT('',(3.07312700507994,-0.003721818839033,0.20842328729948));
#14397=CARTESIAN_POINT('Ctrl Pts',(3.07349774975442,-0.00371917390008725,
0.208423447177455));
#14398=CARTESIAN_POINT('Ctrl Pts',(3.07361316870223,0.0916621892469147,
0.213347842393274));
#14399=CARTESIAN_POINT('Ctrl Pts',(3.06928430893304,0.187123126142624,0.218272237609092));
#14400=CARTESIAN_POINT('Ctrl Pts',(3.06051597387791,0.282213081975554,0.22319663282491));
#14401=CARTESIAN_POINT('Ctrl Pts',(3.05175038029966,0.377273307316475,0.228119488396596));
#14402=CARTESIAN_POINT('Ctrl Pts',(3.03854810894313,0.471962334451556,0.233042343968281));
#14403=CARTESIAN_POINT('Ctrl Pts',(3.02096597683338,0.565832852364695,0.237965199539966));
#14404=CARTESIAN_POINT('Ctrl Pts',(3.00338428142197,0.659701038757444,0.242887932839628));
#14405=CARTESIAN_POINT('Ctrl Pts',(2.98142302492759,0.752750314370692,0.24781066613929));
#14406=CARTESIAN_POINT('Ctrl Pts',(2.9551902667484,0.844542916207064,0.252733399438952));
#14407=CARTESIAN_POINT('Ctrl Pts',(2.92895060932353,0.936359659603639,0.257657427423152));
#14408=CARTESIAN_POINT('Ctrl Pts',(2.89843734394202,1.02691864090875,0.262581455407353));
#14409=CARTESIAN_POINT('Ctrl Pts',(2.86380821853239,1.11579780312849,0.267505483391553));
#14410=CARTESIAN_POINT('Ctrl Pts',(2.82913852575285,1.20478108561716,0.272435279782038));
#14411=CARTESIAN_POINT('Ctrl Pts',(2.79034351655396,1.29208020342226,0.277365076172523));
#14412=CARTESIAN_POINT('Ctrl Pts',(2.7476287120519,1.37729398122116,0.282294872563008));
#14413=CARTESIAN_POINT('Ctrl Pts',(2.7048845348696,1.462566355965,0.287228058910085));
#14414=CARTESIAN_POINT('Ctrl Pts',(2.65821542095587,1.54575014745966,0.292161245257162));
#14415=CARTESIAN_POINT('Ctrl Pts',(2.60787122855021,1.62647161220232,0.297094431604238));
#14416=CARTESIAN_POINT('Ctrl Pts',(2.55744525952703,1.70732419690207,0.302035631175359));
#14417=CARTESIAN_POINT('Ctrl Pts',(2.50333255845057,1.78570610794303,0.306976830746478));
#14418=CARTESIAN_POINT('Ctrl Pts',(2.4458241421049,1.86127550778944,0.311918030317599));
#14419=CARTESIAN_POINT('Ctrl Pts',(2.42712569901718,1.88584634823316,0.313524625401182));
#14420=CARTESIAN_POINT('Ctrl Pts',(2.40806856342506,1.91012014284281,0.315131220484766));
#14421=CARTESIAN_POINT('Ctrl Pts',(2.38866356117224,1.93408599641483,0.31673781556835));
#14422=CARTESIAN_POINT('Ctrl Pts',(2.32818661500641,2.00877713107227,0.32174487318753));
#14423=CARTESIAN_POINT('Ctrl Pts',(2.26409871749897,2.08075782097448,0.326751930806709));
#14424=CARTESIAN_POINT('Ctrl Pts',(2.19667160266441,2.14965953584464,0.331758988425889));
#14425=CARTESIAN_POINT('Ctrl Pts',(2.12933568438833,2.21846805972945,0.33675927389674));
#14426=CARTESIAN_POINT('Ctrl Pts',(2.05866982887286,2.28420557567377,0.341759559367591));
#14427=CARTESIAN_POINT('Ctrl Pts',(1.98498641726937,2.34653599445142,0.346759844838442));
#14428=CARTESIAN_POINT('Ctrl Pts',(1.91138064299977,2.40880073810045,0.351754861703726));
#14429=CARTESIAN_POINT('Ctrl Pts',(1.83476396597669,2.46766524067924,0.356749878569008));
#14430=CARTESIAN_POINT('Ctrl Pts',(1.75548533902005,2.52283044901667,0.361744895434291));
#14431=CARTESIAN_POINT('Ctrl Pts',(1.67626391327478,2.57795585448587,0.366736308288929));
#14432=CARTESIAN_POINT('Ctrl Pts',(1.59438471424826,2.62938702330613,0.371727721143567));
#14433=CARTESIAN_POINT('Ctrl Pts',(1.51022870707359,2.67686598512717,0.376719133998204));
#14434=CARTESIAN_POINT('Ctrl Pts',(1.42610372539023,2.72432744305077,0.381708706686686));
#14435=CARTESIAN_POINT('Ctrl Pts',(1.33970398406318,2.76783937455939,0.386698279375168));
#14436=CARTESIAN_POINT('Ctrl Pts',(1.25143748023826,2.80718835902668,0.39168785206365));
#14437=CARTESIAN_POINT('Ctrl Pts',(1.16317963125899,2.84653348518564,0.396676935506727));
#14438=CARTESIAN_POINT('Ctrl Pts',(1.07305578331699,2.88171629801509,0.401666018949803));
#14439=CARTESIAN_POINT('Ctrl Pts',(0.98149550589776,2.91257082693323,0.406655102392879));
#14440=CARTESIAN_POINT('Ctrl Pts',(0.889919429458282,2.94343067989953,0.411645046718343));
#14441=CARTESIAN_POINT('Ctrl Pts',(0.796906845792688,2.96996062600182,0.416634991043808));
#14442=CARTESIAN_POINT('Ctrl Pts',(0.702903124588431,2.99204435920389,0.421624935369272));
#14443=CARTESIAN_POINT('Ctrl Pts',(0.608800402423276,3.01415135011086,0.426620134904602));
#14444=CARTESIAN_POINT('Ctrl Pts',(0.513704885280354,3.03180267934536,0.431615334439933));
#14445=CARTESIAN_POINT('Ctrl Pts',(0.418072580235202,3.04493309740222,0.436610533975263));
#14446=CARTESIAN_POINT('Ctrl Pts',(0.322384911934895,3.0580711168934,0.441608625321119));
#14447=CARTESIAN_POINT('Ctrl Pts',(0.226160272395216,3.06668297410534,0.446606716666975));
#14448=CARTESIAN_POINT('Ctrl Pts',(0.129858157580303,3.07075546224538,0.451604808012832));
#14449=CARTESIAN_POINT('Ctrl Pts',(0.0334036979499793,3.07483439284471,
0.456610806072938));
#14450=CARTESIAN_POINT('Ctrl Pts',(-0.0631280445224013,3.07435961705346,
0.461616804133045));
#14451=CARTESIAN_POINT('Ctrl Pts',(-0.15927927418525,3.06937002702754,0.466622802193152));
#14452=CARTESIAN_POINT('Ctrl Pts',(-0.213596744417433,3.06655132248622,
0.469450775912943));
#14453=CARTESIAN_POINT('Ctrl Pts',(-0.267792888430964,3.06229274258228,
0.472278749632735));
#14454=CARTESIAN_POINT('Ctrl Pts',(-0.32178651822468,3.05660852689526,0.475106723352527));
#14455=CARTESIAN_POINT('Ctrl Pts',(-0.417397797165186,3.04654298520664,
0.480114465658285));
#14456=CARTESIAN_POINT('Ctrl Pts',(-0.51269765553892,3.0319700686472,0.485122207964043));
#14457=CARTESIAN_POINT('Ctrl Pts',(-0.607228892070632,3.01291807433171,
0.490129950269802));
#14458=CARTESIAN_POINT('Ctrl Pts',(-0.701640883960441,2.9938901127944,0.495131375653663));
#14459=CARTESIAN_POINT('Ctrl Pts',(-0.795285755605436,2.97039438641494,
0.500132801037524));
#14460=CARTESIAN_POINT('Ctrl Pts',(-0.887711441776127,2.94251094239932,
0.505134226421385));
#14461=CARTESIAN_POINT('Ctrl Pts',(-0.980035738273924,2.91465808612814,
0.510130165312208));
#14462=CARTESIAN_POINT('Ctrl Pts',(-1.07114309297848,2.88242721119824,0.515126104203032));
#14463=CARTESIAN_POINT('Ctrl Pts',(-1.16059282370576,2.84594914704439,0.520122043093856));
#14464=CARTESIAN_POINT('Ctrl Pts',(-1.2499841043487,2.8094949191381,0.525114717435451));
#14465=CARTESIAN_POINT('Ctrl Pts',(-1.33771951023168,2.76879918260247,0.530107391777045));
#14466=CARTESIAN_POINT('Ctrl Pts',(-1.4233754604941,2.72404195056964,0.53510006611864));
#14467=CARTESIAN_POINT('Ctrl Pts',(-1.50901251334216,2.6792945928766,0.540091638976503));
#14468=CARTESIAN_POINT('Ctrl Pts',(-1.59257063149162,2.63048771559511,0.545083211834367));
#14469=CARTESIAN_POINT('Ctrl Pts',(-1.67364885409248,2.57784828164788,0.550074784692231));
#14470=CARTESIAN_POINT('Ctrl Pts',(-1.74172381310375,2.53365112002564,0.554265812896852));
#14471=CARTESIAN_POINT('Ctrl Pts',(-1.80805081637324,2.48675303952213,0.558456841101473));
#14472=CARTESIAN_POINT('Ctrl Pts',(-1.87240768645124,2.43731239395329,0.562647869306095));
#14473=CARTESIAN_POINT('',(0.793799282532869,-2.96922295374569,0.));
#14474=CARTESIAN_POINT('Ctrl Pts',(0.793799282532864,-2.9692229537457,-2.77555756156289E-16));
#14475=CARTESIAN_POINT('Ctrl Pts',(1.77865212890011,-2.70592999965461,0.0527896359280583));
#14476=CARTESIAN_POINT('Ctrl Pts',(2.87781245894031,-1.66713001938774,0.122263670929926));
#14477=CARTESIAN_POINT('Ctrl Pts',(3.07278338813921,-0.326580109130746,
0.191737705931794));
#14478=CARTESIAN_POINT('Ctrl Pts',(3.07038535690584,-0.00374137810051507,
0.208422105005604));
#14479=CARTESIAN_POINT('',(-0.794090168544026,-2.96914517230494,1.17075019123725E-8));
#14480=CARTESIAN_POINT('Origin',(0.,0.,0.));
#14481=CARTESIAN_POINT('',(3.07349932342359,0.00203934174087983,0.291576552822545));
#14482=CARTESIAN_POINT('Ctrl Pts',(-0.794090168544026,-2.96914517230494,
1.17075020789059E-8));
#14483=CARTESIAN_POINT('Ctrl Pts',(-0.701681804640572,-2.99385954934229,
0.00498338006721378));
#14484=CARTESIAN_POINT('Ctrl Pts',(-0.607952002928877,-3.01430028785914,
0.00996674842692535));
#14485=CARTESIAN_POINT('Ctrl Pts',(-0.513333254559353,-3.0303285663049,
0.014950116786637));
#14486=CARTESIAN_POINT('Ctrl Pts',(-0.418842318648037,-3.04633519350601,
0.0199267535358467));
#14487=CARTESIAN_POINT('Ctrl Pts',(-0.323465254399358,-3.05794113166517,
0.0249033902850561));
#14488=CARTESIAN_POINT('Ctrl Pts',(-0.22764855061392,-3.06505764830017,
0.0298800270342658));
#14489=CARTESIAN_POINT('Ctrl Pts',(-0.127996697095714,-3.07245900991306,
0.0350558581446337));
#14490=CARTESIAN_POINT('Ctrl Pts',(-0.0278697350491978,-3.07500388554417,
0.0402316892550016));
#14491=CARTESIAN_POINT('Ctrl Pts',(0.0722193954406267,-3.0726513972337,
0.0454075203653694));
#14492=CARTESIAN_POINT('Ctrl Pts',(0.16828711453244,-3.07039342791104,0.0503753953658225));
#14493=CARTESIAN_POINT('Ctrl Pts',(0.264319494128326,-3.06362406015239,
0.0553432703662757));
#14494=CARTESIAN_POINT('Ctrl Pts',(0.359860335496799,-3.05236019973661,
0.0603111453667289));
#14495=CARTESIAN_POINT('Ctrl Pts',(0.455369297438528,-3.04110009777018,
0.0652773627199928));
#14496=CARTESIAN_POINT('Ctrl Pts',(0.550386608294095,-3.02534853439546,
0.070243580073257));
#14497=CARTESIAN_POINT('Ctrl Pts',(0.644460645377193,-3.00517432548596,
0.0752097974265209));
#14498=CARTESIAN_POINT('Ctrl Pts',(0.738529417198413,-2.98500124571365,
0.0801757368238713));
#14499=CARTESIAN_POINT('Ctrl Pts',(0.831654588017938,-2.96040610585117,
0.0851416762212218));
#14500=CARTESIAN_POINT('Ctrl Pts',(0.92339529074792,-2.93150872197655,0.0901076156185723));
#14501=CARTESIAN_POINT('Ctrl Pts',(1.01515633557142,-2.90260493055034,0.0950746561368062));
#14502=CARTESIAN_POINT('Ctrl Pts',(1.10553188114381,-2.86939713383231,0.10004169665504));
#14503=CARTESIAN_POINT('Ctrl Pts',(1.19409783655646,-2.83205448512757,0.105008737173274));
#14504=CARTESIAN_POINT('Ctrl Pts',(1.28275886820376,-2.79467174880209,0.109981109847725));
#14505=CARTESIAN_POINT('Ctrl Pts',(1.36960602534491,-2.75314547478082,0.114953482522177));
#14506=CARTESIAN_POINT('Ctrl Pts',(1.45423707810273,-2.70769214843033,0.119925855196628));
#14507=CARTESIAN_POINT('Ctrl Pts',(1.53892195546335,-2.66220991416533,0.124901390256227));
#14508=CARTESIAN_POINT('Ctrl Pts',(1.62138754456656,-2.61279588348197,0.129876925315825));
#14509=CARTESIAN_POINT('Ctrl Pts',(1.70125981259282,-2.55971039378611,0.134852460375423));
#14510=CARTESIAN_POINT('Ctrl Pts',(1.78125220835393,-2.5065450636176,0.139835478630018));
#14511=CARTESIAN_POINT('Ctrl Pts',(1.85864314528324,-2.44969751742716,0.144818496884613));
#14512=CARTESIAN_POINT('Ctrl Pts',(1.93309117950554,-2.38946871536705,0.149801515139208));
#14513=CARTESIAN_POINT('Ctrl Pts',(1.95449800380548,-2.37215049606194,0.151234334653837));
#14514=CARTESIAN_POINT('Ctrl Pts',(1.97566174365417,-2.35455294918859,0.152667154168466));
#14515=CARTESIAN_POINT('Ctrl Pts',(1.99657486217591,-2.33668377615099,0.154099973683096));
#14516=CARTESIAN_POINT('Ctrl Pts',(2.06861067308952,-2.27513291902838,0.159035359839011));
#14517=CARTESIAN_POINT('Ctrl Pts',(2.13793692587052,-2.21012849622858,0.163970745994926));
#14518=CARTESIAN_POINT('Ctrl Pts',(2.20419808661067,-2.14194141959622,0.168906132150841));
#14519=CARTESIAN_POINT('Ctrl Pts',(2.27282058312028,-2.07132437371387,0.174017399678828));
#14520=CARTESIAN_POINT('Ctrl Pts',(2.33815500896462,-1.99729382004998,0.179128667206816));
#14521=CARTESIAN_POINT('Ctrl Pts',(2.39984250587212,-1.92019743698648,0.184239934734803));
#14522=CARTESIAN_POINT('Ctrl Pts',(2.45926136987769,-1.84593636739824,0.189163229168309));
#14523=CARTESIAN_POINT('Ctrl Pts',(2.51529650561875,-1.76883138580461,0.194086523601816));
#14524=CARTESIAN_POINT('Ctrl Pts',(2.56766478650435,-1.68923053315572,0.199009818035321));
#14525=CARTESIAN_POINT('Ctrl Pts',(2.62000290232932,-1.60967553201286,0.203930276563723));
#14526=CARTESIAN_POINT('Ctrl Pts',(2.66867810976985,-1.52762789052164,0.208850735092124));
#14527=CARTESIAN_POINT('Ctrl Pts',(2.71344918565114,-1.44346657976178,0.213771193620525));
#14528=CARTESIAN_POINT('Ctrl Pts',(2.75820745226931,-1.35932934803849,0.218690244377353));
#14529=CARTESIAN_POINT('Ctrl Pts',(2.79906359485162,-1.2730800467947,0.223609295134181));
#14530=CARTESIAN_POINT('Ctrl Pts',(2.83582177726882,-1.18512324151031,0.228528345891009));
#14531=CARTESIAN_POINT('Ctrl Pts',(2.87258009899405,-1.09716610288277,0.233447415290305));
#14532=CARTESIAN_POINT('Ctrl Pts',(2.90524025808181,-1.00750186476344,0.238366484689601));
#14533=CARTESIAN_POINT('Ctrl Pts',(2.93365459175633,-0.916554955399307,
0.243285554088897));
#14534=CARTESIAN_POINT('Ctrl Pts',(2.96209109854565,-0.825537075648002,
0.248208462082184));
#14535=CARTESIAN_POINT('Ctrl Pts',(2.98627503311865,-0.733234958457678,
0.253131370075472));
#14536=CARTESIAN_POINT('Ctrl Pts',(3.00610882031872,-0.640087502144834,
0.258054278068759));
#14537=CARTESIAN_POINT('Ctrl Pts',(3.02595191484239,-0.546896334890099,
0.262979496215793));
#14538=CARTESIAN_POINT('Ctrl Pts',(3.04144072570293,-0.452859483996052,
0.267904714362827));
#14539=CARTESIAN_POINT('Ctrl Pts',(3.05252927802725,-0.35842329275095,0.272829932509862));
#14540=CARTESIAN_POINT('Ctrl Pts',(3.06363201734979,-0.263866277250587,
0.277761452116186));
#14541=CARTESIAN_POINT('Ctrl Pts',(3.07032323534061,-0.168909351265706,
0.282692971722511));
#14542=CARTESIAN_POINT('Ctrl Pts',(3.07260901440491,-0.0740006391709276,
0.287624491328835));
#14543=CARTESIAN_POINT('Ctrl Pts',(3.07321961317529,-0.0486477326681363,
0.288941845160071));
#14544=CARTESIAN_POINT('Ctrl Pts',(3.07351613553083,-0.0232982459732372,
0.290259198991308));
#14545=CARTESIAN_POINT('Ctrl Pts',(3.07349932342359,0.00203934174087994,
0.291576552822545));
#14546=CARTESIAN_POINT('Ctrl Pts',(3.07648182967171,0.00204132070649662,
0.291576552822545));
#14547=CARTESIAN_POINT('Ctrl Pts',(3.07754652659738,0.136117656503392,0.298540662370786));
#14548=CARTESIAN_POINT('Ctrl Pts',(3.00879647423619,1.28547432247006,0.358294407847086));
#14549=CARTESIAN_POINT('Ctrl Pts',(1.56063394451812,3.27734706691301,0.470837789251445));
#14550=CARTESIAN_POINT('Ctrl Pts',(-0.867537302958989,3.14799344447871,
0.581990140766207));
#14551=CARTESIAN_POINT('Ctrl Pts',(-1.79004208889524,2.50612566616128,0.64035285635291));
#14552=CARTESIAN_POINT('Ctrl Pts',(-1.87460960294492,2.44013607231272,0.645925936011554));
#14553=CARTESIAN_POINT('Origin',(0.,0.,10.));
#14554=CARTESIAN_POINT('',(2.36142200728635,0.872635292378032,18.6688222409353));
#14555=CARTESIAN_POINT('',(2.36142200730535,0.872635292326632,18.9466764589532));
#14556=CARTESIAN_POINT('',(2.36142200728636,0.87263529237802,10.));
#14557=CARTESIAN_POINT('',(1.91346599666504,1.63598720337497,19.));
#14558=CARTESIAN_POINT('Ctrl Pts',(2.36142200732435,0.872635292275214,18.9466764589532));
#14559=CARTESIAN_POINT('Ctrl Pts',(2.31565239500422,0.99649158224678,18.9546790697769));
#14560=CARTESIAN_POINT('Ctrl Pts',(2.26020795009562,1.11655953327844,18.9624334565676));
#14561=CARTESIAN_POINT('Ctrl Pts',(2.13159976529488,1.34580753201374,18.9779049061883));
#14562=CARTESIAN_POINT('Ctrl Pts',(2.05881463877152,1.45471361970388,18.985602132961));
#14563=CARTESIAN_POINT('Ctrl Pts',(1.96587805277887,1.57273895687923,18.9948599363643));
#14564=CARTESIAN_POINT('Ctrl Pts',(1.95367226283063,1.58787562286953,18.9960660351914));
#14565=CARTESIAN_POINT('Ctrl Pts',(1.93624377484013,1.60898389621206,18.9977767766616));
#14566=CARTESIAN_POINT('Ctrl Pts',(1.93116605552455,1.61507485795793,18.9982738626392));
#14567=CARTESIAN_POINT('Ctrl Pts',(1.92188090786595,1.62610643482651,18.9991806156347));
#14568=CARTESIAN_POINT('Ctrl Pts',(1.91768297315338,1.63105498807247,18.9995897567832));
#14569=CARTESIAN_POINT('Ctrl Pts',(1.91346599666504,1.63598720337497,19.));
#14570=CARTESIAN_POINT('',(2.36142200728636,0.87263529237802,19.));
#14571=CARTESIAN_POINT('Origin',(0.,0.,19.));
#14572=CARTESIAN_POINT('',(2.36142200728636,0.87263529237802,20.));
#14573=CARTESIAN_POINT('',(2.36142200728636,0.87263529237802,10.));
#14574=CARTESIAN_POINT('Origin',(0.,0.,20.));
#14575=CARTESIAN_POINT('',(-1.91360951419324,1.63581932901806,18.9999983489143));
#14576=CARTESIAN_POINT('Origin',(0.,0.,19.));
#14577=CARTESIAN_POINT('Ctrl Pts',(-1.91360951419324,1.63581932901806,18.9999983489143));
#14578=CARTESIAN_POINT('Ctrl Pts',(-1.8600938132237,1.6984229140946,18.9947600671717));
#14579=CARTESIAN_POINT('Ctrl Pts',(-1.80340132000449,1.75851618901605,18.9895217854291));
#14580=CARTESIAN_POINT('Ctrl Pts',(-1.74379734202027,1.81575799047204,18.9842835036865));
#14581=CARTESIAN_POINT('Ctrl Pts',(-1.68427750262003,1.87291898785618,18.9790526164438));
#14582=CARTESIAN_POINT('Ctrl Pts',(-1.62185467307349,1.92723618657456,18.9738217292011));
#14583=CARTESIAN_POINT('Ctrl Pts',(-1.55683385998117,1.97840202750001,18.9685908419584));
#14584=CARTESIAN_POINT('Ctrl Pts',(-1.4918868023647,2.02950982914902,18.9633658883015));
#14585=CARTESIAN_POINT('Ctrl Pts',(-1.42434798122953,2.0774730912236,18.9581409346447));
#14586=CARTESIAN_POINT('Ctrl Pts',(-1.35455755196941,2.12202264087889,18.9529159809879));
#14587=CARTESIAN_POINT('Ctrl Pts',(-1.28481020389697,2.1665446903808,18.9476942526617));
#14588=CARTESIAN_POINT('Ctrl Pts',(-1.21281439735469,2.20765696094641,18.9424725243355));
#14589=CARTESIAN_POINT('Ctrl Pts',(-1.13894057102776,2.24513265213149,18.9372507960092));
#14590=CARTESIAN_POINT('Ctrl Pts',(-1.06508967852922,2.28259670914092,18.9320306887473));
#14591=CARTESIAN_POINT('Ctrl Pts',(-0.989362338275737,2.31642621871755,
18.9268105814854));
#14592=CARTESIAN_POINT('Ctrl Pts',(-0.912153717615124,2.34644024970612,
18.9215904742235));
#14593=CARTESIAN_POINT('Ctrl Pts',(-0.834945375056506,2.37645417258549,
18.9163703857641));
#14594=CARTESIAN_POINT('Ctrl Pts',(-0.756256196450567,2.402652477312,18.9111502973048));
#14595=CARTESIAN_POINT('Ctrl Pts',(-0.676500116885295,2.42490285204463,
18.9059302088455));
#14596=CARTESIAN_POINT('Ctrl Pts',(-0.596667246521566,2.44717464989699,
18.9007050943773));
#14597=CARTESIAN_POINT('Ctrl Pts',(-0.515765872187058,2.46549080080498,
18.8954799799091));
#14598=CARTESIAN_POINT('Ctrl Pts',(-0.434223277835914,2.47976942375404,
18.890254865441));
#14599=CARTESIAN_POINT('Ctrl Pts',(-0.352641288274004,2.49405494505316,
18.8850272265929));
#14600=CARTESIAN_POINT('Ctrl Pts',(-0.270417923313533,2.50429899596022,
18.8797995877449));
#14601=CARTESIAN_POINT('Ctrl Pts',(-0.187986351410114,2.5104715456829,18.8745719488968));
#14602=CARTESIAN_POINT('Ctrl Pts',(-0.105413386187175,2.51665468306364,
18.8693353431785));
#14603=CARTESIAN_POINT('Ctrl Pts',(-0.0226319659163586,2.51875235648336,
18.8640987374602));
#14604=CARTESIAN_POINT('Ctrl Pts',(0.0599242294916328,2.51678670862666,
18.8588621317418));
#14605=CARTESIAN_POINT('Ctrl Pts',(0.128041006268894,2.51516486067672,18.8545414299336));
#14606=CARTESIAN_POINT('Ctrl Pts',(0.196004367846044,2.51077775312145,18.8502207281253));
#14607=CARTESIAN_POINT('Ctrl Pts',(0.263574962959677,2.50366421248953,18.845900026317));
#14608=CARTESIAN_POINT('Ctrl Pts',(0.345901422450609,2.49499723813942,18.8406357825761));
#14609=CARTESIAN_POINT('Ctrl Pts',(0.427945987928208,2.48224996490047,18.8353715388353));
#14610=CARTESIAN_POINT('Ctrl Pts',(0.509273644888992,2.4654505885581,18.8301072950944));
#14611=CARTESIAN_POINT('Ctrl Pts',(0.590489053101737,2.44867439878021,18.8248503170832));
#14612=CARTESIAN_POINT('Ctrl Pts',(0.670989071903334,2.4278573082844,18.819593339072));
#14613=CARTESIAN_POINT('Ctrl Pts',(0.750344228463646,2.40307923065622,18.8143363610608));
#14614=CARTESIAN_POINT('Ctrl Pts',(0.830100521369724,2.37817590108544,18.8090528092888));
#14615=CARTESIAN_POINT('Ctrl Pts',(0.908699876890739,2.34927147444271,18.8037692575168));
#14616=CARTESIAN_POINT('Ctrl Pts',(0.985717073963406,2.31649910427287,18.7984857057448));
#14617=CARTESIAN_POINT('Ctrl Pts',(1.06221586746298,2.2839473252754,18.793237717616));
#14618=CARTESIAN_POINT('Ctrl Pts',(1.13715330866122,2.24757969720965,18.7879897294872));
#14619=CARTESIAN_POINT('Ctrl Pts',(1.21012998151385,2.20757597328864,18.7827417413584));
#14620=CARTESIAN_POINT('Ctrl Pts',(1.28308439897037,2.16758444913896,18.777495353687));
#14621=CARTESIAN_POINT('Ctrl Pts',(1.35407883312648,2.12395925246732,18.7722489660156));
#14622=CARTESIAN_POINT('Ctrl Pts',(1.42273781237011,2.07692642316773,18.7670025783441));
#14623=CARTESIAN_POINT('Ctrl Pts',(1.49139635411015,2.02989389356721,18.7617562241033));
#14624=CARTESIAN_POINT('Ctrl Pts',(1.55771909206239,1.97945403520153,18.7565098698626));
#14625=CARTESIAN_POINT('Ctrl Pts',(1.6213600736698,1.92587584270364,18.7512635156218));
#14626=CARTESIAN_POINT('Ctrl Pts',(1.68578564307139,1.87163711991841,18.745952482531));
#14627=CARTESIAN_POINT('Ctrl Pts',(1.74746249947729,1.81418244866758,18.7406414494403));
#14628=CARTESIAN_POINT('Ctrl Pts',(1.80606817423016,1.75383123476374,18.7353304163495));
#14629=CARTESIAN_POINT('Ctrl Pts',(1.86404498763655,1.69412761251034,18.7300763726789));
#14630=CARTESIAN_POINT('Ctrl Pts',(1.91901595311641,1.63158970209983,18.7248223290083));
#14631=CARTESIAN_POINT('Ctrl Pts',(1.97070894874087,1.56656071996991,18.7195682853376));
#14632=CARTESIAN_POINT('Ctrl Pts',(2.02324299766552,1.50047370590806,18.7142287575368));
#14633=CARTESIAN_POINT('Ctrl Pts',(2.07239117086506,1.43181423934472,18.708889229736));
#14634=CARTESIAN_POINT('Ctrl Pts',(2.11791422955211,1.36097228710239,18.7035497019352));
#14635=CARTESIAN_POINT('Ctrl Pts',(2.16343728823915,1.29013033486007,18.6982101741343));
#14636=CARTESIAN_POINT('Ctrl Pts',(2.20533504378927,1.21710635501938,18.6928706463335));
#14637=CARTESIAN_POINT('Ctrl Pts',(2.24341832330765,1.14231365073149,18.6875311185327));
#14638=CARTESIAN_POINT('Ctrl Pts',(2.2832324761903,1.06412164099167,18.6819489108323));
#14639=CARTESIAN_POINT('Ctrl Pts',(2.31901070827217,0.98373642613171,18.6763667031319));
#14640=CARTESIAN_POINT('Ctrl Pts',(2.3505213598588,0.901585041384082,18.6707844954316));
#14641=CARTESIAN_POINT('Ctrl Pts',(2.35421356200506,0.891959105270082,18.6701304105995));
#14642=CARTESIAN_POINT('Ctrl Pts',(2.3578472220091,0.882308951807992,18.6694763257674));
#14643=CARTESIAN_POINT('Ctrl Pts',(2.36142200728635,0.872635292378032,18.6688222409353));
#14644=CARTESIAN_POINT('Origin',(0.,0.,10.));
#14645=CARTESIAN_POINT('',(2.36142200245778,0.872635305444532,17.6666805052528));
#14646=CARTESIAN_POINT('',(2.36142200728635,0.872635292378034,17.9438262109491));
#14647=CARTESIAN_POINT('',(2.36142200728636,0.87263529237802,10.));
#14648=CARTESIAN_POINT('',(2.51749787287094,-0.00327262742782446,18.8874150286091));
#14649=CARTESIAN_POINT('Ctrl Pts',(2.36142200728635,0.872635292378034,17.9438262109491));
#14650=CARTESIAN_POINT('Ctrl Pts',(2.33264089115126,0.950519331253507,17.9490650608475));
#14651=CARTESIAN_POINT('Ctrl Pts',(2.2999848229152,1.02702598391504,17.9543039107459));
#14652=CARTESIAN_POINT('Ctrl Pts',(2.26361541332485,1.10174929569216,17.9595427606443));
#14653=CARTESIAN_POINT('Ctrl Pts',(2.22725452555323,1.17645509883978,17.9647803830131));
#14654=CARTESIAN_POINT('Ctrl Pts',(2.18718222668459,1.24937797670333,17.9700180053818));
#14655=CARTESIAN_POINT('Ctrl Pts',(2.14360739219153,1.32013393189548,17.9752556277506));
#14656=CARTESIAN_POINT('Ctrl Pts',(2.10002963900747,1.39089462640042,17.9804936009411));
#14657=CARTESIAN_POINT('Ctrl Pts',(2.05294912741505,1.45948771806852,17.9857315741316));
#14658=CARTESIAN_POINT('Ctrl Pts',(2.00261888863162,1.52555689402128,17.9909695473222));
#14659=CARTESIAN_POINT('Ctrl Pts',(1.95223681038431,1.59169412032992,17.9962129155541));
#14660=CARTESIAN_POINT('Ctrl Pts',(1.89859860128339,1.65530187235901,18.0014562837861));
#14661=CARTESIAN_POINT('Ctrl Pts',(1.84199822589728,1.71605617209673,18.006699652018));
#14662=CARTESIAN_POINT('Ctrl Pts',(1.78536754283389,1.77684300380438,18.0119458279047));
#14663=CARTESIAN_POINT('Ctrl Pts',(1.72577186567806,1.83477301881369,18.0171920037913));
#14664=CARTESIAN_POINT('Ctrl Pts',(1.66354099252487,1.88956016474453,18.022438179678));
#14665=CARTESIAN_POINT('Ctrl Pts',(1.60120331408269,1.94444134048175,18.027693359445));
#14666=CARTESIAN_POINT('Ctrl Pts',(1.53622176737099,1.99616858588041,18.0329485392119));
#14667=CARTESIAN_POINT('Ctrl Pts',(1.46895787176047,2.04449725384823,18.0382037189789));
#14668=CARTESIAN_POINT('Ctrl Pts',(1.41953954591432,2.08000399694817,18.0420646637509));
#14669=CARTESIAN_POINT('Ctrl Pts',(1.36888992101459,2.11367715937145,18.0459256085229));
#14670=CARTESIAN_POINT('Ctrl Pts',(1.31716077966232,2.14543555729818,18.049786553295));
#14671=CARTESIAN_POINT('Ctrl Pts',(1.24673044471657,2.18867529692748,18.0550433123749));
#14672=CARTESIAN_POINT('Ctrl Pts',(1.17403926396638,2.22852266631261,18.0603000714548));
#14673=CARTESIAN_POINT('Ctrl Pts',(1.09944747821751,2.26473430950325,18.0655568305348));
#14674=CARTESIAN_POINT('Ctrl Pts',(1.02496115897755,2.30089475247726,18.0708061569997));
#14675=CARTESIAN_POINT('Ctrl Pts',(0.948579983971734,2.33342948049938,18.0760554834646));
#14676=CARTESIAN_POINT('Ctrl Pts',(0.87069149526328,2.36213940530109,18.0813048099295));
#14677=CARTESIAN_POINT('Ctrl Pts',(0.79226710456764,2.39104686514307,18.0865902537274));
#14678=CARTESIAN_POINT('Ctrl Pts',(0.712314978667257,2.41607643120506,18.0918756975253));
#14679=CARTESIAN_POINT('Ctrl Pts',(0.631254210649159,2.43707291059125,18.0971611413232));
#14680=CARTESIAN_POINT('Ctrl Pts',(0.550890606996052,2.45788880943798,18.1024011275815));
#14681=CARTESIAN_POINT('Ctrl Pts',(0.469437811902277,2.47474061061156,18.1076411138399));
#14682=CARTESIAN_POINT('Ctrl Pts',(0.387320725466731,2.48752666430411,18.1128811000982));
#14683=CARTESIAN_POINT('Ctrl Pts',(0.305230502026731,2.50030853528976,18.1181193721978));
#14684=CARTESIAN_POINT('Ctrl Pts',(0.222476874103383,2.50902722947594,18.1233576442973));
#14685=CARTESIAN_POINT('Ctrl Pts',(0.139494101629973,2.51363236086951,18.1285959163968));
#14686=CARTESIAN_POINT('Ctrl Pts',(0.0565134860927702,2.51823737256385,
18.1338340523401));
#14687=CARTESIAN_POINT('Ctrl Pts',(-0.0266958016974763,2.51872900954754,
18.1390721882835));
#14688=CARTESIAN_POINT('Ctrl Pts',(-0.109696611036355,2.5151089247838,18.1443103242268));
#14689=CARTESIAN_POINT('Ctrl Pts',(-0.194001379126069,2.51143196778901,
18.1496307522978));
#14690=CARTESIAN_POINT('Ctrl Pts',(-0.278090571199433,2.5035129838956,18.1549511803689));
#14691=CARTESIAN_POINT('Ctrl Pts',(-0.36151034579989,2.49140854134356,18.1602716084399));
#14692=CARTESIAN_POINT('Ctrl Pts',(-0.443757757009223,2.47947421199772,
18.1655172643705));
#14693=CARTESIAN_POINT('Ctrl Pts',(-0.525354000224621,2.4634714718566,18.1707629203012));
#14694=CARTESIAN_POINT('Ctrl Pts',(-0.605875105640386,2.44350600702459,
18.1760085762319));
#14695=CARTESIAN_POINT('Ctrl Pts',(-0.688117845721868,2.42311365738773,
18.1813663903731));
#14696=CARTESIAN_POINT('Ctrl Pts',(-0.769238453549124,2.39858731570485,
18.1867242045143));
#14697=CARTESIAN_POINT('Ctrl Pts',(-0.848804130873332,2.37009236052361,
18.1920820186555));
#14698=CARTESIAN_POINT('Ctrl Pts',(-0.928369808197552,2.34159740534236,
18.1974398327967));
#14699=CARTESIAN_POINT('Ctrl Pts',(-1.00638011389758,2.30913409197741,18.2027976469379));
#14700=CARTESIAN_POINT('Ctrl Pts',(-1.08242824839124,2.27291780253591,18.2081554610792));
#14701=CARTESIAN_POINT('Ctrl Pts',(-1.15691530191002,2.23744494435415,18.2134032924867));
#14702=CARTESIAN_POINT('Ctrl Pts',(-1.22979665503187,2.19823998620112,18.2186511238942));
#14703=CARTESIAN_POINT('Ctrl Pts',(-1.30067285720552,2.15547126367503,18.2238989553018));
#14704=CARTESIAN_POINT('Ctrl Pts',(-1.3714481990332,2.1127634031593,18.2291393187853));
#14705=CARTESIAN_POINT('Ctrl Pts',(-1.44022366427724,2.06650208784539,18.2343796822688));
#14706=CARTESIAN_POINT('Ctrl Pts',(-1.50662195862707,2.01690270558169,18.2396200457524));
#14707=CARTESIAN_POINT('Ctrl Pts',(-1.57361978096847,1.96685547720503,18.244907725882));
#14708=CARTESIAN_POINT('Ctrl Pts',(-1.63819684952987,1.91340979165176,18.2501954060116));
#14709=CARTESIAN_POINT('Ctrl Pts',(-1.69999317353582,1.85683318042618,18.2554830861412));
#14710=CARTESIAN_POINT('Ctrl Pts',(-1.76112710793961,1.80086300914027,18.260714088072));
#14711=CARTESIAN_POINT('Ctrl Pts',(-1.81953927606449,1.74182903057646,18.2659450900029));
#14712=CARTESIAN_POINT('Ctrl Pts',(-1.87491370595946,1.68003120364039,18.2711760919337));
#14713=CARTESIAN_POINT('Ctrl Pts',(-1.93027011185859,1.61825349147168,18.2764053912094));
#14714=CARTESIAN_POINT('Ctrl Pts',(-1.98259043442758,1.55371406188586,18.281634690485));
#14715=CARTESIAN_POINT('Ctrl Pts',(-2.03159657928035,1.48674866371434,18.2868639897607));
#14716=CARTESIAN_POINT('Ctrl Pts',(-2.08060166653038,1.41978471072462,18.2920931761828));
#14717=CARTESIAN_POINT('Ctrl Pts',(-2.12629244576203,1.35039526739066,18.2973223626048));
#14718=CARTESIAN_POINT('Ctrl Pts',(-2.16843289020646,1.27894685216816,18.3025515490269));
#14719=CARTESIAN_POINT('Ctrl Pts',(-2.21139437029597,1.20610638481011,18.3078826173466));
#14720=CARTESIAN_POINT('Ctrl Pts',(-2.25066543593152,1.13112628537219,18.3132136856663));
#14721=CARTESIAN_POINT('Ctrl Pts',(-2.28604494139125,1.05442153617018,18.318544753986));
#14722=CARTESIAN_POINT('Ctrl Pts',(-2.32079919680567,0.979072364082393,
18.3237816081366));
#14723=CARTESIAN_POINT('Ctrl Pts',(-2.35179821306474,0.902059468043717,
18.3290184622873));
#14724=CARTESIAN_POINT('Ctrl Pts',(-2.37890060185484,0.823794984504448,
18.3342553164379));
#14725=CARTESIAN_POINT('Ctrl Pts',(-2.40673437315984,0.743418462973202,
18.3396334918421));
#14726=CARTESIAN_POINT('Ctrl Pts',(-2.4304580292705,0.661722333881856,18.3450116672464));
#14727=CARTESIAN_POINT('Ctrl Pts',(-2.44997408672011,0.579165973102676,
18.3503898426506));
#14728=CARTESIAN_POINT('Ctrl Pts',(-2.46949014416972,0.496609612323496,
18.3557680180548));
#14729=CARTESIAN_POINT('Ctrl Pts',(-2.48479857801772,0.413193544991591,
18.361146193459));
#14730=CARTESIAN_POINT('Ctrl Pts',(-2.49585925389778,0.329382505201515,
18.3665243688632));
#14731=CARTESIAN_POINT('Ctrl Pts',(-2.50668767148743,0.247331376743258,
18.3717896103167));
#14732=CARTESIAN_POINT('Ctrl Pts',(-2.51348535610504,0.164596633023612,
18.3770548517702));
#14733=CARTESIAN_POINT('Ctrl Pts',(-2.51617695364797,0.0816075237390802,
18.3823200932237));
#14734=CARTESIAN_POINT('Ctrl Pts',(-2.51886472713688,-0.00126367979163271,
18.3875778541503));
#14735=CARTESIAN_POINT('Ctrl Pts',(-2.51745798731002,-0.0843880754561358,
18.3928356150769));
#14736=CARTESIAN_POINT('Ctrl Pts',(-2.51193293504969,-0.167329554510471,
18.3980933760035));
#14737=CARTESIAN_POINT('Ctrl Pts',(-2.50638101469612,-0.250674374435956,
18.403376705197));
#14738=CARTESIAN_POINT('Ctrl Pts',(-2.49667055461409,-0.333834027997151,
18.4086600343905));
#14739=CARTESIAN_POINT('Ctrl Pts',(-2.48283047278443,-0.416364135598939,
18.413943363584));
#14740=CARTESIAN_POINT('Ctrl Pts',(-2.46908230145528,-0.498346169599006,
18.4191916067544));
#14741=CARTESIAN_POINT('Ctrl Pts',(-2.45125926710657,-0.579706534825325,
18.4244398499249));
#14742=CARTESIAN_POINT('Ctrl Pts',(-2.42944167002257,-0.660014713440488,
18.4296880930953));
#14743=CARTESIAN_POINT('Ctrl Pts',(-2.40763155202069,-0.740295362375832,
18.4349345371656));
#14744=CARTESIAN_POINT('Ctrl Pts',(-2.38182971157803,-0.81952409805105,
18.4401809812359));
#14745=CARTESIAN_POINT('Ctrl Pts',(-2.35216708556151,-0.897282704392028,
18.4454274253062));
#14746=CARTESIAN_POINT('Ctrl Pts',(-2.322505770802,-0.975037873359741,18.4506736374538));
#14747=CARTESIAN_POINT('Ctrl Pts',(-2.28898417448708,-1.05132261320712,
18.4559198496013));
#14748=CARTESIAN_POINT('Ctrl Pts',(-2.2517819549871,-1.12573721498157,18.4611660617489));
#14749=CARTESIAN_POINT('Ctrl Pts',(-2.21412313610845,-1.20106514024561,
18.4664766629905));
#14750=CARTESIAN_POINT('Ctrl Pts',(-2.17269292696622,-1.27447626811301,
18.471787264232));
#14751=CARTESIAN_POINT('Ctrl Pts',(-2.12772552152618,-1.34558179054495,
18.4770978654736));
#14752=CARTESIAN_POINT('Ctrl Pts',(-2.08324233497737,-1.41592163310507,
18.4823512809954));
#14753=CARTESIAN_POINT('Ctrl Pts',(-2.03529808117403,-1.48400493984633,
18.4876046965172));
#14754=CARTESIAN_POINT('Ctrl Pts',(-1.98416200106852,-1.54948617403182,
18.492858112039));
#14755=CARTESIAN_POINT('Ctrl Pts',(-1.93219096315314,-1.61603659591747,
18.4981973061404));
#14756=CARTESIAN_POINT('Ctrl Pts',(-1.87692325468778,-1.67989883468787,
18.5035365002418));
#14757=CARTESIAN_POINT('Ctrl Pts',(-1.81868142999892,-1.74074814553314,
18.5088756943432));
#14758=CARTESIAN_POINT('Ctrl Pts',(-1.76043960531006,-1.80159745637843,
18.5142148884447));
#14759=CARTESIAN_POINT('Ctrl Pts',(-1.69922406428985,-1.85943354653535,
18.5195540825461));
#14760=CARTESIAN_POINT('Ctrl Pts',(-1.63539194646763,-1.91397477293428,
18.5248932766475));
#14761=CARTESIAN_POINT('Ctrl Pts',(-1.5724748745046,-1.96773414021472,18.5301559323601));
#14762=CARTESIAN_POINT('Ctrl Pts',(-1.50679150832135,-2.01848415799354,
18.5354185880727));
#14763=CARTESIAN_POINT('Ctrl Pts',(-1.43866120240419,-2.06592840986733,
18.5406812437853));
#14764=CARTESIAN_POINT('Ctrl Pts',(-1.37062575312898,-2.11330660593302,
18.5459365723937));
#14765=CARTESIAN_POINT('Ctrl Pts',(-1.30015050609536,-2.15738791838507,
18.5511919010021));
#14766=CARTESIAN_POINT('Ctrl Pts',(-1.22758857361836,-2.19791549972278,
18.5564472296105));
#14767=CARTESIAN_POINT('Ctrl Pts',(-1.15463136774808,-2.23866385074027,
18.5617311860614));
#14768=CARTESIAN_POINT('Ctrl Pts',(-1.07956502959159,-2.27581932701635,
18.5670151425123));
#14769=CARTESIAN_POINT('Ctrl Pts',(-1.00277889174594,-2.30916451217075,
18.5722990989632));
#14770=CARTESIAN_POINT('Ctrl Pts',(-0.926541476321039,-2.34227140886279,
18.577545295664));
#14771=CARTESIAN_POINT('Ctrl Pts',(-0.848609189515541,-2.3716221112681,
18.5827914923648));
#14772=CARTESIAN_POINT('Ctrl Pts',(-0.769387001676135,-2.39705024804484,
18.5880376890656));
#14773=CARTESIAN_POINT('Ctrl Pts',(-0.690189743594728,-2.42247038305699,
18.5932822348852));
#14774=CARTESIAN_POINT('Ctrl Pts',(-0.609703828204644,-2.44397026379184,
18.5985267807049));
#14775=CARTESIAN_POINT('Ctrl Pts',(-0.528351380128789,-2.46143272691252,
18.6037713265246));
#14776=CARTESIAN_POINT('Ctrl Pts',(-0.447000207173294,-2.4788949163261,
18.6090157901411));
#14777=CARTESIAN_POINT('Ctrl Pts',(-0.364782978333853,-2.49231971854964,
18.6142602537577));
#14778=CARTESIAN_POINT('Ctrl Pts',(-0.282132717401159,-2.50164093741924,
18.6195047173742));
#14779=CARTESIAN_POINT('Ctrl Pts',(-0.198400428870973,-2.51108418634593,
18.624817839629));
#14780=CARTESIAN_POINT('Ctrl Pts',(-0.114224166418886,-2.51631555418445,
18.6301309618838));
#14781=CARTESIAN_POINT('Ctrl Pts',(-0.0300584464804562,-2.51732054768462,
18.6354440841385));
#14782=CARTESIAN_POINT('Ctrl Pts',(0.0531397919727716,-2.51831398882588,
18.6406961322718));
#14783=CARTESIAN_POINT('Ctrl Pts',(0.136327266117714,-2.51517779919644,
18.645948180405));
#14784=CARTESIAN_POINT('Ctrl Pts',(0.219067828737113,-2.50795046530278,
18.6512002285383));
#14785=CARTESIAN_POINT('Ctrl Pts',(0.303251630370289,-2.50059706542755,
18.6565438878538));
#14786=CARTESIAN_POINT('Ctrl Pts',(0.386972287484825,-2.48900850579982,
18.6618875471694));
#14787=CARTESIAN_POINT('Ctrl Pts',(0.469780780888515,-2.4732796582489,18.6672312064849));
#14788=CARTESIAN_POINT('Ctrl Pts',(0.552589274292217,-2.45755081069797,
18.6725748658005));
#14789=CARTESIAN_POINT('Ctrl Pts',(0.634485138727603,-2.43768185432414,
18.6779185251161));
#14790=CARTESIAN_POINT('Ctrl Pts',(0.715036925982957,-2.4138203007848,18.6832621844316));
#14791=CARTESIAN_POINT('Ctrl Pts',(0.793401155857259,-2.39060675915616,
18.6884607251623));
#14792=CARTESIAN_POINT('Ctrl Pts',(0.870796489168577,-2.36352475954149,
18.693659265893));
#14793=CARTESIAN_POINT('Ctrl Pts',(0.946807723733528,-2.33267258402857,
18.6988578066236));
#14794=CARTESIAN_POINT('Ctrl Pts',(1.02270947544916,-2.3018648464741,18.7040488596315));
#14795=CARTESIAN_POINT('Ctrl Pts',(1.0972306524512,-2.2672978882898,18.7092399126394));
#14796=CARTESIAN_POINT('Ctrl Pts',(1.16997007122369,-2.22912006909472,18.7144309656473));
#14797=CARTESIAN_POINT('Ctrl Pts',(1.24423617918151,-2.19014095584659,18.719730970921));
#14798=CARTESIAN_POINT('Ctrl Pts',(1.31664440076205,-2.14739780935237,18.7250309761947));
#14799=CARTESIAN_POINT('Ctrl Pts',(1.38678828785133,-2.1011007816567,18.7303309814684));
#14800=CARTESIAN_POINT('Ctrl Pts',(1.45536987689799,-2.05583491660041,18.7355129409906));
#14801=CARTESIAN_POINT('Ctrl Pts',(1.52178654142308,-2.00717212042383,18.7406949005128));
#14802=CARTESIAN_POINT('Ctrl Pts',(1.58568414928241,-1.95535470662346,18.745876860035));
#14803=CARTESIAN_POINT('Ctrl Pts',(1.64956311077339,-1.90355241399299,18.7510573073765));
#14804=CARTESIAN_POINT('Ctrl Pts',(1.71092410785923,-1.84859762784992,18.756237754718));
#14805=CARTESIAN_POINT('Ctrl Pts',(1.76944477290446,-1.79077397949632,18.7614182020596));
#14806=CARTESIAN_POINT('Ctrl Pts',(1.82796693099788,-1.73294885587763,18.7665987815708));
#14807=CARTESIAN_POINT('Ctrl Pts',(1.88364827803949,-1.67225505749713,18.771779361082));
#14808=CARTESIAN_POINT('Ctrl Pts',(1.93620323103858,-1.60901314417122,18.7769599405932));
#14809=CARTESIAN_POINT('Ctrl Pts',(1.99087519271403,-1.54322373205442,18.7823492032284));
#14810=CARTESIAN_POINT('Ctrl Pts',(2.04216318445828,-1.47467698774535,18.7877384658637));
#14811=CARTESIAN_POINT('Ctrl Pts',(2.08979333702531,-1.403769945014,18.7931277284989));
#14812=CARTESIAN_POINT('Ctrl Pts',(2.135656399308,-1.33549357087281,18.7983170481751));
#14813=CARTESIAN_POINT('Ctrl Pts',(2.17812806476868,-1.26502939632748,18.8035063678513));
#14814=CARTESIAN_POINT('Ctrl Pts',(2.21701030897764,-1.19275795528132,18.8086956875275));
#14815=CARTESIAN_POINT('Ctrl Pts',(2.25592432173553,-1.12042746520499,18.8138892471122));
#14816=CARTESIAN_POINT('Ctrl Pts',(2.29124288223879,-1.04628719853895,18.8190828066968));
#14817=CARTESIAN_POINT('Ctrl Pts',(2.32281609350656,-0.970737681223372,
18.8242763662815));
#14818=CARTESIAN_POINT('Ctrl Pts',(2.35444365066132,-0.895058123111655,
18.8294788653624));
#14819=CARTESIAN_POINT('Ctrl Pts',(2.38231285023912,-0.817964920789799,
18.8346813644433));
#14820=CARTESIAN_POINT('Ctrl Pts',(2.40632380071148,-0.739872972968649,
18.8398838635241));
#14821=CARTESIAN_POINT('Ctrl Pts',(2.4090117795033,-0.731130732639723,18.840466273088));
#14822=CARTESIAN_POINT('Ctrl Pts',(2.41165145841306,-0.722375984062057,
18.841048682652));
#14823=CARTESIAN_POINT('Ctrl Pts',(2.41424273752183,-0.713609314907739,
18.8416310922159));
#14824=CARTESIAN_POINT('Ctrl Pts',(2.44544639966121,-0.608042847191675,
18.848644351111));
#14825=CARTESIAN_POINT('Ctrl Pts',(2.46972564711354,-0.50041571271031,18.855657610006));
#14826=CARTESIAN_POINT('Ctrl Pts',(2.48687075747628,-0.391510007036009,
18.8626708689011));
#14827=CARTESIAN_POINT('Ctrl Pts',(2.50358555430506,-0.285337652042246,
18.8695081067526));
#14828=CARTESIAN_POINT('Ctrl Pts',(2.51351991815498,-0.177949699224724,
18.876345344604));
#14829=CARTESIAN_POINT('Ctrl Pts',(2.51652405256726,-0.0700923879638654,
18.8831825824554));
#14830=CARTESIAN_POINT('Ctrl Pts',(2.51714393432919,-0.0478367991762561,
18.88459339784));
#14831=CARTESIAN_POINT('Ctrl Pts',(2.51746889864049,-0.0255613129373036,
18.8860042132245));
#14832=CARTESIAN_POINT('Ctrl Pts',(2.51749787287094,-0.00327262742782446,
18.8874150286091));
#14833=CARTESIAN_POINT('Ctrl Pts',(2.5174977918681,-0.00333435739759424,
18.8883467778039));
#14834=CARTESIAN_POINT('Ctrl Pts',(2.51765838212971,0.117914081443941,18.8967380675264));
#14835=CARTESIAN_POINT('Ctrl Pts',(2.50905949712985,0.239027813720937,18.9050106031213));
#14836=CARTESIAN_POINT('Ctrl Pts',(2.4843513699158,0.410492998213102,18.916492485084));
#14837=CARTESIAN_POINT('Ctrl Pts',(2.4753494131927,0.461684008912046,18.9198922662718));
#14838=CARTESIAN_POINT('Ctrl Pts',(2.46095346766611,0.530910030959187,18.9244560997678));
#14839=CARTESIAN_POINT('Ctrl Pts',(2.45693322385993,0.549214523906593,18.9256596523586));
#14840=CARTESIAN_POINT('Ctrl Pts',(2.44967583322526,0.58058213555707,18.9277171463199));
#14841=CARTESIAN_POINT('Ctrl Pts',(2.44653768751871,0.593667127329751,18.9285739324056));
#14842=CARTESIAN_POINT('Ctrl Pts',(2.44005564336439,0.619770394269378,18.9302804135346));
#14843=CARTESIAN_POINT('Ctrl Pts',(2.43671210086245,0.632788299594441,18.9311300876594));
#14844=CARTESIAN_POINT('Ctrl Pts',(2.4298915001758,0.658487997445961,18.9328051096885));
#14845=CARTESIAN_POINT('Ctrl Pts',(2.42641901716019,0.671170550557235,18.9336305591408));
#14846=CARTESIAN_POINT('Ctrl Pts',(2.4177027392349,0.702053006102434,18.9356381287255));
#14847=CARTESIAN_POINT('Ctrl Pts',(2.41235257431326,0.720222217601793,18.9368171788481));
#14848=CARTESIAN_POINT('Ctrl Pts',(2.39320910069792,0.782625872440048,18.9408614814428));
#14849=CARTESIAN_POINT('Ctrl Pts',(2.37839963254998,0.826540131713007,18.9436981953647));
#14850=CARTESIAN_POINT('Ctrl Pts',(2.36206508692986,0.870893585294821,18.9465639241001));
#14851=CARTESIAN_POINT('Ctrl Pts',(2.3617437862239,0.871764532426716,18.9466201973601));
#14852=CARTESIAN_POINT('Ctrl Pts',(2.36142200732435,0.872635292275211,18.9466764589532));
#14853=CARTESIAN_POINT('',(2.51749995481779,0.000475351647371232,18.6124102744318));
#14854=CARTESIAN_POINT('Ctrl Pts',(2.36142200728635,0.872635292378032,18.6688222409353));
#14855=CARTESIAN_POINT('Ctrl Pts',(2.39182664777468,0.790357864682992,18.6632590496871));
#14856=CARTESIAN_POINT('Ctrl Pts',(2.41796845445713,0.706378112618749,18.6576958584389));
#14857=CARTESIAN_POINT('Ctrl Pts',(2.43966855119106,0.621147011849314,18.6521326671906));
#14858=CARTESIAN_POINT('Ctrl Pts',(2.46132648786374,0.53608150243519,18.6465802843958));
#14859=CARTESIAN_POINT('Ctrl Pts',(2.47855979566509,0.449769843114856,18.6410279016009));
#14860=CARTESIAN_POINT('Ctrl Pts',(2.49123848450133,0.362680387310241,18.6354755188061));
#14861=CARTESIAN_POINT('Ctrl Pts',(2.50388458458775,0.2758147824514,18.6299374076143));
#14862=CARTESIAN_POINT('Ctrl Pts',(2.51199933246258,0.188175732793444,18.6243992964224));
#14863=CARTESIAN_POINT('Ctrl Pts',(2.51550346002756,0.10024266850695,18.6188611852306));
#14864=CARTESIAN_POINT('Ctrl Pts',(2.51682752769016,0.0670163304993951,
18.6167685576635));
#14865=CARTESIAN_POINT('Ctrl Pts',(2.51749381825413,0.0337481357832397,
18.6146759300965));
#14866=CARTESIAN_POINT('Ctrl Pts',(2.51749995717886,0.000464332231146367,
18.6125833025294));
#14867=CARTESIAN_POINT('Ctrl Pts',(2.5174999250055,0.000614489468989278,
18.6102255169021));
#14868=CARTESIAN_POINT('Ctrl Pts',(2.51750215682766,-0.00852905554551879,
18.6096432037694));
#14869=CARTESIAN_POINT('Ctrl Pts',(2.51745457472059,-0.0176726609456453,
18.6090624523556));
#14870=CARTESIAN_POINT('Ctrl Pts',(2.51724081692323,-0.0377392730921901,
18.6077912985835));
#14871=CARTESIAN_POINT('Ctrl Pts',(2.51705335857769,-0.0486618879025092,
18.6071015767941));
#14872=CARTESIAN_POINT('Ctrl Pts',(2.51652321895366,-0.0710550350449813,
18.6056918967218));
#14873=CARTESIAN_POINT('Ctrl Pts',(2.51617319279684,-0.0825251503035088,
18.6049721848102));
#14874=CARTESIAN_POINT('Ctrl Pts',(2.51517505996313,-0.1092405163893,18.6033011595809));
#14875=CARTESIAN_POINT('Ctrl Pts',(2.51446674850497,-0.124483169890081,
18.6023517496857));
#14876=CARTESIAN_POINT('Ctrl Pts',(2.51179270181138,-0.172590805891551,
18.5993672322175));
#14877=CARTESIAN_POINT('Ctrl Pts',(2.50932080267067,-0.205424990720745,
18.5973479059267));
#14878=CARTESIAN_POINT('Ctrl Pts',(2.50294237901877,-0.272534459338966,
18.5932509609013));
#14879=CARTESIAN_POINT('Ctrl Pts',(2.49897407636564,-0.306796851110074,
18.5911755754704));
#14880=CARTESIAN_POINT('Ctrl Pts',(2.47388169562043,-0.49035655441772,18.5801220371626));
#14881=CARTESIAN_POINT('Ctrl Pts',(2.44008132633024,-0.637610747818397,
18.5715104264123));
#14882=CARTESIAN_POINT('Ctrl Pts',(2.34828874984688,-0.918914003074701,
18.554520694451));
#14883=CARTESIAN_POINT('Ctrl Pts',(2.29143671601587,-1.05269615862231,18.5461696239991));
#14884=CARTESIAN_POINT('Ctrl Pts',(2.21484386812655,-1.19691481828407,18.5360963819896));
#14885=CARTESIAN_POINT('Ctrl Pts',(2.20612073906994,-1.21291783819977,18.5349627942739));
#14886=CARTESIAN_POINT('Ctrl Pts',(2.19309766363557,-1.23620402197328,18.5332879029808));
#14887=CARTESIAN_POINT('Ctrl Pts',(2.18893332199568,-1.24356288667622,18.5327548497083));
#14888=CARTESIAN_POINT('Ctrl Pts',(2.18150138742202,-1.25654296434937,18.5318076962865));
#14889=CARTESIAN_POINT('Ctrl Pts',(2.17824898891568,-1.2621726763102,18.5313945655384));
#14890=CARTESIAN_POINT('Ctrl Pts',(2.17115908911866,-1.27433585449356,18.5304968911937));
#14891=CARTESIAN_POINT('Ctrl Pts',(2.16731392855611,-1.28086454857782,18.5300118764737));
#14892=CARTESIAN_POINT('Ctrl Pts',(2.15663661342312,-1.29880781465307,18.5286703027629));
#14893=CARTESIAN_POINT('Ctrl Pts',(2.14974347720989,-1.3101855539294,18.5278100006524));
#14894=CARTESIAN_POINT('Ctrl Pts',(2.11236129470614,-1.37079894464956,18.5231773356763));
#14895=CARTESIAN_POINT('Ctrl Pts',(2.08027262538127,-1.41902242933382,18.5193157565869));
#14896=CARTESIAN_POINT('Ctrl Pts',(1.96135817837331,-1.58501790711836,18.5055018677823));
#14897=CARTESIAN_POINT('Ctrl Pts',(1.86596150603354,-1.69628845843337,18.4952931815981));
#14898=CARTESIAN_POINT('Ctrl Pts',(1.65596353148766,-1.90194316928332,18.4751138802844));
#14899=CARTESIAN_POINT('Ctrl Pts',(1.54158667528325,-1.99577722167655,18.46518817903));
#14900=CARTESIAN_POINT('Ctrl Pts',(1.3994938472954,-2.09280133522046,18.4540948901075));
#14901=CARTESIAN_POINT('Ctrl Pts',(1.37916369961352,-2.10625449912207,18.4525341443093));
#14902=CARTESIAN_POINT('Ctrl Pts',(1.34737181736315,-2.12663457366111,18.4501333128665));
#14903=CARTESIAN_POINT('Ctrl Pts',(1.33604526466212,-2.13376861119355,18.4492856397384));
#14904=CARTESIAN_POINT('Ctrl Pts',(1.31497877597158,-2.14680384247007,18.4477229673254));
#14905=CARTESIAN_POINT('Ctrl Pts',(1.30525471416179,-2.15272990811629,18.4470070751909));
#14906=CARTESIAN_POINT('Ctrl Pts',(1.28389210564039,-2.165550805658,18.4454459824142));
#14907=CARTESIAN_POINT('Ctrl Pts',(1.27223747322,-2.17241825020526,18.4446017842655));
#14908=CARTESIAN_POINT('Ctrl Pts',(1.23958226989907,-2.19130727091362,18.4422567395579));
#14909=CARTESIAN_POINT('Ctrl Pts',(1.21846254718342,-2.20312070543127,18.4407633018467));
#14910=CARTESIAN_POINT('Ctrl Pts',(1.05574709208051,-2.291080804161,18.4294252073927));
#14911=CARTESIAN_POINT('Ctrl Pts',(0.907314559160761,-2.35381450550131,
18.4200773793681));
#14912=CARTESIAN_POINT('Ctrl Pts',(0.63631902210136,-2.43887071743909,18.4037250874671));
#14913=CARTESIAN_POINT('Ctrl Pts',(0.516198619736816,-2.46708894810063,
18.3966955322491));
#14914=CARTESIAN_POINT('Ctrl Pts',(0.351086272340018,-2.49328641539471,
18.3868073814731));
#14915=CARTESIAN_POINT('Ctrl Pts',(0.307498870734705,-2.49903636165727,
18.3841752962588));
#14916=CARTESIAN_POINT('Ctrl Pts',(0.235944972828393,-2.50657534043136,
18.3797870180712));
#14917=CARTESIAN_POINT('Ctrl Pts',(0.208058453146061,-2.50904394094888,
18.3780601133164));
#14918=CARTESIAN_POINT('Ctrl Pts',(0.170066351849919,-2.51176942506044,
18.3756777559617));
#14919=CARTESIAN_POINT('Ctrl Pts',(0.15999071874977,-2.51243132652685,18.3750431142095));
#14920=CARTESIAN_POINT('Ctrl Pts',(0.143108231205909,-2.51343842860559,
18.3739745751576));
#14921=CARTESIAN_POINT('Ctrl Pts',(0.136303352677024,-2.51381663887619,
18.3735424756562));
#14922=CARTESIAN_POINT('Ctrl Pts',(0.123379379834958,-2.51448231342796,
18.3727190237121));
#14923=CARTESIAN_POINT('Ctrl Pts',(0.117260598476626,-2.51477508458086,
18.3723279758135));
#14924=CARTESIAN_POINT('Ctrl Pts',(0.102699251475504,-2.51541855645151,
18.3713946362235));
#14925=CARTESIAN_POINT('Ctrl Pts',(0.0942559322292057,-2.51574908621491,
18.3708512598506));
#14926=CARTESIAN_POINT('Ctrl Pts',(0.0643087139798407,-2.51677045761506,
18.3689166154294));
#14927=CARTESIAN_POINT('Ctrl Pts',(0.0427984857373781,-2.51722811127943,
18.3675135515741));
#14928=CARTESIAN_POINT('Ctrl Pts',(-0.106888217363795,-2.51849378338224,
18.3576681227493));
#14929=CARTESIAN_POINT('Ctrl Pts',(-0.234946055302919,-2.5097868758584,
18.3488381640748));
#14930=CARTESIAN_POINT('Ctrl Pts',(-0.503575502989314,-2.47077936348239,
18.3300900861767));
#14931=CARTESIAN_POINT('Ctrl Pts',(-0.643378209288076,-2.43811636455717,
18.3202072137338));
#14932=CARTESIAN_POINT('Ctrl Pts',(-0.849548430825008,-2.37096551133567,
18.3057367769633));
#14933=CARTESIAN_POINT('Ctrl Pts',(-0.918419064808094,-2.34514780102968,
18.3009172323515));
#14934=CARTESIAN_POINT('Ctrl Pts',(-1.00494494794857,-2.30831385722584,
18.2948785592409));
#14935=CARTESIAN_POINT('Ctrl Pts',(-1.02372444467275,-2.30004685037655,
18.2935688292029));
#14936=CARTESIAN_POINT('Ctrl Pts',(-1.0539941776916,-2.28627748301375,18.2914587031916));
#14937=CARTESIAN_POINT('Ctrl Pts',(-1.06554709736118,-2.28091601093088,
18.290653568122));
#14938=CARTESIAN_POINT('Ctrl Pts',(-1.0876582576966,-2.27045001681488,18.2891128712107));
#14939=CARTESIAN_POINT('Ctrl Pts',(-1.09822246495921,-2.26535895374548,
18.2883768732966));
#14940=CARTESIAN_POINT('Ctrl Pts',(-1.12234339922585,-2.25352629498757,
18.2866964456641));
#14941=CARTESIAN_POINT('Ctrl Pts',(-1.13587573993024,-2.24673580716248,
18.2857537318026));
#14942=CARTESIAN_POINT('Ctrl Pts',(-1.1787994319751,-2.22470988276268,18.2827629298786));
#14943=CARTESIAN_POINT('Ctrl Pts',(-1.20795263313733,-2.20901624153878,
18.2807308004649));
#14944=CARTESIAN_POINT('Ctrl Pts',(-1.38669512353555,-2.10819919986852,
18.2682485152041));
#14945=CARTESIAN_POINT('Ctrl Pts',(-1.52754018283228,-2.00849614696838,
18.2583523836813));
#14946=CARTESIAN_POINT('Ctrl Pts',(-1.73133497450843,-1.83030151883563,
18.2427990255119));
#14947=CARTESIAN_POINT('Ctrl Pts',(-1.8016680470265,-1.76111177525823,18.2371410928996));
#14948=CARTESIAN_POINT('Ctrl Pts',(-1.89796815155397,-1.65455522497619,
18.2286576468602));
#14949=CARTESIAN_POINT('Ctrl Pts',(-1.92727228067405,-1.62032626177155,
18.2259632270064));
#14950=CARTESIAN_POINT('Ctrl Pts',(-1.97357354142685,-1.56320974065637,
18.221481791625));
#14951=CARTESIAN_POINT('Ctrl Pts',(-1.99112899057248,-1.54078629321933,
18.2197259042988));
#14952=CARTESIAN_POINT('Ctrl Pts',(-2.01441083786353,-1.50998607333527,
18.2173113740732));
#14953=CARTESIAN_POINT('Ctrl Pts',(-2.02047323228907,-1.50186446617077,
18.2166744459023));
#14954=CARTESIAN_POINT('Ctrl Pts',(-2.03052157048186,-1.48823205725804,
18.2156045152353));
#14955=CARTESIAN_POINT('Ctrl Pts',(-2.03453459191065,-1.48274121026991,
18.2151733485443));
#14956=CARTESIAN_POINT('Ctrl Pts',(-2.04210065786843,-1.47230033616332,
18.2143529248706));
#14957=CARTESIAN_POINT('Ctrl Pts',(-2.04565807661919,-1.46735353899278,
18.2139639825756));
#14958=CARTESIAN_POINT('Ctrl Pts',(-2.05499196665383,-1.45427431102632,
18.2129351218001));
#14959=CARTESIAN_POINT('Ctrl Pts',(-2.06073805160998,-1.44612047541567,
18.2122931984065));
#14960=CARTESIAN_POINT('Ctrl Pts',(-2.08090968685881,-1.41713206975643,
18.2100098541999));
#14961=CARTESIAN_POINT('Ctrl Pts',(-2.09506842391018,-1.39611482742013,
18.2083522321623));
#14962=CARTESIAN_POINT('Ctrl Pts',(-2.20280946246587,-1.23085355228727,
18.1953233523252));
#14963=CARTESIAN_POINT('Ctrl Pts',(-2.28170313318702,-1.07758730895573,
18.183305322428));
#14964=CARTESIAN_POINT('Ctrl Pts',(-2.40096807913243,-0.772842550326007,
18.16077654559));
#14965=CARTESIAN_POINT('Ctrl Pts',(-2.44407672341112,-0.623247284441368,
18.1502789325224));
#14966=CARTESIAN_POINT('Ctrl Pts',(-2.47830648694301,-0.44336480746625,
18.1384347767445));
#14967=CARTESIAN_POINT('Ctrl Pts',(-2.48304045724959,-0.41603555603686,
18.1366549545893));
#14968=CARTESIAN_POINT('Ctrl Pts',(-2.48952296639736,-0.374546288205229,
18.1339816503384));
#14969=CARTESIAN_POINT('Ctrl Pts',(-2.49160424266433,-0.360441165509516,
18.1330777936971));
#14970=CARTESIAN_POINT('Ctrl Pts',(-2.49516000834397,-0.334838937390025,
18.1314460033085));
#14971=CARTESIAN_POINT('Ctrl Pts',(-2.49667512519751,-0.323347966905891,
18.1307168153441));
#14972=CARTESIAN_POINT('Ctrl Pts',(-2.49976791433957,-0.298572562846173,
18.1291513500969));
#14973=CARTESIAN_POINT('Ctrl Pts',(-2.50131917156891,-0.285285144660354,
18.1283159196029));
#14974=CARTESIAN_POINT('Ctrl Pts',(-2.50523947138852,-0.249211248167154,
18.1260586744285));
#14975=CARTESIAN_POINT('Ctrl Pts',(-2.50740355604969,-0.226403435474002,
18.124643263406));
#14976=CARTESIAN_POINT('Ctrl Pts',(-2.51727053576669,-0.104779714195217,
18.1171533110186));
#14977=CARTESIAN_POINT('Ctrl Pts',(-2.51944471725618,-0.00559727014803007,
18.1112529460383));
#14978=CARTESIAN_POINT('Ctrl Pts',(-2.50951361894324,0.261716261458144,
18.0956166396101));
#14979=CARTESIAN_POINT('Ctrl Pts',(-2.48640071093977,0.428908180040172,
18.0861402634124));
#14980=CARTESIAN_POINT('Ctrl Pts',(-2.4332504101922,0.648382920894336,18.0729323896871));
#14981=CARTESIAN_POINT('Ctrl Pts',(-2.41781887649505,0.703746411155615,
18.0695291981744));
#14982=CARTESIAN_POINT('Ctrl Pts',(-2.39365247952273,0.780225453935727,
18.0646673341947));
#14983=CARTESIAN_POINT('Ctrl Pts',(-2.38650335343618,0.801826428148148,
18.0632758613125));
#14984=CARTESIAN_POINT('Ctrl Pts',(-2.37348422768559,0.839446142002436,
18.0608155720463));
#14985=CARTESIAN_POINT('Ctrl Pts',(-2.36774225033013,0.855507921418181,
18.0597532270337));
#14986=CARTESIAN_POINT('Ctrl Pts',(-2.35897550264946,0.879266277089992,
18.0581623230088));
#14987=CARTESIAN_POINT('Ctrl Pts',(-2.35607517117383,0.887008676011476,
18.0576407800213));
#14988=CARTESIAN_POINT('Ctrl Pts',(-2.35104486999594,0.900238254329221,
18.0567440697138));
#14989=CARTESIAN_POINT('Ctrl Pts',(-2.34893371664179,0.905732459996498,
18.0563700177828));
#14990=CARTESIAN_POINT('Ctrl Pts',(-2.34408774918382,0.918213025561536,
18.0555165174362));
#14991=CARTESIAN_POINT('Ctrl Pts',(-2.3413410133645,0.925194461628468,18.0550363783652));
#14992=CARTESIAN_POINT('Ctrl Pts',(-2.33375633283213,0.944222514339445,
18.0537205576419));
#14993=CARTESIAN_POINT('Ctrl Pts',(-2.32885642554597,0.956243959366076,
18.0528813549417));
#14994=CARTESIAN_POINT('Ctrl Pts',(-2.30336102467174,1.01743607856899,18.0485710949978));
#14995=CARTESIAN_POINT('Ctrl Pts',(-2.28130184340732,1.0659780358445,18.0450245042719));
#14996=CARTESIAN_POINT('Ctrl Pts',(-2.16229088158447,1.307222895608,18.0268732345917));
#14997=CARTESIAN_POINT('Ctrl Pts',(-2.04239454666965,1.4876065921646,18.0116674768687));
#14998=CARTESIAN_POINT('Ctrl Pts',(-1.86275853591999,1.69450022495305,17.9932464886632));
#14999=CARTESIAN_POINT('Ctrl Pts',(-1.82304533522172,1.73715483612866,17.989379074569));
#15000=CARTESIAN_POINT('Ctrl Pts',(-1.75321018681335,1.80712701078356,17.9829169698991));
#15001=CARTESIAN_POINT('Ctrl Pts',(-1.72384321403486,1.83516181250431,17.9802928554026));
#15002=CARTESIAN_POINT('Ctrl Pts',(-1.68154310476118,1.87363122150665,17.9766394603273));
#15003=CARTESIAN_POINT('Ctrl Pts',(-1.66916641951126,1.88466566074717,17.9755851193295));
#15004=CARTESIAN_POINT('Ctrl Pts',(-1.64770536912818,1.90342201726563,17.97378148613));
#15005=CARTESIAN_POINT('Ctrl Pts',(-1.63867363253257,1.91120304866168,17.973029766383));
#15006=CARTESIAN_POINT('Ctrl Pts',(-1.6213032622306,1.92595433096631,17.9715977739447));
#15007=CARTESIAN_POINT('Ctrl Pts',(-1.61297411930702,1.93293529365318,17.9709170746223));
#15008=CARTESIAN_POINT('Ctrl Pts',(-1.59333973553138,1.94917630856568,17.9693261455656));
#15009=CARTESIAN_POINT('Ctrl Pts',(-1.58199847862048,1.95839235661377,17.9684176916708));
#15010=CARTESIAN_POINT('Ctrl Pts',(-1.54824618255078,1.98533535237214,17.9657442862546));
#15011=CARTESIAN_POINT('Ctrl Pts',(-1.52561241840828,2.00278045533442,17.9639903776879));
#15012=CARTESIAN_POINT('Ctrl Pts',(-1.3448027711089,2.13729630868681,17.9502668259166));
#15013=CARTESIAN_POINT('Ctrl Pts',(-1.17369340217554,2.23584047429716,17.9390565443938));
#15014=CARTESIAN_POINT('Ctrl Pts',(-0.868694022597619,2.36673347575912,
17.9199538483269));
#15015=CARTESIAN_POINT('Ctrl Pts',(-0.740478007227817,2.40992517383426,
17.9121320784809));
#15016=CARTESIAN_POINT('Ctrl Pts',(-0.59195237903389,2.44698250183437,17.9026836557075));
#15017=CARTESIAN_POINT('Ctrl Pts',(-0.57442225536348,2.45115687235571,17.9015624038222));
#15018=CARTESIAN_POINT('Ctrl Pts',(-0.548597167432117,2.45701424511822,
17.89989966211));
#15019=CARTESIAN_POINT('Ctrl Pts',(-0.54033567518004,2.45884428259756,17.8993661115137));
#15020=CARTESIAN_POINT('Ctrl Pts',(-0.525682492459146,2.46201275618266,
17.8984166181944));
#15021=CARTESIAN_POINT('Ctrl Pts',(-0.519294610278079,2.46336801978397,
17.898001630626));
#15022=CARTESIAN_POINT('Ctrl Pts',(-0.505433697216426,2.46625246260113,
17.897098779707));
#15023=CARTESIAN_POINT('Ctrl Pts',(-0.497959087383205,2.46777251285386,
17.8966104371215));
#15024=CARTESIAN_POINT('Ctrl Pts',(-0.477206012533261,2.47189477157104,
17.8952507019427));
#15025=CARTESIAN_POINT('Ctrl Pts',(-0.463913527443257,2.47442388446784,
17.8943754034019));
#15026=CARTESIAN_POINT('Ctrl Pts',(-0.390016087292666,2.48786772124458,
17.8894874567727));
#15027=CARTESIAN_POINT('Ctrl Pts',(-0.329051614929678,2.49666218118155,
17.8853738880233));
#15028=CARTESIAN_POINT('Ctrl Pts',(-0.0907274039402323,2.52216174314133,
17.8691277088495));
#15029=CARTESIAN_POINT('Ctrl Pts',(0.0878890297624799,2.52226318313915,
17.8566408237309));
#15030=CARTESIAN_POINT('Ctrl Pts',(0.37784878674303,2.49156733109126,17.8368264141302));
#15031=CARTESIAN_POINT('Ctrl Pts',(0.489745303522463,2.47200996762349,17.8292830768543));
#15032=CARTESIAN_POINT('Ctrl Pts',(0.622430834440168,2.43945110547026,17.820485205456));
#15033=CARTESIAN_POINT('Ctrl Pts',(0.644830326647705,2.43362604931074,17.81900476532));
#15034=CARTESIAN_POINT('Ctrl Pts',(0.679975037906846,2.42396724141288,17.8166888698142));
#15035=CARTESIAN_POINT('Ctrl Pts',(0.692775186326517,2.42034001575675,17.8158468428201));
#15036=CARTESIAN_POINT('Ctrl Pts',(0.716690810139699,2.41335768634948,17.8142761340494));
#15037=CARTESIAN_POINT('Ctrl Pts',(0.727812942920345,2.41002683947314,17.8135466926743));
#15038=CARTESIAN_POINT('Ctrl Pts',(0.752667534497244,2.40239565658569,17.8119187306687));
#15039=CARTESIAN_POINT('Ctrl Pts',(0.766387037348629,2.39805425936081,17.8110215675678));
#15040=CARTESIAN_POINT('Ctrl Pts',(0.801213112165103,2.38670449902357,17.8087474211037));
#15041=CARTESIAN_POINT('Ctrl Pts',(0.822265691116809,2.3795335673898,17.8073757456373));
#15042=CARTESIAN_POINT('Ctrl Pts',(0.995633971855635,2.31790516357311,17.796098633377));
#15043=CARTESIAN_POINT('Ctrl Pts',(1.14247782094492,2.24916100652835,17.786700276714));
#15044=CARTESIAN_POINT('Ctrl Pts',(1.38842169511592,2.10367748891348,17.7702622177524));
#15045=CARTESIAN_POINT('Ctrl Pts',(1.49030434171812,2.03277231051378,17.7631969895323));
#15046=CARTESIAN_POINT('Ctrl Pts',(1.62060746778923,1.92700867776693,17.7532734308492));
#15047=CARTESIAN_POINT('Ctrl Pts',(1.65394055401943,1.89847602683982,17.7506470757152));
#15048=CARTESIAN_POINT('Ctrl Pts',(1.70725102104016,1.85037312391305,17.746268079972));
#15049=CARTESIAN_POINT('Ctrl Pts',(1.72767883130065,1.83131440570978,17.7445448003496));
#15050=CARTESIAN_POINT('Ctrl Pts',(1.75502617637599,1.80493507186594,17.7421682616341));
#15051=CARTESIAN_POINT('Ctrl Pts',(1.762225996684,1.797906288429,17.7415358440357));
#15052=CARTESIAN_POINT('Ctrl Pts',(1.77421124589107,1.78606460329909,17.7404713325206));
#15053=CARTESIAN_POINT('Ctrl Pts',(1.77901978727859,1.78127507893163,17.7400410328778));
#15054=CARTESIAN_POINT('Ctrl Pts',(1.78812124143953,1.77213600586748,17.7392203078144));
#15055=CARTESIAN_POINT('Ctrl Pts',(1.79241778971287,1.76779016361785,17.7388301856064));
#15056=CARTESIAN_POINT('Ctrl Pts',(1.80259739227062,1.75741850810234,17.737899587598));
#15057=CARTESIAN_POINT('Ctrl Pts',(1.80846607340502,1.75137877907153,17.7373580349747));
#15058=CARTESIAN_POINT('Ctrl Pts',(1.829143066152,1.7298843972971,17.7354323911853));
#15059=CARTESIAN_POINT('Ctrl Pts',(1.843783994868,1.71427095094739,17.7340366112429));
#15060=CARTESIAN_POINT('Ctrl Pts',(1.95060687708032,1.59740082862512,17.72362332876));
#15061=CARTESIAN_POINT('Ctrl Pts',(2.03458155198715,1.48896864539858,17.7141630399245));
#15062=CARTESIAN_POINT('Ctrl Pts',(2.18154057222212,1.26340494733854,17.6955637949297));
#15063=CARTESIAN_POINT('Ctrl Pts',(2.24491992639096,1.14701884207999,17.6864546519252));
#15064=CARTESIAN_POINT('Ctrl Pts',(2.3213954756214,0.975697529016985,17.6739183267136));
#15065=CARTESIAN_POINT('Ctrl Pts',(2.3422604104862,0.924488129415224,17.6702722055998));
#15066=CARTESIAN_POINT('Ctrl Pts',(2.36142200245778,0.872635305444532,17.6666805052528));
#15067=CARTESIAN_POINT('Origin',(0.,0.,10.));
#15068=CARTESIAN_POINT('',(2.36142200368728,0.872635302117405,16.6687517122259));
#15069=CARTESIAN_POINT('',(2.36142200728636,0.872635292378013,16.9437682627171));
#15070=CARTESIAN_POINT('',(2.36142200728636,0.87263529237802,10.));
#15071=CARTESIAN_POINT('',(2.5174999670525,0.000407296750592275,17.8874166974728));
#15072=CARTESIAN_POINT('Ctrl Pts',(2.36142200728636,0.872635292378013,16.9437682627171));
#15073=CARTESIAN_POINT('Ctrl Pts',(2.33277467475577,0.950157301949081,16.9490221933786));
#15074=CARTESIAN_POINT('Ctrl Pts',(2.30025475204426,1.02640554539073,16.9542761240401));
#15075=CARTESIAN_POINT('Ctrl Pts',(2.26399624137994,1.10096651584755,16.9595300547015));
#15076=CARTESIAN_POINT('Ctrl Pts',(2.22778717431102,1.17542581190054,16.9647768208872));
#15077=CARTESIAN_POINT('Ctrl Pts',(2.18784984627795,1.2482019935627,16.9700235870729));
#15078=CARTESIAN_POINT('Ctrl Pts',(2.14436702227656,1.31889966402785,16.9752703532586));
#15079=CARTESIAN_POINT('Ctrl Pts',(2.10093090803895,1.38952139021929,16.980511483306));
#15080=CARTESIAN_POINT('Ctrl Pts',(2.0539571081917,1.45806865172029,16.9857526133534));
#15081=CARTESIAN_POINT('Ctrl Pts',(2.00367452828408,1.52417014624535,16.9909937434007));
#15082=CARTESIAN_POINT('Ctrl Pts',(1.95342131699091,1.59023303278111,16.9962318122542));
#15083=CARTESIAN_POINT('Ctrl Pts',(1.89986344117179,1.65385262204952,17.0014698811077));
#15084=CARTESIAN_POINT('Ctrl Pts',(1.84327274321826,1.71468709801778,17.0067079499612));
#15085=CARTESIAN_POINT('Ctrl Pts',(1.78669802791096,1.77550439278942,17.0119445394513));
#15086=CARTESIAN_POINT('Ctrl Pts',(1.72709250588652,1.83353779898866,17.0171811289415));
#15087=CARTESIAN_POINT('Ctrl Pts',(1.66476695867383,1.88848013579913,17.0224177184317));
#15088=CARTESIAN_POINT('Ctrl Pts',(1.60244021392815,1.9434235282804,17.0276544085385));
#15089=CARTESIAN_POINT('Ctrl Pts',(1.53739368726397,1.9952754293427,17.0328910986454));
#15090=CARTESIAN_POINT('Ctrl Pts',(1.46997247333479,2.04376788741726,17.0381277887522));
#15091=CARTESIAN_POINT('Ctrl Pts',(1.40248354220258,2.09230905083896,17.043369738539));
#15092=CARTESIAN_POINT('Ctrl Pts',(1.33261553516941,2.13748376155191,17.0486116883258));
#15093=CARTESIAN_POINT('Ctrl Pts',(1.26074345964852,2.1790668137883,17.0538536381126));
#15094=CARTESIAN_POINT('Ctrl Pts',(1.18883594453469,2.22067037032254,17.0590981726663));
#15095=CARTESIAN_POINT('Ctrl Pts',(1.11492280324316,2.25867852924783,17.0643427072201));
#15096=CARTESIAN_POINT('Ctrl Pts',(1.03940244297438,2.29291273526467,17.0695872417738));
#15097=CARTESIAN_POINT('Ctrl Pts',(0.963748038937281,2.32720770478903,17.0748410850381));
#15098=CARTESIAN_POINT('Ctrl Pts',(0.886481146144829,2.35771516755753,17.0800949283025));
#15099=CARTESIAN_POINT('Ctrl Pts',(0.808018755863324,2.38430533702651,17.0853487715668));
#15100=CARTESIAN_POINT('Ctrl Pts',(0.737208666948436,2.40830221320636,17.0900902165744));
#15101=CARTESIAN_POINT('Ctrl Pts',(0.665425344416089,2.42910922742866,17.0948316615821));
#15102=CARTESIAN_POINT('Ctrl Pts',(0.592982195154382,2.44666678692255,17.0995731065898));
#15103=CARTESIAN_POINT('Ctrl Pts',(0.512687973536151,2.46612715808869,17.1048284087145));
#15104=CARTESIAN_POINT('Ctrl Pts',(0.431286506734991,2.48166665495804,17.1100837108393));
#15105=CARTESIAN_POINT('Ctrl Pts',(0.349195168056678,2.49316445197782,17.115339012964));
#15106=CARTESIAN_POINT('Ctrl Pts',(0.267220209607418,2.50464594866346,17.1205868646893));
#15107=CARTESIAN_POINT('Ctrl Pts',(0.18455777506545,2.5120970632641,17.1258347164146));
#15108=CARTESIAN_POINT('Ctrl Pts',(0.101637619020051,2.51544748392805,17.1310825681398));
#15109=CARTESIAN_POINT('Ctrl Pts',(0.0181176884826902,2.51882213871006,
17.1363683783996));
#15110=CARTESIAN_POINT('Ctrl Pts',(-0.0656632470085882,2.51803641614374,
17.1416541886594));
#15111=CARTESIAN_POINT('Ctrl Pts',(-0.149258427858184,2.51307146172036,
17.1469399989191));
#15112=CARTESIAN_POINT('Ctrl Pts',(-0.232105070298294,2.50815096511201,
17.1521784783164));
#15113=CARTESIAN_POINT('Ctrl Pts',(-0.314768802335826,2.49912580955793,
17.1574169577138));
#15114=CARTESIAN_POINT('Ctrl Pts',(-0.39681426657695,2.48602990485654,17.1626554371111));
#15115=CARTESIAN_POINT('Ctrl Pts',(-0.4788327485456,2.47293830700224,17.1678921937309));
#15116=CARTESIAN_POINT('Ctrl Pts',(-0.560232911258984,2.45577869149736,
17.1731289503508));
#15117=CARTESIAN_POINT('Ctrl Pts',(-0.640586253136465,2.43463662633515,
17.1783657069706));
#15118=CARTESIAN_POINT('Ctrl Pts',(-0.720937405960774,2.41349513714282,
17.1836023209264));
#15119=CARTESIAN_POINT('Ctrl Pts',(-0.800241348690656,2.38837153241022,
17.1888389348821));
#15120=CARTESIAN_POINT('Ctrl Pts',(-0.878082833579531,2.35940178591374,
17.1940755488378));
#15121=CARTESIAN_POINT('Ctrl Pts',(-0.957196623425065,2.32995853416343,
17.1993977542992));
#15122=CARTESIAN_POINT('Ctrl Pts',(-1.03479925207399,2.29654243797504,17.2047199597605));
#15123=CARTESIAN_POINT('Ctrl Pts',(-1.11047572288176,2.25934723291712,17.2100421652219));
#15124=CARTESIAN_POINT('Ctrl Pts',(-1.18504209113089,2.22269764648891,17.2152862989413));
#15125=CARTESIAN_POINT('Ctrl Pts',(-1.25773805734807,2.18237936896989,17.2205304326607));
#15126=CARTESIAN_POINT('Ctrl Pts',(-1.32819293953474,2.13862333414981,17.2257745663801));
#15127=CARTESIAN_POINT('Ctrl Pts',(-1.40022116128764,2.09389017611688,17.2311358077125));
#15128=CARTESIAN_POINT('Ctrl Pts',(-1.46990658020088,2.04556416416079,17.2364970490448));
#15129=CARTESIAN_POINT('Ctrl Pts',(-1.5368875120115,1.99393656504491,17.2418582903771));
#15130=CARTESIAN_POINT('Ctrl Pts',(-1.60386844382214,1.94230896592902,17.2472195317095));
#15131=CARTESIAN_POINT('Ctrl Pts',(-1.6681445457099,1.8873801604566,17.2525807730418));
#15132=CARTESIAN_POINT('Ctrl Pts',(-1.72939442071244,1.8294811252398,17.2579420143741));
#15133=CARTESIAN_POINT('Ctrl Pts',(-1.78943161985282,1.77272842317791,17.2631971094008));
#15134=CARTESIAN_POINT('Ctrl Pts',(-1.84678312947741,1.71291243033947,17.2684522044274));
#15135=CARTESIAN_POINT('Ctrl Pts',(-1.90112037151567,1.65031741886466,17.2737072994541));
#15136=CARTESIAN_POINT('Ctrl Pts',(-1.95538057174684,1.58781115743711,17.2789549435686));
#15137=CARTESIAN_POINT('Ctrl Pts',(-2.00663469334919,1.52253404934597,17.284202587683));
#15138=CARTESIAN_POINT('Ctrl Pts',(-2.05458978583795,1.45480825607032,17.2894502317975));
#15139=CARTESIAN_POINT('Ctrl Pts',(-2.1028941297072,1.38658922369182,17.2947360938959));
#15140=CARTESIAN_POINT('Ctrl Pts',(-2.14785084336907,1.31588601347509,17.3000219559943));
#15141=CARTESIAN_POINT('Ctrl Pts',(-2.18920084141125,1.2430631222767,17.3053078180926));
#15142=CARTESIAN_POINT('Ctrl Pts',(-2.23017855419591,1.17089587533675,17.3105460901396));
#15143=CARTESIAN_POINT('Ctrl Pts',(-2.26761400262287,1.0966473707698,17.3157843621865));
#15144=CARTESIAN_POINT('Ctrl Pts',(-2.30129860612775,1.02070121751396,17.3210226342335));
#15145=CARTESIAN_POINT('Ctrl Pts',(-2.33497213490514,0.944780033616912,
17.3262591840564));
#15146=CARTESIAN_POINT('Ctrl Pts',(-2.36489708099854,0.867162731030279,
17.3314957338792));
#15147=CARTESIAN_POINT('Ctrl Pts',(-2.39091192672311,0.788255294085104,
17.3367322837021));
#15148=CARTESIAN_POINT('Ctrl Pts',(-2.41692606781552,0.709349994408706,
17.341968691689));
#15149=CARTESIAN_POINT('Ctrl Pts',(-2.43903017560629,0.629155068422387,
17.3472050996759));
#15150=CARTESIAN_POINT('Ctrl Pts',(-2.45711222843626,0.548092826872433,
17.3524415076628));
#15151=CARTESIAN_POINT('Ctrl Pts',(-2.47549140060318,0.465698592783337,
17.3577639588707));
#15152=CARTESIAN_POINT('Ctrl Pts',(-2.48971502236485,0.382408759267712,
17.3630864100787));
#15153=CARTESIAN_POINT('Ctrl Pts',(-2.49971964547033,0.298676989488158,
17.3684088612866));
#15154=CARTESIAN_POINT('Ctrl Pts',(-2.50957667561334,0.21618047063444,17.3736527931608));
#15155=CARTESIAN_POINT('Ctrl Pts',(-2.51533838730665,0.133255439081672,
17.3788967250349));
#15156=CARTESIAN_POINT('Ctrl Pts',(-2.51699667917541,0.0503385242130254,
17.384140656909));
#15157=CARTESIAN_POINT('Ctrl Pts',(-2.51869221637152,-0.0344407091621792,
17.3895023677839));
#15158=CARTESIAN_POINT('Ctrl Pts',(-2.51609779009976,-0.119210944760911,
17.3948640786588));
#15159=CARTESIAN_POINT('Ctrl Pts',(-2.5092608266804,-0.203510082519756,
17.4002257895336));
#15160=CARTESIAN_POINT('Ctrl Pts',(-2.50242386326104,-0.287809220278612,
17.4055875004085));
#15161=CARTESIAN_POINT('Ctrl Pts',(-2.4913444955995,-0.371636764972206,
17.4109492112834));
#15162=CARTESIAN_POINT('Ctrl Pts',(-2.47612541957012,-0.454542799479524,
17.4163109221582));
#15163=CARTESIAN_POINT('Ctrl Pts',(-2.46120816605392,-0.535804653509427,
17.421566300359));
#15164=CARTESIAN_POINT('Ctrl Pts',(-2.44225883457613,-0.616481443158024,
17.4268216785598));
#15165=CARTESIAN_POINT('Ctrl Pts',(-2.41933699953252,-0.696142753099517,
17.4320770567606));
#15166=CARTESIAN_POINT('Ctrl Pts',(-2.39644766574833,-0.775691109915955,
17.4373249832713));
#15167=CARTESIAN_POINT('Ctrl Pts',(-2.36959714308071,-0.854226407314903,
17.4425729097821));
#15168=CARTESIAN_POINT('Ctrl Pts',(-2.33889618428474,-0.931327487588705,
17.4478208362928));
#15169=CARTESIAN_POINT('Ctrl Pts',(-2.30797371162681,-1.0089848683405,17.4531066276949));
#15170=CARTESIAN_POINT('Ctrl Pts',(-2.27314509150085,-1.08518678259642,
17.4583924190969));
#15171=CARTESIAN_POINT('Ctrl Pts',(-2.23457499040448,-1.15951751270035,
17.463678210499));
#15172=CARTESIAN_POINT('Ctrl Pts',(-2.19634960303706,-1.23318392452612,
17.468916761038));
#15173=CARTESIAN_POINT('Ctrl Pts',(-2.15444956181177,-1.30501204838975,
17.474155311577));
#15174=CARTESIAN_POINT('Ctrl Pts',(-2.10908309225795,-1.37461804147611,
17.479393862116));
#15175=CARTESIAN_POINT('Ctrl Pts',(-2.06373155526043,-1.44420112346933,
17.484630688365));
#15176=CARTESIAN_POINT('Ctrl Pts',(-2.01491610773994,-1.51156314109537,
17.4898675146139));
#15177=CARTESIAN_POINT('Ctrl Pts',(-1.96288936701981,-1.57634754506757,
17.4951043408629));
#15178=CARTESIAN_POINT('Ctrl Pts',(-1.91086405949419,-1.6411301644065,17.5003410228516));
#15179=CARTESIAN_POINT('Ctrl Pts',(-1.85562792436406,-1.70333495216445,
17.5055777048404));
#15180=CARTESIAN_POINT('Ctrl Pts',(-1.79747422211945,-1.76263798631939,
17.5108143868291));
#15181=CARTESIAN_POINT('Ctrl Pts',(-1.7383717221883,-1.82290856990695,17.5161365070885));
#15182=CARTESIAN_POINT('Ctrl Pts',(-1.67625593135551,-1.88018150174497,
17.521458627348));
#15183=CARTESIAN_POINT('Ctrl Pts',(-1.6114727360507,-1.93415663041163,17.5267807476074));
#15184=CARTESIAN_POINT('Ctrl Pts',(-1.54763805495449,-1.98734148968497,
17.532024944778));
#15185=CARTESIAN_POINT('Ctrl Pts',(-1.48121397244005,-2.03732424332915,
17.5372691419485));
#15186=CARTESIAN_POINT('Ctrl Pts',(-1.4125623381495,-2.08386033381358,17.5425133391191));
#15187=CARTESIAN_POINT('Ctrl Pts',(-1.34238057048667,-2.13143363813568,
17.547874420923));
#15188=CARTESIAN_POINT('Ctrl Pts',(-1.26987119731387,-2.17540452485945,
17.5532355027269));
#15189=CARTESIAN_POINT('Ctrl Pts',(-1.19544746063087,-2.21556124241042,
17.5585965845308));
#15190=CARTESIAN_POINT('Ctrl Pts',(-1.12102372394787,-2.25571795996139,
17.5639576663347));
#15191=CARTESIAN_POINT('Ctrl Pts',(-1.04468611101973,-2.29206035026829,
17.5693187481386));
#15192=CARTESIAN_POINT('Ctrl Pts',(-0.966867730000397,-2.3244296166337,
17.5746798299424));
#15193=CARTESIAN_POINT('Ctrl Pts',(-0.890581262222371,-2.35616166969414,
17.579935374827));
#15194=CARTESIAN_POINT('Ctrl Pts',(-0.812590244233387,-2.38419277371056,
17.5851909197115));
#15195=CARTESIAN_POINT('Ctrl Pts',(-0.733288179464249,-2.40833857583563,
17.590446464596));
#15196=CARTESIAN_POINT('Ctrl Pts',(-0.654098502204564,-2.43245015834017,
17.595694561281));
#15197=CARTESIAN_POINT('Ctrl Pts',(-0.573601906437922,-2.45268724280885,
17.600942657966));
#15198=CARTESIAN_POINT('Ctrl Pts',(-0.492211990480921,-2.46891344652396,
17.606190754651));
#15199=CARTESIAN_POINT('Ctrl Pts',(-0.410238140398427,-2.48525606557093,
17.6114765039458));
#15200=CARTESIAN_POINT('Ctrl Pts',(-0.327358535705637,-2.49752982911297,
17.6167622532406));
#15201=CARTESIAN_POINT('Ctrl Pts',(-0.244011507871158,-2.50564655009968,
17.6220480025355));
#15202=CARTESIAN_POINT('Ctrl Pts',(-0.161405925479705,-2.51369106568274,
17.6272867304207));
#15203=CARTESIAN_POINT('Ctrl Pts',(-0.0783416707482684,-2.51765216040642,
17.6325254583061));
#15204=CARTESIAN_POINT('Ctrl Pts',(0.00474589535283771,-2.51749552660522,
17.6377641861914));
#15205=CARTESIAN_POINT('Ctrl Pts',(0.0878061498949002,-2.51733894429083,
17.6430011920642));
#15206=CARTESIAN_POINT('Ctrl Pts',(0.170889239592013,-2.51306732251811,
17.648238197937));
#15207=CARTESIAN_POINT('Ctrl Pts',(0.253558530604507,-2.50469844922651,
17.6534752038098));
#15208=CARTESIAN_POINT('Ctrl Pts',(0.33622557626592,-2.49632980323889,17.6587120674422));
#15209=CARTESIAN_POINT('Ctrl Pts',(0.418478386678491,-2.48386417448843,
17.6639489310745));
#15210=CARTESIAN_POINT('Ctrl Pts',(0.499885569466697,-2.4673712058462,17.6691857947069));
#15211=CARTESIAN_POINT('Ctrl Pts',(0.582614830094737,-2.4506103862895,17.6745077066252));
#15212=CARTESIAN_POINT('Ctrl Pts',(0.664470266354718,-2.42969032947554,
17.6798296185435));
#15213=CARTESIAN_POINT('Ctrl Pts',(0.745011870101685,-2.40473773276996,
17.6851515304618));
#15214=CARTESIAN_POINT('Ctrl Pts',(0.824380137189749,-2.38014864753034,
17.6903959123328));
#15215=CARTESIAN_POINT('Ctrl Pts',(0.902472181408065,-2.35164396016609,
17.6956402942038));
#15216=CARTESIAN_POINT('Ctrl Pts',(0.978885838437445,-2.31939405132173,
17.7008846760748));
#15217=CARTESIAN_POINT('Ctrl Pts',(1.0569939814684,-2.28642899519594,17.7062453530168));
#15218=CARTESIAN_POINT('Ctrl Pts',(1.13334794865923,-2.24955084994424,17.7116060299587));
#15219=CARTESIAN_POINT('Ctrl Pts',(1.20754524343109,-2.20899088614393,17.7169667069007));
#15220=CARTESIAN_POINT('Ctrl Pts',(1.28174253820295,-2.16843092234362,17.7223273838426));
#15221=CARTESIAN_POINT('Ctrl Pts',(1.35378276292312,-2.12418946243883,17.7276880607846));
#15222=CARTESIAN_POINT('Ctrl Pts',(1.42329700739684,-2.07654325231506,17.7330487377266));
#15223=CARTESIAN_POINT('Ctrl Pts',(1.49114503923816,-2.03003909182148,17.7382809226205));
#15224=CARTESIAN_POINT('Ctrl Pts',(1.55684230741931,-1.98011643527403,17.7435131075144));
#15225=CARTESIAN_POINT('Ctrl Pts',(1.62002178070411,-1.92700173327485,17.7487452924084));
#15226=CARTESIAN_POINT('Ctrl Pts',(1.68311147158066,-1.8739625109467,17.7539700420051));
#15227=CARTESIAN_POINT('Ctrl Pts',(1.74369011917883,-1.81774054837828,17.7591947916019));
#15228=CARTESIAN_POINT('Ctrl Pts',(1.80141980490829,-1.75860539533011,17.7644195411987));
#15229=CARTESIAN_POINT('Ctrl Pts',(1.85908359270269,-1.69953774454575,17.7696383267891));
#15230=CARTESIAN_POINT('Ctrl Pts',(1.91390455729977,-1.63756384313869,17.7748571123796));
#15231=CARTESIAN_POINT('Ctrl Pts',(1.96557915130772,-1.57299232354911,17.78007589797));
#15232=CARTESIAN_POINT('Ctrl Pts',(2.0172216290745,-1.50846093575999,17.7852914400366));
#15233=CARTESIAN_POINT('Ctrl Pts',(2.06572132715847,-1.44133549699604,17.7905069821033));
#15234=CARTESIAN_POINT('Ctrl Pts',(2.11081356801578,-1.37195930372606,17.7957225241699));
#15235=CARTESIAN_POINT('Ctrl Pts',(2.15589170309462,-1.3026048127533,17.8009364347079));
#15236=CARTESIAN_POINT('Ctrl Pts',(2.19756424383842,-1.23100135583603,17.8061503452459));
#15237=CARTESIAN_POINT('Ctrl Pts',(2.23560946646314,-1.15752173347216,17.811364255784));
#15238=CARTESIAN_POINT('Ctrl Pts',(2.27365453179013,-1.08404241490932,17.8165781447651));
#15239=CARTESIAN_POINT('Ctrl Pts',(2.30807209595416,-1.00868736085614,17.8217920337462));
#15240=CARTESIAN_POINT('Ctrl Pts',(2.33868677023716,-0.931853229171688,
17.8270059227274));
#15241=CARTESIAN_POINT('Ctrl Pts',(2.36933131546493,-0.854944129905247,
17.8322248989353));
#15242=CARTESIAN_POINT('Ctrl Pts',(2.39616538709405,-0.776553504509373,
17.8374438751432));
#15243=CARTESIAN_POINT('Ctrl Pts',(2.41906231446636,-0.697096671006736,
17.842662851351));
#15244=CARTESIAN_POINT('Ctrl Pts',(2.44197035495879,-0.61760127279533,17.847884360611));
#15245=CARTESIAN_POINT('Ctrl Pts',(2.46093733889407,-0.53703908994231,17.853105869871));
#15246=CARTESIAN_POINT('Ctrl Pts',(2.47588753009016,-0.455836800120435,
17.8583273791309));
#15247=CARTESIAN_POINT('Ctrl Pts',(2.49086382410593,-0.374492732263679,
17.8635580050713));
#15248=CARTESIAN_POINT('Ctrl Pts',(2.50180925357153,-0.292506787464058,
17.8687886310116));
#15249=CARTESIAN_POINT('Ctrl Pts',(2.50869990928057,-0.210311709554351,
17.874019256952));
#15250=CARTESIAN_POINT('Ctrl Pts',(2.51458302607921,-0.140135043641119,
17.8784850704589));
#15251=CARTESIAN_POINT('Ctrl Pts',(2.51751132661983,-0.0698061540768173,
17.8829508839658));
#15252=CARTESIAN_POINT('Ctrl Pts',(2.5174999670525,0.000407296750591967,
17.8874166974728));
#15253=CARTESIAN_POINT('Ctrl Pts',(2.51749996705241,0.000407297304472808,
17.887416697508));
#15254=CARTESIAN_POINT('Ctrl Pts',(2.51749657468057,0.0213755087636416,
17.8887503468423));
#15255=CARTESIAN_POINT('Ctrl Pts',(2.51723122171354,0.0423413984397853,
17.8900839961765));
#15256=CARTESIAN_POINT('Ctrl Pts',(2.51670405080776,0.0633006370255141,
17.8914176455107));
#15257=CARTESIAN_POINT('Ctrl Pts',(2.5146266529764,0.145893732181795,17.896673095317));
#15258=CARTESIAN_POINT('Ctrl Pts',(2.50847531607989,0.228536699531577,17.9019285451234));
#15259=CARTESIAN_POINT('Ctrl Pts',(2.49824190001089,0.310795204322675,17.9071839949297));
#15260=CARTESIAN_POINT('Ctrl Pts',(2.48802121681506,0.392951359409476,17.9124329056707));
#15261=CARTESIAN_POINT('Ctrl Pts',(2.47372859023847,0.474723547684112,17.9176818164117));
#15262=CARTESIAN_POINT('Ctrl Pts',(2.45540786448767,0.555678386310031,17.9229307271527));
#15263=CARTESIAN_POINT('Ctrl Pts',(2.43710787198325,0.63654160975444,17.9281736977929));
#15264=CARTESIAN_POINT('Ctrl Pts',(2.41478894139686,0.716588874401286,17.933416668433));
#15265=CARTESIAN_POINT('Ctrl Pts',(2.38854638991777,0.795394489049787,17.9386596390731));
#15266=CARTESIAN_POINT('Ctrl Pts',(2.37992633856821,0.821280251165781,17.9403818296984));
#15267=CARTESIAN_POINT('Ctrl Pts',(2.37088335268766,0.847032122939052,17.9421040203238));
#15268=CARTESIAN_POINT('Ctrl Pts',(2.36142200728635,0.872635292378034,17.9438262109491));
#15269=CARTESIAN_POINT('Ctrl Pts',(2.36142200245778,0.872635305444532,17.6666805052528));
#15270=CARTESIAN_POINT('Ctrl Pts',(2.36852647042101,0.853410038188607,17.6653488246657));
#15271=CARTESIAN_POINT('Ctrl Pts',(2.37539678106655,0.834096324145541,17.664024563499));
#15272=CARTESIAN_POINT('Ctrl Pts',(2.38873305764868,0.795103455874879,17.6613777297893));
#15273=CARTESIAN_POINT('Ctrl Pts',(2.39519300344129,0.775426105040596,17.66005555027));
#15274=CARTESIAN_POINT('Ctrl Pts',(2.40524360830356,0.743486775147538,17.6579307055959));
#15275=CARTESIAN_POINT('Ctrl Pts',(2.40898492362142,0.731273579197981,17.6571231700799));
#15276=CARTESIAN_POINT('Ctrl Pts',(2.41597663677348,0.707813659158462,17.6555813333287));
#15277=CARTESIAN_POINT('Ctrl Pts',(2.41924184681766,0.696571733251215,17.6548465694267));
#15278=CARTESIAN_POINT('Ctrl Pts',(2.42652206522257,0.670837570782211,17.6531737039883));
#15279=CARTESIAN_POINT('Ctrl Pts',(2.43048590078596,0.656331228056072,17.6522372708427));
#15280=CARTESIAN_POINT('Ctrl Pts',(2.44262275397272,0.610295951665459,17.64928557178));
#15281=CARTESIAN_POINT('Ctrl Pts',(2.4503142302106,0.578642712636493,17.6472856822565));
#15282=CARTESIAN_POINT('Ctrl Pts',(2.4975046369567,0.366581558053989,17.6340659710036));
#15283=CARTESIAN_POINT('Ctrl Pts',(2.51766433186062,0.182446283241399,17.6234981640375));
#15284=CARTESIAN_POINT('Ctrl Pts',(2.51737314526642,-0.142834673721351,
17.6047994949253));
#15285=CARTESIAN_POINT('Ctrl Pts',(2.50547210456535,-0.283140984149819,
17.5967034201887));
#15286=CARTESIAN_POINT('Ctrl Pts',(2.47836124638302,-0.442702605875776,
17.586762917611));
#15287=CARTESIAN_POINT('Ctrl Pts',(2.47452654459574,-0.463657606306495,
17.5854424349002));
#15288=CARTESIAN_POINT('Ctrl Pts',(2.46880880944116,-0.492808231115945,
17.5835813541932));
#15289=CARTESIAN_POINT('Ctrl Pts',(2.46714981917896,-0.501047557853925,
17.5830526232002));
#15290=CARTESIAN_POINT('Ctrl Pts',(2.46421419884374,-0.515259088736036,
17.5821357333558));
#15291=CARTESIAN_POINT('Ctrl Pts',(2.46295702464022,-0.52123530116268,17.5817486602479));
#15292=CARTESIAN_POINT('Ctrl Pts',(2.46025563017538,-0.533848878301397,
17.5809283994724));
#15293=CARTESIAN_POINT('Ctrl Pts',(2.45880627580423,-0.540485046418643,
17.5804949144544));
#15294=CARTESIAN_POINT('Ctrl Pts',(2.45513795121516,-0.556961074306295,
17.5794139983031));
#15295=CARTESIAN_POINT('Ctrl Pts',(2.45288668210509,-0.566793537660574,
17.5787647830077));
#15296=CARTESIAN_POINT('Ctrl Pts',(2.44413713215133,-0.603978751760093,
17.5762944641234));
#15297=CARTESIAN_POINT('Ctrl Pts',(2.43724017005016,-0.631234386566123,
17.5744528644979));
#15298=CARTESIAN_POINT('Ctrl Pts',(2.41831461962658,-0.701084408853424,
17.5696631146307));
#15299=CARTESIAN_POINT('Ctrl Pts',(2.40561685005594,-0.743486432645809,
17.566687766892));
#15300=CARTESIAN_POINT('Ctrl Pts',(2.35326574772843,-0.902887038657014,
17.5552960553576));
#15301=CARTESIAN_POINT('Ctrl Pts',(2.30613835098239,-1.01724605370534,17.5467044586598));
#15302=CARTESIAN_POINT('Ctrl Pts',(2.1784670537797,-1.27207300962614,17.5270809238036));
#15303=CARTESIAN_POINT('Ctrl Pts',(2.09238842307821,-1.40918985266541,17.5161731667699));
#15304=CARTESIAN_POINT('Ctrl Pts',(1.98017136880731,-1.55474178976035,17.5043194883343));
#15305=CARTESIAN_POINT('Ctrl Pts',(1.96636158319714,-1.57217138333776,17.5028944245018));
#15306=CARTESIAN_POINT('Ctrl Pts',(1.9432378780257,-1.60057484736021,17.5005622258075));
#15307=CARTESIAN_POINT('Ctrl Pts',(1.93405779151004,-1.61165559772919,17.4996498425999));
#15308=CARTESIAN_POINT('Ctrl Pts',(1.91729955697565,-1.63153408181015,17.4980081898046));
#15309=CARTESIAN_POINT('Ctrl Pts',(1.90975464670018,-1.64035918261111,17.4972776066568));
#15310=CARTESIAN_POINT('Ctrl Pts',(1.89343293617127,-1.65918504066857,17.4957151231963));
#15311=CARTESIAN_POINT('Ctrl Pts',(1.88463733026128,-1.66916908284766,17.4948840246181));
#15312=CARTESIAN_POINT('Ctrl Pts',(1.86032366647938,-1.69633073303629,17.4926158484728));
#15313=CARTESIAN_POINT('Ctrl Pts',(1.84464695245412,-1.71336504447413,17.4911854083391));
#15314=CARTESIAN_POINT('Ctrl Pts',(1.75069344833865,-1.81267040253474,17.4827934073785));
#15315=CARTESIAN_POINT('Ctrl Pts',(1.66715297498732,-1.88979022795572,17.4760660046176));
#15316=CARTESIAN_POINT('Ctrl Pts',(1.49822145318466,-2.02578578548784,17.4634503421306));
#15317=CARTESIAN_POINT('Ctrl Pts',(1.41385019477008,-2.08554635922527,17.4575516252619));
#15318=CARTESIAN_POINT('Ctrl Pts',(1.2746231586498,-2.17181993181033,17.4481173036935));
#15319=CARTESIAN_POINT('Ctrl Pts',(1.22206953903167,-2.20182005116195,17.4446172366581));
#15320=CARTESIAN_POINT('Ctrl Pts',(1.10254187341139,-2.26445375093377,17.436685062568));
#15321=CARTESIAN_POINT('Ctrl Pts',(1.03510107053155,-2.29606466647722,17.4322283108932));
#15322=CARTESIAN_POINT('Ctrl Pts',(0.954372317157444,-2.32962409901796,
17.4268033747336));
#15323=CARTESIAN_POINT('Ctrl Pts',(0.942340328305685,-2.3345170060709,17.4259925276703));
#15324=CARTESIAN_POINT('Ctrl Pts',(0.92265979136514,-2.34234332592722,17.4246616525941));
#15325=CARTESIAN_POINT('Ctrl Pts',(0.915033669660928,-2.34533296698862,
17.4241448293723));
#15326=CARTESIAN_POINT('Ctrl Pts',(0.90132122913042,-2.35063154618716,17.4232133058139));
#15327=CARTESIAN_POINT('Ctrl Pts',(0.895240384186967,-2.35295415948832,
17.4227994217957));
#15328=CARTESIAN_POINT('Ctrl Pts',(0.881825309052589,-2.3580185920181,17.4218845545394));
#15329=CARTESIAN_POINT('Ctrl Pts',(0.87448736370691,-2.36074975436955,17.4213829782638));
#15330=CARTESIAN_POINT('Ctrl Pts',(0.853181412280496,-2.36856680301356,
17.4199235527773));
#15331=CARTESIAN_POINT('Ctrl Pts',(0.83918122564888,-2.37356315861529,17.4189607341301));
#15332=CARTESIAN_POINT('Ctrl Pts',(0.721029303889196,-2.41455298544116,
17.4108079374253));
#15333=CARTESIAN_POINT('Ctrl Pts',(0.614672686949972,-2.44379241553572,
17.4032962562693));
#15334=CARTESIAN_POINT('Ctrl Pts',(0.336499328528819,-2.50095706370979,
17.3837385649846));
#15335=CARTESIAN_POINT('Ctrl Pts',(0.163053289205865,-2.5182225300802,17.3716617216909));
#15336=CARTESIAN_POINT('Ctrl Pts',(-0.0818745105656113,-2.51717197942581,
17.3553260338495));
#15337=CARTESIAN_POINT('Ctrl Pts',(-0.152911277046764,-2.51385719079346,
17.3506665708687));
#15338=CARTESIAN_POINT('Ctrl Pts',(-0.244680875857199,-2.50566965780357,
17.3447468227948));
#15339=CARTESIAN_POINT('Ctrl Pts',(-0.265619383338332,-2.50353660891511,
17.3434027949171));
#15340=CARTESIAN_POINT('Ctrl Pts',(-0.299293162852124,-2.49967896122964,
17.3412514821693));
#15341=CARTESIAN_POINT('Ctrl Pts',(-0.31204592046886,-2.49811902438594,
17.3404391051219));
#15342=CARTESIAN_POINT('Ctrl Pts',(-0.336376510593825,-2.49495364647654,
17.3388935122801));
#15343=CARTESIAN_POINT('Ctrl Pts',(-0.347956160916023,-2.49336507002573,
17.3381597907208));
#15344=CARTESIAN_POINT('Ctrl Pts',(-0.374515202248042,-2.4895328905997,
17.3364810306681));
#15345=CARTESIAN_POINT('Ctrl Pts',(-0.389486343124227,-2.48723461989581,
17.3355377292126));
#15346=CARTESIAN_POINT('Ctrl Pts',(-0.436284966240024,-2.47961749090798,
17.3325977646291));
#15347=CARTESIAN_POINT('Ctrl Pts',(-0.468032269140274,-2.473821621065,17.3306160580795));
#15348=CARTESIAN_POINT('Ctrl Pts',(-0.628555134452087,-2.44131518036286,
17.3206472409808));
#15349=CARTESIAN_POINT('Ctrl Pts',(-0.755213322066048,-2.4051527878217,
17.312963795227));
#15350=CARTESIAN_POINT('Ctrl Pts',(-1.01011534986747,-2.31023897717009,
17.2972746945933));
#15351=CARTESIAN_POINT('Ctrl Pts',(-1.13741126208741,-2.25029517202352,
17.2893089230232));
#15352=CARTESIAN_POINT('Ctrl Pts',(-1.31597236321481,-2.14717161568439,
17.2771259365905));
#15353=CARTESIAN_POINT('Ctrl Pts',(-1.37159344056241,-2.11207458757824,
17.2731708088443));
#15354=CARTESIAN_POINT('Ctrl Pts',(-1.4371224858811,-2.06704496328576,17.2682333979137));
#15355=CARTESIAN_POINT('Ctrl Pts',(-1.4484084966615,-2.05915242918485,17.267372675277));
#15356=CARTESIAN_POINT('Ctrl Pts',(-1.46588726439985,-2.04671438631972,
17.2660224823702));
#15357=CARTESIAN_POINT('Ctrl Pts',(-1.47212512858,-2.04223232106142,17.2655371706916));
#15358=CARTESIAN_POINT('Ctrl Pts',(-1.48309119450267,-2.03427657432648,
17.2646777043376));
#15359=CARTESIAN_POINT('Ctrl Pts',(-1.48782788829705,-2.03081482286425,
17.2643043643747));
#15360=CARTESIAN_POINT('Ctrl Pts',(-1.49902503710075,-2.02257133117975,
17.2634168335519));
#15361=CARTESIAN_POINT('Ctrl Pts',(-1.50547466017881,-2.01777523398066,
17.2629016683259));
#15362=CARTESIAN_POINT('Ctrl Pts',(-1.52459393713099,-2.0034149773373,17.2613630152951));
#15363=CARTESIAN_POINT('Ctrl Pts',(-1.53719594113133,-1.99376198496496,
17.2603337224881));
#15364=CARTESIAN_POINT('Ctrl Pts',(-1.66124153343151,-1.89686933218797,
17.2500579089718));
#15365=CARTESIAN_POINT('Ctrl Pts',(-1.76522068708018,-1.800506636014,17.2402943683696));
#15366=CARTESIAN_POINT('Ctrl Pts',(-1.9908605028757,-1.55296586749063,17.217154659469));
#15367=CARTESIAN_POINT('Ctrl Pts',(-2.10428986702762,-1.39542791838508,
17.2038855962678));
#15368=CARTESIAN_POINT('Ctrl Pts',(-2.21415981578012,-1.19846881134589,
17.1892427120159));
#15369=CARTESIAN_POINT('Ctrl Pts',(-2.22922187092713,-1.1702141624134,17.1871827037195));
#15370=CARTESIAN_POINT('Ctrl Pts',(-2.25051523571947,-1.12836631022428,
17.1841892486697));
#15371=CARTESIAN_POINT('Ctrl Pts',(-2.25717050774065,-1.11499357438125,
17.1832411284448));
#15372=CARTESIAN_POINT('Ctrl Pts',(-2.26882302673851,-1.09104768752096,
17.1815581356364));
#15373=CARTESIAN_POINT('Ctrl Pts',(-2.27386631628235,-1.08049755493998,
17.1808216890569));
#15374=CARTESIAN_POINT('Ctrl Pts',(-2.2842867905785,-1.05830270130007,17.1792827712986));
#15375=CARTESIAN_POINT('Ctrl Pts',(-2.28964887319293,-1.04665122957376,
17.1784808341678));
#15376=CARTESIAN_POINT('Ctrl Pts',(-2.30353301862119,-1.01586447963842,
17.1763771207906));
#15377=CARTESIAN_POINT('Ctrl Pts',(-2.31190582387938,-0.996662686845945,
17.1750804273303));
#15378=CARTESIAN_POINT('Ctrl Pts',(-2.35054783521849,-0.904934858698359,
17.1689557611542));
#15379=CARTESIAN_POINT('Ctrl Pts',(-2.3776514490624,-0.831118286420926,
17.1642342406773));
#15380=CARTESIAN_POINT('Ctrl Pts',(-2.44373228989777,-0.621269042164098,
17.1512420651925));
#15381=CARTESIAN_POINT('Ctrl Pts',(-2.47476609064376,-0.483050291452884,
17.1431862309463));
#15382=CARTESIAN_POINT('Ctrl Pts',(-2.50195272400195,-0.285342698903077,
17.1316932275178));
#15383=CARTESIAN_POINT('Ctrl Pts',(-2.50787587372179,-0.227477582243425,
17.1283304593088));
#15384=CARTESIAN_POINT('Ctrl Pts',(-2.51329123624318,-0.147210017682062,
17.1236095816729));
#15385=CARTESIAN_POINT('Ctrl Pts',(-2.51449667804207,-0.124940147803237,
17.1222937910304));
#15386=CARTESIAN_POINT('Ctrl Pts',(-2.51774068580823,-0.0454527179734783,
17.1175670775158));
#15387=CARTESIAN_POINT('Ctrl Pts',(-2.51812301768035,0.01181060981283,17.1141060973369));
#15388=CARTESIAN_POINT('Ctrl Pts',(-2.5161898701013,0.0822830847172104,
17.1097244262833));
#15389=CARTESIAN_POINT('Ctrl Pts',(-2.5157217375488,0.0955305703542631,
17.1088954189292));
#15390=CARTESIAN_POINT('Ctrl Pts',(-2.51482219019189,0.116330651720235,
17.1075845361629));
#15391=CARTESIAN_POINT('Ctrl Pts',(-2.51446130557067,0.12388627060511,17.1071064410165));
#15392=CARTESIAN_POINT('Ctrl Pts',(-2.51375936165838,0.137312420783076,
17.1062532872409));
#15393=CARTESIAN_POINT('Ctrl Pts',(-2.51343177838748,0.143183526404349,
17.1058789792501));
#15394=CARTESIAN_POINT('Ctrl Pts',(-2.51259883877228,0.157227128567068,
17.1049807090772));
#15395=CARTESIAN_POINT('Ctrl Pts',(-2.51207418207066,0.165398288499605,
17.104455696716));
#15396=CARTESIAN_POINT('Ctrl Pts',(-2.51036351088478,0.190151709419325,
17.102858381021));
#15397=CARTESIAN_POINT('Ctrl Pts',(-2.50905312027644,0.206724537112013,
17.1017796145281));
#15398=CARTESIAN_POINT('Ctrl Pts',(-2.49564153304598,0.357343549882187,
17.0918977360187));
#15399=CARTESIAN_POINT('Ctrl Pts',(-2.47297397648725,0.490217386015908,
17.0826310717887));
#15400=CARTESIAN_POINT('Ctrl Pts',(-2.39047438510124,0.81453871419814,17.059515922372));
#15401=CARTESIAN_POINT('Ctrl Pts',(-2.31819608817071,1.00191670106038,17.0457675949804));
#15402=CARTESIAN_POINT('Ctrl Pts',(-2.20975742059279,1.20655140952358,17.0307387114162));
#15403=CARTESIAN_POINT('Ctrl Pts',(-2.19452099841641,1.23404695822713,17.0287169450877));
#15404=CARTESIAN_POINT('Ctrl Pts',(-2.17126358267775,1.27422344232747,17.0257578820989));
#15405=CARTESIAN_POINT('Ctrl Pts',(-2.16363825053626,1.28712876709745,17.0248066183301));
#15406=CARTESIAN_POINT('Ctrl Pts',(-2.14987271574392,1.30995790351896,17.0231222368029));
#15407=CARTESIAN_POINT('Ctrl Pts',(-2.14377797723277,1.31990847963964,17.0223875054212));
#15408=CARTESIAN_POINT('Ctrl Pts',(-2.1307845751477,1.3407947309133,17.0208439532374));
#15409=CARTESIAN_POINT('Ctrl Pts',(-2.12387038762523,1.35172038625714,17.0200357265744));
#15410=CARTESIAN_POINT('Ctrl Pts',(-2.1052786611993,1.38060379103463,17.0178966212008));
#15411=CARTESIAN_POINT('Ctrl Pts',(-2.09345542343198,1.39846684013917,17.0165711451767));
#15412=CARTESIAN_POINT('Ctrl Pts',(-2.03379995725953,1.48614457009966,17.0100491507113));
#15413=CARTESIAN_POINT('Ctrl Pts',(-1.98269395186465,1.55367140362027,17.0049773569991));
#15414=CARTESIAN_POINT('Ctrl Pts',(-1.86426094576879,1.6947722449797,16.9941315085167));
#15415=CARTESIAN_POINT('Ctrl Pts',(-1.79577175247373,1.76718053498851,16.9884023009395));
#15416=CARTESIAN_POINT('Ctrl Pts',(-1.60595414008019,1.94539693318515,16.9734409095532));
#15417=CARTESIAN_POINT('Ctrl Pts',(-1.47847874253534,2.04395315689368,16.9642635590213));
#15418=CARTESIAN_POINT('Ctrl Pts',(-1.32516284582363,2.14060031858582,16.9531207272754));
#15419=CARTESIAN_POINT('Ctrl Pts',(-1.30769305100589,2.15131706505944,16.951849367027));
#15420=CARTESIAN_POINT('Ctrl Pts',(-1.28299466097652,2.16605616711589,16.9500467706899));
#15421=CARTESIAN_POINT('Ctrl Pts',(-1.27587359057164,2.1702583246172,16.9495264476917));
#15422=CARTESIAN_POINT('Ctrl Pts',(-1.26296498426474,2.17779022883212,16.9485819250208));
#15423=CARTESIAN_POINT('Ctrl Pts',(-1.25718459163581,2.18113221363248,16.9481584998522));
#15424=CARTESIAN_POINT('Ctrl Pts',(-1.24533274748168,2.18792169545012,16.9472892220381));
#15425=CARTESIAN_POINT('Ctrl Pts',(-1.23926015649566,2.1913669841099,16.9468432439203));
#15426=CARTESIAN_POINT('Ctrl Pts',(-1.22361179927868,2.20015924442058,16.945692673882));
#15427=CARTESIAN_POINT('Ctrl Pts',(-1.21401539841958,2.20546891569288,16.9449858036987));
#15428=CARTESIAN_POINT('Ctrl Pts',(-1.17344779959629,2.22756990430983,16.9419932027643));
#15429=CARTESIAN_POINT('Ctrl Pts',(-1.14216218370164,2.24377197341134,16.9396746249137));
#15430=CARTESIAN_POINT('Ctrl Pts',(-1.05570762704758,2.28626811364174,16.9332588189138));
#15431=CARTESIAN_POINT('Ctrl Pts',(-0.999906399621586,2.31121758519661,
16.9291087384412));
#15432=CARTESIAN_POINT('Ctrl Pts',(-0.769907649540935,2.4041642736662,16.9121072641027));
#15433=CARTESIAN_POINT('Ctrl Pts',(-0.589268904905663,2.45469747938334,
16.8990469173539));
#15434=CARTESIAN_POINT('Ctrl Pts',(-0.328019710017269,2.49724735320643,
16.8813303737569));
#15435=CARTESIAN_POINT('Ctrl Pts',(-0.250801782163873,2.50618072842428,
16.8762247917211));
#15436=CARTESIAN_POINT('Ctrl Pts',(-0.151648156964318,2.51302199753124,
16.8698343664724));
#15437=CARTESIAN_POINT('Ctrl Pts',(-0.129990276075862,2.514235331034,16.8684484209119));
#15438=CARTESIAN_POINT('Ctrl Pts',(-0.0953427365522925,2.51572747022526,
16.8662464797875));
#15439=CARTESIAN_POINT('Ctrl Pts',(-0.0823622982543662,2.51618588422144,
16.8654249534322));
#15440=CARTESIAN_POINT('Ctrl Pts',(-0.0577272197924998,2.51686504964141,
16.8638720936828));
#15441=CARTESIAN_POINT('Ctrl Pts',(-0.0460735021914871,2.51710535134083,
16.8631401736264));
#15442=CARTESIAN_POINT('Ctrl Pts',(-0.0195375784786025,2.51746817508612,
16.8614794388107));
#15443=CARTESIAN_POINT('Ctrl Pts',(-0.00465502397778445,2.51753968693572,
16.8605522284459));
#15444=CARTESIAN_POINT('Ctrl Pts',(0.0410955819904817,2.51735381988979,
16.8577141679389));
#15445=CARTESIAN_POINT('Ctrl Pts',(0.0719596710107643,2.51666069115791,
16.8558167976196));
#15446=CARTESIAN_POINT('Ctrl Pts',(0.222730710596222,2.51049868640108,16.8466211458042));
#15447=CARTESIAN_POINT('Ctrl Pts',(0.342160070320115,2.49702701188625,16.8395727410772));
#15448=CARTESIAN_POINT('Ctrl Pts',(0.551896097116948,2.45803149504487,16.8272310651655));
#15449=CARTESIAN_POINT('Ctrl Pts',(0.642589129244993,2.43589559007007,16.8219037203371));
#15450=CARTESIAN_POINT('Ctrl Pts',(0.850847305419339,2.37262177351255,16.8093448610315));
#15451=CARTESIAN_POINT('Ctrl Pts',(0.966992219218174,2.32770123747517,16.8020888789459));
#15452=CARTESIAN_POINT('Ctrl Pts',(1.09171545978951,2.26851309564244,16.7935331180829));
#15453=CARTESIAN_POINT('Ctrl Pts',(1.10405612927462,2.26253273001271,16.7926778683132));
#15454=CARTESIAN_POINT('Ctrl Pts',(1.12388270772251,2.25272381693973,16.7912887441196));
#15455=CARTESIAN_POINT('Ctrl Pts',(1.13139955807838,2.24895797455137,16.7907585580609));
#15456=CARTESIAN_POINT('Ctrl Pts',(1.14471441206514,2.24220376224245,16.7898128931002));
#15457=CARTESIAN_POINT('Ctrl Pts',(1.15051984913076,2.2392304195662,16.789398342989));
#15458=CARTESIAN_POINT('Ctrl Pts',(1.15634887610778,2.23621634201296,16.7889798335824));
#15459=CARTESIAN_POINT('Ctrl Pts',(1.15638397704102,2.23619819094917,16.7889773133415));
#15460=CARTESIAN_POINT('Ctrl Pts',(1.1564526386876,2.23616268323664,16.7889723832859));
#15461=CARTESIAN_POINT('Ctrl Pts',(1.15648619946039,2.236145326647,16.788969973474));
#15462=CARTESIAN_POINT('Ctrl Pts',(1.1565518499205,2.23611137239421,16.7889652593329));
#15463=CARTESIAN_POINT('Ctrl Pts',(1.15658393963845,2.23609477479726,16.7889629550081));
#15464=CARTESIAN_POINT('Ctrl Pts',(1.15665248055706,2.23605932186635,16.7889580330181));
#15465=CARTESIAN_POINT('Ctrl Pts',(1.15668893168188,2.23604046631738,16.7889554153385));
#15466=CARTESIAN_POINT('Ctrl Pts',(1.15676146848256,2.23600294201165,16.7889502060462));
#15467=CARTESIAN_POINT('Ctrl Pts',(1.15679755411129,2.23598427330176,16.7889476144387));
#15468=CARTESIAN_POINT('Ctrl Pts',(1.15686936439946,2.2359471204239,16.7889424569744));
#15469=CARTESIAN_POINT('Ctrl Pts',(1.15690508909205,2.23592863626075,16.788939891117));
#15470=CARTESIAN_POINT('Ctrl Pts',(1.15697618209334,2.23589185016955,16.7889347848285));
#15471=CARTESIAN_POINT('Ctrl Pts',(1.15701155040356,2.2358735482622,16.7889322443992));
#15472=CARTESIAN_POINT('Ctrl Pts',(1.15708193506811,2.23583712445553,16.788927188654));
#15473=CARTESIAN_POINT('Ctrl Pts',(1.15711695145003,2.23581900256294,16.7889246733378));
#15474=CARTESIAN_POINT('Ctrl Pts',(1.15718663671241,2.23578293654329,16.788919667504));
#15475=CARTESIAN_POINT('Ctrl Pts',(1.15722130559132,2.23576499243759,16.7889171769881));
#15476=CARTESIAN_POINT('Ctrl Pts',(1.15729030017731,2.23572927981218,16.7889122204486));
#15477=CARTESIAN_POINT('Ctrl Pts',(1.15732462589627,2.23571151130642,16.7889097544258));
#15478=CARTESIAN_POINT('Ctrl Pts',(1.15739293846639,2.235676147713,16.788904846568));
#15479=CARTESIAN_POINT('Ctrl Pts',(1.1574269253212,2.23565855264309,16.7889024047343));
#15480=CARTESIAN_POINT('Ctrl Pts',(1.1574945643791,2.23562353379743,16.7888975449567));
#15481=CARTESIAN_POINT('Ctrl Pts',(1.15752821659453,2.23560611003449,16.7888951270133));
#15482=CARTESIAN_POINT('Ctrl Pts',(1.15759519056256,2.23557143169134,16.7888903147196));
#15483=CARTESIAN_POINT('Ctrl Pts',(1.15762851231809,2.2355541771284,16.7888879203707));
#15484=CARTESIAN_POINT('Ctrl Pts',(1.15769482944929,2.23551983512718,16.788883154977));
#15485=CARTESIAN_POINT('Ctrl Pts',(1.15772782484072,2.23550274769911,16.7888807839326));
#15486=CARTESIAN_POINT('Ctrl Pts',(1.15779349337626,2.23546873788239,16.7888760648554));
#15487=CARTESIAN_POINT('Ctrl Pts',(1.15782616649475,2.23545181552499,16.7888737168259));
#15488=CARTESIAN_POINT('Ctrl Pts',(1.15789119438795,2.23541813388157,16.7888690435022));
#15489=CARTESIAN_POINT('Ctrl Pts',(1.15792354919917,2.23540137459422,16.7888667182068));
#15490=CARTESIAN_POINT('Ctrl Pts',(1.15798794447562,2.23536801707263,16.788862090068));
#15491=CARTESIAN_POINT('Ctrl Pts',(1.15801998493697,2.2353514188576,16.7888597872264));
#15492=CARTESIAN_POINT('Ctrl Pts',(1.15808375540778,2.23531838151474,16.7888552037195));
#15493=CARTESIAN_POINT('Ctrl Pts',(1.15811548541356,2.23530194240563,16.7888529230557));
#15494=CARTESIAN_POINT('Ctrl Pts',(1.15817863878579,2.2352692213496,16.7888483836346));
#15495=CARTESIAN_POINT('Ctrl Pts',(1.15821006216592,2.23525293941203,16.7888461248774));
#15496=CARTESIAN_POINT('Ctrl Pts',(1.15827260605423,2.23522053079621,16.7888416290025));
#15497=CARTESIAN_POINT('Ctrl Pts',(1.15830372658138,2.23520440412421,16.7888393918846));
#15498=CARTESIAN_POINT('Ctrl Pts',(1.1583656685171,2.23517230414258,16.7888349390222));
#15499=CARTESIAN_POINT('Ctrl Pts',(1.158396489928,2.23515633084749,16.7888327232787));
#15500=CARTESIAN_POINT('Ctrl Pts',(1.15845783728866,2.23512453577125,16.7888283129059));
#15501=CARTESIAN_POINT('Ctrl Pts',(1.1584883632538,2.23510871399753,16.7888261182766));
#15502=CARTESIAN_POINT('Ctrl Pts',(1.15854912333037,2.23507722014031,16.7888217498764));
#15503=CARTESIAN_POINT('Ctrl Pts',(1.15857935745914,2.23506154806289,16.7888195761055));
#15504=CARTESIAN_POINT('Ctrl Pts',(1.15863953749895,2.23503035175856,16.7888152491641));
#15505=CARTESIAN_POINT('Ctrl Pts',(1.15866948339032,2.23501482755658,16.7888130959963));
#15506=CARTESIAN_POINT('Ctrl Pts',(1.15872909039696,2.23498392526302,16.7888088100171));
#15507=CARTESIAN_POINT('Ctrl Pts',(1.1587587515387,2.23496854717214,16.7888066772051));
#15508=CARTESIAN_POINT('Ctrl Pts',(1.15881779260454,2.23493793529896,16.788802431685));
#15509=CARTESIAN_POINT('Ctrl Pts',(1.15884717250253,2.23492270154432,16.7888003189799));
#15510=CARTESIAN_POINT('Ctrl Pts',(1.15890565443687,2.23489237664567,16.788796113436));
#15511=CARTESIAN_POINT('Ctrl Pts',(1.1589347564993,2.23487728550195,16.7887940205962));
#15512=CARTESIAN_POINT('Ctrl Pts',(1.16596386831419,2.23123210032163,16.7882885168057));
#15513=CARTESIAN_POINT('Ctrl Pts',(1.17294667193779,2.22756919723958,16.7877830656492));
#15514=CARTESIAN_POINT('Ctrl Pts',(1.19364229379309,2.21658880102117,16.7862755062734));
#15515=CARTESIAN_POINT('Ctrl Pts',(1.20730438741661,2.20917720562903,16.7852678403533));
#15516=CARTESIAN_POINT('Ctrl Pts',(1.23874542671307,2.19174190270448,16.7829214176238));
#15517=CARTESIAN_POINT('Ctrl Pts',(1.25647266220078,2.18162764752998,16.7815778823021));
#15518=CARTESIAN_POINT('Ctrl Pts',(1.45450050518641,2.06542893160591,16.7663527645449));
#15519=CARTESIAN_POINT('Ctrl Pts',(1.62102341867364,1.93748633406573,16.7515932693172));
#15520=CARTESIAN_POINT('Ctrl Pts',(1.85413250927938,1.70706149253897,16.7292684387356));
#15521=CARTESIAN_POINT('Ctrl Pts',(1.93247656960569,1.6178404408104,16.7213655716422));
#15522=CARTESIAN_POINT('Ctrl Pts',(2.01867499737448,1.50443540966903,16.7121834708676));
#15523=CARTESIAN_POINT('Ctrl Pts',(2.03283199644166,1.48525041154071,16.7106571168647));
#15524=CARTESIAN_POINT('Ctrl Pts',(2.05463125985263,1.45481321337406,16.7082768056118));
#15525=CARTESIAN_POINT('Ctrl Pts',(2.0624582331433,1.44369565632973,16.7074158218379));
#15526=CARTESIAN_POINT('Ctrl Pts',(2.07672674084776,1.42307556476004,16.7058342215236));
#15527=CARTESIAN_POINT('Ctrl Pts',(2.08319404391952,1.41359138423154,16.7051126441305));
#15528=CARTESIAN_POINT('Ctrl Pts',(2.09738946126581,1.39246506121984,16.7035180989009));
#15529=CARTESIAN_POINT('Ctrl Pts',(2.1050860088038,1.38080208826186,16.7026463256163));
#15530=CARTESIAN_POINT('Ctrl Pts',(2.12698956236018,1.34700167723768,16.7001437507135));
#15531=CARTESIAN_POINT('Ctrl Pts',(2.14094751390689,1.32470447247281,16.69852211908));
#15532=CARTESIAN_POINT('Ctrl Pts',(2.23694643938591,1.16586855219531,16.6871649981279));
#15533=CARTESIAN_POINT('Ctrl Pts',(2.30621050315556,1.02204210687976,16.6779144161415));
#15534=CARTESIAN_POINT('Ctrl Pts',(2.36142200368728,0.872635302117406,16.6687517122259));
#15535=CARTESIAN_POINT('Origin',(0.,0.,10.));
#15536=CARTESIAN_POINT('',(2.36142199860763,0.87263531586336,15.670984110559));
#15537=CARTESIAN_POINT('',(2.36142200728636,0.872635292378008,15.9436790867324));
#15538=CARTESIAN_POINT('',(2.36142200728636,0.87263529237802,10.));
#15539=CARTESIAN_POINT('',(2.5174993049387,0.00187073064801871,16.8874166975661));
#15540=CARTESIAN_POINT('Ctrl Pts',(2.36142200728636,0.872635292378007,15.9436790867324));
#15541=CARTESIAN_POINT('Ctrl Pts',(2.33256006636991,0.950738049679249,15.9489328860113));
#15542=CARTESIAN_POINT('Ctrl Pts',(2.29984299449287,1.02734321032059,15.9541866852901));
#15543=CARTESIAN_POINT('Ctrl Pts',(2.263465206547,1.10205785181685,15.959440484569));
#15544=CARTESIAN_POINT('Ctrl Pts',(2.22701756461404,1.17691596315821,15.9647043723894));
#15545=CARTESIAN_POINT('Ctrl Pts',(2.18689538095588,1.24987589771121,15.9699682602098));
#15546=CARTESIAN_POINT('Ctrl Pts',(2.14333851663164,1.32057042717277,15.9752321480303));
#15547=CARTESIAN_POINT('Ctrl Pts',(2.09987283734388,1.39111695968029,15.9804850160537));
#15548=CARTESIAN_POINT('Ctrl Pts',(2.05298716645419,1.45940723729897,15.9857378840772));
#15549=CARTESIAN_POINT('Ctrl Pts',(2.00295963408966,1.5251094892523,15.9909907521006));
#15550=CARTESIAN_POINT('Ctrl Pts',(1.95290942195784,1.59084152703984,15.9962460014893));
#15551=CARTESIAN_POINT('Ctrl Pts',(1.89952761462273,1.65422856365248,16.0015012508779));
#15552=CARTESIAN_POINT('Ctrl Pts',(1.84306196642989,1.71491365319061,16.0067565002666));
#15553=CARTESIAN_POINT('Ctrl Pts',(1.78667637373961,1.77551270501385,16.0120042989016));
#15554=CARTESIAN_POINT('Ctrl Pts',(1.72721593632925,1.83341708376036,16.0172520975367));
#15555=CARTESIAN_POINT('Ctrl Pts',(1.66496986958113,1.88830124275418,16.0224998961717));
#15556=CARTESIAN_POINT('Ctrl Pts',(1.6022727760879,1.9435830850858,16.0277857196598));
#15557=CARTESIAN_POINT('Ctrl Pts',(1.536749801404,1.99580037773037,16.0330715431478));
#15558=CARTESIAN_POINT('Ctrl Pts',(1.46873581844402,2.0446567794179,16.0383573666359));
#15559=CARTESIAN_POINT('Ctrl Pts',(1.40133171264408,2.09307508878655,16.0435957924731));
#15560=CARTESIAN_POINT('Ctrl Pts',(1.3314814747371,2.13819226543406,16.0488342183103));
#15561=CARTESIAN_POINT('Ctrl Pts',(1.25954438553007,2.17976012232532,16.0540726441475));
#15562=CARTESIAN_POINT('Ctrl Pts',(1.18763095527944,2.22131430821425,16.0593093471503));
#15563=CARTESIAN_POINT('Ctrl Pts',(1.11363243602454,2.25932126202357,16.0645460501531));
#15564=CARTESIAN_POINT('Ctrl Pts',(1.0379353599718,2.29357721442296,16.069782753156));
#15565=CARTESIAN_POINT('Ctrl Pts',(0.962240345915608,2.32783223368651,16.0750193135105));
#15566=CARTESIAN_POINT('Ctrl Pts',(0.884847287860035,2.35833626539672,16.080255873865));
#15567=CARTESIAN_POINT('Ctrl Pts',(0.806164213719876,2.38493302013231,16.0854924342194));
#15568=CARTESIAN_POINT('Ctrl Pts',(0.726193308647712,2.4119650924227,16.0908147030249));
#15569=CARTESIAN_POINT('Ctrl Pts',(0.644890239921313,2.4349606605837,16.0961369718304));
#15570=CARTESIAN_POINT('Ctrl Pts',(0.562699290720848,2.45380841921741,16.1014592406358));
#15571=CARTESIAN_POINT('Ctrl Pts',(0.481715787896842,2.47237929021218,16.1067033213409));
#15572=CARTESIAN_POINT('Ctrl Pts',(0.399870790227692,2.48692339010019,16.111947402046));
#15573=CARTESIAN_POINT('Ctrl Pts',(0.317597611250558,2.49738623511221,16.1171914827511));
#15574=CARTESIAN_POINT('Ctrl Pts',(0.233484419523207,2.5080830782323,16.1225528456068));
#15575=CARTESIAN_POINT('Ctrl Pts',(0.148924173671973,2.51451387293495,16.1279142084624));
#15576=CARTESIAN_POINT('Ctrl Pts',(0.0643812902686016,2.51667663784272,
16.133275571318));
#15577=CARTESIAN_POINT('Ctrl Pts',(-0.020161593134758,2.51883940275049,
16.1386369341736));
#15578=CARTESIAN_POINT('Ctrl Pts',(-0.10468660780405,2.51673421729153,16.1439982970293));
#15579=CARTESIAN_POINT('Ctrl Pts',(-0.188735569826069,2.51041533111205,
16.1493596598849));
#15580=CARTESIAN_POINT('Ctrl Pts',(-0.271121035916884,2.50422150824325,
16.1546149107186));
#15581=CARTESIAN_POINT('Ctrl Pts',(-0.353353424571359,2.49395642717338,
16.1598701615524));
#15582=CARTESIAN_POINT('Ctrl Pts',(-0.434998441876353,2.47963356275986,
16.1651254123862));
#15583=CARTESIAN_POINT('Ctrl Pts',(-0.516527705220022,2.46533100489225,
16.1703732124762));
#15584=CARTESIAN_POINT('Ctrl Pts',(-0.597470800626601,2.4469821698992,16.1756210125662));
#15585=CARTESIAN_POINT('Ctrl Pts',(-0.677397198106076,2.4246524051909,16.1808688126562));
#15586=CARTESIAN_POINT('Ctrl Pts',(-0.757902703820998,2.40216084974706,
16.1861546357817));
#15587=CARTESIAN_POINT('Ctrl Pts',(-0.837376243884293,2.37563046891055,
16.1914404589073));
#15588=CARTESIAN_POINT('Ctrl Pts',(-0.91538692772202,2.34518080807337,16.1967262820328));
#15589=CARTESIAN_POINT('Ctrl Pts',(-0.992698121574452,2.315004176926,16.2019647093382));
#15590=CARTESIAN_POINT('Ctrl Pts',(-1.06857215004843,2.28097844032329,16.2072031366436));
#15591=CARTESIAN_POINT('Ctrl Pts',(-1.14260522462048,2.24326983456515,16.2124415639489));
#15592=CARTESIAN_POINT('Ctrl Pts',(-1.21661395093089,2.20557363054778,16.2176782684217));
#15593=CARTESIAN_POINT('Ctrl Pts',(-1.2887825149814,2.1641971722119,16.2229149728944));
#15594=CARTESIAN_POINT('Ctrl Pts',(-1.35872954841789,2.11935373740584,16.2281516773671));
#15595=CARTESIAN_POINT('Ctrl Pts',(-1.42867467648605,2.07451152414209,16.2333882391912));
#15596=CARTESIAN_POINT('Ctrl Pts',(-1.49639800636966,2.02620277208412,16.2386248010153));
#15597=CARTESIAN_POINT('Ctrl Pts',(-1.56154629212837,1.97468464002234,16.2438613628393));
#15598=CARTESIAN_POINT('Ctrl Pts',(-1.62776084044333,1.92232332606336,16.2491836299085));
#15599=CARTESIAN_POINT('Ctrl Pts',(-1.69131490038314,1.86664692509891,16.2545058969776));
#15600=CARTESIAN_POINT('Ctrl Pts',(-1.75187321961527,1.80796749760465,16.2598281640467));
#15601=CARTESIAN_POINT('Ctrl Pts',(-1.81154192795574,1.75015007979753,16.2650722462056));
#15602=CARTESIAN_POINT('Ctrl Pts',(-1.8683020524125,1.68941766349438,16.2703163283645));
#15603=CARTESIAN_POINT('Ctrl Pts',(-1.92187197401931,1.62610404509648,16.2755604105234));
#15604=CARTESIAN_POINT('Ctrl Pts',(-1.97663992019507,1.56137449648783,16.2809217700477));
#15605=CARTESIAN_POINT('Ctrl Pts',(-2.02807294138086,1.49394730907183,16.2862831295719));
#15606=CARTESIAN_POINT('Ctrl Pts',(-2.07591652376069,1.42421095220383,16.2916444890962));
#15607=CARTESIAN_POINT('Ctrl Pts',(-2.12376010614051,1.35447459533585,16.2970058486204));
#15608=CARTESIAN_POINT('Ctrl Pts',(-2.1680140406906,1.28242953692711,16.3023672081447));
#15609=CARTESIAN_POINT('Ctrl Pts',(-2.20847437293236,1.20848963342721,16.3077285676689));
#15610=CARTESIAN_POINT('Ctrl Pts',(-2.24813390682169,1.13601316212423,16.3129838141774));
#15611=CARTESIAN_POINT('Ctrl Pts',(-2.28429516385635,1.06144849006884,16.3182390606859));
#15612=CARTESIAN_POINT('Ctrl Pts',(-2.31673299462772,0.985167235348021,
16.3234943071943));
#15613=CARTESIAN_POINT('Ctrl Pts',(-2.34912483590618,0.908994130159408,
16.3287421029542));
#15614=CARTESIAN_POINT('Ctrl Pts',(-2.37780355744491,0.831109697474887,
16.3339898987141));
#15615=CARTESIAN_POINT('Ctrl Pts',(-2.40258956938183,0.751910640367356,
16.3392376944739));
#15616=CARTESIAN_POINT('Ctrl Pts',(-2.42755519455052,0.672137662830976,
16.3445235186814));
#15617=CARTESIAN_POINT('Ctrl Pts',(-2.44857122708091,0.591031343189288,
16.3498093428889));
#15618=CARTESIAN_POINT('Ctrl Pts',(-2.46550334123449,0.509018196493554,
16.3550951670963));
#15619=CARTESIAN_POINT('Ctrl Pts',(-2.48228361478307,0.427740511754887,
16.360333590091));
#15620=CARTESIAN_POINT('Ctrl Pts',(-2.49505282753447,0.345572659178892,
16.3655720130857));
#15621=CARTESIAN_POINT('Ctrl Pts',(-2.50373057391308,0.262943840492387,
16.3708104360804));
#15622=CARTESIAN_POINT('Ctrl Pts',(-2.51240546634888,0.180342196824877,
16.3760471362592));
#15623=CARTESIAN_POINT('Ctrl Pts',(-2.51699151669958,0.0972803466739266,
16.381283836438));
#15624=CARTESIAN_POINT('Ctrl Pts',(-2.51745998417278,0.0141942977555527,
16.3865205366168));
#15625=CARTESIAN_POINT('Ctrl Pts',(-2.51792843888685,-0.0688894882392182,
16.3917570941693));
#15626=CARTESIAN_POINT('Ctrl Pts',(-2.51427953212815,-0.151997010271273,
16.3969936517218));
#15627=CARTESIAN_POINT('Ctrl Pts',(-2.50653664139236,-0.23469195844231,
16.4022302092743));
#15628=CARTESIAN_POINT('Ctrl Pts',(-2.49866701109522,-0.318740499452894,
16.4075524814559));
#15629=CARTESIAN_POINT('Ctrl Pts',(-2.48656819550601,-0.402362347490421,
16.4128747536375));
#15630=CARTESIAN_POINT('Ctrl Pts',(-2.47031942034519,-0.485106391903289,
16.4181970258191));
#15631=CARTESIAN_POINT('Ctrl Pts',(-2.45430937027496,-0.566634770562661,
16.4234411038047));
#15632=CARTESIAN_POINT('Ctrl Pts',(-2.43427066495096,-0.647310528120108,
16.4286851817903));
#15633=CARTESIAN_POINT('Ctrl Pts',(-2.41032996240741,-0.726715709422255,
16.4339292597759));
#15634=CARTESIAN_POINT('Ctrl Pts',(-2.38585379185858,-0.807896901013318,
16.4392906290555));
#15635=CARTESIAN_POINT('Ctrl Pts',(-2.35729914260083,-0.887749511803182,
16.444651998335));
#15636=CARTESIAN_POINT('Ctrl Pts',(-2.32485329087844,-0.965848552254288,
16.4500133676146));
#15637=CARTESIAN_POINT('Ctrl Pts',(-2.29240743915605,-1.04394759270539,
16.4553747368941));
#15638=CARTESIAN_POINT('Ctrl Pts',(-2.25607066365104,-1.1202926327294,16.4607361061737));
#15639=CARTESIAN_POINT('Ctrl Pts',(-2.2160790626755,-1.19448726990759,16.4660974754532));
#15640=CARTESIAN_POINT('Ctrl Pts',(-2.17687902638735,-1.2672133523555,16.4713527256854));
#15641=CARTESIAN_POINT('Ctrl Pts',(-2.13402277703882,-1.33814202835465,
16.4766079759176));
#15642=CARTESIAN_POINT('Ctrl Pts',(-2.08769944242106,-1.40688211592685,
16.4818632261498));
#15643=CARTESIAN_POINT('Ctrl Pts',(-2.04144178397511,-1.47552474536399,
16.4871110256075));
#15644=CARTESIAN_POINT('Ctrl Pts',(-1.99172705969588,-1.54198457024853,
16.4923588250653));
#15645=CARTESIAN_POINT('Ctrl Pts',(-1.93879024342378,-1.60589496605624,
16.497606624523));
#15646=CARTESIAN_POINT('Ctrl Pts',(-1.88546986446111,-1.67026843548827,
16.5028924478028));
#15647=CARTESIAN_POINT('Ctrl Pts',(-1.8288807289112,-1.73205495816942,16.5081782710826));
#15648=CARTESIAN_POINT('Ctrl Pts',(-1.76930746003082,-1.79090964648674,
16.5134640943623));
#15649=CARTESIAN_POINT('Ctrl Pts',(-1.71026836998505,-1.84923659930446,
16.5187025209661));
#15650=CARTESIAN_POINT('Ctrl Pts',(-1.64829878254551,-1.90468375498875,
16.52394094757));
#15651=CARTESIAN_POINT('Ctrl Pts',(-1.58371493216762,-1.95694999006855,
16.5291793741738));
#15652=CARTESIAN_POINT('Ctrl Pts',(-1.51915232265853,-2.00919903539836,
16.5344160779207));
#15653=CARTESIAN_POINT('Ctrl Pts',(-1.45197751621885,-2.05826894782693,
16.5396527816677));
#15654=CARTESIAN_POINT('Ctrl Pts',(-1.3825405850962,-2.10389823436445,16.5448894854146));
#15655=CARTESIAN_POINT('Ctrl Pts',(-1.3131055457531,-2.14952627775153,16.5501260464898));
#15656=CARTESIAN_POINT('Ctrl Pts',(-1.24140889044425,-2.19171362908595,
16.5553626075649));
#15657=CARTESIAN_POINT('Ctrl Pts',(-1.16782932078672,-2.23024234725979,
16.5605991686401));
#15658=CARTESIAN_POINT('Ctrl Pts',(-1.09304547413255,-2.26940166505825,
16.5659214365232));
#15659=CARTESIAN_POINT('Ctrl Pts',(-1.01631695125543,-2.30478126775819,
16.5712437044063));
#15660=CARTESIAN_POINT('Ctrl Pts',(-0.938065273354438,-2.33620200173839,
16.5765659722894));
#15661=CARTESIAN_POINT('Ctrl Pts',(-0.860963147983039,-2.36716115092965,
16.5818100536509));
#15662=CARTESIAN_POINT('Ctrl Pts',(-0.782382784649652,-2.39427687982042,
16.5870541350123));
#15663=CARTESIAN_POINT('Ctrl Pts',(-0.702743720441128,-2.41742787139153,
16.5922982163738));
#15664=CARTESIAN_POINT('Ctrl Pts',(-0.621323590783215,-2.44109661680136,
16.5976595775177));
#15665=CARTESIAN_POINT('Ctrl Pts',(-0.538797333086823,-2.46062103062427,
16.6030209386616));
#15666=CARTESIAN_POINT('Ctrl Pts',(-0.455623385630417,-2.4759268124213,
16.6083822998056));
#15667=CARTESIAN_POINT('Ctrl Pts',(-0.372449438174011,-2.49123259421832,
16.6137436609495));
#15668=CARTESIAN_POINT('Ctrl Pts',(-0.288628313434993,-2.50231974358233,
16.6191050220934));
#15669=CARTESIAN_POINT('Ctrl Pts',(-0.204621052373853,-2.50917047546105,
16.6244663832373));
#15670=CARTESIAN_POINT('Ctrl Pts',(-0.122276319118097,-2.51588562938981,
16.6297216415056));
#15671=CARTESIAN_POINT('Ctrl Pts',(-0.0394486079889621,-2.51855536563663,
16.6349768997738));
#15672=CARTESIAN_POINT('Ctrl Pts',(0.0434309883450006,-2.51712534436634,
16.6402321580421));
#15673=CARTESIAN_POINT('Ctrl Pts',(0.126193081175941,-2.5156973505252,16.6454799656073));
#15674=CARTESIAN_POINT('Ctrl Pts',(0.209006455596838,-2.51018115234066,
16.6507277731726));
#15675=CARTESIAN_POINT('Ctrl Pts',(0.29143565672779,-2.50057423564821,16.6559755807379));
#15676=CARTESIAN_POINT('Ctrl Pts',(0.374461952664628,-2.49089772905342,
16.6612614019997));
#15677=CARTESIAN_POINT('Ctrl Pts',(0.457098013823339,-2.47707095133006,
16.6665472232615));
#15678=CARTESIAN_POINT('Ctrl Pts',(0.538899589046655,-2.45914486822663,
16.6718330445233));
#15679=CARTESIAN_POINT('Ctrl Pts',(0.619967827861354,-2.44137948923393,
16.6770714793483));
#15680=CARTESIAN_POINT('Ctrl Pts',(0.700216023835672,-2.41958811021566,
16.6823099141732));
#15681=CARTESIAN_POINT('Ctrl Pts',(0.779219421588435,-2.39387203981737,
16.6875483489982));
#15682=CARTESIAN_POINT('Ctrl Pts',(0.858196836457926,-2.36816442700034,
16.6927850609904));
#15683=CARTESIAN_POINT('Ctrl Pts',(0.935929827769396,-2.33853482903941,
16.6980217729826));
#15684=CARTESIAN_POINT('Ctrl Pts',(1.01200845890472,-2.30513451431913,16.7032584849748));
#15685=CARTESIAN_POINT('Ctrl Pts',(1.08808501750054,-2.27173510949261,16.7084950543081));
#15686=CARTESIAN_POINT('Ctrl Pts',(1.16250688344625,-2.23456537857441,16.7137316236414));
#15687=CARTESIAN_POINT('Ctrl Pts',(1.2348850638382,-2.19382431591715,16.7189681929747));
#15688=CARTESIAN_POINT('Ctrl Pts',(1.30844760783264,-2.15241658505302,16.7242904511453));
#15689=CARTESIAN_POINT('Ctrl Pts',(1.37989854415171,-2.10731981863762,16.7296127093159));
#15690=CARTESIAN_POINT('Ctrl Pts',(1.44885810514049,-2.0587900430031,16.7349349674864));
#15691=CARTESIAN_POINT('Ctrl Pts',(1.51680484930424,-2.01097302963929,16.7401790570529));
#15692=CARTESIAN_POINT('Ctrl Pts',(1.58233258353913,-1.95982351619309,16.7454231466194));
#15693=CARTESIAN_POINT('Ctrl Pts',(1.64511112944355,-1.9056273564842,16.7506672361858));
#15694=CARTESIAN_POINT('Ctrl Pts',(1.70929334453757,-1.85021942166199,16.7560285786584));
#15695=CARTESIAN_POINT('Ctrl Pts',(1.77060157946887,-1.79162731043557,16.7613899211311));
#15696=CARTESIAN_POINT('Ctrl Pts',(1.82872391766773,-1.73019509967807,16.7667512636037));
#15697=CARTESIAN_POINT('Ctrl Pts',(1.88684625586659,-1.66876288892055,16.7721126060763));
#15698=CARTESIAN_POINT('Ctrl Pts',(1.94178241797934,-1.60449100825937,16.7774739485489));
#15699=CARTESIAN_POINT('Ctrl Pts',(1.99326647407452,-1.53775648700648,16.7828352910216));
#15700=CARTESIAN_POINT('Ctrl Pts',(2.04375865853867,-1.47230764686464,16.788093343973));
#15701=CARTESIAN_POINT('Ctrl Pts',(2.0911200889309,-1.4042446607204,16.7933513969245));
#15702=CARTESIAN_POINT('Ctrl Pts',(2.13506909127537,-1.3338988812802,16.7986094498759));
#15703=CARTESIAN_POINT('Ctrl Pts',(2.17895674914168,-1.26365129121632,16.8038601635819));
#15704=CARTESIAN_POINT('Ctrl Pts',(2.21944119444765,-1.19112762062856,16.8091108772879));
#15705=CARTESIAN_POINT('Ctrl Pts',(2.25628160460562,-1.11669134980006,16.8143615909939));
#15706=CARTESIAN_POINT('Ctrl Pts',(2.29308163742164,-1.04233666163441,16.8196065498817));
#15707=CARTESIAN_POINT('Ctrl Pts',(2.32624536463931,-0.966073946613376,
16.8248515087695));
#15708=CARTESIAN_POINT('Ctrl Pts',(2.35557655574188,-0.888293498816241,
16.8300964676574));
#15709=CARTESIAN_POINT('Ctrl Pts',(2.3848851679442,-0.810572925743141,16.8353373890206));
#15710=CARTESIAN_POINT('Ctrl Pts',(2.41036694330135,-0.73133737020881,16.8405783103839));
#15711=CARTESIAN_POINT('Ctrl Pts',(2.43187326239833,-0.65099822244927,16.8458192317472));
#15712=CARTESIAN_POINT('Ctrl Pts',(2.45336962702427,-0.570696260677519,
16.8510577272839));
#15713=CARTESIAN_POINT('Ctrl Pts',(2.47089407458419,-0.489292166094003,
16.8562962228207));
#15714=CARTESIAN_POINT('Ctrl Pts',(2.48434787328852,-0.407212345695463,
16.8615347183574));
#15715=CARTESIAN_POINT('Ctrl Pts',(2.49780301782331,-0.325124314565895,
16.8667737379191));
#15716=CARTESIAN_POINT('Ctrl Pts',(2.50718661818065,-0.242360875602271,
16.8720127574809));
#15717=CARTESIAN_POINT('Ctrl Pts',(2.51245128260683,-0.159357467748757,
16.8772517770426));
#15718=CARTESIAN_POINT('Ctrl Pts',(2.51585617510238,-0.10567547443881,16.8806400838644));
#15719=CARTESIAN_POINT('Ctrl Pts',(2.51753925645563,-0.0518932709951306,
16.8840283906862));
#15720=CARTESIAN_POINT('Ctrl Pts',(2.51749930493939,0.00187072972653814,
16.887416697508));
#15721=CARTESIAN_POINT('Ctrl Pts',(2.5174993049387,0.00187073064803274,
16.8874166975661));
#15722=CARTESIAN_POINT('Ctrl Pts',(2.51742785555538,0.0980223455464406,
16.8934763502764));
#15723=CARTESIAN_POINT('Ctrl Pts',(2.51184391185846,0.193950007534804,16.8995360029868));
#15724=CARTESIAN_POINT('Ctrl Pts',(2.50084792088994,0.289077717198135,16.9055956556972));
#15725=CARTESIAN_POINT('Ctrl Pts',(2.4897455630997,0.385125619699227,16.9117139248616));
#15726=CARTESIAN_POINT('Ctrl Pts',(2.47312604616118,0.480357869841915,16.917832194026));
#15727=CARTESIAN_POINT('Ctrl Pts',(2.45114240622494,0.574201318707828,16.9239504631905));
#15728=CARTESIAN_POINT('Ctrl Pts',(2.43047752529607,0.662415267917,16.9297017083956));
#15729=CARTESIAN_POINT('Ctrl Pts',(2.4050733126551,0.749402139891612,16.9354529536007));
#15730=CARTESIAN_POINT('Ctrl Pts',(2.37509512959371,0.834703166029845,16.9412041988058));
#15731=CARTESIAN_POINT('Ctrl Pts',(2.37064009567936,0.847379683602514,16.9420588867762));
#15732=CARTESIAN_POINT('Ctrl Pts',(2.36608223827853,0.860024328645438,16.9429135747467));
#15733=CARTESIAN_POINT('Ctrl Pts',(2.36142200728636,0.872635292378013,16.9437682627171));
#15734=CARTESIAN_POINT('',(2.51750016131132,0.00131518048836379,16.6143270326092));
#15735=CARTESIAN_POINT('Ctrl Pts',(2.36142200368728,0.872635302117405,16.6687517122259));
#15736=CARTESIAN_POINT('Ctrl Pts',(2.36386197625392,0.866032538175512,16.6683467830721));
#15737=CARTESIAN_POINT('Ctrl Pts',(2.36627450067557,0.859418878191297,16.6679419651352));
#15738=CARTESIAN_POINT('Ctrl Pts',(2.40176087186149,0.760854533318875,16.6619195611102));
#15739=CARTESIAN_POINT('Ctrl Pts',(2.42947996278743,0.667068696889583,16.6563300599534));
#15740=CARTESIAN_POINT('Ctrl Pts',(2.46403571560758,0.518935114137275,16.6474234120279));
#15741=CARTESIAN_POINT('Ctrl Pts',(2.47467296806581,0.465573459107778,16.6441989244266));
#15742=CARTESIAN_POINT('Ctrl Pts',(2.48911195965705,0.378515460182014,16.6388530720024));
#15743=CARTESIAN_POINT('Ctrl Pts',(2.49397652107123,0.34501182288473,16.6367754829283));
#15744=CARTESIAN_POINT('Ctrl Pts',(2.49954909251244,0.300309820509292,16.633964475721));
#15745=CARTESIAN_POINT('Ctrl Pts',(2.5008601765897,0.289188555031691,16.6332619344937));
#15746=CARTESIAN_POINT('Ctrl Pts',(2.50287375753636,0.271069479635317,16.6321115906921));
#15747=CARTESIAN_POINT('Ctrl Pts',(2.50362121993825,0.264076680409275,16.6316662412482));
#15748=CARTESIAN_POINT('Ctrl Pts',(2.50496858734813,0.250951377569079,16.6308275702593));
#15749=CARTESIAN_POINT('Ctrl Pts',(2.50557529337874,0.244819655441212,16.6304346320055));
#15750=CARTESIAN_POINT('Ctrl Pts',(2.5067905206519,0.232059984209922,16.629614669477));
#15751=CARTESIAN_POINT('Ctrl Pts',(2.5073952811417,0.22543170232375,16.6291874416678));
#15752=CARTESIAN_POINT('Ctrl Pts',(2.50876413858236,0.209741392274904,16.6281732117087));
#15753=CARTESIAN_POINT('Ctrl Pts',(2.50950542443588,0.200677536296804,16.6275850269434));
#15754=CARTESIAN_POINT('Ctrl Pts',(2.51192971671358,0.168917963066522,16.6255164749279));
#15755=CARTESIAN_POINT('Ctrl Pts',(2.51335401207864,0.146204337379204,16.624023585749));
#15756=CARTESIAN_POINT('Ctrl Pts',(2.51646841711688,0.0827821850118265,
16.6198230050186));
#15757=CARTESIAN_POINT('Ctrl Pts',(2.51747843504179,0.0420488464344308,
16.6170884128516));
#15758=CARTESIAN_POINT('Ctrl Pts',(2.51749965834993,0.0013115669903107,
16.614327662638));
#15759=CARTESIAN_POINT('Ctrl Pts',(2.51749965649576,0.0013151211919122,
16.6143279035048));
#15760=CARTESIAN_POINT('Ctrl Pts',(2.51759289161941,-0.177162264168698,
16.6022325643764));
#15761=CARTESIAN_POINT('Ctrl Pts',(2.49870710678302,-0.355153439427492,
16.5897184849106));
#15762=CARTESIAN_POINT('Ctrl Pts',(2.43726528490359,-0.640649853452946,
16.5698726053172));
#15763=CARTESIAN_POINT('Ctrl Pts',(2.40589806630083,-0.749903381947059,
16.5623241462808));
#15764=CARTESIAN_POINT('Ctrl Pts',(2.35938061982181,-0.878444698619027,
16.5535212616552));
#15765=CARTESIAN_POINT('Ctrl Pts',(2.35120419892183,-0.900100478352394,
16.552040602573));
#15766=CARTESIAN_POINT('Ctrl Pts',(2.33785941558209,-0.934021738630407,
16.5497244548122));
#15767=CARTESIAN_POINT('Ctrl Pts',(2.3328906417668,-0.946363841163944,16.5488823916523));
#15768=CARTESIAN_POINT('Ctrl Pts',(2.32340323799045,-0.969401065830408,
16.5473116667831));
#15769=CARTESIAN_POINT('Ctrl Pts',(2.31890803128904,-0.980105393528043,
16.5465822450454));
#15770=CARTESIAN_POINT('Ctrl Pts',(2.30867634272983,-1.00400538456234,16.5449543920492));
#15771=CARTESIAN_POINT('Ctrl Pts',(2.30290042967158,-1.0171838045857,16.5440573176961));
#15772=CARTESIAN_POINT('Ctrl Pts',(2.28791197026316,-1.05059956672344,16.5417835160231));
#15773=CARTESIAN_POINT('Ctrl Pts',(2.27854360037989,-1.07076596078246,16.5404120938657));
#15774=CARTESIAN_POINT('Ctrl Pts',(2.19810978992022,-1.23807067337564,16.5290344982388));
#15775=CARTESIAN_POINT('Ctrl Pts',(2.11313902604193,-1.378099666811,16.5195468522991));
#15776=CARTESIAN_POINT('Ctrl Pts',(1.93712822666715,-1.61316467487242,16.5026564872387));
#15777=CARTESIAN_POINT('Ctrl Pts',(1.85110631844529,-1.71118874366793,16.4952363316092));
#15778=CARTESIAN_POINT('Ctrl Pts',(1.73000489045211,-1.82931884466891,16.4851849149801));
#15779=CARTESIAN_POINT('Ctrl Pts',(1.70148750335004,-1.85587292589741,16.4828423303225));
#15780=CARTESIAN_POINT('Ctrl Pts',(1.6592958469584,-1.89336983817612,16.4793911610366));
#15781=CARTESIAN_POINT('Ctrl Pts',(1.64610441488601,-1.90484967149928,16.4783141319773));
#15782=CARTESIAN_POINT('Ctrl Pts',(1.62516539795622,-1.92269190255638,16.4766056776944));
#15783=CARTESIAN_POINT('Ctrl Pts',(1.617497324431,-1.92914725222831,16.4759802597479));
#15784=CARTESIAN_POINT('Ctrl Pts',(1.60315590119635,-1.94107493017673,16.4748105475923));
#15785=CARTESIAN_POINT('Ctrl Pts',(1.59649253495555,-1.9465590946027,16.4742670686335));
#15786=CARTESIAN_POINT('Ctrl Pts',(1.58480568065266,-1.95607737918198,16.4733135929471));
#15787=CARTESIAN_POINT('Ctrl Pts',(1.57979459138374,-1.96012673239326,16.4729046728288));
#15788=CARTESIAN_POINT('Ctrl Pts',(1.56916424229675,-1.96864964341147,16.4720369042345));
#15789=CARTESIAN_POINT('Ctrl Pts',(1.5635413554041,-1.97311841121173,16.4715777422625));
#15790=CARTESIAN_POINT('Ctrl Pts',(1.54857089409316,-1.98491195428991,16.4703550169703));
#15791=CARTESIAN_POINT('Ctrl Pts',(1.53919061363268,-1.99219464964125,16.4695886228376));
#15792=CARTESIAN_POINT('Ctrl Pts',(1.49828695429828,-2.02349025176069,16.4662468719358));
#15793=CARTESIAN_POINT('Ctrl Pts',(1.4662523367576,-2.04682199414114,16.463630243415));
#15794=CARTESIAN_POINT('Ctrl Pts',(1.28087937831617,-2.17524942720514,16.4485512790733));
#15795=CARTESIAN_POINT('Ctrl Pts',(1.11682524071258,-2.26386031841253,16.4354948518298));
#15796=CARTESIAN_POINT('Ctrl Pts',(0.834698003934132,-2.37804964211992,
16.4146975686557));
#15797=CARTESIAN_POINT('Ctrl Pts',(0.721871972396797,-2.4146942946323,16.4067595857975));
#15798=CARTESIAN_POINT('Ctrl Pts',(0.577102821528507,-2.45065283711551,
16.397085751441));
#15799=CARTESIAN_POINT('Ctrl Pts',(0.547202113978372,-2.45750218245596,
16.3951137372499));
#15800=CARTESIAN_POINT('Ctrl Pts',(0.50265464564233,-2.46685324216732,16.3922130129569));
#15801=CARTESIAN_POINT('Ctrl Pts',(0.488099766178357,-2.46977433074594,
16.3912711175394));
#15802=CARTESIAN_POINT('Ctrl Pts',(0.46207588530407,-2.47475814754733,16.3895971989709));
#15803=CARTESIAN_POINT('Ctrl Pts',(0.450616899134009,-2.47687028933969,
16.3888636344728));
#15804=CARTESIAN_POINT('Ctrl Pts',(0.426333297382346,-2.48117218687824,
16.3873163189472));
#15805=CARTESIAN_POINT('Ctrl Pts',(0.413505505118304,-2.48334224559086,
16.3865032078872));
#15806=CARTESIAN_POINT('Ctrl Pts',(0.379149894493703,-2.48888054598132,
16.3843365400638));
#15807=CARTESIAN_POINT('Ctrl Pts',(0.357593902639592,-2.49206895198495,
16.3829886410434));
#15808=CARTESIAN_POINT('Ctrl Pts',(0.257918958424257,-2.50549218156433,
16.3768057569194));
#15809=CARTESIAN_POINT('Ctrl Pts',(0.179383957081291,-2.51233685060237,
16.372076860921));
#15810=CARTESIAN_POINT('Ctrl Pts',(-0.0661259408356384,-2.52216032100304,
16.35757867813));
#15811=CARTESIAN_POINT('Ctrl Pts',(-0.233148880538158,-2.51223152947583,
16.3481491135309));
#15812=CARTESIAN_POINT('Ctrl Pts',(-0.49975620372696,-2.4695501001532,16.3325004386518));
#15813=CARTESIAN_POINT('Ctrl Pts',(-0.600442451799385,-2.44701817055557,
16.3264382890751));
#15814=CARTESIAN_POINT('Ctrl Pts',(-0.716675633348967,-2.41340087224932,
16.318969233596));
#15815=CARTESIAN_POINT('Ctrl Pts',(-0.733845391944648,-2.40823558480896,
16.3178535163201));
#15816=CARTESIAN_POINT('Ctrl Pts',(-0.759014912144487,-2.40036952742121,
16.3161976698582));
#15817=CARTESIAN_POINT('Ctrl Pts',(-0.767059028962156,-2.39781107392871,
16.3156653967585));
#15818=CARTESIAN_POINT('Ctrl Pts',(-0.781298646312219,-2.39320313790047,
16.3147174713582));
#15819=CARTESIAN_POINT('Ctrl Pts',(-0.787499246513019,-2.39116995827077,
16.31430276528));
#15820=CARTESIAN_POINT('Ctrl Pts',(-0.800938615137099,-2.38670523818564,
16.313399650953));
#15821=CARTESIAN_POINT('Ctrl Pts',(-0.808174134120746,-2.38426490232591,
16.3129107568972));
#15822=CARTESIAN_POINT('Ctrl Pts',(-0.828238283458461,-2.37739600880764,
16.3115478337123));
#15823=CARTESIAN_POINT('Ctrl Pts',(-0.841042153799331,-2.37289665032012,
16.3106698685911));
#15824=CARTESIAN_POINT('Ctrl Pts',(-0.912313496079961,-2.34720216820449,
16.3057391968499));
#15825=CARTESIAN_POINT('Ctrl Pts',(-0.970011692361758,-2.32395135073942,
16.3015835485047));
#15826=CARTESIAN_POINT('Ctrl Pts',(-1.18887120298118,-2.22618642353206,
16.2853308152295));
#15827=CARTESIAN_POINT('Ctrl Pts',(-1.34284623923541,-2.13684099658062,
16.2728867280455));
#15828=CARTESIAN_POINT('Ctrl Pts',(-1.57768099278886,-1.96509257177471,
16.2531161751137));
#15829=CARTESIAN_POINT('Ctrl Pts',(-1.66459649026258,-1.89203354085314,
16.2455762824394));
#15830=CARTESIAN_POINT('Ctrl Pts',(-1.76296726235267,-1.79730024189398,
16.236781824801));
#15831=CARTESIAN_POINT('Ctrl Pts',(-1.77941358195077,-1.781019115675,16.2353015455611));
#15832=CARTESIAN_POINT('Ctrl Pts',(-1.80495763932047,-1.75502454158789,
16.2329858561261));
#15833=CARTESIAN_POINT('Ctrl Pts',(-1.81420652360025,-1.74546209414179,
16.2321438757622));
#15834=CARTESIAN_POINT('Ctrl Pts',(-1.83138425864606,-1.72741793794416,
16.2305732280437));
#15835=CARTESIAN_POINT('Ctrl Pts',(-1.8393310385493,-1.71895386006696,16.2298438013301));
#15836=CARTESIAN_POINT('Ctrl Pts',(-1.85699579174829,-1.69987645027589,
16.2282158385925));
#15837=CARTESIAN_POINT('Ctrl Pts',(-1.86668194087161,-1.68923410514482,
16.2273186603392));
#15838=CARTESIAN_POINT('Ctrl Pts',(-1.89110495250793,-1.66193349557615,
16.22504440843));
#15839=CARTESIAN_POINT('Ctrl Pts',(-1.90571347972684,-1.64516171444362,
16.2236726436586));
#15840=CARTESIAN_POINT('Ctrl Pts',(-2.02160224910991,-1.50849664043799,
16.2126904082288));
#15841=CARTESIAN_POINT('Ctrl Pts',(-2.11169609937389,-1.37956020168648,
16.2035542764276));
#15842=CARTESIAN_POINT('Ctrl Pts',(-2.24505023613386,-1.14470424688722,
16.1880088556805));
#15843=CARTESIAN_POINT('Ctrl Pts',(-2.29420258616721,-1.0427036265657,16.1815602012426));
#15844=CARTESIAN_POINT('Ctrl Pts',(-2.36605453057775,-0.863690071597645,
16.1702479232374));
#15845=CARTESIAN_POINT('Ctrl Pts',(-2.39223888327035,-0.788267117122985,
16.1654812347327));
#15846=CARTESIAN_POINT('Ctrl Pts',(-2.41875379370783,-0.698306789192273,
16.1596578469722));
#15847=CARTESIAN_POINT('Ctrl Pts',(-2.4225999686992,-0.684844257639382,
16.15878280108));
#15848=CARTESIAN_POINT('Ctrl Pts',(-2.42837278742728,-0.663980670796985,
16.157420178114));
#15849=CARTESIAN_POINT('Ctrl Pts',(-2.43037840550998,-0.656601498836276,
16.1569369817138));
#15850=CARTESIAN_POINT('Ctrl Pts',(-2.43403284599777,-0.642909730771618,
16.1560379115385));
#15851=CARTESIAN_POINT('Ctrl Pts',(-2.43569077904126,-0.636599750950935,
16.1556225619017));
#15852=CARTESIAN_POINT('Ctrl Pts',(-2.43943364212482,-0.622125991391422,
16.1546675670903));
#15853=CARTESIAN_POINT('Ctrl Pts',(-2.44150212120969,-0.613958166933839,
16.1541270108892));
#15854=CARTESIAN_POINT('Ctrl Pts',(-2.44684419526516,-0.592409898267039,
16.152696900001));
#15855=CARTESIAN_POINT('Ctrl Pts',(-2.4500489862197,-0.579012908933841,
16.1518036977012));
#15856=CARTESIAN_POINT('Ctrl Pts',(-2.47885905152827,-0.454054642828202,
16.1434388881598));
#15857=CARTESIAN_POINT('Ctrl Pts',(-2.49693503496261,-0.340906659924204,
16.1356215462103));
#15858=CARTESIAN_POINT('Ctrl Pts',(-2.52728333596821,-0.0056107239324921,
16.1124169950894));
#15859=CARTESIAN_POINT('Ctrl Pts',(-2.51792543437029,0.217445891382168,
16.0970339492602));
#15860=CARTESIAN_POINT('Ctrl Pts',(-2.47391616444877,0.467484091589759,
16.0805566478802));
#15861=CARTESIAN_POINT('Ctrl Pts',(-2.46786025408798,0.498466125902654,
16.0785261406324));
#15862=CARTESIAN_POINT('Ctrl Pts',(-2.45806615829862,0.544005919350389,
16.075556852166));
#15863=CARTESIAN_POINT('Ctrl Pts',(-2.45477796215965,0.558656290817961,
16.0746039641146));
#15864=CARTESIAN_POINT('Ctrl Pts',(-2.44870107279725,0.58464136612793,16.0729177681316));
#15865=CARTESIAN_POINT('Ctrl Pts',(-2.44596427222349,0.595987631851077,
16.0721828339529));
#15866=CARTESIAN_POINT('Ctrl Pts',(-2.44003290182603,0.619848772653278,
16.0706399172626));
#15867=CARTESIAN_POINT('Ctrl Pts',(-2.43682072120239,0.632358953098329,
16.0698325210998));
#15868=CARTESIAN_POINT('Ctrl Pts',(-2.42804166570517,0.66548935126612,16.0676980711492));
#15869=CARTESIAN_POINT('Ctrl Pts',(-2.42230834459651,0.686064671963054,
16.0663763776353));
#15870=CARTESIAN_POINT('Ctrl Pts',(-2.3954430660026,0.777938651026193,16.0604890705995));
#15871=CARTESIAN_POINT('Ctrl Pts',(-2.37141908583245,0.848356695051183,
16.0560171969866));
#15872=CARTESIAN_POINT('Ctrl Pts',(-2.27493468183705,1.09485429123281,16.0403612520508));
#15873=CARTESIAN_POINT('Ctrl Pts',(-2.18568686480429,1.26364718455792,16.0296822624048));
#15874=CARTESIAN_POINT('Ctrl Pts',(-2.02710574017071,1.49561652745872,16.0132887333093));
#15875=CARTESIAN_POINT('Ctrl Pts',(-1.97193758034223,1.56763674165819,16.0079048511246));
#15876=CARTESIAN_POINT('Ctrl Pts',(-1.90366402768768,1.64744540558377,16.0013874995212));
#15877=CARTESIAN_POINT('Ctrl Pts',(-1.8942216302322,1.65829354691348,16.0004890691247));
#15878=CARTESIAN_POINT('Ctrl Pts',(-1.87956350060414,1.67484537192479,15.9990977580429));
#15879=CARTESIAN_POINT('Ctrl Pts',(-1.874413406773,1.68060713713614,15.9986095550046));
#15880=CARTESIAN_POINT('Ctrl Pts',(-1.86487219101607,1.69118314201114,15.9977060506394));
#15881=CARTESIAN_POINT('Ctrl Pts',(-1.86048882638238,1.69600413692736,15.9972913185129));
#15882=CARTESIAN_POINT('Ctrl Pts',(-1.85046865409002,1.70693912124457,15.9963440708932));
#15883=CARTESIAN_POINT('Ctrl Pts',(-1.84482026449249,1.71304220334033,15.9958107020503));
#15884=CARTESIAN_POINT('Ctrl Pts',(-1.82998774095959,1.72891029914376,15.99441190415));
#15885=CARTESIAN_POINT('Ctrl Pts',(-1.82075580039909,1.73862999268947,15.9935430719766));
#15886=CARTESIAN_POINT('Ctrl Pts',(-1.75162844533053,1.81025517568678,15.9870537318084));
#15887=CARTESIAN_POINT('Ctrl Pts',(-1.68867429811614,1.86911797805562,15.9812357022869));
#15888=CARTESIAN_POINT('Ctrl Pts',(-1.50478902899741,2.02416860962639,15.9647659885821));
#15889=CARTESIAN_POINT('Ctrl Pts',(-1.37782621288012,2.11264005859239,15.9539931270428));
#15890=CARTESIAN_POINT('Ctrl Pts',(-1.14721582443178,2.24365314824624,15.9359872780276));
#15891=CARTESIAN_POINT('Ctrl Pts',(-1.04735623476565,2.29197172313424,15.9286265249638));
#15892=CARTESIAN_POINT('Ctrl Pts',(-0.923290051217735,2.34219373005328,
15.92000857197));
#15893=CARTESIAN_POINT('Ctrl Pts',(-0.901837712462627,2.35053712704448,
15.9185363874946));
#15894=CARTESIAN_POINT('Ctrl Pts',(-0.867835234898131,2.36322756249511,
15.9162304451631));
#15895=CARTESIAN_POINT('Ctrl Pts',(-0.855360380794269,2.36777134390335,
15.9153902091923));
#15896=CARTESIAN_POINT('Ctrl Pts',(-0.831907616156793,2.37610412618105,
15.9138211480979));
#15897=CARTESIAN_POINT('Ctrl Pts',(-0.82093834970085,2.37991624506652,15.9130915780007));
#15898=CARTESIAN_POINT('Ctrl Pts',(-0.796282577539754,2.38829404754364,
15.9114611588432));
#15899=CARTESIAN_POINT('Ctrl Pts',(-0.782582338762797,2.39281827508362,
15.9105616863973));
#15900=CARTESIAN_POINT('Ctrl Pts',(-0.747547802876016,2.40405463731448,
15.9082775535478));
#15901=CARTESIAN_POINT('Ctrl Pts',(-0.726161301554181,2.41060080271731,
15.9068982834207));
#15902=CARTESIAN_POINT('Ctrl Pts',(-0.554688243337949,2.46059760152126,
15.8959526373461));
#15903=CARTESIAN_POINT('Ctrl Pts',(-0.400933388541469,2.49027727997339,
15.886855644023));
#15904=CARTESIAN_POINT('Ctrl Pts',(-0.133708233663857,2.51645055530821,
15.8713997478473));
#15905=CARTESIAN_POINT('Ctrl Pts',(-0.0214131073894728,2.51990889726814,
15.8650007404159));
#15906=CARTESIAN_POINT('Ctrl Pts',(0.145430270638465,2.51389179599546,15.8552161590877));
#15907=CARTESIAN_POINT('Ctrl Pts',(0.200045295743299,2.5101360641009,15.8519677776078));
#15908=CARTESIAN_POINT('Ctrl Pts',(0.276411999706423,2.50237650075648,15.8473094807242));
#15909=CARTESIAN_POINT('Ctrl Pts',(0.298302127918328,2.49986149959144,15.8459607122724));
#15910=CARTESIAN_POINT('Ctrl Pts',(0.336661007584157,2.4949433904305,15.8435691075759));
#15911=CARTESIAN_POINT('Ctrl Pts',(0.353144478526909,2.49266365531695,15.8425322430868));
#15912=CARTESIAN_POINT('Ctrl Pts',(0.377706045048438,2.48901817770437,15.8409719481176));
#15913=CARTESIAN_POINT('Ctrl Pts',(0.385802413220178,2.48777608295063,15.8404551322775));
#15914=CARTESIAN_POINT('Ctrl Pts',(0.399700717814768,2.48557441426652,15.8395634631105));
#15915=CARTESIAN_POINT('Ctrl Pts',(0.405505564717805,2.48463399087122,15.8391896851294));
#15916=CARTESIAN_POINT('Ctrl Pts',(0.41876768858446,2.48243772508089,15.838332574971));
#15917=CARTESIAN_POINT('Ctrl Pts',(0.426222494394662,2.48116863949323,15.837848520655));
#15918=CARTESIAN_POINT('Ctrl Pts',(0.446719361255199,2.47758421035862,15.8365116035778));
#15919=CARTESIAN_POINT('Ctrl Pts',(0.459748826400814,2.47519952847301,15.8356550358795));
#15920=CARTESIAN_POINT('Ctrl Pts',(0.52884460967535,2.46198908661189,15.8310790700527));
#15921=CARTESIAN_POINT('Ctrl Pts',(0.584545101902249,2.44936171562828,15.8272729187443));
#15922=CARTESIAN_POINT('Ctrl Pts',(0.78168348264611,2.39756315553294,15.8134895325377));
#15923=CARTESIAN_POINT('Ctrl Pts',(0.920068473247469,2.34793766702451,15.8032493558316));
#15924=CARTESIAN_POINT('Ctrl Pts',(1.18281032727238,2.22690039498695,15.7833881009054));
#15925=CARTESIAN_POINT('Ctrl Pts',(1.30699644478953,2.1563621333607,15.7737943703504));
#15926=CARTESIAN_POINT('Ctrl Pts',(1.44712430400242,2.06019088908982,15.7628048887434));
#15927=CARTESIAN_POINT('Ctrl Pts',(1.46943576383536,2.0443370277864,15.7610489455182));
#15928=CARTESIAN_POINT('Ctrl Pts',(1.50291799094005,2.01971413011972,15.7584034285225));
#15929=CARTESIAN_POINT('Ctrl Pts',(1.51427986098309,2.01120962879152,15.7575038251017));
#15930=CARTESIAN_POINT('Ctrl Pts',(1.53479476913275,1.99558156035767,15.7558758549031));
#15931=CARTESIAN_POINT('Ctrl Pts',(1.54397158663948,1.98849000357109,15.7551462727766));
#15932=CARTESIAN_POINT('Ctrl Pts',(1.56368756266869,1.97303534111945,15.7535756869592));
#15933=CARTESIAN_POINT('Ctrl Pts',(1.57420938425578,1.96465062456972,15.7527355641207));
#15934=CARTESIAN_POINT('Ctrl Pts',(1.60269865975992,1.94157203415329,15.7504550687707));
#15935=CARTESIAN_POINT('Ctrl Pts',(1.62053120718329,1.92671316485822,15.7490213110135));
#15936=CARTESIAN_POINT('Ctrl Pts',(1.71743690111907,1.84366970388247,15.7411898989989));
#15937=CARTESIAN_POINT('Ctrl Pts',(1.79241960300952,1.77085944606404,15.734986805943));
#15938=CARTESIAN_POINT('Ctrl Pts',(1.97397931773628,1.57117422265329,15.7192423172525));
#15939=CARTESIAN_POINT('Ctrl Pts',(2.07294262786278,1.43808483452379,15.7099240427029));
#15940=CARTESIAN_POINT('Ctrl Pts',(2.20035052168185,1.22596375165347,15.6954290193888));
#15941=CARTESIAN_POINT('Ctrl Pts',(2.23910624318266,1.15365935879761,15.6905371491669));
#15942=CARTESIAN_POINT('Ctrl Pts',(2.28030223325077,1.06687693025528,15.6845731586594));
#15943=CARTESIAN_POINT('Ctrl Pts',(2.28623570035812,1.05410196872915,15.683692923656));
#15944=CARTESIAN_POINT('Ctrl Pts',(2.2952318659338,1.03429961038054,15.6823239315309));
#15945=CARTESIAN_POINT('Ctrl Pts',(2.29837030001894,1.02730665467101,15.6818396202343));
#15946=CARTESIAN_POINT('Ctrl Pts',(2.30412006610345,1.01433698099556,15.6809395779089));
#15947=CARTESIAN_POINT('Ctrl Pts',(2.30674015503032,1.00836434087861,15.6805243811195));
#15948=CARTESIAN_POINT('Ctrl Pts',(2.31268177619179,0.994675736080053,15.6795711799718));
#15949=CARTESIAN_POINT('Ctrl Pts',(2.31598790517059,0.986953310011539,15.6790322778378));
#15950=CARTESIAN_POINT('Ctrl Pts',(2.32458006008421,0.966602918775715,15.6776093934698));
#15951=CARTESIAN_POINT('Ctrl Pts',(2.32980175824751,0.953948324631367,15.6767218207374));
#15952=CARTESIAN_POINT('Ctrl Pts',(2.34408940327186,0.918505635343549,15.6742294616949));
#15953=CARTESIAN_POINT('Ctrl Pts',(2.35292426096839,0.895630883696691,15.672613486953));
#15954=CARTESIAN_POINT('Ctrl Pts',(2.36142199860763,0.87263531586336,15.670984110559));
#15955=CARTESIAN_POINT('Origin',(0.,0.,10.));
#15956=CARTESIAN_POINT('',(2.36142197356233,0.87263538363797,14.6670478768675));
#15957=CARTESIAN_POINT('',(2.36142200728636,0.87263529237801,14.9438284014526));
#15958=CARTESIAN_POINT('',(2.36142200728636,0.87263529237802,10.));
#15959=CARTESIAN_POINT('',(2.51749934288794,-0.0018189444229938,15.8874166974484));
#15960=CARTESIAN_POINT('Ctrl Pts',(2.36142200728636,0.872635292378009,14.9438284014526));
#15961=CARTESIAN_POINT('Ctrl Pts',(2.33277648153847,0.950152412648301,14.9490388977595));
#15962=CARTESIAN_POINT('Ctrl Pts',(2.30029580664879,1.02629583242825,14.9542493940664));
#15963=CARTESIAN_POINT('Ctrl Pts',(2.26414317539008,1.10066431364632,14.9594598903733));
#15964=CARTESIAN_POINT('Ctrl Pts',(2.22799445285202,1.17502475435369,14.9646698233361));
#15965=CARTESIAN_POINT('Ctrl Pts',(2.18817476734327,1.24761021831179,14.9698797562988));
#15966=CARTESIAN_POINT('Ctrl Pts',(2.1448943452171,1.31804191809505,14.9750896892615));
#15967=CARTESIAN_POINT('Ctrl Pts',(2.09942050746829,1.39204303756151,14.9805636572727));
#15968=CARTESIAN_POINT('Ctrl Pts',(2.0501261611078,1.46366582484097,14.9860376252838));
#15969=CARTESIAN_POINT('Ctrl Pts',(1.99730698814324,1.53250482710959,14.991511593295));
#15970=CARTESIAN_POINT('Ctrl Pts',(1.94696848714391,1.59811078021334,14.9967284743769));
#15971=CARTESIAN_POINT('Ctrl Pts',(1.89342914441608,1.66118820601892,15.0019453554588));
#15972=CARTESIAN_POINT('Ctrl Pts',(1.83698530511478,1.72142128451822,15.0071622365407));
#15973=CARTESIAN_POINT('Ctrl Pts',(1.78050276468467,1.78169566226574,15.0123826946151));
#15974=CARTESIAN_POINT('Ctrl Pts',(1.7211121013311,1.83912148975098,15.0176031526894));
#15975=CARTESIAN_POINT('Ctrl Pts',(1.65914462916598,1.89342159845864,15.0228236107638));
#15976=CARTESIAN_POINT('Ctrl Pts',(1.59708124854021,1.94780574867482,15.0280521486594));
#15977=CARTESIAN_POINT('Ctrl Pts',(1.5324334707376,1.99905424477454,15.033280686555));
#15978=CARTESIAN_POINT('Ctrl Pts',(1.46556295352631,2.04693221168929,15.0385092244506));
#15979=CARTESIAN_POINT('Ctrl Pts',(1.45589372738709,2.05385518624506,15.0392652514323));
#15980=CARTESIAN_POINT('Ctrl Pts',(1.44617807104084,2.06070776737762,15.0400212784139));
#15981=CARTESIAN_POINT('Ctrl Pts',(1.43641711978723,2.06748932475652,15.0407773053956));
#15982=CARTESIAN_POINT('Ctrl Pts',(1.36856738098678,2.11462887958713,15.046032554797));
#15983=CARTESIAN_POINT('Ctrl Pts',(1.2982693825395,2.15851196661367,15.0512878041983));
#15984=CARTESIAN_POINT('Ctrl Pts',(1.22586870228417,2.19887520672732,15.0565430535997));
#15985=CARTESIAN_POINT('Ctrl Pts',(1.15357066974716,2.23918122093527,15.0617908522512));
#15986=CARTESIAN_POINT('Ctrl Pts',(1.07917627644597,2.27597707769949,15.0670386509027));
#15987=CARTESIAN_POINT('Ctrl Pts',(1.00306088631776,2.30904203260561,15.0722864495542));
#15988=CARTESIAN_POINT('Ctrl Pts',(0.926393974459495,2.34234657166288,15.0775722730386));
#15989=CARTESIAN_POINT('Ctrl Pts',(0.847981409502392,2.37186564312825,15.082858096523));
#15990=CARTESIAN_POINT('Ctrl Pts',(0.76823300944464,2.39742034136687,15.0881439200074));
#15991=CARTESIAN_POINT('Ctrl Pts',(0.689199707900845,2.42274589235336,15.0933823458698));
#15992=CARTESIAN_POINT('Ctrl Pts',(0.608854879500604,2.44417773849274,15.0986207717323));
#15993=CARTESIAN_POINT('Ctrl Pts',(0.527616746581242,2.46159030277726,15.1038591975947));
#15994=CARTESIAN_POINT('Ctrl Pts',(0.446405331532488,2.47899714035902,15.109095900626));
#15995=CARTESIAN_POINT('Ctrl Pts',(0.36430164627102,2.492387224774,15.1143326036573));
#15996=CARTESIAN_POINT('Ctrl Pts',(0.281736172863987,2.50168562751197,15.1195693066886));
#15997=CARTESIAN_POINT('Ctrl Pts',(0.19917294849977,2.51098377696603,15.1248058670747));
#15998=CARTESIAN_POINT('Ctrl Pts',(0.116148419637579,2.51619041573157,15.1300424274607));
#15999=CARTESIAN_POINT('Ctrl Pts',(0.0330989093399816,2.51728240612779,
15.1352789878468));
#16000=CARTESIAN_POINT('Ctrl Pts',(-0.051309897791966,2.51839226946611,
15.1406012566246));
#16001=CARTESIAN_POINT('Ctrl Pts',(-0.13574401998502,2.51525155821139,15.1459235254023));
#16002=CARTESIAN_POINT('Ctrl Pts',(-0.219746481833127,2.50789109287504,
15.1512457941801));
#16003=CARTESIAN_POINT('Ctrl Pts',(-0.302514885877946,2.50063875817539,
15.1564898749241));
#16004=CARTESIAN_POINT('Ctrl Pts',(-0.384863772944501,2.48928995367179,
15.1617339556682));
#16005=CARTESIAN_POINT('Ctrl Pts',(-0.466364091257801,2.47392618814412,
15.1669780364122));
#16006=CARTESIAN_POINT('Ctrl Pts',(-0.549687135977597,2.45821881731883,
15.1723393992068));
#16007=CARTESIAN_POINT('Ctrl Pts',(-0.632122700302753,2.4383148521548,15.1777007620014));
#16008=CARTESIAN_POINT('Ctrl Pts',(-0.713228296029433,2.4143553275653,15.183062124796));
#16009=CARTESIAN_POINT('Ctrl Pts',(-0.794333891756125,2.3903958029758,15.1884234875906));
#16010=CARTESIAN_POINT('Ctrl Pts',(-0.874109061611535,2.36238095033946,
15.1937848503852));
#16011=CARTESIAN_POINT('Ctrl Pts',(-0.952134552185257,2.33050338865555,
15.1991462131798));
#16012=CARTESIAN_POINT('Ctrl Pts',(-1.0286157438934,2.29925675517194,15.2044014626206));
#16013=CARTESIAN_POINT('Ctrl Pts',(-1.10369839428042,2.26418355135292,15.2096567120615));
#16014=CARTESIAN_POINT('Ctrl Pts',(-1.17697343258409,2.22543024806243,15.2149119615023));
#16015=CARTESIAN_POINT('Ctrl Pts',(-1.25014458353137,2.18673188815134,15.2201597601934));
#16016=CARTESIAN_POINT('Ctrl Pts',(-1.32151280834504,2.14436400625807,15.2254075588846));
#16017=CARTESIAN_POINT('Ctrl Pts',(-1.3906885808284,2.09852127012177,15.2306553575757));
#16018=CARTESIAN_POINT('Ctrl Pts',(-1.4603655908628,2.05234636421029,15.2359411810502));
#16019=CARTESIAN_POINT('Ctrl Pts',(-1.52781780343736,2.0026462142322,15.2412270045247));
#16020=CARTESIAN_POINT('Ctrl Pts',(-1.59267202784433,1.94966716690881,15.2465128279992));
#16021=CARTESIAN_POINT('Ctrl Pts',(-1.65694470941202,1.89716317862567,15.2517512539014));
#16022=CARTESIAN_POINT('Ctrl Pts',(-1.71866544419385,1.84143915801312,15.2569896798036));
#16023=CARTESIAN_POINT('Ctrl Pts',(-1.77750119735707,1.78277753614807,15.2622281057058));
#16024=CARTESIAN_POINT('Ctrl Pts',(-1.83631760041949,1.72413520711493,15.2674648087768));
#16025=CARTESIAN_POINT('Ctrl Pts',(-1.89225057977768,1.66255752114573,15.2727015118479));
#16026=CARTESIAN_POINT('Ctrl Pts',(-1.94500290933897,1.59836476833761,15.2779382149189));
#16027=CARTESIAN_POINT('Ctrl Pts',(-1.99775380195184,1.5341737641096,15.2831747753446));
#16028=CARTESIAN_POINT('Ctrl Pts',(-2.04732392486907,1.46736819181756,15.2884113357704));
#16029=CARTESIAN_POINT('Ctrl Pts',(-2.09345631360712,1.39830143853838,15.2936478961961));
#16030=CARTESIAN_POINT('Ctrl Pts',(-2.14034376454627,1.32810424965462,15.2989701649267));
#16031=CARTESIAN_POINT('Ctrl Pts',(-2.18367964919649,1.25557159477232,15.3042924336574));
#16032=CARTESIAN_POINT('Ctrl Pts',(-2.22324101859935,1.1811035615971,15.3096147023881));
#16033=CARTESIAN_POINT('Ctrl Pts',(-2.26222120309141,1.10772951727694,15.3148587831711));
#16034=CARTESIAN_POINT('Ctrl Pts',(-2.29753689359051,1.03247703115664,15.3201028639542));
#16035=CARTESIAN_POINT('Ctrl Pts',(-2.32902286112003,0.955750366141851,
15.3253469447373));
#16036=CARTESIAN_POINT('Ctrl Pts',(-2.3612130006334,0.877307737726311,15.3307083074417));
#16037=CARTESIAN_POINT('Ctrl Pts',(-2.3893998792421,0.797324678732944,15.3360696701462));
#16038=CARTESIAN_POINT('Ctrl Pts',(-2.41346088255415,0.716249131504479,
15.3414310328506));
#16039=CARTESIAN_POINT('Ctrl Pts',(-2.43752188586621,0.635173584276002,
15.3467923955551));
#16040=CARTESIAN_POINT('Ctrl Pts',(-2.45745695899733,0.553006058343721,
15.3521537582595));
#16041=CARTESIAN_POINT('Ctrl Pts',(-2.47319940610295,0.470203091920946,
15.357515120964));
#16042=CARTESIAN_POINT('Ctrl Pts',(-2.4886302750115,0.389038981186634,15.3627703703231));
#16043=CARTESIAN_POINT('Ctrl Pts',(-2.50009000836156,0.306964573930027,
15.3680256196823));
#16044=CARTESIAN_POINT('Ctrl Pts',(-2.50747874556489,0.224402741828887,
15.3732808690415));
#16045=CARTESIAN_POINT('Ctrl Pts',(-2.51485700721747,0.141957963648953,
15.378528667651));
#16046=CARTESIAN_POINT('Ctrl Pts',(-2.51817569631215,0.0590275890165934,
15.3837764662605));
#16047=CARTESIAN_POINT('Ctrl Pts',(-2.51738602049689,-0.0239556633564388,
15.38902426487));
#16048=CARTESIAN_POINT('Ctrl Pts',(-2.51659062279048,-0.107540201887602,
15.3943100883649));
#16049=CARTESIAN_POINT('Ctrl Pts',(-2.51162698306217,-0.191177922134853,
15.3995959118598));
#16050=CARTESIAN_POINT('Ctrl Pts',(-2.5024985507745,-0.274421670739607,
15.4048817353547));
#16051=CARTESIAN_POINT('Ctrl Pts',(-2.49345197261146,-0.356918977462784,
15.4101201611759));
#16052=CARTESIAN_POINT('Ctrl Pts',(-2.4803150448715,-0.439028882564209,
15.4153585869972));
#16053=CARTESIAN_POINT('Ctrl Pts',(-2.46314334722548,-0.520318268965132,
15.4205970128184));
#16054=CARTESIAN_POINT('Ctrl Pts',(-2.445977297064,-0.601580920644586,15.4258337158088));
#16055=CARTESIAN_POINT('Ctrl Pts',(-2.42477920772006,-0.682023138468348,
15.4310704187993));
#16056=CARTESIAN_POINT('Ctrl Pts',(-2.39965591084302,-0.761221229049839,
15.4363071217897));
#16057=CARTESIAN_POINT('Ctrl Pts',(-2.37453329831013,-0.840417162320947,
15.4415436821354));
#16058=CARTESIAN_POINT('Ctrl Pts',(-2.34548583133283,-0.918368596220602,
15.4467802424811));
#16059=CARTESIAN_POINT('Ctrl Pts',(-2.31267002354775,-0.994667588787157,
15.4520168028267));
#16060=CARTESIAN_POINT('Ctrl Pts',(-2.27931710879627,-1.07221539170466,
15.4573390716535));
#16061=CARTESIAN_POINT('Ctrl Pts',(-2.2420715672161,-1.14805571627183,15.4626613404803));
#16062=CARTESIAN_POINT('Ctrl Pts',(-2.20114760439853,-1.22178372621778,
15.4679836093071));
#16063=CARTESIAN_POINT('Ctrl Pts',(-2.16082484529459,-1.29442861638924,
15.4732276900122));
#16064=CARTESIAN_POINT('Ctrl Pts',(-2.11693132432732,-1.36502247789413,
15.4784717707173));
#16065=CARTESIAN_POINT('Ctrl Pts',(-2.06971617492699,-1.43320661638355,
15.4837158514225));
#16066=CARTESIAN_POINT('Ctrl Pts',(-2.02144507385857,-1.50291567125448,
15.4890772143101));
#16067=CARTESIAN_POINT('Ctrl Pts',(-1.96970228962038,-1.57010551141682,
15.4944385771977));
#16068=CARTESIAN_POINT('Ctrl Pts',(-1.91479679524017,-1.6344294059206,15.4997999400853));
#16069=CARTESIAN_POINT('Ctrl Pts',(-1.85989130085996,-1.69875330042438,
15.5051613029729));
#16070=CARTESIAN_POINT('Ctrl Pts',(-1.80182349384693,-1.76021092581791,
15.5105226658605));
#16071=CARTESIAN_POINT('Ctrl Pts',(-1.74094000232509,-1.81849777517167,
15.5158840287482));
#16072=CARTESIAN_POINT('Ctrl Pts',(-1.68126153286005,-1.87563099589251,
15.5211392781332));
#16073=CARTESIAN_POINT('Ctrl Pts',(-1.61865742272164,-1.92992887109054,
15.5263945275182));
#16074=CARTESIAN_POINT('Ctrl Pts',(-1.55342800415825,-1.98107740532694,
15.5316497769033));
#16075=CARTESIAN_POINT('Ctrl Pts',(-1.4882910660995,-2.0321534225555,15.536897575538));
#16076=CARTESIAN_POINT('Ctrl Pts',(-1.42053657284844,-2.08008868537052,
15.5421453741726));
#16077=CARTESIAN_POINT('Ctrl Pts',(-1.35050092045069,-2.12460667274247,
15.5473931728073));
#16078=CARTESIAN_POINT('Ctrl Pts',(-1.27995779899129,-2.1694472315549,15.5526789962958));
#16079=CARTESIAN_POINT('Ctrl Pts',(-1.20710066325347,-2.21082045600598,
15.5579648197844));
#16080=CARTESIAN_POINT('Ctrl Pts',(-1.13230646008424,-2.24848578613508,
15.5632506432729));
#16081=CARTESIAN_POINT('Ctrl Pts',(-1.05818293179129,-2.2858133736377,15.5684890691175));
#16082=CARTESIAN_POINT('Ctrl Pts',(-0.98215735576056,-2.31949908603407,
15.573727494962));
#16083=CARTESIAN_POINT('Ctrl Pts',(-0.904623287695934,-2.34935373185014,
15.5789659208066));
#16084=CARTESIAN_POINT('Ctrl Pts',(-0.827114719301739,-2.37919855896783,
15.5842026238197));
#16085=CARTESIAN_POINT('Ctrl Pts',(-0.748099074453607,-2.40521465621004,
15.5894393268328));
#16086=CARTESIAN_POINT('Ctrl Pts',(-0.667989908555241,-2.42726095261065,
15.5946760298458));
#16087=CARTESIAN_POINT('Ctrl Pts',(-0.587882924796029,-2.44930664847965,
15.5999125902134));
#16088=CARTESIAN_POINT('Ctrl Pts',(-0.506682924365674,-2.46738263706995,
15.6051491505809));
#16089=CARTESIAN_POINT('Ctrl Pts',(-0.424817299930151,-2.4813980961708,
15.6103857109485));
#16090=CARTESIAN_POINT('Ctrl Pts',(-0.341611755062269,-2.4956429507004,
15.6157079797472));
#16091=CARTESIAN_POINT('Ctrl Pts',(-0.257719083109179,-2.50569306067364,
15.6210302485458));
#16092=CARTESIAN_POINT('Ctrl Pts',(-0.173595482170129,-2.51150768634502,
15.6263525173445));
#16093=CARTESIAN_POINT('Ctrl Pts',(-0.0907077192844954,-2.51723689085527,
15.6315965980694));
#16094=CARTESIAN_POINT('Ctrl Pts',(-0.00759623653741434,-2.51885428207375,
15.6368406787943));
#16095=CARTESIAN_POINT('Ctrl Pts',(0.0753024549304608,-2.51637353949716,
15.6420847595193));
#16096=CARTESIAN_POINT('Ctrl Pts',(0.160055147892539,-2.51383731594297,
15.6474461223548));
#16097=CARTESIAN_POINT('Ctrl Pts',(0.244584906330077,-2.50701748102916,
15.6528074851903));
#16098=CARTESIAN_POINT('Ctrl Pts',(0.328432674164168,-2.4959844207329,15.6581688480258));
#16099=CARTESIAN_POINT('Ctrl Pts',(0.412280441998259,-2.48495136043665,
15.6635302108613));
#16100=CARTESIAN_POINT('Ctrl Pts',(0.495445731495645,-2.46970523208183,
15.6688915736969));
#16101=CARTESIAN_POINT('Ctrl Pts',(0.577484402382204,-2.45037099538116,
15.6742529365324));
#16102=CARTESIAN_POINT('Ctrl Pts',(0.657899346862904,-2.43141942590716,
15.6795081861616));
#16103=CARTESIAN_POINT('Ctrl Pts',(0.73752889484594,-2.40847014295311,15.6847634357908));
#16104=CARTESIAN_POINT('Ctrl Pts',(0.815946152988599,-2.38160410761804,
15.69001868542));
#16105=CARTESIAN_POINT('Ctrl Pts',(0.894252233289506,-2.35477616221235,
15.6952664843002));
#16106=CARTESIAN_POINT('Ctrl Pts',(0.971349004820566,-2.32404264273536,
15.7005142831804));
#16107=CARTESIAN_POINT('Ctrl Pts',(1.04682137249731,-2.2895351633209,15.7057620820606));
#16108=CARTESIAN_POINT('Ctrl Pts',(1.12284059851767,-2.25477764930946,15.7110479054879));
#16109=CARTESIAN_POINT('Ctrl Pts',(1.19721131986629,-2.21619136251645,15.7163337289152));
#16110=CARTESIAN_POINT('Ctrl Pts',(1.26952652745185,-2.17396150980096,15.7216195523426));
#16111=CARTESIAN_POINT('Ctrl Pts',(1.34119329336554,-2.13211032703901,15.726857978434));
#16112=CARTESIAN_POINT('Ctrl Pts',(1.41084085516088,-2.08668089644513,15.7320964045255));
#16113=CARTESIAN_POINT('Ctrl Pts',(1.47809624844896,-2.03790032394156,15.737334830617));
#16114=CARTESIAN_POINT('Ctrl Pts',(1.54532952255311,-1.98913579455963,15.742571533877));
#16115=CARTESIAN_POINT('Ctrl Pts',(1.61017181744542,-1.93702258286824,15.747808237137));
#16116=CARTESIAN_POINT('Ctrl Pts',(1.67227964298106,-1.8818307696685,15.753044940397));
#16117=CARTESIAN_POINT('Ctrl Pts',(1.73438577672219,-1.82664045987361,15.7582815010111));
#16118=CARTESIAN_POINT('Ctrl Pts',(1.79375724497693,-1.76837202258052,15.7635180616252));
#16119=CARTESIAN_POINT('Ctrl Pts',(1.85008517215019,-1.70733450319204,15.7687546222393));
#16120=CARTESIAN_POINT('Ctrl Pts',(1.90733503039106,-1.64529796984657,15.7740768907457));
#16121=CARTESIAN_POINT('Ctrl Pts',(1.96144047700552,-1.58040124476285,15.7793991592521));
#16122=CARTESIAN_POINT('Ctrl Pts',(2.01211896210389,-1.51300480248476,15.7847214277586));
#16123=CARTESIAN_POINT('Ctrl Pts',(2.0620529477485,-1.44659845717513,15.7899655087267));
#16124=CARTESIAN_POINT('Ctrl Pts',(2.10865978046098,-1.37776577400283,15.7952095896948));
#16125=CARTESIAN_POINT('Ctrl Pts',(2.15171327529958,-1.30688034299225,15.8004536706629));
#16126=CARTESIAN_POINT('Ctrl Pts',(2.19572964050522,-1.23440959396672,15.8058150329385));
#16127=CARTESIAN_POINT('Ctrl Pts',(2.23603156928824,-1.15979362226863,15.8111763952141));
#16128=CARTESIAN_POINT('Ctrl Pts',(2.27242816711791,-1.08345580218537,15.8165377574897));
#16129=CARTESIAN_POINT('Ctrl Pts',(2.30882476494757,-1.00711798210211,15.8218991197653));
#16130=CARTESIAN_POINT('Ctrl Pts',(2.34131589823886,-0.929058808395344,
15.8272604820409));
#16131=CARTESIAN_POINT('Ctrl Pts',(2.36976456938881,-0.849718856839985,
15.8326218443165));
#16132=CARTESIAN_POINT('Ctrl Pts',(2.40208841605574,-0.759571502852221,
15.8387135120506));
#16133=CARTESIAN_POINT('Ctrl Pts',(2.42929323465991,-0.667497677878766,
15.8448051797847));
#16134=CARTESIAN_POINT('Ctrl Pts',(2.45117917360797,-0.574044343993166,
15.8508968475188));
#16135=CARTESIAN_POINT('Ctrl Pts',(2.47304705502787,-0.480668116061849,
15.8569834891737));
#16136=CARTESIAN_POINT('Ctrl Pts',(2.48960468448161,-0.385914782985989,
15.8630701308287));
#16137=CARTESIAN_POINT('Ctrl Pts',(2.50070035307118,-0.290351501028792,
15.8691567724836));
#16138=CARTESIAN_POINT('Ctrl Pts',(2.51179602166076,-0.194788219071594,
15.8752434141385));
#16139=CARTESIAN_POINT('Ctrl Pts',(2.51742955018304,-0.0984151276298001,
15.8813300557935));
#16140=CARTESIAN_POINT('Ctrl Pts',(2.51749934288794,-0.00181894442298069,
15.8874166974484));
#16141=CARTESIAN_POINT('Ctrl Pts',(2.51749934288862,-0.00181894347718374,
15.887416697508));
#16142=CARTESIAN_POINT('Ctrl Pts',(2.517559487875,0.0814244148722606,15.8926619616126));
#16143=CARTESIAN_POINT('Ctrl Pts',(2.51348653829097,0.164706578703061,15.8979072257173));
#16144=CARTESIAN_POINT('Ctrl Pts',(2.50529558016625,0.247588986022126,15.9031524898219));
#16145=CARTESIAN_POINT('Ctrl Pts',(2.49710604212937,0.330457023801282,15.9083968445414));
#16146=CARTESIAN_POINT('Ctrl Pts',(2.48479996515358,0.412924986783603,15.9136411992608));
#16147=CARTESIAN_POINT('Ctrl Pts',(2.46844432551966,0.494559260159785,15.9188855539803));
#16148=CARTESIAN_POINT('Ctrl Pts',(2.45208034576598,0.576235160744154,15.9241325829178));
#16149=CARTESIAN_POINT('Ctrl Pts',(2.4316627733015,0.657076073200728,15.9293796118553));
#16150=CARTESIAN_POINT('Ctrl Pts',(2.40730957902637,0.73665924329223,15.9346266407928));
#16151=CARTESIAN_POINT('Ctrl Pts',(2.39330444855097,0.782426244868507,15.9376441227726));
#16152=CARTESIAN_POINT('Ctrl Pts',(2.37799865629738,0.827777533216081,15.9406616047525));
#16153=CARTESIAN_POINT('Ctrl Pts',(2.36142200728636,0.872635292378007,15.9436790867324));
#16154=CARTESIAN_POINT('Ctrl Pts',(2.36142199860763,0.87263531586336,15.670984110559));
#16155=CARTESIAN_POINT('Ctrl Pts',(2.38881140575593,0.798517356856821,15.6657324005925));
#16156=CARTESIAN_POINT('Ctrl Pts',(2.41269859977669,0.723144194438671,15.6603427311849));
#16157=CARTESIAN_POINT('Ctrl Pts',(2.48897985726643,0.436189773331056,15.6399181512781));
#16158=CARTESIAN_POINT('Ctrl Pts',(2.51739377276997,0.219189285637256,15.6247664971261));
#16159=CARTESIAN_POINT('Ctrl Pts',(2.51751982902625,-0.0401892803670483,
15.6077912659681));
#16160=CARTESIAN_POINT('Ctrl Pts',(2.51651810043557,-0.0815980963299537,
15.6051113332934));
#16161=CARTESIAN_POINT('Ctrl Pts',(2.5136565021235,-0.14011433710098,15.601364814718));
#16162=CARTESIAN_POINT('Ctrl Pts',(2.51264244759951,-0.157254546783502,
15.600272320509));
#16163=CARTESIAN_POINT('Ctrl Pts',(2.51070321221152,-0.185183230864893,
15.5984998713506));
#16164=CARTESIAN_POINT('Ctrl Pts',(2.50988365856385,-0.195978251874473,
15.5978166571824));
#16165=CARTESIAN_POINT('Ctrl Pts',(2.50801290938118,-0.218678593221559,
15.5963837736142));
#16166=CARTESIAN_POINT('Ctrl Pts',(2.50694651663212,-0.230582417778358,
15.5956345955265));
#16167=CARTESIAN_POINT('Ctrl Pts',(2.50418055193433,-0.259166170399388,
15.5938407360676));
#16168=CARTESIAN_POINT('Ctrl Pts',(2.50239903003582,-0.275837735524215,
15.5927986313873));
#16169=CARTESIAN_POINT('Ctrl Pts',(2.49559433710554,-0.334009870738131,
15.5891759084683));
#16170=CARTESIAN_POINT('Ctrl Pts',(2.48970405154831,-0.375403424295379,
15.5866222670278));
#16171=CARTESIAN_POINT('Ctrl Pts',(2.4467489135997,-0.631380244526915,15.5709426874391));
#16172=CARTESIAN_POINT('Ctrl Pts',(2.38300758603946,-0.840534570131567,
15.5587213945927));
#16173=CARTESIAN_POINT('Ctrl Pts',(2.25010360397097,-1.13389598543474,15.5400367430987));
#16174=CARTESIAN_POINT('Ctrl Pts',(2.20120110001263,-1.22613000538683,15.5338902104286));
#16175=CARTESIAN_POINT('Ctrl Pts',(2.13957096552891,-1.32673661154938,15.5265782160125));
#16176=CARTESIAN_POINT('Ctrl Pts',(2.13231925254442,-1.33836039203338,15.5257237644765));
#16177=CARTESIAN_POINT('Ctrl Pts',(2.1204670366814,-1.35701747145425,15.5243356851403));
#16178=CARTESIAN_POINT('Ctrl Pts',(2.11592544650851,-1.36408810987468,15.5238057367336));
#16179=CARTESIAN_POINT('Ctrl Pts',(2.10779620020278,-1.37660596076598,15.5228603269342));
#16180=CARTESIAN_POINT('Ctrl Pts',(2.10422266555543,-1.38206214227595,15.5224457923324));
#16181=CARTESIAN_POINT('Ctrl Pts',(2.09640464151786,-1.39389832708489,15.5215411183615));
#16182=CARTESIAN_POINT('Ctrl Pts',(2.09215227908852,-1.40027276079334,15.5210504782031));
#16183=CARTESIAN_POINT('Ctrl Pts',(2.08000666891873,-1.41830060767409,15.5196533596124));
#16184=CARTESIAN_POINT('Ctrl Pts',(2.07204484475086,-1.42990716352752,15.5187425254391));
#16185=CARTESIAN_POINT('Ctrl Pts',(2.01720154697946,-1.50843651182806,15.512505498258));
#16186=CARTESIAN_POINT('Ctrl Pts',(1.96718763891124,-1.57310292610649,15.5070003396374));
#16187=CARTESIAN_POINT('Ctrl Pts',(1.84152149819552,-1.72020311889623,15.4937775149866));
#16188=CARTESIAN_POINT('Ctrl Pts',(1.76333971063287,-1.80025916687264,15.4860096425698));
#16189=CARTESIAN_POINT('Ctrl Pts',(1.56385461702373,-1.97902204085724,15.4675845595447));
#16190=CARTESIAN_POINT('Ctrl Pts',(1.43815965630078,-2.07216834872263,15.4570590777913));
#16191=CARTESIAN_POINT('Ctrl Pts',(1.2855460439328,-2.16464205996158,15.4455491516549));
#16192=CARTESIAN_POINT('Ctrl Pts',(1.26631427043085,-2.17594855169479,15.444119404117));
#16193=CARTESIAN_POINT('Ctrl Pts',(1.23441582180643,-2.19413570298014,15.4417811928913));
#16194=CARTESIAN_POINT('Ctrl Pts',(1.22183614917437,-2.20116567819165,15.4408674333296));
#16195=CARTESIAN_POINT('Ctrl Pts',(1.19901245798483,-2.21366442707653,15.4392243454714));
#16196=CARTESIAN_POINT('Ctrl Pts',(1.1887897274702,-2.21917103019417,15.4384936925878));
#16197=CARTESIAN_POINT('Ctrl Pts',(1.16678671473362,-2.23082755822618,15.4369321819197));
#16198=CARTESIAN_POINT('Ctrl Pts',(1.15499506001769,-2.23695535366888,15.4361021172352));
#16199=CARTESIAN_POINT('Ctrl Pts',(1.12259845212116,-2.25346651036378,15.4338396319747));
#16200=CARTESIAN_POINT('Ctrl Pts',(1.10189808677716,-2.26366058824857,15.4324137932811));
#16201=CARTESIAN_POINT('Ctrl Pts',(0.979934341541557,-2.32165316581012,
15.4241229314208));
#16202=CARTESIAN_POINT('Ctrl Pts',(0.875706732592535,-2.36294031080028,
15.4174851316121));
#16203=CARTESIAN_POINT('Ctrl Pts',(0.612895949574018,-2.44725641560329,
15.4014207549164));
#16204=CARTESIAN_POINT('Ctrl Pts',(0.452213364262973,-2.48197584425831,
15.392182657108));
#16205=CARTESIAN_POINT('Ctrl Pts',(0.213842815866966,-2.50955136071224,
15.378089232579));
#16206=CARTESIAN_POINT('Ctrl Pts',(0.1380329374517,-2.51486011073486,15.3735457787418));
#16207=CARTESIAN_POINT('Ctrl Pts',(0.0490628643820267,-2.51705568975932,
15.368023961927));
#16208=CARTESIAN_POINT('Ctrl Pts',(0.036016478002413,-2.51727616812457,
15.3672094718865));
#16209=CARTESIAN_POINT('Ctrl Pts',(0.0147608659385897,-2.51747010919017,
15.3658738352442));
#16210=CARTESIAN_POINT('Ctrl Pts',(0.0065522617272382,-2.5175048554485,
15.3653559325133));
#16211=CARTESIAN_POINT('Ctrl Pts',(-0.00816613720818674,-2.51749517241507,
15.3644233113043));
#16212=CARTESIAN_POINT('Ctrl Pts',(-0.0146757652788879,-2.51746564008284,
15.3640094184943));
#16213=CARTESIAN_POINT('Ctrl Pts',(-0.0289991101952524,-2.51734510179127,
15.3630955629884));
#16214=CARTESIAN_POINT('Ctrl Pts',(-0.0368124436567685,-2.51724296601848,
15.3625950156029));
#16215=CARTESIAN_POINT('Ctrl Pts',(-0.0594131698256786,-2.51684228399823,
15.361141475967));
#16216=CARTESIAN_POINT('Ctrl Pts',(-0.0741982781822732,-2.51644980040659,
15.3601835736814));
#16217=CARTESIAN_POINT('Ctrl Pts',(-0.195396873408821,-2.51216347321171,
15.3522784220622));
#16218=CARTESIAN_POINT('Ctrl Pts',(-0.30145770675546,-2.50165213318503,
15.3450302451222));
#16219=CARTESIAN_POINT('Ctrl Pts',(-0.418811623063205,-2.48245003380248,
15.3368466175873));
#16220=CARTESIAN_POINT('Ctrl Pts',(-0.431086785658288,-2.48034786394589,
15.3359885270153));
#16221=CARTESIAN_POINT('Ctrl Pts',(-0.636301071400487,-2.44363470479067,
15.321612183756));
#16222=CARTESIAN_POINT('Ctrl Pts',(-0.824599525550887,-2.38668996798914,
15.3080393549895));
#16223=CARTESIAN_POINT('Ctrl Pts',(-1.04713468432362,-2.28986624573079,
15.2920970503824));
#16224=CARTESIAN_POINT('Ctrl Pts',(-1.08934929702491,-2.27008745421015,
15.2890733021061));
#16225=CARTESIAN_POINT('Ctrl Pts',(-1.14707478540443,-2.24105995338555,
15.2849368436095));
#16226=CARTESIAN_POINT('Ctrl Pts',(-1.16306990017164,-2.23280064331093,
15.2837904565796));
#16227=CARTESIAN_POINT('Ctrl Pts',(-1.1886733129984,-2.21923015383286,15.281954716087));
#16228=CARTESIAN_POINT('Ctrl Pts',(-1.19833763043849,-2.21402656948294,
15.2812616259039));
#16229=CARTESIAN_POINT('Ctrl Pts',(-1.21834298804327,-2.20308566698797,
15.2798264310971));
#16230=CARTESIAN_POINT('Ctrl Pts',(-1.22867827250917,-2.19733834511559,
15.2790847020833));
#16231=CARTESIAN_POINT('Ctrl Pts',(-1.25295371490377,-2.18361424668106,
15.2773416766438));
#16232=CARTESIAN_POINT('Ctrl Pts',(-1.26685889988727,-2.17557641477953,
15.2763425846859));
#16233=CARTESIAN_POINT('Ctrl Pts',(-1.31291527988052,-2.14836241563089,
15.2730302719432));
#16234=CARTESIAN_POINT('Ctrl Pts',(-1.34471651039098,-2.12860173128764,
15.2707380947528));
#16235=CARTESIAN_POINT('Ctrl Pts',(-1.48882062067564,-2.03453919354006,
15.2603077924118));
#16236=CARTESIAN_POINT('Ctrl Pts',(-1.59549388633856,-1.95200957712699,
15.2524774388167));
#16237=CARTESIAN_POINT('Ctrl Pts',(-1.81300488204768,-1.753928719302,15.235538490969));
#16238=CARTESIAN_POINT('Ctrl Pts',(-1.92045942321415,-1.63556665368369,
15.2265001596354));
#16239=CARTESIAN_POINT('Ctrl Pts',(-2.03977441565233,-1.47604344114202,
15.2144986766687));
#16240=CARTESIAN_POINT('Ctrl Pts',(-2.0628068788277,-1.44367977347344,15.2120710098848));
#16241=CARTESIAN_POINT('Ctrl Pts',(-2.09172327607617,-1.40094298731833,
15.2088553258887));
#16242=CARTESIAN_POINT('Ctrl Pts',(-2.09831391981306,-1.39105219107801,
15.2081104297761));
#16243=CARTESIAN_POINT('Ctrl Pts',(-2.10877568167771,-1.37510835714715,
15.2069079558654));
#16244=CARTESIAN_POINT('Ctrl Pts',(-2.11269144420212,-1.36908463144331,
15.2064532623436));
#16245=CARTESIAN_POINT('Ctrl Pts',(-2.12017744243631,-1.35746012022529,
15.2055748876328));
#16246=CARTESIAN_POINT('Ctrl Pts',(-2.12375136059673,-1.35186187152455,
15.2051514522374));
#16247=CARTESIAN_POINT('Ctrl Pts',(-2.13227574337301,-1.33839189942268,
15.2041317199498));
#16248=CARTESIAN_POINT('Ctrl Pts',(-2.13720480023032,-1.3305068047939,15.2035340569879));
#16249=CARTESIAN_POINT('Ctrl Pts',(-2.15407972621147,-1.30317597643868,
15.2014604553677));
#16250=CARTESIAN_POINT('Ctrl Pts',(-2.1658043868312,-1.28359587260666,15.1999714007256));
#16251=CARTESIAN_POINT('Ctrl Pts',(-2.19398761626698,-1.23504441653125,
15.1962755836971));
#16252=CARTESIAN_POINT('Ctrl Pts',(-2.21014000107759,-1.20590104590893,
15.1940541475708));
#16253=CARTESIAN_POINT('Ctrl Pts',(-2.27530537861129,-1.08261533106032,
15.184669676121));
#16254=CARTESIAN_POINT('Ctrl Pts',(-2.31891642286823,-0.985745831882188,
15.1773317781199));
#16255=CARTESIAN_POINT('Ctrl Pts',(-2.42115219806167,-0.713982399962587,
15.1572729264982));
#16256=CARTESIAN_POINT('Ctrl Pts',(-2.46690840652586,-0.534915639120533,
15.1446676848096));
#16257=CARTESIAN_POINT('Ctrl Pts',(-2.49727129684068,-0.320163201604435,
15.1305791461148));
#16258=CARTESIAN_POINT('Ctrl Pts',(-2.50120688379339,-0.287806693320121,
15.1284813581798));
#16259=CARTESIAN_POINT('Ctrl Pts',(-2.5060391771045,-0.240416661009576,
15.1254438908344));
#16260=CARTESIAN_POINT('Ctrl Pts',(-2.50743099894337,-0.225438083781834,
15.124488917134));
#16261=CARTESIAN_POINT('Ctrl Pts',(-2.50966724307612,-0.198780434511985,
15.122798102588));
#16262=CARTESIAN_POINT('Ctrl Pts',(-2.51056458739767,-0.187106365737418,
15.1220606358));
#16263=CARTESIAN_POINT('Ctrl Pts',(-2.5122705510553,-0.162684008276177,
15.1205239076267));
#16264=CARTESIAN_POINT('Ctrl Pts',(-2.51306365425366,-0.149934944204064,
15.1197251490001));
#16265=CARTESIAN_POINT('Ctrl Pts',(-2.51488797229082,-0.116505214851965,
15.1176394154671));
#16266=CARTESIAN_POINT('Ctrl Pts',(-2.51576115537954,-0.0958166318843272,
15.1163573633316));
#16267=CARTESIAN_POINT('Ctrl Pts',(-2.5186384570955,0.000568677124928038,
15.1104222386679));
#16268=CARTESIAN_POINT('Ctrl Pts',(-2.5174821168074,0.0763244139333311,
15.1058674751591));
#16269=CARTESIAN_POINT('Ctrl Pts',(-2.50493933800149,0.283796631592991,
15.0935748077665));
#16270=CARTESIAN_POINT('Ctrl Pts',(-2.48659714810952,0.414847705627033,
15.0860204203589));
#16271=CARTESIAN_POINT('Ctrl Pts',(-2.42841472277007,0.677813731246231,
15.0705340399385));
#16272=CARTESIAN_POINT('Ctrl Pts',(-2.38787836655046,0.809108773280037,
15.0626207255028));
#16273=CARTESIAN_POINT('Ctrl Pts',(-2.32889676410057,0.956297121081916,
15.052882981077));
#16274=CARTESIAN_POINT('Ctrl Pts',(-2.3206829501584,0.97606090820723,15.0515564353465));
#16275=CARTESIAN_POINT('Ctrl Pts',(-2.30888747632026,1.00345194182823,15.0496881162314));
#16276=CARTESIAN_POINT('Ctrl Pts',(-2.30551773684484,1.0111701826154,15.0491583279628));
#16277=CARTESIAN_POINT('Ctrl Pts',(-2.29963581490471,1.0244602110262,15.0482400780457));
#16278=CARTESIAN_POINT('Ctrl Pts',(-2.2971419261892,1.0300400837845,15.0478527092524));
#16279=CARTESIAN_POINT('Ctrl Pts',(-2.29183545771371,1.0417977542909,15.0470324635551));
#16280=CARTESIAN_POINT('Ctrl Pts',(-2.28901818103231,1.04797332484206,15.0465992931731));
#16281=CARTESIAN_POINT('Ctrl Pts',(-2.281961819795,1.06327691346483,15.0455201599903));
#16282=CARTESIAN_POINT('Ctrl Pts',(-2.2776929397021,1.07239097627057,15.0448724251353));
#16283=CARTESIAN_POINT('Ctrl Pts',(-2.26136242005423,1.10671924959317,15.0424142477346));
#16284=CARTESIAN_POINT('Ctrl Pts',(-2.24893629088401,1.13175655434347,15.0405835595723));
#16285=CARTESIAN_POINT('Ctrl Pts',(-2.21592779748154,1.19557414097106,15.0358289372114));
#16286=CARTESIAN_POINT('Ctrl Pts',(-2.19474362889226,1.23403140130677,15.0328782670417));
#16287=CARTESIAN_POINT('Ctrl Pts',(-2.10996816826968,1.37883715093957,15.0214880860647));
#16288=CARTESIAN_POINT('Ctrl Pts',(-2.03956370666671,1.48099167872028,15.0128701946067));
#16289=CARTESIAN_POINT('Ctrl Pts',(-1.86060732884295,1.70355211466464,14.993207170834));
#16290=CARTESIAN_POINT('Ctrl Pts',(-1.74736961478691,1.81952351801807,14.982286003529));
#16291=CARTESIAN_POINT('Ctrl Pts',(-1.60677702348184,1.93818684678772,14.9704201840154));
#16292=CARTESIAN_POINT('Ctrl Pts',(-1.58959541222314,1.95230303320891,14.9689951585419));
#16293=CARTESIAN_POINT('Ctrl Pts',(-1.56099121460858,1.97517586556778,14.9666630443253));
#16294=CARTESIAN_POINT('Ctrl Pts',(-1.54967684211776,1.98406526379702,14.9657507069784));
#16295=CARTESIAN_POINT('Ctrl Pts',(-1.52909651461544,1.99995121980013,14.9641091512604));
#16296=CARTESIAN_POINT('Ctrl Pts',(-1.51985726059715,2.00698155130553,14.9633786192623));
#16297=CARTESIAN_POINT('Ctrl Pts',(-1.49992650584378,2.02193069327464,14.9618162618917));
#16298=CARTESIAN_POINT('Ctrl Pts',(-1.48922016222383,2.02982919738463,14.9609852380707));
#16299=CARTESIAN_POINT('Ctrl Pts',(-1.45971767887471,2.05123530286599,14.9587173122495));
#16300=CARTESIAN_POINT('Ctrl Pts',(-1.44079679234585,2.06456935650309,14.957287046414));
#16301=CARTESIAN_POINT('Ctrl Pts',(-1.32801153730688,2.1417463806301,14.948897744424));
#16302=CARTESIAN_POINT('Ctrl Pts',(-1.23009425552339,2.19944650556234,14.9421727064589));
#16303=CARTESIAN_POINT('Ctrl Pts',(-0.969073344892513,2.33035519740223,
14.9251860656122));
#16304=CARTESIAN_POINT('Ctrl Pts',(-0.801498018579548,2.39316763673473,
14.9151704027721));
#16305=CARTESIAN_POINT('Ctrl Pts',(-0.569392832980046,2.45302868214434,
14.9009671154989));
#16306=CARTESIAN_POINT('Ctrl Pts',(-0.509549310245642,2.46615411296971,
14.8972730613384));
#16307=CARTESIAN_POINT('Ctrl Pts',(-0.435999532412581,2.4794945389303,14.8926291769369));
#16308=CARTESIAN_POINT('Ctrl Pts',(-0.422687911373011,2.4817984752291,14.891784573943));
#16309=CARTESIAN_POINT('Ctrl Pts',(-0.401838141655966,2.48523448658922,
14.8904543485869));
#16310=CARTESIAN_POINT('Ctrl Pts',(-0.394312074285199,2.48643968956872,
14.8899726904463));
#16311=CARTESIAN_POINT('Ctrl Pts',(-0.380330784147522,2.48861354023739,
14.8890749464072));
#16312=CARTESIAN_POINT('Ctrl Pts',(-0.373877154234701,2.48959127733828,
14.8886593706427));
#16313=CARTESIAN_POINT('Ctrl Pts',(-0.359048939490664,2.49177882359664,
14.8877018327678));
#16314=CARTESIAN_POINT('Ctrl Pts',(-0.350672029781081,2.49297151392958,
14.8871589409402));
#16315=CARTESIAN_POINT('Ctrl Pts',(-0.324420325786182,2.49657425693135,
14.8854518519568));
#16316=CARTESIAN_POINT('Ctrl Pts',(-0.306525997128382,2.49883439573106,
14.8842798663823));
#16317=CARTESIAN_POINT('Ctrl Pts',(-0.141649521573048,2.51786150066191,
14.87341389261));
#16318=CARTESIAN_POINT('Ctrl Pts',(0.00650513065036972,2.52183274284893,
14.8631750668824));
#16319=CARTESIAN_POINT('Ctrl Pts',(0.336348971714478,2.5016000164923,14.8403463504556));
#16320=CARTESIAN_POINT('Ctrl Pts',(0.516838295960918,2.4706343014458,14.8278613649218));
#16321=CARTESIAN_POINT('Ctrl Pts',(0.723475030893875,2.41152107796648,14.8138987483381));
#16322=CARTESIAN_POINT('Ctrl Pts',(0.754363778964595,2.40203777595943,14.8118187778432));
#16323=CARTESIAN_POINT('Ctrl Pts',(0.799520622156711,2.38721690999601,14.8087874026054));
#16324=CARTESIAN_POINT('Ctrl Pts',(0.813935539385937,2.3823406043055,14.8078211419135));
#16325=CARTESIAN_POINT('Ctrl Pts',(0.839386144979637,2.37347315811431,14.8061173829471));
#16326=CARTESIAN_POINT('Ctrl Pts',(0.850439691476767,2.36953503273654,14.8053781727174));
#16327=CARTESIAN_POINT('Ctrl Pts',(0.87339104543088,2.36117670098505,14.8038446976425));
#16328=CARTESIAN_POINT('Ctrl Pts',(0.885283794193366,2.35674350421294,14.8030508859994));
#16329=CARTESIAN_POINT('Ctrl Pts',(0.915027327187574,2.34539924753365,14.8010672685988));
#16330=CARTESIAN_POINT('Ctrl Pts',(0.93283396080928,2.33837410881037,14.799881272571));
#16331=CARTESIAN_POINT('Ctrl Pts',(1.01005308277905,2.30688687962633,14.7947427787229));
#16332=CARTESIAN_POINT('Ctrl Pts',(1.06859977710096,2.2803573963202,14.7908596590706));
#16333=CARTESIAN_POINT('Ctrl Pts',(1.22815297925636,2.20056210977424,14.7802425810399));
#16334=CARTESIAN_POINT('Ctrl Pts',(1.32664980754301,2.14262368778261,14.773653449442));
#16335=CARTESIAN_POINT('Ctrl Pts',(1.56183499231316,1.98182592477016,14.7572750215297));
#16336=CARTESIAN_POINT('Ctrl Pts',(1.6926009103257,1.87137605714634,14.7475711753274));
#16337=CARTESIAN_POINT('Ctrl Pts',(1.82395545053425,1.73531894033377,14.7359355338547));
#16338=CARTESIAN_POINT('Ctrl Pts',(1.83659872920183,1.72193216282107,14.7347934592627));
#16339=CARTESIAN_POINT('Ctrl Pts',(1.85568782044743,1.70127110917447,14.733032725243));
#16340=CARTESIAN_POINT('Ctrl Pts',(1.86224052985465,1.694095887354,14.7324216023394));
#16341=CARTESIAN_POINT('Ctrl Pts',(1.87320854792724,1.68194537150281,14.7313869475562));
#16342=CARTESIAN_POINT('Ctrl Pts',(1.87764606076477,1.67699009119724,14.7309650497652));
#16343=CARTESIAN_POINT('Ctrl Pts',(1.88672632177683,1.66676912580199,14.7300948125163));
#16344=CARTESIAN_POINT('Ctrl Pts',(1.8913667453634,1.66150153886609,14.7296463210225));
#16345=CARTESIAN_POINT('Ctrl Pts',(1.90331460362784,1.64782398831414,14.7284819581567));
#16346=CARTESIAN_POINT('Ctrl Pts',(1.91058825832425,1.63938490692625,14.7277637061883));
#16347=CARTESIAN_POINT('Ctrl Pts',(1.94117681057694,1.60341521833078,14.7247040330188));
#16348=CARTESIAN_POINT('Ctrl Pts',(1.96395329172995,1.57543483711423,14.7223282075242));
#16349=CARTESIAN_POINT('Ctrl Pts',(2.04973601817565,1.46530082597472,14.7130235856465));
#16350=CARTESIAN_POINT('Ctrl Pts',(2.10824951106603,1.37978445616766,14.7059009304884));
#16351=CARTESIAN_POINT('Ctrl Pts',(2.21633923608816,1.19881426405434,14.6913445031883));
#16352=CARTESIAN_POINT('Ctrl Pts',(2.26540931700534,1.10328513542836,14.6839244519033));
#16353=CARTESIAN_POINT('Ctrl Pts',(2.32721433607724,0.961322021669879,14.6734116019023));
#16354=CARTESIAN_POINT('Ctrl Pts',(2.34494933737997,0.917211670335576,14.6702119075418));
#16355=CARTESIAN_POINT('Ctrl Pts',(2.36142197356233,0.872635383637971,14.6670478768675));
#16356=CARTESIAN_POINT('Origin',(0.,0.,10.));
#16357=CARTESIAN_POINT('',(2.36142191786124,0.872635534369624,13.6679749024944));
#16358=CARTESIAN_POINT('',(2.36142200728636,0.872635292378013,13.9438095899177));
#16359=CARTESIAN_POINT('',(2.36142200728636,0.87263529237802,10.));
#16360=CARTESIAN_POINT('',(2.5174999540924,-0.000480775158033205,14.8874166975507));
#16361=CARTESIAN_POINT('Ctrl Pts',(2.36142200728636,0.872635292378013,13.9438095899177));
#16362=CARTESIAN_POINT('Ctrl Pts',(2.33274328543006,0.950242244015014,13.9490591804899));
#16363=CARTESIAN_POINT('Ctrl Pts',(2.30018971864896,1.02655575865372,13.9543087710621));
#16364=CARTESIAN_POINT('Ctrl Pts',(2.26390046374053,1.1011634484832,13.9595583616344));
#16365=CARTESIAN_POINT('Ctrl Pts',(2.22616663310737,1.17874106585397,13.9650169240117));
#16366=CARTESIAN_POINT('Ctrl Pts',(2.18439357996264,1.25447371190632,13.9704754863891));
#16367=CARTESIAN_POINT('Ctrl Pts',(2.13879413279158,1.32791788433484,13.9759340487664));
#16368=CARTESIAN_POINT('Ctrl Pts',(2.09502845327483,1.39840852210115,13.9811730967472));
#16369=CARTESIAN_POINT('Ctrl Pts',(2.04773848948028,1.46679077534903,13.9864121447281));
#16370=CARTESIAN_POINT('Ctrl Pts',(1.99715956760326,1.53269694053676,13.9916511927089));
#16371=CARTESIAN_POINT('Ctrl Pts',(1.94660080083145,1.59857684289319,13.9968881529908));
#16372=CARTESIAN_POINT('Ctrl Pts',(1.89275595920445,1.66198225093666,14.0021251132727));
#16373=CARTESIAN_POINT('Ctrl Pts',(1.83590271087396,1.72257582886956,14.0073620735545));
#16374=CARTESIAN_POINT('Ctrl Pts',(1.77905496837645,1.78316353874514,14.012598526674));
#16375=CARTESIAN_POINT('Ctrl Pts',(1.71919971426181,1.84093962357419,14.0178349797935));
#16376=CARTESIAN_POINT('Ctrl Pts',(1.65665284537889,1.89560217342617,14.023071432913));
#16377=CARTESIAN_POINT('Ctrl Pts',(1.59409316714979,1.95027591794763,14.0283089584369));
#16378=CARTESIAN_POINT('Ctrl Pts',(1.52884112790565,2.00183455884925,14.0335464839608));
#16379=CARTESIAN_POINT('Ctrl Pts',(1.46124612495801,2.05001610049658,14.0387840094848));
#16380=CARTESIAN_POINT('Ctrl Pts',(1.39357582607775,2.09825131288812,14.0440273692324));
#16381=CARTESIAN_POINT('Ctrl Pts',(1.32355773220934,2.14310165189018,14.0492707289801));
#16382=CARTESIAN_POINT('Ctrl Pts',(1.25157017303084,2.18434849600048,14.0545140887277));
#16383=CARTESIAN_POINT('Ctrl Pts',(1.17953513628648,2.22562254341897,14.0597609066001));
#16384=CARTESIAN_POINT('Ctrl Pts',(1.10552845998846,2.26328815725627,14.0650077244724));
#16385=CARTESIAN_POINT('Ctrl Pts',(1.02995087051983,2.29717379715063,14.0702545423448));
#16386=CARTESIAN_POINT('Ctrl Pts',(0.954253109036032,2.33111331684798,14.0755097029108));
#16387=CARTESIAN_POINT('Ctrl Pts',(0.87697987943064,2.36126070341817,14.0807648634769));
#16388=CARTESIAN_POINT('Ctrl Pts',(0.798548999298957,2.38749361166028,14.0860200240429));
#16389=CARTESIAN_POINT('Ctrl Pts',(0.775944111138288,2.39505430657976,14.0875346355921));
#16390=CARTESIAN_POINT('Ctrl Pts',(0.7532431325843,2.4022901592352,14.0890492471413));
#16391=CARTESIAN_POINT('Ctrl Pts',(0.730456218411384,2.40919902934235,14.0905638586905));
#16392=CARTESIAN_POINT('Ctrl Pts',(0.651392436506789,2.43317074377522,14.0958191080976));
#16393=CARTESIAN_POINT('Ctrl Pts',(0.571001358182961,2.453290596041,14.1010743575047));
#16394=CARTESIAN_POINT('Ctrl Pts',(0.489692843030049,2.46941433734502,14.1063296069117));
#16395=CARTESIAN_POINT('Ctrl Pts',(0.408499604880611,2.48551521884673,14.111577405569));
#16396=CARTESIAN_POINT('Ctrl Pts',(0.326391962337084,2.49763115387252,14.1168252042263));
#16397=CARTESIAN_POINT('Ctrl Pts',(0.243794995117869,2.50566762567494,14.1220730028835));
#16398=CARTESIAN_POINT('Ctrl Pts',(0.160599541659662,2.51376232864425,14.1273588263665));
#16399=CARTESIAN_POINT('Ctrl Pts',(0.0769080959480587,2.51771806298627,
14.1326446498495));
#16400=CARTESIAN_POINT('Ctrl Pts',(-0.00683435580937276,2.51749072323627,
14.1379304733324));
#16401=CARTESIAN_POINT('Ctrl Pts',(-0.0898258947777812,2.51726542202612,
14.1431688992008));
#16402=CARTESIAN_POINT('Ctrl Pts',(-0.172867058799017,2.51293176621098,
14.1484073250692));
#16403=CARTESIAN_POINT('Ctrl Pts',(-0.255521276603785,2.50449897728124,
14.1536457509375));
#16404=CARTESIAN_POINT('Ctrl Pts',(-0.338148310811867,2.49606896175544,
14.1588824539748));
#16405=CARTESIAN_POINT('Ctrl Pts',(-0.420388192873449,2.48354253738479,
14.1641191570121));
#16406=CARTESIAN_POINT('Ctrl Pts',(-0.501808273384028,2.46698088901461,
14.1693558600494));
#16407=CARTESIAN_POINT('Ctrl Pts',(-0.583226136052318,2.45041969177546,
14.1745924204415));
#16408=CARTESIAN_POINT('Ctrl Pts',(-0.663823789613585,2.42982358206545,
14.1798289808336));
#16409=CARTESIAN_POINT('Ctrl Pts',(-0.743178965304525,2.40530481967024,
14.1850655412257));
#16410=CARTESIAN_POINT('Ctrl Pts',(-0.823832971322326,2.38038475122412,
14.1903878099965));
#16411=CARTESIAN_POINT('Ctrl Pts',(-0.903202986807447,2.35141259770563,
14.1957100787672));
#16412=CARTESIAN_POINT('Ctrl Pts',(-0.980863698073059,2.31855831408279,
14.201032347538));
#16413=CARTESIAN_POINT('Ctrl Pts',(-1.0573835166936,2.2861866839141,14.2062764282881));
#16414=CARTESIAN_POINT('Ctrl Pts',(-1.13224352479191,2.25004648791044,14.2115205090382));
#16415=CARTESIAN_POINT('Ctrl Pts',(-1.20506057604794,2.21034731615984,14.2167645897883));
#16416=CARTESIAN_POINT('Ctrl Pts',(-1.27950615517514,2.16976028632459,14.2221259525694));
#16417=CARTESIAN_POINT('Ctrl Pts',(-1.35181585815272,2.12545343681934,14.2274873153505));
#16418=CARTESIAN_POINT('Ctrl Pts',(-1.42161207295006,2.0776971300078,14.2328486781316));
#16419=CARTESIAN_POINT('Ctrl Pts',(-1.4914082877474,2.02994082319626,14.2382100409126));
#16420=CARTESIAN_POINT('Ctrl Pts',(-1.55869065048786,1.97873541994997,14.2435714036937));
#16421=CARTESIAN_POINT('Ctrl Pts',(-1.62311953090137,1.92439321304315,14.2489327664748));
#16422=CARTESIAN_POINT('Ctrl Pts',(-1.68627321952089,1.87112656007844,14.2541880158828));
#16423=CARTESIAN_POINT('Ctrl Pts',(-1.74691864447732,1.81464942874646,14.2594432652908));
#16424=CARTESIAN_POINT('Ctrl Pts',(-1.80471166230083,1.75522706962814,14.2646985146988));
#16425=CARTESIAN_POINT('Ctrl Pts',(-1.86242274275407,1.69588895791589,14.269946313357));
#16426=CARTESIAN_POINT('Ctrl Pts',(-1.91728912974502,1.63361424052214,14.2751941120152));
#16427=CARTESIAN_POINT('Ctrl Pts',(-1.96900010803878,1.56870801124469,14.2804419106734));
#16428=CARTESIAN_POINT('Ctrl Pts',(-2.02108577694166,1.50333148039134,14.2857277341562));
#16429=CARTESIAN_POINT('Ctrl Pts',(-2.06996975464811,1.43528544713269,14.2910135576389));
#16430=CARTESIAN_POINT('Ctrl Pts',(-2.11537277239941,1.36491914917743,14.2962993811216));
#16431=CARTESIAN_POINT('Ctrl Pts',(-2.16036866443207,1.29518382094713,14.3015378069909));
#16432=CARTESIAN_POINT('Ctrl Pts',(-2.20194551875351,1.22317006752683,14.3067762328602));
#16433=CARTESIAN_POINT('Ctrl Pts',(-2.23987337836964,1.14924910218411,14.3120146587295));
#16434=CARTESIAN_POINT('Ctrl Pts',(-2.27778876414393,1.07535244821671,14.3172513617677));
#16435=CARTESIAN_POINT('Ctrl Pts',(-2.31205732819042,0.999550238292341,
14.3224880648059));
#16436=CARTESIAN_POINT('Ctrl Pts',(-2.34249483524164,0.922238687578345,
14.3277247678441));
#16437=CARTESIAN_POINT('Ctrl Pts',(-2.37293151319036,0.844929242792407,
14.3329613282371));
#16438=CARTESIAN_POINT('Ctrl Pts',(-2.39953717355716,0.766110968683968,
14.3381978886301));
#16439=CARTESIAN_POINT('Ctrl Pts',(-2.42217607409677,0.686199181049617,
14.3434344490232));
#16440=CARTESIAN_POINT('Ctrl Pts',(-2.44518551240696,0.60497945288248,14.3487567177928));
#16441=CARTESIAN_POINT('Ctrl Pts',(-2.46409702237147,0.522630562025979,
14.3540789865624));
#16442=CARTESIAN_POINT('Ctrl Pts',(-2.4788215982056,0.439601790566655,14.3594012553321));
#16443=CARTESIAN_POINT('Ctrl Pts',(-2.49332985925757,0.357792772451314,
14.3646453360831));
#16444=CARTESIAN_POINT('Ctrl Pts',(-2.50377338992976,0.275324189044946,
14.3698894168341));
#16445=CARTESIAN_POINT('Ctrl Pts',(-2.51011938815899,0.192631532175615,
14.3751334975851));
#16446=CARTESIAN_POINT('Ctrl Pts',(-2.51660731241434,0.108089483019304,
14.3804948603641));
#16447=CARTESIAN_POINT('Ctrl Pts',(-2.5188121995278,0.0233137286734454,
14.385856223143));
#16448=CARTESIAN_POINT('Ctrl Pts',(-2.51675523590462,-0.0612317935935599,
14.391217585922));
#16449=CARTESIAN_POINT('Ctrl Pts',(-2.51469827228144,-0.145777315860577,
14.3965789487009));
#16450=CARTESIAN_POINT('Ctrl Pts',(-2.50837956250467,-0.230092104354747,
14.4019403114799));
#16451=CARTESIAN_POINT('Ctrl Pts',(-2.49787614311308,-0.313721251537898,
14.4073016742588));
#16452=CARTESIAN_POINT('Ctrl Pts',(-2.4875806099061,-0.395695190671064,
14.4125569236655));
#16453=CARTESIAN_POINT('Ctrl Pts',(-2.47322652414794,-0.477313167553763,
14.4178121730721));
#16454=CARTESIAN_POINT('Ctrl Pts',(-2.45484900653005,-0.55814210120581,
14.4230674224788));
#16455=CARTESIAN_POINT('Ctrl Pts',(-2.43649754405725,-0.638856437792109,
14.4283152211356));
#16456=CARTESIAN_POINT('Ctrl Pts',(-2.41413408159974,-0.718783506996741,
14.4335630197925));
#16457=CARTESIAN_POINT('Ctrl Pts',(-2.38784536008661,-0.797496574483465,
14.4388108184493));
#16458=CARTESIAN_POINT('Ctrl Pts',(-2.36136615411844,-0.876779986015132,
14.4440966419324));
#16459=CARTESIAN_POINT('Ctrl Pts',(-2.33090462435669,-0.954831258423609,
14.4493824654155));
#16460=CARTESIAN_POINT('Ctrl Pts',(-2.2966016603855,-1.03122600021263,14.4546682888985));
#16461=CARTESIAN_POINT('Ctrl Pts',(-2.26260628872966,-1.10693571561366,
14.4599067147665));
#16462=CARTESIAN_POINT('Ctrl Pts',(-2.22483829118455,-1.18101806071211,
14.4651451406344));
#16463=CARTESIAN_POINT('Ctrl Pts',(-2.18348383813068,-1.25307804171253,
14.4703835665024));
#16464=CARTESIAN_POINT('Ctrl Pts',(-2.14214298586814,-1.32511432338453,
14.4756202695393));
#16465=CARTESIAN_POINT('Ctrl Pts',(-2.09721825018888,-1.39512916204231,
14.4808569725762));
#16466=CARTESIAN_POINT('Ctrl Pts',(-2.04894166613948,-1.46275230259863,
14.486093675613));
#16467=CARTESIAN_POINT('Ctrl Pts',(-2.00066639712001,-1.53037360113451,
14.4913302360047));
#16468=CARTESIAN_POINT('Ctrl Pts',(-1.94903973020372,-1.59560295615947,
14.4965667963965));
#16469=CARTESIAN_POINT('Ctrl Pts',(-1.89433612399927,-1.65810038879177,
14.5018033567882));
#16470=CARTESIAN_POINT('Ctrl Pts',(-1.83873716720369,-1.72162073594717,
14.5071256255594));
#16471=CARTESIAN_POINT('Ctrl Pts',(-1.77995995396854,-1.78231854680815,
14.5124478943307));
#16472=CARTESIAN_POINT('Ctrl Pts',(-1.71833287930394,-1.83987455167547,
14.5177701631019));
#16473=CARTESIAN_POINT('Ctrl Pts',(-1.65761115144655,-1.89658501672892,
14.5230142438516));
#16474=CARTESIAN_POINT('Ctrl Pts',(-1.59412313651235,-1.9502451186521,14.5282583246014));
#16475=CARTESIAN_POINT('Ctrl Pts',(-1.5282162625524,-2.00059023912204,14.5335024053511));
#16476=CARTESIAN_POINT('Ctrl Pts',(-1.46083540440216,-2.05206131060698,
14.5388637681331));
#16477=CARTESIAN_POINT('Ctrl Pts',(-1.39092660988126,-2.1000670447314,14.5442251309151));
#16478=CARTESIAN_POINT('Ctrl Pts',(-1.31889056096353,-2.14437262111819,
14.5495864936971));
#16479=CARTESIAN_POINT('Ctrl Pts',(-1.24685451204578,-2.188678197505,14.5549478564791));
#16480=CARTESIAN_POINT('Ctrl Pts',(-1.17269168648866,-2.22928343072958,
14.5603092192611));
#16481=CARTESIAN_POINT('Ctrl Pts',(-1.09682559989037,-2.26600526332688,
14.5656705820431));
#16482=CARTESIAN_POINT('Ctrl Pts',(-1.02246107304345,-2.30200028862073,
14.5709258314492));
#16483=CARTESIAN_POINT('Ctrl Pts',(-0.946185439314126,-2.33439722714392,
14.5761810808553));
#16484=CARTESIAN_POINT('Ctrl Pts',(-0.868381085202565,-2.36298974624572,
14.5814363302613));
#16485=CARTESIAN_POINT('Ctrl Pts',(-0.790687039990303,-2.3915417276508,
14.5866841289176));
#16486=CARTESIAN_POINT('Ctrl Pts',(-0.711469008929585,-2.41629984546682,
14.5919319275739));
#16487=CARTESIAN_POINT('Ctrl Pts',(-0.631132159723589,-2.43710452114033,
14.5971797262301));
#16488=CARTESIAN_POINT('Ctrl Pts',(-0.550213200762819,-2.45805994463099,
14.6024655497133));
#16489=CARTESIAN_POINT('Ctrl Pts',(-0.468159568186418,-2.47500418557747,
14.6077513731966));
#16490=CARTESIAN_POINT('Ctrl Pts',(-0.385403945861432,-2.48782436046326,
14.6130371966798));
#16491=CARTESIAN_POINT('Ctrl Pts',(-0.303390387513959,-2.50052957772199,
14.6182756225471));
#16492=CARTESIAN_POINT('Ctrl Pts',(-0.220687842766615,-2.50918432118937,
14.6235140484144));
#16493=CARTESIAN_POINT('Ctrl Pts',(-0.137728990121894,-2.51372969415568,
14.6287524742818));
#16494=CARTESIAN_POINT('Ctrl Pts',(-0.0547974212632767,-2.51827357222446,
14.633989177318));
#16495=CARTESIAN_POINT('Ctrl Pts',(0.0283898277111877,-2.51871073872867,
14.6392258803543));
#16496=CARTESIAN_POINT('Ctrl Pts',(0.111395857847538,-2.51503423691496,
14.6444625833905));
#16497=CARTESIAN_POINT('Ctrl Pts',(0.19439962694111,-2.51135783524732,14.6496991437816));
#16498=CARTESIAN_POINT('Ctrl Pts',(0.277221726088093,-2.50356800950175,
14.6549357041727));
#16499=CARTESIAN_POINT('Ctrl Pts',(0.359427554207529,-2.49170987140887,
14.6601722645637));
#16500=CARTESIAN_POINT('Ctrl Pts',(0.442978870185704,-2.4796576475535,14.6654945333357));
#16501=CARTESIAN_POINT('Ctrl Pts',(0.525893071175531,-2.46340279242345,
14.6708168021077));
#16502=CARTESIAN_POINT('Ctrl Pts',(0.607723561040238,-2.44304693433355,
14.6761390708796));
#16503=CARTESIAN_POINT('Ctrl Pts',(0.688351901128603,-2.42299011869459,
14.6813831516287));
#16504=CARTESIAN_POINT('Ctrl Pts',(0.767927729473984,-2.39895218782986,
14.6866272323778));
#16505=CARTESIAN_POINT('Ctrl Pts',(0.846039928523892,-2.37108048984915,
14.6918713131269));
#16506=CARTESIAN_POINT('Ctrl Pts',(0.925899079622809,-2.34258545107803,
14.6972326759103));
#16507=CARTESIAN_POINT('Ctrl Pts',(1.00422787138072,-2.31008329044402,14.7025940386937));
#16508=CARTESIAN_POINT('Ctrl Pts',(1.08061118635039,-2.27378224857491,14.7079554014771));
#16509=CARTESIAN_POINT('Ctrl Pts',(1.15699450132007,-2.23748120670581,14.7133167642605));
#16510=CARTESIAN_POINT('Ctrl Pts',(1.23143192385297,-2.19738158338615,14.7186781270439));
#16511=CARTESIAN_POINT('Ctrl Pts',(1.30353932303076,-2.15373895431004,14.7240394898273));
#16512=CARTESIAN_POINT('Ctrl Pts',(1.37421955536285,-2.11096011055952,14.7292947392395));
#16513=CARTESIAN_POINT('Ctrl Pts',(1.44292224538896,-2.06461926113376,14.7345499886517));
#16514=CARTESIAN_POINT('Ctrl Pts',(1.50926613194603,-2.01492481074621,14.739805238064));
#16515=CARTESIAN_POINT('Ctrl Pts',(1.57551595794375,-1.9653008157999,14.7450530367264));
#16516=CARTESIAN_POINT('Ctrl Pts',(1.63941325689886,-1.91233293832158,14.7503008353889));
#16517=CARTESIAN_POINT('Ctrl Pts',(1.70060358136297,-1.85627414706326,14.7555486340513));
#16518=CARTESIAN_POINT('Ctrl Pts',(1.76223728240759,-1.79980916160033,14.760834457533));
#16519=CARTESIAN_POINT('Ctrl Pts',(1.82112420930131,-1.74020852606853,14.7661202810147));
#16520=CARTESIAN_POINT('Ctrl Pts',(1.87693410081557,-1.67777371275021,14.7714061044963));
#16521=CARTESIAN_POINT('Ctrl Pts',(1.93224354894996,-1.61589874802058,14.7766445303699));
#16522=CARTESIAN_POINT('Ctrl Pts',(1.98453061063023,-1.55124058003066,14.7818829562434));
#16523=CARTESIAN_POINT('Ctrl Pts',(2.03351031126417,-1.48413006976555,14.7871213821169));
#16524=CARTESIAN_POINT('Ctrl Pts',(2.08247390328959,-1.41704163103055,14.7923580851593));
#16525=CARTESIAN_POINT('Ctrl Pts',(2.12813202276749,-1.3475028242608,14.7975947882018));
#16526=CARTESIAN_POINT('Ctrl Pts',(2.17024096410897,-1.27587632931384,14.8028314912442));
#16527=CARTESIAN_POINT('Ctrl Pts',(2.21234875842374,-1.20425178543714,14.8080680516414));
#16528=CARTESIAN_POINT('Ctrl Pts',(2.25090733386203,-1.13054006474639,14.8133046120386));
#16529=CARTESIAN_POINT('Ctrl Pts',(2.28571791055815,-1.05513026842835,14.8185411724359));
#16530=CARTESIAN_POINT('Ctrl Pts',(2.32109824248877,-0.978486217172226,
14.8238634412005));
#16531=CARTESIAN_POINT('Ctrl Pts',(2.3526065614897,-0.900088443901519,14.8291857099651));
#16532=CARTESIAN_POINT('Ctrl Pts',(2.38008496264434,-0.8203668817025,14.8345079787297));
#16533=CARTESIAN_POINT('Ctrl Pts',(2.40715968604695,-0.74181648739041,14.8397520594849));
#16534=CARTESIAN_POINT('Ctrl Pts',(2.43032203904185,-0.661981407406311,
14.84499614024));
#16535=CARTESIAN_POINT('Ctrl Pts',(2.44947178249304,-0.581286707890679,
14.8502402209951));
#16536=CARTESIAN_POINT('Ctrl Pts',(2.46904980319419,-0.49878729991598,14.8556015837645));
#16537=CARTESIAN_POINT('Ctrl Pts',(2.48443347448112,-0.415389861801244,
14.8609629465339));
#16538=CARTESIAN_POINT('Ctrl Pts',(2.49557145564365,-0.331555967789178,
14.8663243093032));
#16539=CARTESIAN_POINT('Ctrl Pts',(2.50670943680618,-0.247722073777111,
14.8716856720726));
#16540=CARTESIAN_POINT('Ctrl Pts',(2.51360175300079,-0.163452235728656,
14.877047034842));
#16541=CARTESIAN_POINT('Ctrl Pts',(2.51625363846893,-0.0792078082760125,
14.8824083976114));
#16542=CARTESIAN_POINT('Ctrl Pts',(2.51707938858055,-0.0529755873869006,
14.8840778309102));
#16543=CARTESIAN_POINT('Ctrl Pts',(2.5174949411117,-0.0267303865065068,
14.8857472642091));
#16544=CARTESIAN_POINT('Ctrl Pts',(2.51749995409227,-0.000480775830062533,
14.887416697508));
#16545=CARTESIAN_POINT('Ctrl Pts',(2.5174999540924,-0.000480775158034882,
14.8874166975507));
#16546=CARTESIAN_POINT('Ctrl Pts',(2.51751564872697,0.0817015945668656,
14.8926433649588));
#16547=CARTESIAN_POINT('Ctrl Pts',(2.51350287472604,0.164042797258516,14.8978700323668));
#16548=CARTESIAN_POINT('Ctrl Pts',(2.5054410199567,0.246112871500738,14.9030966997749));
#16549=CARTESIAN_POINT('Ctrl Pts',(2.49738907413895,0.328082072133129,14.9083169430044));
#16550=CARTESIAN_POINT('Ctrl Pts',(2.4852979657381,0.409780345309913,14.9135371862339));
#16551=CARTESIAN_POINT('Ctrl Pts',(2.46919906474516,0.490777168032105,14.9187574294635));
#16552=CARTESIAN_POINT('Ctrl Pts',(2.4531173359169,0.571687594125189,14.9239721044324));
#16553=CARTESIAN_POINT('Ctrl Pts',(2.43303639711601,0.651897600727632,14.9291867794013));
#16554=CARTESIAN_POINT('Ctrl Pts',(2.40903928768665,0.730982872837808,14.9344014543702));
#16555=CARTESIAN_POINT('Ctrl Pts',(2.39457884786559,0.778638938308824,14.9375437700643));
#16556=CARTESIAN_POINT('Ctrl Pts',(2.37869738372328,0.825886720026406,14.9406860857585));
#16557=CARTESIAN_POINT('Ctrl Pts',(2.36142200728636,0.872635292378009,14.9438284014526));
#16558=CARTESIAN_POINT('',(2.51749903103506,-0.00220878644373725,14.6120681308043));
#16559=CARTESIAN_POINT('Ctrl Pts',(2.36142197356233,0.872635383637971,14.6670478768675));
#16560=CARTESIAN_POINT('Ctrl Pts',(2.3830264806342,0.814171838973078,14.662898126802));
#16561=CARTESIAN_POINT('Ctrl Pts',(2.40245955452755,0.754906799200612,14.6588100797912));
#16562=CARTESIAN_POINT('Ctrl Pts',(2.42615252031912,0.672413936199539,14.653279758481));
#16563=CARTESIAN_POINT('Ctrl Pts',(2.4323130090463,0.649776915793715,14.6517783272278));
#16564=CARTESIAN_POINT('Ctrl Pts',(2.44152137461929,0.613972427929959,14.6494282374261));
#16565=CARTESIAN_POINT('Ctrl Pts',(2.44478106226665,0.600861326874552,14.6485728408));
#16566=CARTESIAN_POINT('Ctrl Pts',(2.45064178630728,0.57645078367163,14.6469896307871));
#16567=CARTESIAN_POINT('Ctrl Pts',(2.45327059448336,0.565158445280051,14.6462609490147));
#16568=CARTESIAN_POINT('Ctrl Pts',(2.45826314377867,0.543020954942658,14.6448395336263));
#16569=CARTESIAN_POINT('Ctrl Pts',(2.46063335403456,0.532177550106636,14.6441466097339));
#16570=CARTESIAN_POINT('Ctrl Pts',(2.46579440974727,0.507794521789542,14.6425957117803));
#16571=CARTESIAN_POINT('Ctrl Pts',(2.46854561521828,0.494246805671042,14.641738999612));
#16572=CARTESIAN_POINT('Ctrl Pts',(2.47519637313375,0.460054910860904,14.6395889327426));
#16573=CARTESIAN_POINT('Ctrl Pts',(2.47894940738897,0.439383069791684,14.6383001296647));
#16574=CARTESIAN_POINT('Ctrl Pts',(2.50589531034888,0.279609775603074,14.6284185095174));
#16575=CARTESIAN_POINT('Ctrl Pts',(2.51762277134393,0.138826173536537,14.6201945782306));
#16576=CARTESIAN_POINT('Ctrl Pts',(2.51749903103506,-0.00220878644373725,
14.6120681308043));
#16577=CARTESIAN_POINT('Ctrl Pts',(2.51749903223328,-0.0022074203295025,
14.6120682095199));
#16578=CARTESIAN_POINT('Ctrl Pts',(2.51734625288752,-0.176447844755141,
14.6020284594246));
#16579=CARTESIAN_POINT('Ctrl Pts',(2.49910489813037,-0.350188088773951,
14.5921890872909));
#16580=CARTESIAN_POINT('Ctrl Pts',(2.45856792263053,-0.541964218877127,
14.58028939457));
#16581=CARTESIAN_POINT('Ctrl Pts',(2.45378307845243,-0.563231730425828,
14.578954613819));
#16582=CARTESIAN_POINT('Ctrl Pts',(2.44601366715268,-0.595784842741711,
14.5768845090396));
#16583=CARTESIAN_POINT('Ctrl Pts',(2.44322565862868,-0.607116799426908,
14.5761588308346));
#16584=CARTESIAN_POINT('Ctrl Pts',(2.43788093129379,-0.628207433113598,
14.5747980756725));
#16585=CARTESIAN_POINT('Ctrl Pts',(2.43534413365638,-0.637970968568624,
14.5741640632016));
#16586=CARTESIAN_POINT('Ctrl Pts',(2.4310011019985,-0.654282838740212,14.5730975889619));
#16587=CARTESIAN_POINT('Ctrl Pts',(2.42922688704112,-0.660839708525803,
14.572666935467));
#16588=CARTESIAN_POINT('Ctrl Pts',(2.42580703534214,-0.673278382807251,
14.5718460944824));
#16589=CARTESIAN_POINT('Ctrl Pts',(2.42416649032558,-0.679161526251899,
14.5714562138903));
#16590=CARTESIAN_POINT('Ctrl Pts',(2.42021743785845,-0.693126576022748,
14.5705269205205));
#16591=CARTESIAN_POINT('Ctrl Pts',(2.41788984890373,-0.701202945441875,
14.5699864382391));
#16592=CARTESIAN_POINT('Ctrl Pts',(2.40952032669336,-0.729706673432705,
14.5680685148678));
#16593=CARTESIAN_POINT('Ctrl Pts',(2.40325979961571,-0.750068196271464,
14.5666795054453));
#16594=CARTESIAN_POINT('Ctrl Pts',(2.35370687914706,-0.904239703959241,
14.5560304303478));
#16595=CARTESIAN_POINT('Ctrl Pts',(2.29953170732172,-1.03427864219943,14.5463032027858));
#16596=CARTESIAN_POINT('Ctrl Pts',(2.17424252029407,-1.27584085291948,14.5275040961828));
#16597=CARTESIAN_POINT('Ctrl Pts',(2.10463444026818,-1.38766737270961,14.518459516005));
#16598=CARTESIAN_POINT('Ctrl Pts',(1.98310654607306,-1.5525686782299,14.5047892093619));
#16599=CARTESIAN_POINT('Ctrl Pts',(1.93705179352577,-1.60966245078824,14.4999825989861));
#16600=CARTESIAN_POINT('Ctrl Pts',(1.87556965954321,-1.67941389037954,14.4940117351049));
#16601=CARTESIAN_POINT('Ctrl Pts',(1.86240059024153,-1.69400609215391,14.4927567045419));
#16602=CARTESIAN_POINT('Ctrl Pts',(1.840272037548,-1.71795600474581,14.4906864918425));
#16603=CARTESIAN_POINT('Ctrl Pts',(1.8314089940245,-1.72740126004728,14.4898673096871));
#16604=CARTESIAN_POINT('Ctrl Pts',(1.81442698629495,-1.74522118796995,14.4883163569763));
#16605=CARTESIAN_POINT('Ctrl Pts',(1.80632197230322,-1.75360862887468,14.487584020239));
#16606=CARTESIAN_POINT('Ctrl Pts',(1.78769787891087,-1.77261556828376,14.4859188900544));
#16607=CARTESIAN_POINT('Ctrl Pts',(1.77714186327992,-1.78319838272559,14.4849877334615));
#16608=CARTESIAN_POINT('Ctrl Pts',(1.74425669843902,-1.81558496429833,14.4821248942249));
#16609=CARTESIAN_POINT('Ctrl Pts',(1.72161538447477,-1.83706853219827,14.4802070430736));
#16610=CARTESIAN_POINT('Ctrl Pts',(1.54600115794843,-1.99760377336749,14.4657117114391));
#16611=CARTESIAN_POINT('Ctrl Pts',(1.37682758565216,-2.1177569598037,14.4539831362561));
#16612=CARTESIAN_POINT('Ctrl Pts',(1.08310027930611,-2.27614155980993,14.4347518683054));
#16613=CARTESIAN_POINT('Ctrl Pts',(0.966961136711867,-2.32785404201039,
14.4273690924806));
#16614=CARTESIAN_POINT('Ctrl Pts',(0.830949845217222,-2.3764753557936,14.4184476305572));
#16615=CARTESIAN_POINT('Ctrl Pts',(0.814403579517508,-2.38219636722863,
14.4173577332219));
#16616=CARTESIAN_POINT('Ctrl Pts',(0.789869955263508,-2.39039360807982,
14.4157331172956));
#16617=CARTESIAN_POINT('Ctrl Pts',(0.781927364103617,-2.39300349776436,
14.4152058371787));
#16618=CARTESIAN_POINT('Ctrl Pts',(0.767768653602804,-2.39757795361037,
14.414263297133));
#16619=CARTESIAN_POINT('Ctrl Pts',(0.761557715226591,-2.3995579997027,14.4138489416665));
#16620=CARTESIAN_POINT('Ctrl Pts',(0.747999255449551,-2.40382249048615,
14.4129423983532));
#16621=CARTESIAN_POINT('Ctrl Pts',(0.740649038230816,-2.40609734847353,
14.4124496920677));
#16622=CARTESIAN_POINT('Ctrl Pts',(0.720058648621119,-2.41236669095845,
14.4110661722716));
#16623=CARTESIAN_POINT('Ctrl Pts',(0.706796052690527,-2.4162857506115,14.4101712353938));
#16624=CARTESIAN_POINT('Ctrl Pts',(0.629272470710851,-2.43850089894496,
14.4049207295255));
#16625=CARTESIAN_POINT('Ctrl Pts',(0.564341138819439,-2.45434062533898,
14.4004463548239));
#16626=CARTESIAN_POINT('Ctrl Pts',(0.281632269446114,-2.51149508125784,
14.3808460556432));
#16627=CARTESIAN_POINT('Ctrl Pts',(0.0595073510815119,-2.52654052793513,
14.3652553615935));
#16628=CARTESIAN_POINT('Ctrl Pts',(-0.208041459279902,-2.50931864733981,
14.3473976783514));
#16629=CARTESIAN_POINT('Ctrl Pts',(-0.254279203346788,-2.50505565874671,
14.3443398744679));
#16630=CARTESIAN_POINT('Ctrl Pts',(-0.334326927527517,-2.49543606011436,
14.3390958261121));
#16631=CARTESIAN_POINT('Ctrl Pts',(-0.368193388823455,-2.49066445765854,
14.3368926872635));
#16632=CARTESIAN_POINT('Ctrl Pts',(-0.417252711845663,-2.48272966962158,
14.3337223255568));
#16633=CARTESIAN_POINT('Ctrl Pts',(-0.432528988805183,-2.48011393474472,
14.3327381093059));
#16634=CARTESIAN_POINT('Ctrl Pts',(-0.459329796269762,-2.47526970937939,
14.3310163700365));
#16635=CARTESIAN_POINT('Ctrl Pts',(-0.470864587517976,-2.47310140181741,
14.3302769770892));
#16636=CARTESIAN_POINT('Ctrl Pts',(-0.494832769384331,-2.46842209925745,
14.3287438063046));
#16637=CARTESIAN_POINT('Ctrl Pts',(-0.507263217263479,-2.4658976393093,
14.3279504767646));
#16638=CARTESIAN_POINT('Ctrl Pts',(-0.539531970799089,-2.45908995010045,
14.3258954323637));
#16639=CARTESIAN_POINT('Ctrl Pts',(-0.559338750579415,-2.4546605324642,
14.3246383720816));
#16640=CARTESIAN_POINT('Ctrl Pts',(-0.641625057460877,-2.43521099985357,
14.3194316741519));
#16641=CARTESIAN_POINT('Ctrl Pts',(-0.703574407161174,-2.41804040715723,
14.3155504950842));
#16642=CARTESIAN_POINT('Ctrl Pts',(-0.956481779059505,-2.33739710838233,
14.2997607199375));
#16643=CARTESIAN_POINT('Ctrl Pts',(-1.1401326653457,-2.25352569000999,14.2884897134711));
#16644=CARTESIAN_POINT('Ctrl Pts',(-1.36515191545438,-2.11614454985564,
14.2731171892448));
#16645=CARTESIAN_POINT('Ctrl Pts',(-1.41722859017158,-2.08162667313111,
14.2694305399331));
#16646=CARTESIAN_POINT('Ctrl Pts',(-1.48749692717594,-2.03119108300949,
14.2641971492547));
#16647=CARTESIAN_POINT('Ctrl Pts',(-1.50682696767897,-2.01689283964196,
14.2627290230078));
#16648=CARTESIAN_POINT('Ctrl Pts',(-1.54010956402366,-1.99152850417433,
14.2601454566726));
#16649=CARTESIAN_POINT('Ctrl Pts',(-1.55415525788796,-1.98058694456151,
14.2590374023261));
#16650=CARTESIAN_POINT('Ctrl Pts',(-1.57466838556011,-1.96425471319443,
14.2573908186262));
#16651=CARTESIAN_POINT('Ctrl Pts',(-1.58122706855388,-1.95897882980861,
14.2568600202831));
#16652=CARTESIAN_POINT('Ctrl Pts',(-1.5928216166371,-1.9495558738129,14.2559136923239));
#16653=CARTESIAN_POINT('Ctrl Pts',(-1.59786798261398,-1.94542198924811,
14.2554990966046));
#16654=CARTESIAN_POINT('Ctrl Pts',(-1.60879952922023,-1.93639585089276,
14.254594999978));
#16655=CARTESIAN_POINT('Ctrl Pts',(-1.61467839704372,-1.93149643722047,
14.2541050038002));
#16656=CARTESIAN_POINT('Ctrl Pts',(-1.63097763164425,-1.91778633542791,
14.2527361370296));
#16657=CARTESIAN_POINT('Ctrl Pts',(-1.64134865631302,-1.90891776461857,
14.2518532767759));
#16658=CARTESIAN_POINT('Ctrl Pts',(-1.69955808780646,-1.85831609948693,
14.2468330356465));
#16659=CARTESIAN_POINT('Ctrl Pts',(-1.74587270943177,-1.81487284860378,
14.2425883852418));
#16660=CARTESIAN_POINT('Ctrl Pts',(-1.93518223429473,-1.62334243535806,
14.2243171725942));
#16661=CARTESIAN_POINT('Ctrl Pts',(-2.06138052702461,-1.45975881848175,
14.2098472249371));
#16662=CARTESIAN_POINT('Ctrl Pts',(-2.21041326093247,-1.20805166917435,
14.1901938165273));
#16663=CARTESIAN_POINT('Ctrl Pts',(-2.25068743696326,-1.13124912266871,
14.1844848553704));
#16664=CARTESIAN_POINT('Ctrl Pts',(-2.29594132457244,-1.03292057246328,
14.1775261244116));
#16665=CARTESIAN_POINT('Ctrl Pts',(-2.30470694481398,-1.01321143929362,
14.1761480675076));
#16666=CARTESIAN_POINT('Ctrl Pts',(-2.31833302716469,-0.981481650712406,
14.1739556506734));
#16667=CARTESIAN_POINT('Ctrl Pts',(-2.32335565994743,-0.969532229028211,
14.1731358435942));
#16668=CARTESIAN_POINT('Ctrl Pts',(-2.3327213006881,-0.946759509891454,
14.1715843851601));
#16669=CARTESIAN_POINT('Ctrl Pts',(-2.33708181328242,-0.935943823970974,
14.17085216215));
#16670=CARTESIAN_POINT('Ctrl Pts',(-2.34685315966793,-0.911213139548342,
14.169188217121));
#16671=CARTESIAN_POINT('Ctrl Pts',(-2.35221571232524,-0.897279441734802,
14.1682581232099));
#16672=CARTESIAN_POINT('Ctrl Pts',(-2.36837167132169,-0.854160466355362,
14.1654019707286));
#16673=CARTESIAN_POINT('Ctrl Pts',(-2.37874843850869,-0.824821479105153,
14.1634896482738));
#16674=CARTESIAN_POINT('Ctrl Pts',(-2.45277431018102,-0.602493565493219,
14.1492127929861));
#16675=CARTESIAN_POINT('Ctrl Pts',(-2.49339098942343,-0.402629297198246,
14.1376649399018));
#16676=CARTESIAN_POINT('Ctrl Pts',(-2.51985688868026,-0.0706115310829718,
14.1184822633901));
#16677=CARTESIAN_POINT('Ctrl Pts',(-2.52014421841247,0.0594062770241095,
14.1109459826088));
#16678=CARTESIAN_POINT('Ctrl Pts',(-2.50905593034063,0.206806568299369,
14.1018223742667));
#16679=CARTESIAN_POINT('Ctrl Pts',(-2.50751227584696,0.224750443401174,
14.10070175336));
#16680=CARTESIAN_POINT('Ctrl Pts',(-2.50496111858431,0.251092725249343,
14.0990399816989));
#16681=CARTESIAN_POINT('Ctrl Pts',(-2.50410355922615,0.259505533805276,
14.0985067675563));
#16682=CARTESIAN_POINT('Ctrl Pts',(-2.50250904005756,0.274403636921412,
14.0975578195258));
#16683=CARTESIAN_POINT('Ctrl Pts',(-2.50178922407814,0.280890598715556,
14.0971430397181));
#16684=CARTESIAN_POINT('Ctrl Pts',(-2.50017372047505,0.294950445521417,
14.0962405378494));
#16685=CARTESIAN_POINT('Ctrl Pts',(-2.49926886428486,0.302521963207046,
14.0957523359419));
#16686=CARTESIAN_POINT('Ctrl Pts',(-2.49666373648765,0.323510986334988,
14.0943931419138));
#16687=CARTESIAN_POINT('Ctrl Pts',(-2.4948897453465,0.336918848998842,14.0935182473147));
#16688=CARTESIAN_POINT('Ctrl Pts',(-2.48444998949582,0.411213869045681,
14.0886358709595));
#16689=CARTESIAN_POINT('Ctrl Pts',(-2.47366400130315,0.471777145237108,
14.0845277090296));
#16690=CARTESIAN_POINT('Ctrl Pts',(-2.42302078937919,0.706071695280246,
14.0682805594306));
#16691=CARTESIAN_POINT('Ctrl Pts',(-2.3669790430704,0.875775041830177,14.055786168493));
#16692=CARTESIAN_POINT('Ctrl Pts',(-2.24668794350813,1.14152381647296,14.0359628702875));
#16693=CARTESIAN_POINT('Ctrl Pts',(-2.19295215680885,1.24163217314924,14.0284177440001));
#16694=CARTESIAN_POINT('Ctrl Pts',(-2.12033774262357,1.35739078723631,14.0196181388173));
#16695=CARTESIAN_POINT('Ctrl Pts',(-2.10776908820302,1.37682657633483,14.0181376283125));
#16696=CARTESIAN_POINT('Ctrl Pts',(-2.08755617416093,1.40715758233037,14.0158216603069));
#16697=CARTESIAN_POINT('Ctrl Pts',(-2.08009074729203,1.41816985437632,14.0149796300023));
#16698=CARTESIAN_POINT('Ctrl Pts',(-2.06594775968526,1.43868025901438,14.0134089364747));
#16699=CARTESIAN_POINT('Ctrl Pts',(-2.05929113966803,1.4481923362499,14.0126795134833));
#16700=CARTESIAN_POINT('Ctrl Pts',(-2.04423762951421,1.46938960130097,14.011051619493));
#16701=CARTESIAN_POINT('Ctrl Pts',(-2.0358058361225,1.48104959320312,14.0101545057334));
#16702=CARTESIAN_POINT('Ctrl Pts',(-2.01409004084545,1.51054362307848,14.0078805318625));
#16703=CARTESIAN_POINT('Ctrl Pts',(-2.00066869935664,1.52827534613825,14.0065089783501));
#16704=CARTESIAN_POINT('Ctrl Pts',(-1.88772051990814,1.67345947361546,13.9952350160761));
#16705=CARTESIAN_POINT('Ctrl Pts',(-1.77635704373441,1.79123434184884,13.9858393255165));
#16706=CARTESIAN_POINT('Ctrl Pts',(-1.56104769672598,1.97896254655044,13.9694063071358));
#16707=CARTESIAN_POINT('Ctrl Pts',(-1.46176418007724,2.05338858387265,13.9623434537998));
#16708=CARTESIAN_POINT('Ctrl Pts',(-1.32045192267171,2.14386075074272,13.9524218009888));
#16709=CARTESIAN_POINT('Ctrl Pts',(-1.28288173889696,2.16655168742379,13.9497946556163));
#16710=CARTESIAN_POINT('Ctrl Pts',(-1.22045084330304,2.20206422283044,13.9454144714827));
#16711=CARTESIAN_POINT('Ctrl Pts',(-1.19593454325564,2.21547455880243,13.9436908091261));
#16712=CARTESIAN_POINT('Ctrl Pts',(-1.16229325002607,2.23315514986017,13.9413137920888));
#16713=CARTESIAN_POINT('Ctrl Pts',(-1.15335736693984,2.23778334484619,13.9406812865326));
#16714=CARTESIAN_POINT('Ctrl Pts',(-1.13834831049038,2.24544326283981,13.9396166395329));
#16715=CARTESIAN_POINT('Ctrl Pts',(-1.13229007603068,2.24850428162906,13.9391862927821));
#16716=CARTESIAN_POINT('Ctrl Pts',(-1.12075323698775,2.25427500298419,13.9383654701466));
#16717=CARTESIAN_POINT('Ctrl Pts',(-1.11527700965938,2.25698932144274,13.9379752975234));
#16718=CARTESIAN_POINT('Ctrl Pts',(-1.10223101886484,2.26339655617169,13.9370445816514));
#16719=CARTESIAN_POINT('Ctrl Pts',(-1.09465255675428,2.26707145115132,13.9365029614504));
#16720=CARTESIAN_POINT('Ctrl Pts',(-1.06774768714296,2.27995161696867,13.9345770817294));
#16721=CARTESIAN_POINT('Ctrl Pts',(-1.04832307777891,2.28894804489453,13.9331811320847));
#16722=CARTESIAN_POINT('Ctrl Pts',(-0.903741556202521,2.3536840314239,13.9227627370341));
#16723=CARTESIAN_POINT('Ctrl Pts',(-0.774345782399214,2.39936638469497,
13.9132971001229));
#16724=CARTESIAN_POINT('Ctrl Pts',(-0.51401932129544,2.46801102296908,13.8946973100706));
#16725=CARTESIAN_POINT('Ctrl Pts',(-0.383678003792294,2.49160426722687,
13.885592891985));
#16726=CARTESIAN_POINT('Ctrl Pts',(-0.176694737400621,2.51243411061752,
13.8716927581285));
#16727=CARTESIAN_POINT('Ctrl Pts',(-0.101003386376267,2.51661408809667,
13.8667213425273));
#16728=CARTESIAN_POINT('Ctrl Pts',(-0.00452354997097181,2.51758111374386,
13.8605243958234));
#16729=CARTESIAN_POINT('Ctrl Pts',(0.0161870093766731,2.51753314762102,
13.8592022145615));
#16730=CARTESIAN_POINT('Ctrl Pts',(0.0496678897407512,2.51704241700615,
13.8570772958137));
#16731=CARTESIAN_POINT('Ctrl Pts',(0.0624392199115469,2.51675799032433,
13.856269689167));
#16732=CARTESIAN_POINT('Ctrl Pts',(0.086910777936425,2.51602659831334,13.8547276690753));
#16733=CARTESIAN_POINT('Ctrl Pts',(0.0986111028927149,2.51559519489167,
13.8539927932796));
#16734=CARTESIAN_POINT('Ctrl Pts',(0.125334640486415,2.51442313613797,13.8523196060479));
#16735=CARTESIAN_POINT('Ctrl Pts',(0.140355169244816,2.5136294320329,13.8513829638745));
#16736=CARTESIAN_POINT('Ctrl Pts',(0.18788779452626,2.5106903454381,13.8484303244437));
#16737=CARTESIAN_POINT('Ctrl Pts',(0.220366614327333,2.5080483524544,13.8464297136977));
#16738=CARTESIAN_POINT('Ctrl Pts',(0.436300996766045,2.48625589844649,13.833223247049));
#16739=CARTESIAN_POINT('Ctrl Pts',(0.61722731865483,2.44762461749861,13.8226674440063));
#16740=CARTESIAN_POINT('Ctrl Pts',(0.836793098595791,2.37482177662283,13.8093699713131));
#16741=CARTESIAN_POINT('Ctrl Pts',(0.880841212095109,2.35883865038029,13.806673117886));
#16742=CARTESIAN_POINT('Ctrl Pts',(1.01700119319479,2.30508623794732,13.7981792328358));
#16743=CARTESIAN_POINT('Ctrl Pts',(1.1073262797376,2.2630815336638,13.7923159518788));
#16744=CARTESIAN_POINT('Ctrl Pts',(1.21069705728322,2.20733783001997,13.7850662566939));
#16745=CARTESIAN_POINT('Ctrl Pts',(1.22638494623779,2.19866040615993,13.7839506642353));
#16746=CARTESIAN_POINT('Ctrl Pts',(1.24932050047618,2.18565225633742,13.7822949683913));
#16747=CARTESIAN_POINT('Ctrl Pts',(1.25664158595892,2.1814512183681,13.7817627190394));
#16748=CARTESIAN_POINT('Ctrl Pts',(1.26958483535283,2.17393725287522,13.7808148191869));
#16749=CARTESIAN_POINT('Ctrl Pts',(1.27521542841474,2.1706391785228,13.7804001147086));
#16750=CARTESIAN_POINT('Ctrl Pts',(1.28740736463745,2.16343403895374,13.7794969840274));
#16751=CARTESIAN_POINT('Ctrl Pts',(1.2939636709954,2.15951906171134,13.7790080718642));
#16752=CARTESIAN_POINT('Ctrl Pts',(1.31212344879682,2.14856289760869,13.7776450515702));
#16753=CARTESIAN_POINT('Ctrl Pts',(1.32368774293938,2.14145773008418,13.7767670065763));
#16754=CARTESIAN_POINT('Ctrl Pts',(1.38793472415581,2.10126479117447,13.7718348928233));
#16755=CARTESIAN_POINT('Ctrl Pts',(1.43943009917202,2.06632914607376,13.7676778134186));
#16756=CARTESIAN_POINT('Ctrl Pts',(1.63267084545332,1.92449976028815,13.7514248972784));
#16757=CARTESIAN_POINT('Ctrl Pts',(1.76426015988295,1.80463410216423,13.7389823071638));
#16758=CARTESIAN_POINT('Ctrl Pts',(1.9574622483997,1.58713804180118,13.7192133243873));
#16759=CARTESIAN_POINT('Ctrl Pts',(2.02696643708287,1.49735732030823,13.7116735878293));
#16760=CARTESIAN_POINT('Ctrl Pts',(2.103085049424,1.3839707358866,13.7028792834288));
#16761=CARTESIAN_POINT('Ctrl Pts',(2.1157176192637,1.36458079160921,13.7013990108488));
#16762=CARTESIAN_POINT('Ctrl Pts',(2.13518878351653,1.33377362379436,13.6990833292935));
#16763=CARTESIAN_POINT('Ctrl Pts',(2.14220702886513,1.32247203271281,13.6982413502282));
#16764=CARTESIAN_POINT('Ctrl Pts',(2.15518181285156,1.3012042071963,13.696670703484));
#16765=CARTESIAN_POINT('Ctrl Pts',(2.16115960237255,1.29125141456129,13.6959412764584));
#16766=CARTESIAN_POINT('Ctrl Pts',(2.17439198684188,1.26887068110694,13.6943133111727));
#16767=CARTESIAN_POINT('Ctrl Pts',(2.18160934280137,1.25642111045781,13.6934161307));
#16768=CARTESIAN_POINT('Ctrl Pts',(2.1997088306205,1.224574191558,13.6911418696493));
#16769=CARTESIAN_POINT('Ctrl Pts',(2.21044152737758,1.20509302236417,13.6897700980273));
#16770=CARTESIAN_POINT('Ctrl Pts',(2.27483086218884,1.08446320456598,13.6813894162444));
#16771=CARTESIAN_POINT('Ctrl Pts',(2.32176837437179,0.979941211286028,13.6746219436779));
#16772=CARTESIAN_POINT('Ctrl Pts',(2.36142191786124,0.872635534369624,13.6679749024944));
#16773=CARTESIAN_POINT('Origin',(0.,0.,10.));
#16774=CARTESIAN_POINT('',(2.36142200728627,0.872635292378268,12.6712695847815));
#16775=CARTESIAN_POINT('',(2.36142200728636,0.872635292378013,12.9436566100381));
#16776=CARTESIAN_POINT('',(2.36142200728636,0.87263529237802,10.));
#16777=CARTESIAN_POINT('',(2.51749904018606,0.00219833170478317,13.8874166975433));
#16778=CARTESIAN_POINT('Ctrl Pts',(2.36142200728636,0.872635292378012,12.9436566100381));
#16779=CARTESIAN_POINT('Ctrl Pts',(2.33220137935874,0.951708685876645,12.9489830833342));
#16780=CARTESIAN_POINT('Ctrl Pts',(2.29903614731653,1.0292286051767,12.9543095566304));
#16781=CARTESIAN_POINT('Ctrl Pts',(2.26213002722283,1.10479590419989,12.9596360299265));
#16782=CARTESIAN_POINT('Ctrl Pts',(2.22515491740963,1.1805044634463,12.9649724601592));
#16783=CARTESIAN_POINT('Ctrl Pts',(2.18442517141745,1.25425272759434,12.970308890392));
#16784=CARTESIAN_POINT('Ctrl Pts',(2.14018926508127,1.3256681936408,12.9756453206247));
#16785=CARTESIAN_POINT('Ctrl Pts',(2.12268150483724,1.35393312502382,12.9777573818169));
#16786=CARTESIAN_POINT('Ctrl Pts',(2.10462498722126,1.38183298711463,12.9798694430091));
#16787=CARTESIAN_POINT('Ctrl Pts',(2.08603685581894,1.40934612007307,12.9819815042013));
#16788=CARTESIAN_POINT('Ctrl Pts',(2.0397857022557,1.47780454173607,12.9872367536086));
#16789=CARTESIAN_POINT('Ctrl Pts',(1.99007561770278,1.54411020833861,12.9924920030159));
#16790=CARTESIAN_POINT('Ctrl Pts',(1.93713376492469,1.60789272863233,12.9977472524232));
#16791=CARTESIAN_POINT('Ctrl Pts',(1.8842669716669,1.67158481980191,13.0029950510807));
#16792=CARTESIAN_POINT('Ctrl Pts',(1.82817780344527,1.73276051803573,13.0082428497382));
#16793=CARTESIAN_POINT('Ctrl Pts',(1.7691365941095,1.79107843529608,13.0134906483957));
#16794=CARTESIAN_POINT('Ctrl Pts',(1.70966758031253,1.84981891614298,13.0187764718786));
#16795=CARTESIAN_POINT('Ctrl Pts',(1.64720383001802,1.90565963442675,13.0240622953615));
#16796=CARTESIAN_POINT('Ctrl Pts',(1.58206291381047,1.95828577759875,13.0293481188444));
#16797=CARTESIAN_POINT('Ctrl Pts',(1.51750611170216,2.01044002577748,13.034586544713));
#16798=CARTESIAN_POINT('Ctrl Pts',(1.45032032884751,2.05943682238185,13.0398249705816));
#16799=CARTESIAN_POINT('Ctrl Pts',(1.38085022903217,2.10500805104917,13.0450633964502));
#16800=CARTESIAN_POINT('Ctrl Pts',(1.31140297677652,2.15056429209778,13.0503000994877));
#16801=CARTESIAN_POINT('Ctrl Pts',(1.2396732851439,2.19269694983328,13.0555368025252));
#16802=CARTESIAN_POINT('Ctrl Pts',(1.16603553866809,2.23118071266382,13.0607735055627));
#16803=CARTESIAN_POINT('Ctrl Pts',(1.09239979804759,2.26966342721594,13.066010065955));
#16804=CARTESIAN_POINT('Ctrl Pts',(1.01685651534262,2.30449723168073,13.0712466263474));
#16805=CARTESIAN_POINT('Ctrl Pts',(0.939804222611933,2.33550300217336,13.0764831867397));
#16806=CARTESIAN_POINT('Ctrl Pts',(0.861490791548575,2.36701625355094,13.0818054555102));
#16807=CARTESIAN_POINT('Ctrl Pts',(0.781618959217072,2.39457483546,13.0871277242807));
#16808=CARTESIAN_POINT('Ctrl Pts',(0.700625999890145,2.4180424847959,13.0924499930512));
#16809=CARTESIAN_POINT('Ctrl Pts',(0.620822886361808,2.44116537720234,13.0976940738015));
#16810=CARTESIAN_POINT('Ctrl Pts',(0.539931837104895,2.46031668865462,13.1029381545518));
#16811=CARTESIAN_POINT('Ctrl Pts',(0.458382389107529,2.47541750728156,13.1081822353021));
#16812=CARTESIAN_POINT('Ctrl Pts',(0.375009116253195,2.49085605043086,13.1135435980827));
#16813=CARTESIAN_POINT('Ctrl Pts',(0.290948147124334,2.50206067115165,13.1189049608633));
#16814=CARTESIAN_POINT('Ctrl Pts',(0.206663042294907,2.50900311616973,13.1242663236438));
#16815=CARTESIAN_POINT('Ctrl Pts',(0.122377937465491,2.51594556118781,13.1296276864244));
#16816=CARTESIAN_POINT('Ctrl Pts',(0.0378692069044778,2.51862588116019,
13.1349890492049));
#16817=CARTESIAN_POINT('Ctrl Pts',(-0.0464026301349656,2.51707231638595,
13.1403504119855));
#16818=CARTESIAN_POINT('Ctrl Pts',(-0.129006538839045,2.51554950013696,
13.1456056613928));
#16819=CARTESIAN_POINT('Ctrl Pts',(-0.211687953583377,2.50995328840564,
13.1508609108001));
#16820=CARTESIAN_POINT('Ctrl Pts',(-0.294012513924601,2.50027256347298,
13.1561161602074));
#16821=CARTESIAN_POINT('Ctrl Pts',(-0.376220356740822,2.49060556360911,
13.1613639588649));
#16822=CARTESIAN_POINT('Ctrl Pts',(-0.458071895655358,2.47686560642358,
13.1666117575223));
#16823=CARTESIAN_POINT('Ctrl Pts',(-0.539133593329459,2.45909357661388,
13.1718595561798));
#16824=CARTESIAN_POINT('Ctrl Pts',(-0.620782652887027,2.44119277312683,
13.1771453796627));
#16825=CARTESIAN_POINT('Ctrl Pts',(-0.70162990293876,2.41920122751533,13.1824312031456));
#16826=CARTESIAN_POINT('Ctrl Pts',(-0.781238379347123,2.39321391535213,
13.1877170266285));
#16827=CARTESIAN_POINT('Ctrl Pts',(-0.860133012042394,2.36745962962336,
13.1929554524971));
#16828=CARTESIAN_POINT('Ctrl Pts',(-0.937810551387549,2.33778109568812,
13.1981938783657));
#16829=CARTESIAN_POINT('Ctrl Pts',(-1.01385845070989,2.30432143849857,13.2034323042343));
#16830=CARTESIAN_POINT('Ctrl Pts',(-1.08988133914377,2.27087278563343,13.2086690072718));
#16831=CARTESIAN_POINT('Ctrl Pts',(-1.16427522998869,2.23364566494832,13.2139057103093));
#16832=CARTESIAN_POINT('Ctrl Pts',(-1.23664729937582,2.19283143605396,13.2191424133468));
#16833=CARTESIAN_POINT('Ctrl Pts',(-1.30901739738391,2.15201831891883,13.2243789737391));
#16834=CARTESIAN_POINT('Ctrl Pts',(-1.37936538202707,2.10761851540647,13.2296155341314));
#16835=CARTESIAN_POINT('Ctrl Pts',(-1.44732402417111,2.05986878685443,13.2348520945238));
#16836=CARTESIAN_POINT('Ctrl Pts',(-1.5163949661006,2.01133752395814,13.2401743632943));
#16837=CARTESIAN_POINT('Ctrl Pts',(-1.58299723579261,1.95934596013539,13.2454966320647));
#16838=CARTESIAN_POINT('Ctrl Pts',(-1.64677846214582,1.90418668901257,13.2508189008352));
#16839=CARTESIAN_POINT('Ctrl Pts',(-1.70962269564365,1.84983774791796,13.2560629815856));
#16840=CARTESIAN_POINT('Ctrl Pts',(-1.76972792598289,1.79241392127716,13.2613070623359));
#16841=CARTESIAN_POINT('Ctrl Pts',(-1.82679410041109,1.73223253771058,13.2665511430862));
#16842=CARTESIAN_POINT('Ctrl Pts',(-1.88513653985392,1.6707052185675,13.2719125058668));
#16843=CARTESIAN_POINT('Ctrl Pts',(-1.94030201513782,1.60629589941926,13.2772738686474));
#16844=CARTESIAN_POINT('Ctrl Pts',(-1.99201444135622,1.53937802875976,13.2826352314279));
#16845=CARTESIAN_POINT('Ctrl Pts',(-2.04372686757461,1.47246015810027,13.2879965942085));
#16846=CARTESIAN_POINT('Ctrl Pts',(-2.09198600956482,1.40303419126785,13.2933579569891));
#16847=CARTESIAN_POINT('Ctrl Pts',(-2.13656482464556,1.33150178373418,13.2987193197697));
#16848=CARTESIAN_POINT('Ctrl Pts',(-2.18026132516609,1.26138516270311,13.303974569177));
#16849=CARTESIAN_POINT('Ctrl Pts',(-2.22058329126614,1.18898576367435,13.3092298185843));
#16850=CARTESIAN_POINT('Ctrl Pts',(-2.25728490926731,1.11466187177729,13.3144850679916));
#16851=CARTESIAN_POINT('Ctrl Pts',(-2.29393449271176,1.04044335427459,13.3197328666491));
#16852=CARTESIAN_POINT('Ctrl Pts',(-2.3269737207614,0.964306173763971,13.3249806653067));
#16853=CARTESIAN_POINT('Ctrl Pts',(-2.3562008471042,0.886636237757878,13.3302284639642));
#16854=CARTESIAN_POINT('Ctrl Pts',(-2.38563974917403,0.808403516106258,
13.3355142874471));
#16855=CARTESIAN_POINT('Ctrl Pts',(-2.4112108218721,0.728616135146873,13.34080011093));
#16856=CARTESIAN_POINT('Ctrl Pts',(-2.43275582416933,0.647692326626021,
13.3460859344129));
#16857=CARTESIAN_POINT('Ctrl Pts',(-2.45410763391817,0.567494156310112,
13.3513243602815));
#16858=CARTESIAN_POINT('Ctrl Pts',(-2.47150516617186,0.486180311444701,
13.3565627861501));
#16859=CARTESIAN_POINT('Ctrl Pts',(-2.48484386135612,0.404174757599766,
13.3618012120187));
#16860=CARTESIAN_POINT('Ctrl Pts',(-2.49817816966551,0.322196174016748,
13.3670379150562));
#16861=CARTESIAN_POINT('Ctrl Pts',(-2.50745621803746,0.239526788341009,
13.3722746180937));
#16862=CARTESIAN_POINT('Ctrl Pts',(-2.51262464386851,0.156600284241947,
13.3775113211312));
#16863=CARTESIAN_POINT('Ctrl Pts',(-2.51779292891423,0.0736760390193401,
13.3827478815236));
#16864=CARTESIAN_POINT('Ctrl Pts',(-2.51885178631918,-0.00950485011003217,
13.3879844419159));
#16865=CARTESIAN_POINT('Ctrl Pts',(-2.51579987119137,-0.092505449101692,
13.3932210023083));
#16866=CARTESIAN_POINT('Ctrl Pts',(-2.51269800443956,-0.176864544165065,
13.3985432710788));
#16867=CARTESIAN_POINT('Ctrl Pts',(-2.50534959151287,-0.261036902242081,
13.4038655398492));
#16868=CARTESIAN_POINT('Ctrl Pts',(-2.49380820869165,-0.344567654114772,
13.4091878086197));
#16869=CARTESIAN_POINT('Ctrl Pts',(-2.48243637722363,-0.426871278161132,
13.41443188937));
#16870=CARTESIAN_POINT('Ctrl Pts',(-2.46699410093623,-0.508551573724599,
13.4196759701204));
#16871=CARTESIAN_POINT('Ctrl Pts',(-2.44758418843864,-0.589184088808537,
13.4249200508707));
#16872=CARTESIAN_POINT('Ctrl Pts',(-2.42774018004294,-0.671619921865025,
13.4302814136513));
#16873=CARTESIAN_POINT('Ctrl Pts',(-2.40374906918141,-0.752960051296445,
13.4356427764318));
#16874=CARTESIAN_POINT('Ctrl Pts',(-2.37577378671128,-0.832769574597652,
13.4410041392123));
#16875=CARTESIAN_POINT('Ctrl Pts',(-2.34779850424114,-0.912579097898858,
13.4463655019928));
#16876=CARTESIAN_POINT('Ctrl Pts',(-2.315839304062,-0.990857569907541,13.4517268647733));
#16877=CARTESIAN_POINT('Ctrl Pts',(-2.28010947794251,-1.0671958670257,13.4570882275539));
#16878=CARTESIAN_POINT('Ctrl Pts',(-2.245086825079,-1.14202325832673,13.4623434769612));
#16879=CARTESIAN_POINT('Ctrl Pts',(-2.20631212510925,-1.21526297823414,
13.4675987263685));
#16880=CARTESIAN_POINT('Ctrl Pts',(-2.16395207119476,-1.2865137712329,13.4728539757758));
#16881=CARTESIAN_POINT('Ctrl Pts',(-2.12165207421362,-1.35766354679352,
13.4781017744333));
#16882=CARTESIAN_POINT('Ctrl Pts',(-2.07577705387296,-1.42682960317198,
13.4833495730908));
#16883=CARTESIAN_POINT('Ctrl Pts',(-2.02654086532252,-1.49363260917063,
13.4885973717483));
#16884=CARTESIAN_POINT('Ctrl Pts',(-1.97694791813944,-1.5609196605387,13.4938831952312));
#16885=CARTESIAN_POINT('Ctrl Pts',(-1.92394508898363,-1.62580884315633,
13.4991690187141));
#16886=CARTESIAN_POINT('Ctrl Pts',(-1.86779703284198,-1.68793971874196,
13.504454842197));
#16887=CARTESIAN_POINT('Ctrl Pts',(-1.81215245244416,-1.74951347105478,
13.5096932680656));
#16888=CARTESIAN_POINT('Ctrl Pts',(-1.75341914028644,-1.80837783666129,
13.5149316939342));
#16889=CARTESIAN_POINT('Ctrl Pts',(-1.69189578779466,-1.86421428308086,
13.5201701198028));
#16890=CARTESIAN_POINT('Ctrl Pts',(-1.63039266930961,-1.92003236582247,
13.5254068228403));
#16891=CARTESIAN_POINT('Ctrl Pts',(-1.56610167430368,-1.97282419729961,
13.5306435258778));
#16892=CARTESIAN_POINT('Ctrl Pts',(-1.49935751994023,-2.0223088976214,13.5358802289153));
#16893=CARTESIAN_POINT('Ctrl Pts',(-1.43261518365407,-2.07179225000477,
13.5411167893076));
#16894=CARTESIAN_POINT('Ctrl Pts',(-1.3634201921449,-2.11796837636223,13.5463533496999));
#16895=CARTESIAN_POINT('Ctrl Pts',(-1.2921383100898,-2.16059825918616,13.5515899100923));
#16896=CARTESIAN_POINT('Ctrl Pts',(-1.21968973577027,-2.20392587828038,
13.5569121788628));
#16897=CARTESIAN_POINT('Ctrl Pts',(-1.14508575630031,-2.24358985796068,
13.5622344476332));
#16898=CARTESIAN_POINT('Ctrl Pts',(-1.06873708216018,-2.27938748334191,
13.5675567164037));
#16899=CARTESIAN_POINT('Ctrl Pts',(-0.993510025873233,-2.31465921542922,
13.5728007971541));
#16900=CARTESIAN_POINT('Ctrl Pts',(-0.916589652672846,-2.34617731763926,
13.5780448779044));
#16901=CARTESIAN_POINT('Ctrl Pts',(-0.838387963927007,-2.3737969314881,
13.5832889586547));
#16902=CARTESIAN_POINT('Ctrl Pts',(-0.758437321787748,-2.40203424833212,
13.5886503214353));
#16903=CARTESIAN_POINT('Ctrl Pts',(-0.677147850984717,-2.42619645007277,
13.5940116842158));
#16904=CARTESIAN_POINT('Ctrl Pts',(-0.594973052343611,-2.44618341850829,
13.5993730469964));
#16905=CARTESIAN_POINT('Ctrl Pts',(-0.512798253702505,-2.46617038694382,
13.6047344097769));
#16906=CARTESIAN_POINT('Ctrl Pts',(-0.429738638858063,-2.48198209267391,
13.6100957725575));
#16907=CARTESIAN_POINT('Ctrl Pts',(-0.346253504564394,-2.49357469520704,
13.615457135338));
#16908=CARTESIAN_POINT('Ctrl Pts',(-0.264420727998077,-2.50493785418069,
13.6207123847453));
#16909=CARTESIAN_POINT('Ctrl Pts',(-0.18187687004404,-2.51228941481937,
13.6259676341526));
#16910=CARTESIAN_POINT('Ctrl Pts',(-0.0990492570846659,-2.51555073386942,
13.6312228835598));
#16911=CARTESIAN_POINT('Ctrl Pts',(-0.0163390748644514,-2.51880742910993,
13.6364706822173));
#16912=CARTESIAN_POINT('Ctrl Pts',(0.0666536060586472,-2.51798538333182,
13.6417184808747));
#16913=CARTESIAN_POINT('Ctrl Pts',(0.149494171832415,-2.51305744912211,
13.6469662795322));
#16914=CARTESIAN_POINT('Ctrl Pts',(0.232934988923193,-2.50809380778062,
13.6522521030151));
#16915=CARTESIAN_POINT('Ctrl Pts',(0.316221007768245,-2.49896446036265,
13.657537926498));
#16916=CARTESIAN_POINT('Ctrl Pts',(0.398905803696967,-2.4856951562444,13.6628237499809));
#16917=CARTESIAN_POINT('Ctrl Pts',(0.48084917076703,-2.47254483706041,13.6680621758495));
#16918=CARTESIAN_POINT('Ctrl Pts',(0.562201589998596,-2.45532858368356,
13.673300601718));
#16919=CARTESIAN_POINT('Ctrl Pts',(0.642533255791257,-2.4341235106712,13.6785390275865));
#16920=CARTESIAN_POINT('Ctrl Pts',(0.7228385018361,-2.41292541165441,13.683775730624));
#16921=CARTESIAN_POINT('Ctrl Pts',(0.802123215391075,-2.38774121609487,
13.6890124336615));
#16922=CARTESIAN_POINT('Ctrl Pts',(0.879969559288569,-2.35869875667188,
13.6942491366989));
#16923=CARTESIAN_POINT('Ctrl Pts',(0.957813782690483,-2.329657088351,13.6994856970912));
#16924=CARTESIAN_POINT('Ctrl Pts',(1.03421928238141,-2.29675752737838,13.7047222574835));
#16925=CARTESIAN_POINT('Ctrl Pts',(1.10878643117052,-2.26017674088823,13.7099588178758));
#16926=CARTESIAN_POINT('Ctrl Pts',(1.18457404318631,-2.22299722552834,13.7152810866463));
#16927=CARTESIAN_POINT('Ctrl Pts',(1.25846213642482,-2.18201509875874,13.7206033554169));
#16928=CARTESIAN_POINT('Ctrl Pts',(1.33005706324213,-2.13746449292607,13.7259256241874));
#16929=CARTESIAN_POINT('Ctrl Pts',(1.40060020822942,-2.09356836807152,13.7311697049377));
#16930=CARTESIAN_POINT('Ctrl Pts',(1.4689167664711,-2.04620823240741,13.736413785688));
#16931=CARTESIAN_POINT('Ctrl Pts',(1.53466091700049,-1.99565080107498,13.7416578664382));
#16932=CARTESIAN_POINT('Ctrl Pts',(1.60187541244369,-1.9439626704877,13.7470192292189));
#16933=CARTESIAN_POINT('Ctrl Pts',(1.66640066013281,-1.88893283796649,13.7523805919996));
#16934=CARTESIAN_POINT('Ctrl Pts',(1.7279057724601,-1.83088718699407,13.7577419547802));
#16935=CARTESIAN_POINT('Ctrl Pts',(1.7894108847874,-1.77284153602164,13.7631033175609));
#16936=CARTESIAN_POINT('Ctrl Pts',(1.8478955585318,-1.71178047974623,13.7684646803415));
#16937=CARTESIAN_POINT('Ctrl Pts',(1.90307295579245,-1.64806540371777,13.7738260431222));
#16938=CARTESIAN_POINT('Ctrl Pts',(1.9567066129225,-1.58613293297104,13.7790374069668));
#16939=CARTESIAN_POINT('Ctrl Pts',(2.00742189654929,-1.52145466982198,13.7842487708115));
#16940=CARTESIAN_POINT('Ctrl Pts',(2.0549218431537,-1.45433918620445,13.7894601346562));
#16941=CARTESIAN_POINT('Ctrl Pts',(2.10235895333399,-1.38731248788658,13.7946646045254));
#16942=CARTESIAN_POINT('Ctrl Pts',(2.14658889768453,-1.31785534577773,13.7998690743945));
#16943=CARTESIAN_POINT('Ctrl Pts',(2.18735350234999,-1.24631091857418,13.8050735442637));
#16944=CARTESIAN_POINT('Ctrl Pts',(2.22807698574385,-1.1748386617706,13.8102727641269));
#16945=CARTESIAN_POINT('Ctrl Pts',(2.26534183691485,-1.10128370481958,13.81547198399));
#16946=CARTESIAN_POINT('Ctrl Pts',(2.29893280601861,-1.02601861747796,13.8206712038532));
#16947=CARTESIAN_POINT('Ctrl Pts',(2.33250043822423,-0.950805819597609,
13.8258668116245));
#16948=CARTESIAN_POINT('Ctrl Pts',(2.36239906650766,-0.873885678457068,
13.8310624193959));
#16949=CARTESIAN_POINT('Ctrl Pts',(2.3884597893834,-0.795654500709079,13.8362580271672));
#16950=CARTESIAN_POINT('Ctrl Pts',(2.41451585326659,-0.717437308700311,
13.8414527060964));
#16951=CARTESIAN_POINT('Ctrl Pts',(2.43673521726414,-0.637909987838495,
13.8466473850256));
#16952=CARTESIAN_POINT('Ctrl Pts',(2.45499791486807,-0.557486760375013,
13.8518420639548));
#16953=CARTESIAN_POINT('Ctrl Pts',(2.47325894911898,-0.477070857799738,
13.8570362697565));
#16954=CARTESIAN_POINT('Ctrl Pts',(2.48756393628175,-0.395759670386109,
13.8622304755582));
#16955=CARTESIAN_POINT('Ctrl Pts',(2.49784379623378,-0.313978692933837,
13.8674246813599));
#16956=CARTESIAN_POINT('Ctrl Pts',(2.5081291916546,-0.232153678300999,13.8726216841222));
#16957=CARTESIAN_POINT('Ctrl Pts',(2.51438508505178,-0.149858835924081,
13.8778186868846));
#16958=CARTESIAN_POINT('Ctrl Pts',(2.51659425685167,-0.0675247834590446,
13.8830156896469));
#16959=CARTESIAN_POINT('Ctrl Pts',(2.51721785875597,-0.0442836430876919,
13.8844826922673));
#16960=CARTESIAN_POINT('Ctrl Pts',(2.51751933182793,-0.0210393816020136,
13.8859496948877));
#16961=CARTESIAN_POINT('Ctrl Pts',(2.51749904018654,0.00219833114617901,
13.887416697508));
#16962=CARTESIAN_POINT('Ctrl Pts',(2.51749904018606,0.0021983317047849,
13.8874166975433));
#16963=CARTESIAN_POINT('Ctrl Pts',(2.51741017424796,0.10396637397242,13.8938413395162));
#16964=CARTESIAN_POINT('Ctrl Pts',(2.51114671053784,0.205464160528413,13.9002659814891));
#16965=CARTESIAN_POINT('Ctrl Pts',(2.49882897256025,0.306039239140149,13.906690623462));
#16966=CARTESIAN_POINT('Ctrl Pts',(2.48631365676307,0.408227552647264,13.9132183173714));
#16967=CARTESIAN_POINT('Ctrl Pts',(2.46754833856782,0.509463401298269,13.9197460112809));
#16968=CARTESIAN_POINT('Ctrl Pts',(2.44270786672858,0.609084992281317,13.9262737051904));
#16969=CARTESIAN_POINT('Ctrl Pts',(2.43519696831622,0.639207111313228,13.9282474537624));
#16970=CARTESIAN_POINT('Ctrl Pts',(2.42713098016237,0.669181796373038,13.9302212023344));
#16971=CARTESIAN_POINT('Ctrl Pts',(2.41851558766797,0.698991131708456,13.9321949509065));
#16972=CARTESIAN_POINT('Ctrl Pts',(2.40161632718108,0.757462724627967,13.9360664972435));
#16973=CARTESIAN_POINT('Ctrl Pts',(2.38257241873794,0.815400560410186,13.9399380435806));
#16974=CARTESIAN_POINT('Ctrl Pts',(2.36142200728636,0.872635292378013,13.9438095899177));
#16975=CARTESIAN_POINT('Ctrl Pts',(2.36142191786124,0.872635534369624,13.6679749024944));
#16976=CARTESIAN_POINT('Ctrl Pts',(2.37809075863486,0.827528311023971,13.6651807393162));
#16977=CARTESIAN_POINT('Ctrl Pts',(2.39347242642984,0.781929253098341,13.6624065957962));
#16978=CARTESIAN_POINT('Ctrl Pts',(2.44479148206397,0.614034034977576,13.6523079455054));
#16979=CARTESIAN_POINT('Ctrl Pts',(2.4727309941405,0.489530988008946,13.6450467174458));
#16980=CARTESIAN_POINT('Ctrl Pts',(2.49706478605095,0.322747949202046,13.6350543391746));
#16981=CARTESIAN_POINT('Ctrl Pts',(2.50200522284528,0.281901199609186,13.6325856636504));
#16982=CARTESIAN_POINT('Ctrl Pts',(2.50849472206676,0.214409857885104,13.6284449640569));
#16983=CARTESIAN_POINT('Ctrl Pts',(2.51062499424916,0.187828018936672,13.6267984228798));
#16984=CARTESIAN_POINT('Ctrl Pts',(2.51296551022381,0.15135484437533,13.6245115902134));
#16985=CARTESIAN_POINT('Ctrl Pts',(2.51354036909397,0.141487631169278,13.6238901612926));
#16986=CARTESIAN_POINT('Ctrl Pts',(2.51441006086061,0.124875440192849,13.6228389055961));
#16987=CARTESIAN_POINT('Ctrl Pts',(2.51473589921992,0.118132067608455,13.6224107745233));
#16988=CARTESIAN_POINT('Ctrl Pts',(2.51530656429679,0.105246939291447,13.6215899081342));
#16989=CARTESIAN_POINT('Ctrl Pts',(2.51555602898852,0.0991054675449234,
13.6211974485973));
#16990=CARTESIAN_POINT('Ctrl Pts',(2.51609896969873,0.0844123345254984,
13.6202557206377));
#16991=CARTESIAN_POINT('Ctrl Pts',(2.51637133932898,0.075860036347716,13.6197053174528));
#16992=CARTESIAN_POINT('Ctrl Pts',(2.51719523687576,0.0450544589039541,
13.6177150116822));
#16993=CARTESIAN_POINT('Ctrl Pts',(2.51749518710519,0.022796223009124,13.6162623979861));
#16994=CARTESIAN_POINT('Ctrl Pts',(2.51750703494928,-0.0326589414498927,
13.6126118173863));
#16995=CARTESIAN_POINT('Ctrl Pts',(2.51685750509814,-0.0658510767202741,
13.6103987212928));
#16996=CARTESIAN_POINT('Ctrl Pts',(2.51140428215516,-0.204388794806129,
13.6010693947918));
#16997=CARTESIAN_POINT('Ctrl Pts',(2.5006404684397,-0.309388435010393,13.5937801096634));
#16998=CARTESIAN_POINT('Ctrl Pts',(2.45291424950533,-0.596085184335655,
13.573701268477));
#16999=CARTESIAN_POINT('Ctrl Pts',(2.40243068465968,-0.774890960910285,
13.5610264877404));
#17000=CARTESIAN_POINT('Ctrl Pts',(2.3205371506762,-0.976715181915555,13.5468788962842));
#17001=CARTESIAN_POINT('Ctrl Pts',(2.30771774987936,-1.00663010236431,13.5447843218245));
#17002=CARTESIAN_POINT('Ctrl Pts',(2.28813308902568,-1.0499901076307,13.5417505937046));
#17003=CARTESIAN_POINT('Ctrl Pts',(2.281822035993,-1.06363549736384,13.540796199055));
#17004=CARTESIAN_POINT('Ctrl Pts',(2.2703796854448,-1.08780484751768,13.5391060459477));
#17005=CARTESIAN_POINT('Ctrl Pts',(2.26529654221601,-1.09835098473381,13.5383686659501));
#17006=CARTESIAN_POINT('Ctrl Pts',(2.25451186580801,-1.12033288202263,13.5368317574778));
#17007=CARTESIAN_POINT('Ctrl Pts',(2.24879644807643,-1.13176148737903,13.5360327343738));
#17008=CARTESIAN_POINT('Ctrl Pts',(2.23358303614245,-1.16161208116453,13.5339455076524));
#17009=CARTESIAN_POINT('Ctrl Pts',(2.22394400716131,-1.17996139732444,13.5326622399996));
#17010=CARTESIAN_POINT('Ctrl Pts',(2.17792925906639,-1.26498989626293,13.526711697645));
#17011=CARTESIAN_POINT('Ctrl Pts',(2.13877259475649,-1.33012357331012,13.5221433803506));
#17012=CARTESIAN_POINT('Ctrl Pts',(2.02319963452841,-1.50403371917174,13.5097954818854));
#17013=CARTESIAN_POINT('Ctrl Pts',(1.94102663771021,-1.60868646600432,13.5022017477818));
#17014=CARTESIAN_POINT('Ctrl Pts',(1.75867271623855,-1.80649446145371,13.4867305559519));
#17015=CARTESIAN_POINT('Ctrl Pts',(1.65840654927995,-1.89895508917419,13.4788721412775));
#17016=CARTESIAN_POINT('Ctrl Pts',(1.5343066374832,-1.99603806000914,13.4691961797086));
#17017=CARTESIAN_POINT('Ctrl Pts',(1.51727370654132,-2.00901598406386,13.4678689624149));
#17018=CARTESIAN_POINT('Ctrl Pts',(1.49331298652176,-2.02679390492557,13.4659998451705));
#17019=CARTESIAN_POINT('Ctrl Pts',(1.48652297403821,-2.03177918378469,13.4654699436876));
#17020=CARTESIAN_POINT('Ctrl Pts',(1.47476311389155,-2.04032285895249,13.4645515513967));
#17021=CARTESIAN_POINT('Ctrl Pts',(1.46980503926398,-2.04389744251115,13.4641641542436));
#17022=CARTESIAN_POINT('Ctrl Pts',(1.45931393713159,-2.05140321531996,13.4633439146791));
#17023=CARTESIAN_POINT('Ctrl Pts',(1.45377796974234,-2.05533012682068,13.4629107792005));
#17024=CARTESIAN_POINT('Ctrl Pts',(1.43999604444607,-2.06502273163781,13.4618318470369));
#17025=CARTESIAN_POINT('Ctrl Pts',(1.43173133570106,-2.07076142141599,13.4611842796785));
#17026=CARTESIAN_POINT('Ctrl Pts',(1.40039401278373,-2.09224354771822,13.4587274821286));
#17027=CARTESIAN_POINT('Ctrl Pts',(1.37709527025043,-2.10765151708069,13.4568980347743));
#17028=CARTESIAN_POINT('Ctrl Pts',(1.31656470663896,-2.14624960109195,13.4521474046048));
#17029=CARTESIAN_POINT('Ctrl Pts',(1.27897528420057,-2.16885955426309,13.4491995381363));
#17030=CARTESIAN_POINT('Ctrl Pts',(1.13297376822004,-2.25156359832945,13.437809516732));
#17031=CARTESIAN_POINT('Ctrl Pts',(1.02076945468084,-2.30460339731891,13.4291886210193));
#17032=CARTESIAN_POINT('Ctrl Pts',(0.754220629113447,-2.40730299872092,
13.4095210718018));
#17033=CARTESIAN_POINT('Ctrl Pts',(0.598050074362739,-2.45077733867244,
13.39859835904));
#17034=CARTESIAN_POINT('Ctrl Pts',(0.416868001374833,-2.48284549033157,
13.3867311280604));
#17035=CARTESIAN_POINT('Ctrl Pts',(0.394922057865349,-2.48643063032723,
13.3853060979199));
#17036=CARTESIAN_POINT('Ctrl Pts',(0.358701370722863,-2.49185605508689,
13.3829739776756));
#17037=CARTESIAN_POINT('Ctrl Pts',(0.344453589169661,-2.4938654758297,13.3820616389215));
#17038=CARTESIAN_POINT('Ctrl Pts',(0.318679815629225,-2.49727535681125,
13.3804200816875));
#17039=CARTESIAN_POINT('Ctrl Pts',(0.307159965330567,-2.49871843063716,
13.3796895495698));
#17040=CARTESIAN_POINT('Ctrl Pts',(0.282418267232902,-2.50164409404214,
13.3781271930396));
#17041=CARTESIAN_POINT('Ctrl Pts',(0.26919377422902,-2.50310167065371,13.3772961701701));
#17042=CARTESIAN_POINT('Ctrl Pts',(0.232932535203316,-2.50680761137186,
13.3750282497524));
#17043=CARTESIAN_POINT('Ctrl Pts',(0.209875004720985,-2.50884326008693,
13.3735979883149));
#17044=CARTESIAN_POINT('Ctrl Pts',(0.073590212145572,-2.5189831937923,13.3652087853792));
#17045=CARTESIAN_POINT('Ctrl Pts',(-0.0400591223554762,-2.51974040778754,
13.3584838351933));
#17046=CARTESIAN_POINT('Ctrl Pts',(-0.331509641175326,-2.50195020746078,
13.3414980921401));
#17047=CARTESIAN_POINT('Ctrl Pts',(-0.507960568904698,-2.47216938436677,
13.3314831810998));
#17048=CARTESIAN_POINT('Ctrl Pts',(-0.738757301150904,-2.40744621896714,
13.3172800196309));
#17049=CARTESIAN_POINT('Ctrl Pts',(-0.797118086428009,-2.38875722866903,
13.3135851423482));
#17050=CARTESIAN_POINT('Ctrl Pts',(-0.867441885713224,-2.36337330082162,
13.3089403323355));
#17051=CARTESIAN_POINT('Ctrl Pts',(-0.8801124209655,-2.35868414413761,13.3080956764112));
#17052=CARTESIAN_POINT('Ctrl Pts',(-0.899871150864326,-2.35119039217152,
13.3067653854445));
#17053=CARTESIAN_POINT('Ctrl Pts',(-0.906985605970703,-2.34845512099487,
13.3062837152547));
#17054=CARTESIAN_POINT('Ctrl Pts',(-0.920169394286457,-2.34331755071924,
13.3053859608971));
#17055=CARTESIAN_POINT('Ctrl Pts',(-0.926241912820787,-2.34092391445327,
13.3049703869733));
#17056=CARTESIAN_POINT('Ctrl Pts',(-0.94016464059317,-2.33537326576604,
13.304012869329));
#17057=CARTESIAN_POINT('Ctrl Pts',(-0.948008269066632,-2.33220028272001,
13.3034699960396));
#17058=CARTESIAN_POINT('Ctrl Pts',(-0.972520217951942,-2.32214037900105,
13.3017630231271));
#17059=CARTESIAN_POINT('Ctrl Pts',(-0.989130198283595,-2.31511401900966,
13.3005911365514));
#17060=CARTESIAN_POINT('Ctrl Pts',(-1.14349679679879,-2.24784938389074,
13.2895671095692));
#17061=CARTESIAN_POINT('Ctrl Pts',(-1.27566014501487,-2.17556760450728,
13.2791528662349));
#17062=CARTESIAN_POINT('Ctrl Pts',(-1.55018979264058,-1.99176740576532,
13.2563319237504));
#17063=CARTESIAN_POINT('Ctrl Pts',(-1.68865442809921,-1.87581810887262,
13.2440271834098));
#17064=CARTESIAN_POINT('Ctrl Pts',(-1.83405660407491,-1.72479406241571,
13.2304071297146));
#17065=CARTESIAN_POINT('Ctrl Pts',(-1.85416158491882,-1.70316268234601,
13.2285044724803));
#17066=CARTESIAN_POINT('Ctrl Pts',(-1.88379652698458,-1.67013092713428,
13.2256692769152));
#17067=CARTESIAN_POINT('Ctrl Pts',(-1.8936132171945,-1.65899236524033,13.2247248418291));
#17068=CARTESIAN_POINT('Ctrl Pts',(-1.9104795445215,-1.63951012345845,13.2230927242107));
#17069=CARTESIAN_POINT('Ctrl Pts',(-1.91757439551896,-1.63120629556808,
13.2224031915989));
#17070=CARTESIAN_POINT('Ctrl Pts',(-1.93226378791115,-1.61378551506635,
13.2209691671538));
#17071=CARTESIAN_POINT('Ctrl Pts',(-1.93984837950974,-1.60466049585197,
13.2202250902542));
#17072=CARTESIAN_POINT('Ctrl Pts',(-1.95769337763586,-1.58287975384526,
13.2184654824269));
#17073=CARTESIAN_POINT('Ctrl Pts',(-1.96789608338595,-1.57017728315698,
13.2174522767995));
#17074=CARTESIAN_POINT('Ctrl Pts',(-2.00199461725012,-1.52686980477434,
13.2140405393533));
#17075=CARTESIAN_POINT('Ctrl Pts',(-2.02530621890243,-1.49581042094412,
13.2116648649744));
#17076=CARTESIAN_POINT('Ctrl Pts',(-2.12043525272134,-1.36276107700484,
13.2017621306102));
#17077=CARTESIAN_POINT('Ctrl Pts',(-2.1853427602699,-1.25604343837688,13.1944898670829));
#17078=CARTESIAN_POINT('Ctrl Pts',(-2.30840032196292,-1.01506700837394,
13.1788906795224));
#17079=CARTESIAN_POINT('Ctrl Pts',(-2.3633084477247,-0.879682099700715,
13.1706242151947));
#17080=CARTESIAN_POINT('Ctrl Pts',(-2.42334987876075,-0.684534769749036,
13.158502365031));
#17081=CARTESIAN_POINT('Ctrl Pts',(-2.43856617758191,-0.628176995431338,
13.1549765580319));
#17082=CARTESIAN_POINT('Ctrl Pts',(-2.45483434578437,-0.558365683251226,
13.1505219224476));
#17083=CARTESIAN_POINT('Ctrl Pts',(-2.45775605746228,-0.545361389739,13.1496884456733));
#17084=CARTESIAN_POINT('Ctrl Pts',(-2.46217731268002,-0.524925329418601,
13.1483720151933));
#17085=CARTESIAN_POINT('Ctrl Pts',(-2.46374682795991,-0.517508729087825,
13.147892894012));
#17086=CARTESIAN_POINT('Ctrl Pts',(-2.46659394342787,-0.503748392895903,
13.1470012404913));
#17087=CARTESIAN_POINT('Ctrl Pts',(-2.46788060677716,-0.497406707271335,
13.1465892221593));
#17088=CARTESIAN_POINT('Ctrl Pts',(-2.4707982469329,-0.482736264189013,
13.1456336173918));
#17089=CARTESIAN_POINT('Ctrl Pts',(-2.4724115631273,-0.474404189844925,
13.1450890621632));
#17090=CARTESIAN_POINT('Ctrl Pts',(-2.47734674171339,-0.448207059155325,
13.1433715385622));
#17091=CARTESIAN_POINT('Ctrl Pts',(-2.48051724127615,-0.430314556324609,
13.14219064942));
#17092=CARTESIAN_POINT('Ctrl Pts',(-2.50457703400831,-0.285421726013943,
13.1325731134126));
#17093=CARTESIAN_POINT('Ctrl Pts',(-2.51589036887427,-0.157036459991599,
13.1237217332443));
#17094=CARTESIAN_POINT('Ctrl Pts',(-2.51964136449002,0.175861940829714,
13.1007301925616));
#17095=CARTESIAN_POINT('Ctrl Pts',(-2.49708142069865,0.379651511722815,
13.0866816259376));
#17096=CARTESIAN_POINT('Ctrl Pts',(-2.4430074841959,0.608672204471248,13.0714164705259));
#17097=CARTESIAN_POINT('Ctrl Pts',(-2.43532632500538,0.638712181759205,
13.0694227651158));
#17098=CARTESIAN_POINT('Ctrl Pts',(-2.42313267639444,0.682976227054846,
13.0664965888944));
#17099=CARTESIAN_POINT('Ctrl Pts',(-2.41904575887019,0.697313506395124,
13.0655505943799));
#17100=CARTESIAN_POINT('Ctrl Pts',(-2.41153608953457,0.722797251760484,
13.0638721110112));
#17101=CARTESIAN_POINT('Ctrl Pts',(-2.40816283368252,0.73395773184295,13.0631380491776));
#17102=CARTESIAN_POINT('Ctrl Pts',(-2.40087234078289,0.757487010302141,
13.0615924408573));
#17103=CARTESIAN_POINT('Ctrl Pts',(-2.39693676518691,0.769849804332523,
13.0607815139856));
#17104=CARTESIAN_POINT('Ctrl Pts',(-2.38618713300383,0.802735836984656,
13.0586271611727));
#17105=CARTESIAN_POINT('Ctrl Pts',(-2.379203827701,0.823202920868137,13.0572892784912));
#17106=CARTESIAN_POINT('Ctrl Pts',(-2.3426622807203,0.925949789014163,13.0505840796357));
#17107=CARTESIAN_POINT('Ctrl Pts',(-2.30909433649126,1.00674490445486,13.0453504820223));
#17108=CARTESIAN_POINT('Ctrl Pts',(-2.18030220991975,1.27620599524215,13.0277903924667));
#17109=CARTESIAN_POINT('Ctrl Pts',(-2.06560711448605,1.45453570666296,13.0160466257753));
#17110=CARTESIAN_POINT('Ctrl Pts',(-1.89283715056426,1.66082056219731,13.0000662862577));
#17111=CARTESIAN_POINT('Ctrl Pts',(-1.8541508456278,1.70390168118828,12.9965681245321));
#17112=CARTESIAN_POINT('Ctrl Pts',(-1.80479716574065,1.75518952634118,12.9921445981148));
#17113=CARTESIAN_POINT('Ctrl Pts',(-1.79550103642579,1.76469801753502,12.9913130109086));
#17114=CARTESIAN_POINT('Ctrl Pts',(-1.7807927482699,1.77950577471563,12.9899989238631));
#17115=CARTESIAN_POINT('Ctrl Pts',(-1.77543110430399,1.78485517755347,12.9895202343738));
#17116=CARTESIAN_POINT('Ctrl Pts',(-1.76544316922027,1.79473077510757,12.9886289408832));
#17117=CARTESIAN_POINT('Ctrl Pts',(-1.76082348175553,1.79926340528292,12.9882168469099));
#17118=CARTESIAN_POINT('Ctrl Pts',(-1.75009798246767,1.80970591781176,12.9872604813368));
#17119=CARTESIAN_POINT('Ctrl Pts',(-1.74397970371148,1.81560272230545,12.9867152354569));
#17120=CARTESIAN_POINT('Ctrl Pts',(-1.72464383691172,1.83405074220905,12.9849933677446));
#17121=CARTESIAN_POINT('Ctrl Pts',(-1.7113200607685,1.84648912628948,12.9838087697132));
#17122=CARTESIAN_POINT('Ctrl Pts',(-1.59734150909223,1.95060032499522,12.9736998379727));
#17123=CARTESIAN_POINT('Ctrl Pts',(-1.48954756252013,2.0341047334634,12.9643130130075));
#17124=CARTESIAN_POINT('Ctrl Pts',(-1.21190425064778,2.21523592114061,12.9414120899283));
#17125=CARTESIAN_POINT('Ctrl Pts',(-1.03635926706881,2.30260042617566,12.9280032078562));
#17126=CARTESIAN_POINT('Ctrl Pts',(-0.822852325842711,2.37943475252667,
12.9132726593402));
#17127=CARTESIAN_POINT('Ctrl Pts',(-0.793057044007318,2.38953057374007,
12.9112485828575));
#17128=CARTESIAN_POINT('Ctrl Pts',(-0.748736707895591,2.40362769830424,
12.9082829694164));
#17129=CARTESIAN_POINT('Ctrl Pts',(-0.734353310004099,2.40806104613763,
12.9073274753791));
#17130=CARTESIAN_POINT('Ctrl Pts',(-0.708710408996641,2.41571374858801,
12.905636066239));
#17131=CARTESIAN_POINT('Ctrl Pts',(-0.697466682370646,2.41898400023712,
12.904898521237));
#17132=CARTESIAN_POINT('Ctrl Pts',(-0.673914463720985,2.42565632441566,
12.9033619539428));
#17133=CARTESIAN_POINT('Ctrl Pts',(-0.661602054593062,2.42904344125737,
12.9025634320681));
#17134=CARTESIAN_POINT('Ctrl Pts',(-0.629276203854807,2.43767218812735,
12.9004790352874));
#17135=CARTESIAN_POINT('Ctrl Pts',(-0.609222733539032,2.44276112994044,
12.8991980713526));
#17136=CARTESIAN_POINT('Ctrl Pts',(-0.515691001673122,2.46527308802374,
12.8932767042149));
#17137=CARTESIAN_POINT('Ctrl Pts',(-0.441511413653369,2.47963261209531,
12.888734033511));
#17138=CARTESIAN_POINT('Ctrl Pts',(-0.236721407293363,2.50979176322334,
12.8764904193053));
#17139=CARTESIAN_POINT('Ctrl Pts',(-0.105344108653229,2.51872918987127,
12.8689709390602));
#17140=CARTESIAN_POINT('Ctrl Pts',(0.164194273390748,2.51593117970867,12.8534726753599));
#17141=CARTESIAN_POINT('Ctrl Pts',(0.30188784765683,2.50314274929702,12.8455123787338));
#17142=CARTESIAN_POINT('Ctrl Pts',(0.458906817720091,2.47541296209981,12.8357205747889));
#17143=CARTESIAN_POINT('Ctrl Pts',(0.479945114370115,2.47142012159577,12.8343933497603));
#17144=CARTESIAN_POINT('Ctrl Pts',(0.509184385006529,2.46548341531214,12.8325242233235));
#17145=CARTESIAN_POINT('Ctrl Pts',(0.517431062808267,2.46376587759491,12.8319943205369));
#17146=CARTESIAN_POINT('Ctrl Pts',(0.531646451170755,2.46073071705992,12.8310759266064));
#17147=CARTESIAN_POINT('Ctrl Pts',(0.537619331044593,2.45943267114636,12.8306885291266));
#17148=CARTESIAN_POINT('Ctrl Pts',(0.550214638937756,2.45664734342314,12.8298682896324));
#17149=CARTESIAN_POINT('Ctrl Pts',(0.556835850641238,2.45515501565242,12.8294351545554));
#17150=CARTESIAN_POINT('Ctrl Pts',(0.573257368282003,2.45138399262925,12.828356224705));
#17151=CARTESIAN_POINT('Ctrl Pts',(0.583050124901039,2.44907330092699,12.8277086592742));
#17152=CARTESIAN_POINT('Ctrl Pts',(0.619974997666589,2.44012652219851,12.8252518775997));
#17153=CARTESIAN_POINT('Ctrl Pts',(0.647008773314897,2.43309801202393,12.8234224445204));
#17154=CARTESIAN_POINT('Ctrl Pts',(0.716177789675453,2.41388055000207,12.8186718602732));
#17155=CARTESIAN_POINT('Ctrl Pts',(0.758120588908801,2.4010378330102,12.8157240260535));
#17156=CARTESIAN_POINT('Ctrl Pts',(0.97681254444608,2.32777390142417,12.800068551787));
#17157=CARTESIAN_POINT('Ctrl Pts',(1.14677140277557,2.24891467940778,12.7869642211667));
#17158=CARTESIAN_POINT('Ctrl Pts',(1.393096444391,2.09937196476488,12.7674641387089));
#17159=CARTESIAN_POINT('Ctrl Pts',(1.47649307708827,2.04158102325674,12.7607469599041));
#17160=CARTESIAN_POINT('Ctrl Pts',(1.57429774356821,1.96466885436951,12.7527331957181));
#17161=CARTESIAN_POINT('Ctrl Pts',(1.59221273355169,1.95017839222046,12.7512590233193));
#17162=CARTESIAN_POINT('Ctrl Pts',(1.6202402878396,1.92686471400428,12.7489420238722));
#17163=CARTESIAN_POINT('Ctrl Pts',(1.63048522565309,1.91820336686881,12.7480927683579));
#17164=CARTESIAN_POINT('Ctrl Pts',(1.64944540036644,1.90191226617537,12.7465165044326));
#17165=CARTESIAN_POINT('Ctrl Pts',(1.65817811779051,1.89430349572399,12.7457886695384));
#17166=CARTESIAN_POINT('Ctrl Pts',(1.66706094061283,1.88645544435058,12.7450463484127));
#17167=CARTESIAN_POINT('Ctrl Pts',(1.66726371892795,1.88627622971385,12.7450294015419));
#17168=CARTESIAN_POINT('Ctrl Pts',(1.66764802512575,1.88593647109887,12.7449972817578));
#17169=CARTESIAN_POINT('Ctrl Pts',(1.66782955872015,1.88577593361091,12.7449821085776));
#17170=CARTESIAN_POINT('Ctrl Pts',(1.66817419178611,1.8854710719843,12.7449533013832));
#17171=CARTESIAN_POINT('Ctrl Pts',(1.668337295705,1.8853267528974,12.7449396671613));
#17172=CARTESIAN_POINT('Ctrl Pts',(1.66864741612383,1.88505227758218,12.7449137421899));
#17173=CARTESIAN_POINT('Ctrl Pts',(1.66879443612225,1.88492212532028,12.7449014512769));
#17174=CARTESIAN_POINT('Ctrl Pts',(1.66907436040821,1.88467425857843,12.74487804846));
#17175=CARTESIAN_POINT('Ctrl Pts',(1.66920726746409,1.88455654724535,12.744866936427));
#17176=CARTESIAN_POINT('Ctrl Pts',(1.66946063508355,1.88433210019086,12.7448457521065));
#17177=CARTESIAN_POINT('Ctrl Pts',(1.66958109786296,1.88422536697763,12.7448356797155));
#17178=CARTESIAN_POINT('Ctrl Pts',(1.66981099989146,1.88402162833352,12.7448164559359));
#17179=CARTESIAN_POINT('Ctrl Pts',(1.66992044092075,1.88392462492056,12.7448073044642));
#17180=CARTESIAN_POINT('Ctrl Pts',(1.67012952021494,1.88373927427328,12.7447898206331));
#17181=CARTESIAN_POINT('Ctrl Pts',(1.6702291599208,1.88365092867105,12.7447814882064));
#17182=CARTESIAN_POINT('Ctrl Pts',(1.67041969000504,1.88348196805897,12.7447655545256));
#17183=CARTESIAN_POINT('Ctrl Pts',(1.67051058155444,1.88340135437842,12.7447579532169));
#17184=CARTESIAN_POINT('Ctrl Pts',(1.67080491686272,1.88314026396033,12.7447333370999));
#17185=CARTESIAN_POINT('Ctrl Pts',(1.67100833726458,1.88295976078979,12.7447163233804));
#17186=CARTESIAN_POINT('Ctrl Pts',(1.68217384108825,1.87304892222698,12.7437824011769));
#17187=CARTESIAN_POINT('Ctrl Pts',(1.69305094316491,1.86322291067464,12.7428694618121));
#17188=CARTESIAN_POINT('Ctrl Pts',(1.72658826258211,1.83239022539699,12.7400441404101));
#17189=CARTESIAN_POINT('Ctrl Pts',(1.74894852584554,1.8110605037083,12.7381453846975));
#17190=CARTESIAN_POINT('Ctrl Pts',(1.80014866667017,1.7603872249161,12.7337565821545));
#17191=CARTESIAN_POINT('Ctrl Pts',(1.82867354011596,1.73073734368324,12.7312797525815));
#17192=CARTESIAN_POINT('Ctrl Pts',(1.92844346603761,1.6218107169829,12.7224745300691));
#17193=CARTESIAN_POINT('Ctrl Pts',(1.99536737966006,1.53872533332381,12.716300611589));
#17194=CARTESIAN_POINT('Ctrl Pts',(2.15310798789481,1.31522352293741,12.7005573373296));
#17195=CARTESIAN_POINT('Ctrl Pts',(2.23556694365276,1.16957872182038,12.6910969366956));
#17196=CARTESIAN_POINT('Ctrl Pts',(2.3153968018407,0.988780316548436,12.6790862762629));
#17197=CARTESIAN_POINT('Ctrl Pts',(2.3272824812662,0.96047119808167,12.6771976976479));
#17198=CARTESIAN_POINT('Ctrl Pts',(2.34263775694275,0.921938615522299,12.6746072249691));
#17199=CARTESIAN_POINT('Ctrl Pts',(2.34656416844794,0.911898604329127,12.6739304541055));
#17200=CARTESIAN_POINT('Ctrl Pts',(2.3526653155969,0.895997345504483,12.6728552887704));
#17201=CARTESIAN_POINT('Ctrl Pts',(2.35488296304312,0.890152547994118,12.6724593907968));
#17202=CARTESIAN_POINT('Ctrl Pts',(2.35853616202579,0.880415036445676,12.6717985584326));
#17203=CARTESIAN_POINT('Ctrl Pts',(2.35998390411294,0.876526916418576,12.6715343551603));
#17204=CARTESIAN_POINT('Ctrl Pts',(2.36142200728627,0.872635292378268,12.6712695847815));
#17205=CARTESIAN_POINT('Origin',(0.,0.,10.));
#17206=CARTESIAN_POINT('',(2.36142193605295,0.872635485141376,11.6676249231292));
#17207=CARTESIAN_POINT('',(2.36142200728635,0.872635292378037,11.9438279118171));
#17208=CARTESIAN_POINT('',(2.36142200728636,0.87263529237802,10.));
#17209=CARTESIAN_POINT('',(2.51749968849485,-0.00125236909203477,12.8874166974535));
#17210=CARTESIAN_POINT('Ctrl Pts',(2.36142200728635,0.872635292378036,11.9438279118171));
#17211=CARTESIAN_POINT('Ctrl Pts',(2.33294410961694,0.949698797447294,11.9490047738285));
#17212=CARTESIAN_POINT('Ctrl Pts',(2.30067936897463,1.02539487449982,11.95418163584));
#17213=CARTESIAN_POINT('Ctrl Pts',(2.26479238961036,1.09932783188773,11.9593584978515));
#17214=CARTESIAN_POINT('Ctrl Pts',(2.22890486521791,1.17326191212148,11.9645354384858));
#17215=CARTESIAN_POINT('Ctrl Pts',(2.18939520142238,1.24543239473698,11.9697123791201));
#17216=CARTESIAN_POINT('Ctrl Pts',(2.14647477656318,1.31546656497915,11.9748893197544));
#17217=CARTESIAN_POINT('Ctrl Pts',(2.10351230570705,1.38556934256892,11.9800713318583));
#17218=CARTESIAN_POINT('Ctrl Pts',(2.05713265121341,1.45353122561535,11.9852533439622));
#17219=CARTESIAN_POINT('Ctrl Pts',(2.00759113030992,1.51900760481998,11.9904353560661));
#17220=CARTESIAN_POINT('Ctrl Pts',(1.95802381995394,1.58451806856501,11.9956200657306));
#17221=CARTESIAN_POINT('Ctrl Pts',(1.90529167198153,1.64754009118975,12.0008047753951));
#17222=CARTESIAN_POINT('Ctrl Pts',(1.84968934232933,1.70776332870608,12.0059894850596));
#17223=CARTESIAN_POINT('Ctrl Pts',(1.79399353595335,1.76808781145754,12.0111829110797));
#17224=CARTESIAN_POINT('Ctrl Pts',(1.73541825291344,1.82560378477774,12.0163763370997));
#17225=CARTESIAN_POINT('Ctrl Pts',(1.67429355538389,1.8800391858682,12.0215697631197));
#17226=CARTESIAN_POINT('Ctrl Pts',(1.63428350827941,1.91567065808494,12.0249691945786));
#17227=CARTESIAN_POINT('Ctrl Pts',(1.59318183758348,1.94998307448256,12.0283686260374));
#17228=CARTESIAN_POINT('Ctrl Pts',(1.55108776789127,1.98291023152791,12.0317680574963));
#17229=CARTESIAN_POINT('Ctrl Pts',(1.4860136996306,2.03381298530929,12.0370233069036));
#17230=CARTESIAN_POINT('Ctrl Pts',(1.41831105347754,2.08160300135593,12.0422785563109));
#17231=CARTESIAN_POINT('Ctrl Pts',(1.34830995266707,2.12599777082172,12.0475338057182));
#17232=CARTESIAN_POINT('Ctrl Pts',(1.27840809751517,2.17032959858971,12.0527816043757));
#17233=CARTESIAN_POINT('Ctrl Pts',(1.20621464682175,2.21127549610313,12.0580294030332));
#17234=CARTESIAN_POINT('Ctrl Pts',(1.13209187433444,2.24859383572621,12.0632772016907));
#17235=CARTESIAN_POINT('Ctrl Pts',(1.05743201845915,2.28618257889205,12.0685630251736));
#17236=CARTESIAN_POINT('Ctrl Pts',(0.980815136875723,2.32009068081077,12.0738488486565));
#17237=CARTESIAN_POINT('Ctrl Pts',(0.902640269298452,2.35011633632057,12.0791346721394));
#17238=CARTESIAN_POINT('Ctrl Pts',(0.825166390362672,2.37987275384996,12.084373098008));
#17239=CARTESIAN_POINT('Ctrl Pts',(0.746162792910291,2.4058159048703,12.0896115238766));
#17240=CARTESIAN_POINT('Ctrl Pts',(0.66603992468444,2.42779675193916,12.0948499497452));
#17241=CARTESIAN_POINT('Ctrl Pts',(0.585943407536478,2.44977036987324,12.1000866527827));
#17242=CARTESIAN_POINT('Ctrl Pts',(0.504728795329191,2.46778414997608,12.1053233558202));
#17243=CARTESIAN_POINT('Ctrl Pts',(0.422821641415746,2.4817389285641,12.1105600588577));
#17244=CARTESIAN_POINT('Ctrl Pts',(0.34091671861231,2.49569332703091,12.1157966192501));
#17245=CARTESIAN_POINT('Ctrl Pts',(0.258319746649563,2.50558886733434,12.1210331796424));
#17246=CARTESIAN_POINT('Ctrl Pts',(0.175465040666664,2.51137776320167,12.1262697400347));
#17247=CARTESIAN_POINT('Ctrl Pts',(0.0912542264867864,2.51726140769003,
12.1315920088052));
#17248=CARTESIAN_POINT('Ctrl Pts',(0.00677765496035548,2.51890271813326,
12.1369142775757));
#17249=CARTESIAN_POINT('Ctrl Pts',(-0.0775066867448587,2.51630661158569,
12.1422365463461));
#17250=CARTESIAN_POINT('Ctrl Pts',(-0.160552829837487,2.5137486437417,12.1474806270965));
#17251=CARTESIAN_POINT('Ctrl Pts',(-0.243411892025351,2.50707703272407,
12.1527247078468));
#17252=CARTESIAN_POINT('Ctrl Pts',(-0.32565089727474,2.49634888248902,12.1579687885971));
#17253=CARTESIAN_POINT('Ctrl Pts',(-0.409729149087675,2.48538080092949,
12.1633301513777));
#17254=CARTESIAN_POINT('Ctrl Pts',(-0.49315877083768,2.47017263631205,12.1686915141582));
#17255=CARTESIAN_POINT('Ctrl Pts',(-0.575490003805714,2.45084016319296,
12.1740528769388));
#17256=CARTESIAN_POINT('Ctrl Pts',(-0.657821236773758,2.43150769007387,
12.1794142397194));
#17257=CARTESIAN_POINT('Ctrl Pts',(-0.739053611328862,2.40805111359026,
12.1847756024999));
#17258=CARTESIAN_POINT('Ctrl Pts',(-0.818757647879546,2.38063902430393,
12.1901369652805));
#17259=CARTESIAN_POINT('Ctrl Pts',(-0.896884163093578,2.35376948163886,
12.1953922146878));
#17260=CARTESIAN_POINT('Ctrl Pts',(-0.973830871246756,2.32300037319786,
12.2006474640951));
#17261=CARTESIAN_POINT('Ctrl Pts',(-1.04918106998781,2.28845479142133,12.2059027135024));
#17262=CARTESIAN_POINT('Ctrl Pts',(-1.12442443926459,2.25395818743193,12.2111505121599));
#17263=CARTESIAN_POINT('Ctrl Pts',(-1.19807537913551,2.21569593576888,12.2163983108174));
#17264=CARTESIAN_POINT('Ctrl Pts',(-1.26973397369639,2.17384035431334,12.2216461094749));
#17265=CARTESIAN_POINT('Ctrl Pts',(-1.34191179655186,2.1316814930864,12.2269319329578));
#17266=CARTESIAN_POINT('Ctrl Pts',(-1.41206783162651,2.08587716292094,12.2322177564407));
#17267=CARTESIAN_POINT('Ctrl Pts',(-1.47981554851215,2.03665220211544,12.2375035799236));
#17268=CARTESIAN_POINT('Ctrl Pts',(-1.54695577629684,1.98786863813568,12.2427420057922));
#17269=CARTESIAN_POINT('Ctrl Pts',(-1.61173032318671,1.93572581916218,12.2479804316608));
#17270=CARTESIAN_POINT('Ctrl Pts',(-1.67379070881036,1.88048688192715,12.2532188575294));
#17271=CARTESIAN_POINT('Ctrl Pts',(-1.73583068380593,1.82526611185936,12.2584555605669));
#17272=CARTESIAN_POINT('Ctrl Pts',(-1.79515792597853,1.76695155239302,12.2636922636044));
#17273=CARTESIAN_POINT('Ctrl Pts',(-1.85145756440794,1.7058461645754,12.2689289666419));
#17274=CARTESIAN_POINT('Ctrl Pts',(-1.90775566926345,1.6447424412379,12.2741655270342));
#17275=CARTESIAN_POINT('Ctrl Pts',(-1.96102602244995,1.58084838074151,12.2794020874266));
#17276=CARTESIAN_POINT('Ctrl Pts',(-2.01099207765506,1.51450226596351,12.2846386478189));
#17277=CARTESIAN_POINT('Ctrl Pts',(-2.06177594249721,1.44707024412675,12.2899609165894));
#17278=CARTESIAN_POINT('Ctrl Pts',(-2.10914606227333,1.37710556168465,12.2952831853599));
#17279=CARTESIAN_POINT('Ctrl Pts',(-2.15285720954222,1.30499505183816,12.3006054541303));
#17280=CARTESIAN_POINT('Ctrl Pts',(-2.19592620809399,1.23394389811207,12.3058495348807));
#17281=CARTESIAN_POINT('Ctrl Pts',(-2.23544285799706,1.16080998695817,12.311093615631));
#17282=CARTESIAN_POINT('Ctrl Pts',(-2.27121932313193,1.08598758567128,12.3163376963813));
#17283=CARTESIAN_POINT('Ctrl Pts',(-2.30779591638548,1.00949180757226,12.3216990591619));
#17284=CARTESIAN_POINT('Ctrl Pts',(-2.34046281303122,0.931231575526155,
12.3270604219424));
#17285=CARTESIAN_POINT('Ctrl Pts',(-2.3690722520371,0.851647177314573,12.332421784723));
#17286=CARTESIAN_POINT('Ctrl Pts',(-2.39768169104297,0.772062779102991,
12.3377831475035));
#17287=CARTESIAN_POINT('Ctrl Pts',(-2.42223358878511,0.691154720335989,
12.3431445102841));
#17288=CARTESIAN_POINT('Ctrl Pts',(-2.44263552689208,0.609375034576103,
12.3485058730646));
#17289=CARTESIAN_POINT('Ctrl Pts',(-2.46263366496502,0.529213951897958,
12.3537611224719));
#17290=CARTESIAN_POINT('Ctrl Pts',(-2.47871852955354,0.447919357606388,
12.3590163718793));
#17291=CARTESIAN_POINT('Ctrl Pts',(-2.49076649540138,0.365907796290177,
12.3642716212866));
#17292=CARTESIAN_POINT('Ctrl Pts',(-2.50279737997062,0.284012508737078,
12.3695194199441));
#17293=CARTESIAN_POINT('Ctrl Pts',(-2.51080266764662,0.201402725930073,
12.3747672186015));
#17294=CARTESIAN_POINT('Ctrl Pts',(-2.51470916250038,0.118507712983695,
12.380015017259));
#17295=CARTESIAN_POINT('Ctrl Pts',(-2.51864396327716,0.0350120542045962,
12.3853008407419));
#17296=CARTESIAN_POINT('Ctrl Pts',(-2.51842020731908,-0.0487725258359569,
12.3905866642249));
#17297=CARTESIAN_POINT('Ctrl Pts',(-2.5140160401722,-0.132399394851013,
12.3958724877078));
#17298=CARTESIAN_POINT('Ctrl Pts',(-2.50965136488812,-0.215276387503942,
12.4011109135763));
#17299=CARTESIAN_POINT('Ctrl Pts',(-2.50118097377524,-0.297998016898358,
12.4063493394449));
#17300=CARTESIAN_POINT('Ctrl Pts',(-2.48863585321229,-0.380128715182573,
12.4115877653135));
#17301=CARTESIAN_POINT('Ctrl Pts',(-2.47609485853071,-0.462232402046997,
12.416824468351));
#17302=CARTESIAN_POINT('Ctrl Pts',(-2.4594818655495,-0.543745088015308,
12.4220611713885));
#17303=CARTESIAN_POINT('Ctrl Pts',(-2.43887956369379,-0.624237714173704,
12.427297874426));
#17304=CARTESIAN_POINT('Ctrl Pts',(-2.41827782303446,-0.704728147753272,
12.4325344348183));
#17305=CARTESIAN_POINT('Ctrl Pts',(-2.39368710497056,-0.784198130013413,
12.4377709952107));
#17306=CARTESIAN_POINT('Ctrl Pts',(-2.36524059249831,-0.862231517400193,
12.443007555603));
#17307=CARTESIAN_POINT('Ctrl Pts',(-2.33632848729624,-0.941542100994626,
12.4483298243735));
#17308=CARTESIAN_POINT('Ctrl Pts',(-2.30343338708723,-1.01936817258425,
12.453652093144));
#17309=CARTESIAN_POINT('Ctrl Pts',(-2.26674625011272,-1.09529342534315,
12.4589743619144));
#17310=CARTESIAN_POINT('Ctrl Pts',(-2.23059807400783,-1.17010328061869,
12.4642184426648));
#17311=CARTESIAN_POINT('Ctrl Pts',(-2.19076881527345,-1.24306741378626,
12.4694625234151));
#17312=CARTESIAN_POINT('Ctrl Pts',(-2.14748691460629,-1.31381360991381,
12.4747066041654));
#17313=CARTESIAN_POINT('Ctrl Pts',(-2.10323702938211,-1.38614201995211,
12.480067966946));
#17314=CARTESIAN_POINT('Ctrl Pts',(-2.05537849337824,-1.45615166634425,
12.4854293297265));
#17315=CARTESIAN_POINT('Ctrl Pts',(-2.00420016786459,-1.52347889290648,
12.4907906925071));
#17316=CARTESIAN_POINT('Ctrl Pts',(-1.95302184235094,-1.59080611946871,
12.4961520552876));
#17317=CARTESIAN_POINT('Ctrl Pts',(-1.89852410590017,-1.65545058077777,
12.5015134180682));
#17318=CARTESIAN_POINT('Ctrl Pts',(-1.8410358034506,-1.71708864663797,12.5068747808488));
#17319=CARTESIAN_POINT('Ctrl Pts',(-1.78468532321994,-1.77750675717024,
12.5121300302561));
#17320=CARTESIAN_POINT('Ctrl Pts',(-1.7252534743354,-1.83525958626136,12.5173852796634));
#17321=CARTESIAN_POINT('Ctrl Pts',(-1.66302234322075,-1.89001664964851,
12.5226405290707));
#17322=CARTESIAN_POINT('Ctrl Pts',(-1.6008794417127,-1.94469607995917,12.5278883277282));
#17323=CARTESIAN_POINT('Ctrl Pts',(-1.53594548458524,-1.99638787870886,
12.5331361263857));
#17324=CARTESIAN_POINT('Ctrl Pts',(-1.46854068446692,-2.04479693565533,
12.5383839250432));
#17325=CARTESIAN_POINT('Ctrl Pts',(-1.40064747846204,-2.09355675795285,
12.5436697485261));
#17326=CARTESIAN_POINT('Ctrl Pts',(-1.33024779482607,-2.13898571857549,
12.548955572009));
#17327=CARTESIAN_POINT('Ctrl Pts',(-1.25770436658404,-2.18082231653004,
12.5542413954919));
#17328=CARTESIAN_POINT('Ctrl Pts',(-1.18581143025568,-2.22228376859854,
12.5594798213605));
#17329=CARTESIAN_POINT('Ctrl Pts',(-1.1118134480378,-2.26021679013605,12.5647182472291));
#17330=CARTESIAN_POINT('Ctrl Pts',(-1.03609264146632,-2.29441022668122,
12.5699566730977));
#17331=CARTESIAN_POINT('Ctrl Pts',(-0.960396738207965,-2.32859241757415,
12.5751933761352));
#17332=CARTESIAN_POINT('Ctrl Pts',(-0.882979556111035,-2.35903727634762,
12.5804300791727));
#17333=CARTESIAN_POINT('Ctrl Pts',(-0.80424600686889,-2.38558056045807,
12.5856667822102));
#17334=CARTESIAN_POINT('Ctrl Pts',(-0.725514602289312,-2.41212312154272,
12.5909033426025));
#17335=CARTESIAN_POINT('Ctrl Pts',(-0.645467339429018,-2.43476417284083,
12.5961399029949));
#17336=CARTESIAN_POINT('Ctrl Pts',(-0.564525787980757,-2.45338885721459,
12.6013764633872));
#17337=CARTESIAN_POINT('Ctrl Pts',(-0.482259441518213,-2.47231837746756,
12.6066987321577));
#17338=CARTESIAN_POINT('Ctrl Pts',(-0.399069744423423,-2.4870987473584,
12.6120210009282));
#17339=CARTESIAN_POINT('Ctrl Pts',(-0.315409859162885,-2.49766348228556,
12.6173432696986));
#17340=CARTESIAN_POINT('Ctrl Pts',(-0.232978998793114,-2.50807301353119,
12.622587350449));
#17341=CARTESIAN_POINT('Ctrl Pts',(-0.15009214470415,-2.51438997478315,
12.6278314311993));
#17342=CARTESIAN_POINT('Ctrl Pts',(-0.0671858828033769,-2.51660332733467,
12.6330755119496));
#17343=CARTESIAN_POINT('Ctrl Pts',(0.0175745486223677,-2.5188661807412,
12.6384368747302));
#17344=CARTESIAN_POINT('Ctrl Pts',(0.102354754540799,-2.51683967122696,
12.6437982375108));
#17345=CARTESIAN_POINT('Ctrl Pts',(0.186692431981194,-2.51056810021974,
12.6491596002913));
#17346=CARTESIAN_POINT('Ctrl Pts',(0.27103010942159,-2.50429652921252,12.6545209630719));
#17347=CARTESIAN_POINT('Ctrl Pts',(0.354924762531114,-2.49378002618991,
12.6598823258524));
#17348=CARTESIAN_POINT('Ctrl Pts',(0.437925892658355,-2.47911822278394,
12.665243688633));
#17349=CARTESIAN_POINT('Ctrl Pts',(0.519284244584921,-2.46474660929443,
12.6704989380403));
#17350=CARTESIAN_POINT('Ctrl Pts',(0.600084634974541,-2.44633925090901,
12.6757541874476));
#17351=CARTESIAN_POINT('Ctrl Pts',(0.679896273783434,-2.42395282687089,
12.6810094368549));
#17352=CARTESIAN_POINT('Ctrl Pts',(0.75959475781951,-2.40159814169649,12.6862572355124));
#17353=CARTESIAN_POINT('Ctrl Pts',(0.838306834140221,-2.37527571993383,
12.6915050341698));
#17354=CARTESIAN_POINT('Ctrl Pts',(0.915610626285604,-2.34509348023333,
12.6967528328273));
#17355=CARTESIAN_POINT('Ctrl Pts',(0.993474551048993,-2.31469254418597,
12.7020386563102));
#17356=CARTESIAN_POINT('Ctrl Pts',(1.06990923039545,-2.28037570120017,12.7073244797932));
#17357=CARTESIAN_POINT('Ctrl Pts',(1.14449782874756,-2.24230483431494,12.7126103032761));
#17358=CARTESIAN_POINT('Ctrl Pts',(1.21841759628679,-2.20457534626519,12.7178487291447));
#17359=CARTESIAN_POINT('Ctrl Pts',(1.29052383903844,-2.16315910245273,12.7230871550133));
#17360=CARTESIAN_POINT('Ctrl Pts',(1.36043134115744,-2.11826174397702,12.7283255808819));
#17361=CARTESIAN_POINT('Ctrl Pts',(1.43031585186234,-2.07337915149537,12.7335622839194));
#17362=CARTESIAN_POINT('Ctrl Pts',(1.49800267016891,-2.0250179672967,12.7387989869569));
#17363=CARTESIAN_POINT('Ctrl Pts',(1.56313357589519,-1.97342840607637,12.7440356899944));
#17364=CARTESIAN_POINT('Ctrl Pts',(1.6282627074881,-1.92184025012994,12.7492722503867));
#17365=CARTESIAN_POINT('Ctrl Pts',(1.69083570386656,-1.86702417931556,12.754508810779));
#17366=CARTESIAN_POINT('Ctrl Pts',(1.75052669947214,-1.8092712688912,12.7597453711714));
#17367=CARTESIAN_POINT('Ctrl Pts',(1.8111946757751,-1.75057309899965,12.7650676399418));
#17368=CARTESIAN_POINT('Ctrl Pts',(1.86888509645734,-1.6888414183296,12.7703899087123));
#17369=CARTESIAN_POINT('Ctrl Pts',(1.92329546973574,-1.62442013841678,12.7757121774828));
#17370=CARTESIAN_POINT('Ctrl Pts',(1.97690651484305,-1.56094525421398,12.7809562582331));
#17371=CARTESIAN_POINT('Ctrl Pts',(2.02733301030535,-1.49485967987571,12.7862003389835));
#17372=CARTESIAN_POINT('Ctrl Pts',(2.07432799706175,-1.42652361025178,12.7914444197338));
#17373=CARTESIAN_POINT('Ctrl Pts',(2.12237401024577,-1.35665922835262,12.7968057825144));
#17374=CARTESIAN_POINT('Ctrl Pts',(2.1668329051569,-1.28444290942349,12.8021671452949));
#17375=CARTESIAN_POINT('Ctrl Pts',(2.20749013991691,-1.21028654961112,12.8075285080755));
#17376=CARTESIAN_POINT('Ctrl Pts',(2.24814737467694,-1.13613018979875,12.812889870856));
#17377=CARTESIAN_POINT('Ctrl Pts',(2.2850027879228,-1.06003427551497,12.8182512336366));
#17378=CARTESIAN_POINT('Ctrl Pts',(2.31789467520479,-0.982430926150674,
12.8236125964172));
#17379=CARTESIAN_POINT('Ctrl Pts',(2.35361447071358,-0.898155562249387,
12.8294349069623));
#17380=CARTESIAN_POINT('Ctrl Pts',(2.38477328167352,-0.811838041542797,
12.8352572175074));
#17381=CARTESIAN_POINT('Ctrl Pts',(2.41115846466759,-0.723962090348533,
12.8410795280525));
#17382=CARTESIAN_POINT('Ctrl Pts',(2.437464413732,-0.636350028055026,12.84688435437));
#17383=CARTESIAN_POINT('Ctrl Pts',(2.45902521036186,-0.547189130624484,
12.8526891806875));
#17384=CARTESIAN_POINT('Ctrl Pts',(2.47567650290169,-0.456981512733812,
12.858494007005));
#17385=CARTESIAN_POINT('Ctrl Pts',(2.49224191268916,-0.367239160737021,
12.864268893637));
#17386=CARTESIAN_POINT('Ctrl Pts',(2.50394821153212,-0.276461124821933,
12.8700437802691));
#17387=CARTESIAN_POINT('Ctrl Pts',(2.51068155182407,-0.185160458333482,
12.8758186669011));
#17388=CARTESIAN_POINT('Ctrl Pts',(2.51518920085692,-0.124039032243293,
12.8796846770852));
#17389=CARTESIAN_POINT('Ctrl Pts',(2.51746912849982,-0.0626837621653072,
12.8835506872694));
#17390=CARTESIAN_POINT('Ctrl Pts',(2.51749968849485,-0.00125236909204737,
12.8874166974535));
#17391=CARTESIAN_POINT('Ctrl Pts',(2.51749968849528,-0.00125236822527237,
12.887416697508));
#17392=CARTESIAN_POINT('Ctrl Pts',(2.51754167409805,0.0831467244342282,
12.8927281146097));
#17393=CARTESIAN_POINT('Ctrl Pts',(2.51333509749615,0.167540690501748,12.8980395317113));
#17394=CARTESIAN_POINT('Ctrl Pts',(2.50490792228564,0.251480716697432,12.9033509488129));
#17395=CARTESIAN_POINT('Ctrl Pts',(2.49647888833066,0.335439257170471,12.9086635374302));
#17396=CARTESIAN_POINT('Ctrl Pts',(2.48382745746316,0.418943218731677,12.9139761260474));
#17397=CARTESIAN_POINT('Ctrl Pts',(2.46703330555087,0.501550515205346,12.9192887146647));
#17398=CARTESIAN_POINT('Ctrl Pts',(2.4502220639129,0.584241872847674,12.924606709371));
#17399=CARTESIAN_POINT('Ctrl Pts',(2.42925978258897,0.66603431133487,12.9299247040774));
#17400=CARTESIAN_POINT('Ctrl Pts',(2.40427682702775,0.746497949774397,12.9352426987838));
#17401=CARTESIAN_POINT('Ctrl Pts',(2.39110116072441,0.788933363271986,12.9380473358686));
#17402=CARTESIAN_POINT('Ctrl Pts',(2.37680803330578,0.830999455775601,12.9408519729533));
#17403=CARTESIAN_POINT('Ctrl Pts',(2.36142200728636,0.872635292378012,12.9436566100381));
#17404=CARTESIAN_POINT('',(2.51749934966675,0.00180953791660804,12.610970894458));
#17405=CARTESIAN_POINT('Ctrl Pts',(2.36142200728627,0.872635292378268,12.6712695847815));
#17406=CARTESIAN_POINT('Ctrl Pts',(2.3622945071155,0.870274236945268,12.6711089481077));
#17407=CARTESIAN_POINT('Ctrl Pts',(2.36316345899157,0.867911891698931,12.6709481031855));
#17408=CARTESIAN_POINT('Ctrl Pts',(2.36727334457552,0.856686765890141,12.6701832599527));
#17409=CARTESIAN_POINT('Ctrl Pts',(2.37046791552923,0.847807264339659,12.6695765880174));
#17410=CARTESIAN_POINT('Ctrl Pts',(2.3815053195227,0.816578034044917,12.66743765534));
#17411=CARTESIAN_POINT('Ctrl Pts',(2.38908231813799,0.794136546107376,12.6658911799632));
#17412=CARTESIAN_POINT('Ctrl Pts',(2.40707461124876,0.738257730667373,12.6620229098741));
#17413=CARTESIAN_POINT('Ctrl Pts',(2.41711073903533,0.704704258671639,12.6596847265558));
#17414=CARTESIAN_POINT('Ctrl Pts',(2.48670743765461,0.453014266688823,12.6420836116566));
#17415=CARTESIAN_POINT('Ctrl Pts',(2.51733680247564,0.227951496130733,12.6261205826785));
#17416=CARTESIAN_POINT('Ctrl Pts',(2.51749934966675,0.00180953791660804,
12.610970894458));
#17417=CARTESIAN_POINT('Ctrl Pts',(2.5174993518837,0.00180645098896169,
12.6109706876588));
#17418=CARTESIAN_POINT('Ctrl Pts',(2.51753502679323,-0.0479106806532836,
12.6076400421281));
#17419=CARTESIAN_POINT('Ctrl Pts',(2.51609793727693,-0.0976210787494668,
12.6043466370876));
#17420=CARTESIAN_POINT('Ctrl Pts',(2.51134124597573,-0.178800545830599,
12.5990304130993));
#17421=CARTESIAN_POINT('Ctrl Pts',(2.50889945893777,-0.210304875616481,
12.5969825419673));
#17422=CARTESIAN_POINT('Ctrl Pts',(2.50439206707403,-0.257025172510051,
12.5939674482425));
#17423=CARTESIAN_POINT('Ctrl Pts',(2.50277941099293,-0.272280740881106,
12.592986394353));
#17424=CARTESIAN_POINT('Ctrl Pts',(2.49970477899756,-0.299025714575572,
12.5912723517902));
#17425=CARTESIAN_POINT('Ctrl Pts',(2.49830278659595,-0.310521422626574,
12.5905375179727));
#17426=CARTESIAN_POINT('Ctrl Pts',(2.4954086528572,-0.332962334552027,12.5891066406945));
#17427=CARTESIAN_POINT('Ctrl Pts',(2.49392370133097,-0.3439081842779,12.5884103894646));
#17428=CARTESIAN_POINT('Ctrl Pts',(2.49082989607196,-0.365638567925284,
12.587031350738));
#17429=CARTESIAN_POINT('Ctrl Pts',(2.48922292550844,-0.376423121792505,
12.5863485205199));
#17430=CARTESIAN_POINT('Ctrl Pts',(2.48527387919882,-0.401793755381892,
12.5847456934798));
#17431=CARTESIAN_POINT('Ctrl Pts',(2.48287336620441,-0.416370434172154,
12.5838275452231));
#17432=CARTESIAN_POINT('Ctrl Pts',(2.47403688916322,-0.467231927160941,
12.5806328050258));
#17433=CARTESIAN_POINT('Ctrl Pts',(2.46693250069783,-0.503396912815185,
12.5783771391568));
#17434=CARTESIAN_POINT('Ctrl Pts',(2.44188583165782,-0.617581774736163,
12.571292907895));
#17435=CARTESIAN_POINT('Ctrl Pts',(2.4210151264175,-0.694910820068047,12.566553177363));
#17436=CARTESIAN_POINT('Ctrl Pts',(2.35621427086737,-0.896299674260321,
12.5542023333951));
#17437=CARTESIAN_POINT('Ctrl Pts',(2.30618943417384,-1.01813028628443,12.5467303653566));
#17438=CARTESIAN_POINT('Ctrl Pts',(2.19889978294303,-1.23043098565515,12.5329781504577));
#17439=CARTESIAN_POINT('Ctrl Pts',(2.14495939077477,-1.32221967013425,12.5267527110818));
#17440=CARTESIAN_POINT('Ctrl Pts',(2.07328091897847,-1.42820841116114,12.518892285439));
#17441=CARTESIAN_POINT('Ctrl Pts',(2.06094819817612,-1.44594795443168,12.5175525565895));
#17442=CARTESIAN_POINT('Ctrl Pts',(2.04309990110297,-1.47092889876943,12.5156280018374));
#17443=CARTESIAN_POINT('Ctrl Pts',(2.03777062349898,-1.47830305116941,12.5150551115847));
#17444=CARTESIAN_POINT('Ctrl Pts',(2.02850160420936,-1.49098328853693,12.5140614088374));
#17445=CARTESIAN_POINT('Ctrl Pts',(2.02458067313543,-1.49630311839935,12.5136418739513));
#17446=CARTESIAN_POINT('Ctrl Pts',(2.01630325866709,-1.50744162532234,12.5127577928314));
#17447=CARTESIAN_POINT('Ctrl Pts',(2.01194250467107,-1.513256898009,12.5122929680561));
#17448=CARTESIAN_POINT('Ctrl Pts',(2.00015559153102,-1.52883429693761,12.5110392410938));
#17449=CARTESIAN_POINT('Ctrl Pts',(1.9926832803624,-1.53856102496411,12.5102472571239));
#17450=CARTESIAN_POINT('Ctrl Pts',(1.95838778671657,-1.58253463224009,12.5066264560169));
#17451=CARTESIAN_POINT('Ctrl Pts',(1.93075240823426,-1.61613526630451,12.5037476749076));
#17452=CARTESIAN_POINT('Ctrl Pts',(1.78284352136868,-1.78676074313925,12.4886066925734));
#17453=CARTESIAN_POINT('Ctrl Pts',(1.64881631912947,-1.91113850022334,12.4758090773104));
#17454=CARTESIAN_POINT('Ctrl Pts',(1.43370485933303,-2.07114820920674,12.4574951990103));
#17455=CARTESIAN_POINT('Ctrl Pts',(1.36230101007205,-2.11879750899754,12.4517145093992));
#17456=CARTESIAN_POINT('Ctrl Pts',(1.25778789962102,-2.18106901929841,12.4436905551074));
#17457=CARTESIAN_POINT('Ctrl Pts',(1.22658834326324,-2.19876640738806,12.4413469831263));
#17458=CARTESIAN_POINT('Ctrl Pts',(1.17056568424307,-2.2289805252545,12.4372288802163));
#17459=CARTESIAN_POINT('Ctrl Pts',(1.14589398531373,-2.24176387660513,12.4354453957186));
#17460=CARTESIAN_POINT('Ctrl Pts',(1.10835981084241,-2.26043016692362,12.4327761325644));
#17461=CARTESIAN_POINT('Ctrl Pts',(1.09565175292343,-2.26661714001533,12.4318798744822));
#17462=CARTESIAN_POINT('Ctrl Pts',(1.0827761806386,-2.27275207823372,12.4309791978059));
#17463=CARTESIAN_POINT('Ctrl Pts',(1.08266030617716,-2.27280727909394,12.4309710927155));
#17464=CARTESIAN_POINT('Ctrl Pts',(1.08242158526773,-2.2729209797659,12.4309543961035));
#17465=CARTESIAN_POINT('Ctrl Pts',(1.0822987383012,-2.27297947847866,12.4309458046201));
#17466=CARTESIAN_POINT('Ctrl Pts',(1.0820456281083,-2.27309998229397,12.4309281043788));
#17467=CARTESIAN_POINT('Ctrl Pts',(1.08191536428114,-2.27316198616499,12.4309189956628));
#17468=CARTESIAN_POINT('Ctrl Pts',(1.08164694547373,-2.27328972169295,12.4309002280064));
#17469=CARTESIAN_POINT('Ctrl Pts',(1.08150878982745,-2.27335545195498,12.430890569114));
#17470=CARTESIAN_POINT('Ctrl Pts',(1.08122407962554,-2.2734908765978,12.4308706658953));
#17471=CARTESIAN_POINT('Ctrl Pts',(1.08107752432224,-2.27356056940229,12.4308604216237));
#17472=CARTESIAN_POINT('Ctrl Pts',(1.08077547179291,-2.2737041714376,12.4308393100165));
#17473=CARTESIAN_POINT('Ctrl Pts',(1.08061997372362,-2.27377807888799,12.4308284427426));
#17474=CARTESIAN_POINT('Ctrl Pts',(1.08029945483932,-2.27393037959636,12.430806044908));
#17475=CARTESIAN_POINT('Ctrl Pts',(1.08013443305777,-2.27400877084948,12.4307945144158));
#17476=CARTESIAN_POINT('Ctrl Pts',(1.07979424537833,-2.27417032678893,12.4307707471446));
#17477=CARTESIAN_POINT('Ctrl Pts',(1.07961907840034,-2.27425348920332,12.4307585104438));
#17478=CARTESIAN_POINT('Ctrl Pts',(1.07925793555186,-2.27442489454415,12.4307332847866));
#17479=CARTESIAN_POINT('Ctrl Pts',(1.07907195845855,-2.27451313490213,12.4307202959186));
#17480=CARTESIAN_POINT('Ctrl Pts',(1.07868848418916,-2.27469502392142,12.4306935167885));
#17481=CARTESIAN_POINT('Ctrl Pts',(1.0784909856272,-2.27478866967816,12.4306797266263));
#17482=CARTESIAN_POINT('Ctrl Pts',(1.0780837076643,-2.27498171930179,12.4306512923904));
#17483=CARTESIAN_POINT('Ctrl Pts',(1.07787392670094,-2.27508111987834,12.4306366484301));
#17484=CARTESIAN_POINT('Ctrl Pts',(1.07744127037446,-2.27528605228095,12.4306064504874));
#17485=CARTESIAN_POINT('Ctrl Pts',(1.07721839324281,-2.27539158038124,12.4305908966333));
#17486=CARTESIAN_POINT('Ctrl Pts',(1.07675867490992,-2.27560916562066,12.430558818982));
#17487=CARTESIAN_POINT('Ctrl Pts',(1.07652183169936,-2.27572121854266,12.4305422953296));
#17488=CARTESIAN_POINT('Ctrl Pts',(1.07613177902632,-2.2759056818959,12.4305150869449));
#17489=CARTESIAN_POINT('Ctrl Pts',(1.07597857978567,-2.27597811381367,12.4305044014736));
#17490=CARTESIAN_POINT('Ctrl Pts',(1.07562125605292,-2.27614701073974,12.4304794809875));
#17491=CARTESIAN_POINT('Ctrl Pts',(1.07541712587571,-2.27624346376778,12.4304652463851));
#17492=CARTESIAN_POINT('Ctrl Pts',(1.06471534816574,-2.28129837247681,12.4297190767861));
#17493=CARTESIAN_POINT('Ctrl Pts',(1.05418340088328,-2.28618424486074,12.4289896462315));
#17494=CARTESIAN_POINT('Ctrl Pts',(1.03052184163024,-2.29696279448139,12.4273616186799));
#17495=CARTESIAN_POINT('Ctrl Pts',(1.01737467487582,-2.30281613026747,12.426464379949));
#17496=CARTESIAN_POINT('Ctrl Pts',(0.983780310747627,-2.31742903458171,
12.4241898681064));
#17497=CARTESIAN_POINT('Ctrl Pts',(0.9632656275026,-2.32603104222524,12.4228179060099));
#17498=CARTESIAN_POINT('Ctrl Pts',(0.792808776154341,-2.39486330421806,
12.411551077741));
#17499=CARTESIAN_POINT('Ctrl Pts',(0.637494800194419,-2.44080433708856,
12.4021620679572));
#17500=CARTESIAN_POINT('Ctrl Pts',(0.357381015113579,-2.49507288997588,
12.3857481191458));
#17501=CARTESIAN_POINT('Ctrl Pts',(0.23436924749912,-2.50961700859083,12.3786973985936));
#17502=CARTESIAN_POINT('Ctrl Pts',(0.0667511149687532,-2.51700102679946,
12.3687782844453));
#17503=CARTESIAN_POINT('Ctrl Pts',(0.022666244979773,-2.51778388432851,
12.3661395576425));
#17504=CARTESIAN_POINT('Ctrl Pts',(-0.0494487216010663,-2.51717045189379,
12.3617419375182));
#17505=CARTESIAN_POINT('Ctrl Pts',(-0.077476295193672,-2.51646369580423,
12.3600127161011));
#17506=CARTESIAN_POINT('Ctrl Pts',(-0.115552088885675,-2.51486689357172,
12.3576292104596));
#17507=CARTESIAN_POINT('Ctrl Pts',(-0.125616505973406,-2.51438427114253,
12.3569959223817));
#17508=CARTESIAN_POINT('Ctrl Pts',(-0.142457978641892,-2.51347529974156,
12.3559303266728));
#17509=CARTESIAN_POINT('Ctrl Pts',(-0.14923682384159,-2.51308191800922,
12.3554998207836));
#17510=CARTESIAN_POINT('Ctrl Pts',(-0.162111950565015,-2.51228248704699,
12.3546789893125));
#17511=CARTESIAN_POINT('Ctrl Pts',(-0.168208496366009,-2.51188166104113,
12.3542889688832));
#17512=CARTESIAN_POINT('Ctrl Pts',(-0.182696756992745,-2.51087612837025,
12.353358993859));
#17513=CARTESIAN_POINT('Ctrl Pts',(-0.191086955732838,-2.51025154269353,
12.3528179661915));
#17514=CARTESIAN_POINT('Ctrl Pts',(-0.220758851074861,-2.50789307959591,
12.3508962330294));
#17515=CARTESIAN_POINT('Ctrl Pts',(-0.242020777320876,-2.50593057393651,
12.3495039009692));
#17516=CARTESIAN_POINT('Ctrl Pts',(-0.400500327497464,-2.48926705164925,
12.3390242943463));
#17517=CARTESIAN_POINT('Ctrl Pts',(-0.536314863442209,-2.4635767446743,
12.3294871342398));
#17518=CARTESIAN_POINT('Ctrl Pts',(-0.796167652203041,-2.39191049262016,
12.31086467475));
#17519=CARTESIAN_POINT('Ctrl Pts',(-0.920082980298449,-2.3470347978668,
12.3018081875349));
#17520=CARTESIAN_POINT('Ctrl Pts',(-1.08552342765433,-2.27199284000306,
12.2896710729925));
#17521=CARTESIAN_POINT('Ctrl Pts',(-1.13049101877052,-2.24995626269979,
12.2863652080218));
#17522=CARTESIAN_POINT('Ctrl Pts',(-1.20680989961236,-2.20968959398645,
12.2807434875941));
#17523=CARTESIAN_POINT('Ctrl Pts',(-1.2384784677822,-2.19209706516752,12.2784072668224));
#17524=CARTESIAN_POINT('Ctrl Pts',(-1.28344736547907,-2.16583020015199,
12.2750831676069));
#17525=CARTESIAN_POINT('Ctrl Pts',(-1.29706138900641,-2.15770465257502,
12.2740759007525));
#17526=CARTESIAN_POINT('Ctrl Pts',(-1.32066558176627,-2.14331232190712,
12.2723275885426));
#17527=CARTESIAN_POINT('Ctrl Pts',(-1.33069004234187,-2.13710301739542,
12.2715844916702));
#17528=CARTESIAN_POINT('Ctrl Pts',(-1.35128588144678,-2.12414453542423,
12.2700563279025));
#17529=CARTESIAN_POINT('Ctrl Pts',(-1.36185120870613,-2.11738632166915,
12.2692716189572));
#17530=CARTESIAN_POINT('Ctrl Pts',(-1.388829843696,-2.09984370663774,12.2672655363098));
#17531=CARTESIAN_POINT('Ctrl Pts',(-1.40516845638597,-2.08894556418483,
12.2660484007814));
#17532=CARTESIAN_POINT('Ctrl Pts',(-1.46979862521322,-2.04473467245724,
12.2612227813788));
#17533=CARTESIAN_POINT('Ctrl Pts',(-1.5170489259708,-2.00992816639374,12.2576705057414));
#17534=CARTESIAN_POINT('Ctrl Pts',(-1.72579779442693,-1.84459582756289,
12.2417770952425));
#17535=CARTESIAN_POINT('Ctrl Pts',(-1.87197322476266,-1.69606194493632,
12.2301558254995));
#17536=CARTESIAN_POINT('Ctrl Pts',(-2.03645719747082,-1.48141591856693,
12.2143912886018));
#17537=CARTESIAN_POINT('Ctrl Pts',(-2.07277844330027,-1.43015367259183,
12.210685005293));
#17538=CARTESIAN_POINT('Ctrl Pts',(-2.12034694811258,-1.35739358746677,
12.2054259727978));
#17539=CARTESIAN_POINT('Ctrl Pts',(-2.13325974157092,-1.33700834659444,
12.2039526674916));
#17540=CARTESIAN_POINT('Ctrl Pts',(-2.15521342002102,-1.30122255840699,
12.2013608065886));
#17541=CARTESIAN_POINT('Ctrl Pts',(-2.16438734261813,-1.28590529261611,
12.2002497016387));
#17542=CARTESIAN_POINT('Ctrl Pts',(-2.17765003278284,-1.26321716174244,
12.1985994297712));
#17543=CARTESIAN_POINT('Ctrl Pts',(-2.18186617108675,-1.25592088509911,
12.1980680435391));
#17544=CARTESIAN_POINT('Ctrl Pts',(-2.18928143734325,-1.24293829535928,
12.197121079376));
#17545=CARTESIAN_POINT('Ctrl Pts',(-2.19249519720356,-1.23726053310948,
12.1967064402557));
#17546=CARTESIAN_POINT('Ctrl Pts',(-2.19942742888982,-1.22490150561083,
12.1958027379516));
#17547=CARTESIAN_POINT('Ctrl Pts',(-2.20313748731257,-1.21821587648048,
12.1953131832861));
#17548=CARTESIAN_POINT('Ctrl Pts',(-2.21336956741047,-1.19957776227024,
12.1939466987359));
#17549=CARTESIAN_POINT('Ctrl Pts',(-2.21982504902044,-1.18758931534281,
12.1930658007409));
#17550=CARTESIAN_POINT('Ctrl Pts',(-2.25558281238821,-1.1198734739857,12.1880817056283));
#17551=CARTESIAN_POINT('Ctrl Pts',(-2.28288131199852,-1.06311895953314,
12.1838729962112));
#17552=CARTESIAN_POINT('Ctrl Pts',(-2.39800619574733,-0.798837093132328,
12.1643198150031));
#17553=CARTESIAN_POINT('Ctrl Pts',(-2.45986770478959,-0.581076485295152,
12.1484505317142));
#17554=CARTESIAN_POINT('Ctrl Pts',(-2.49856032727949,-0.311746033951842,
12.1303222117129));
#17555=CARTESIAN_POINT('Ctrl Pts',(-2.50391599256939,-0.26531953030825,
12.1272439758556));
#17556=CARTESIAN_POINT('Ctrl Pts',(-2.51096291740736,-0.18453306064284,
12.1219686601374));
#17557=CARTESIAN_POINT('Ctrl Pts',(-2.51324803412135,-0.150238917919318,
12.1197544124582));
#17558=CARTESIAN_POINT('Ctrl Pts',(-2.51554529255956,-0.100395507988638,
12.1165711760848));
#17559=CARTESIAN_POINT('Ctrl Pts',(-2.51611670303056,-0.0848771540916381,
12.1155849997241));
#17560=CARTESIAN_POINT('Ctrl Pts',(-2.51686795494256,-0.0576176892375606,
12.113861013185));
#17561=CARTESIAN_POINT('Ctrl Pts',(-2.51710930161321,-0.0458788841228253,
12.1131213177217));
#17562=CARTESIAN_POINT('Ctrl Pts',(-2.51741935106567,-0.0230168916542543,
12.1116858325763));
#17563=CARTESIAN_POINT('Ctrl Pts',(-2.51749647525531,-0.0118941091298984,
12.1109897988483));
#17564=CARTESIAN_POINT('Ctrl Pts',(-2.51750563405195,0.0180101399364491,
12.109124590416));
#17565=CARTESIAN_POINT('Ctrl Pts',(-2.51730121793708,0.036791174643719,
12.1079596596674));
#17566=CARTESIAN_POINT('Ctrl Pts',(-2.5157390714679,0.107546023137503,12.1035937154676));
#17567=CARTESIAN_POINT('Ctrl Pts',(-2.51298161306114,0.159477908940482,
12.1004358860706));
#17568=CARTESIAN_POINT('Ctrl Pts',(-2.49057414599155,0.425518691437462,
12.0844327093301));
#17569=CARTESIAN_POINT('Ctrl Pts',(-2.44516671392129,0.636540634410002,
12.0724081630507));
#17570=CARTESIAN_POINT('Ctrl Pts',(-2.35230662518016,0.899167255119664,
12.05617656775));
#17571=CARTESIAN_POINT('Ctrl Pts',(-2.32885134072189,0.958278965263406,
12.0524268683046));
#17572=CARTESIAN_POINT('Ctrl Pts',(-2.28857712867055,1.04953807732663,12.0463938697484));
#17573=CARTESIAN_POINT('Ctrl Pts',(-2.27325727258668,1.08231996759801,12.0441754055428));
#17574=CARTESIAN_POINT('Ctrl Pts',(-2.25233428925201,1.12468622344181,12.0412261952961));
#17575=CARTESIAN_POINT('Ctrl Pts',(-2.24736597711045,1.13458142328223,12.0405314138683));
#17576=CARTESIAN_POINT('Ctrl Pts',(-2.23914821849367,1.15068265638373,12.0393906069351));
#17577=CARTESIAN_POINT('Ctrl Pts',(-2.23593779605627,1.15690859163188,12.0389469584269));
#17578=CARTESIAN_POINT('Ctrl Pts',(-2.22962375471788,1.16902888690866,12.0380781890607));
#17579=CARTESIAN_POINT('Ctrl Pts',(-2.22652266056816,1.1749244504983,12.0376532235637));
#17580=CARTESIAN_POINT('Ctrl Pts',(-2.21954745574235,1.18805839315335,12.0367012914962));
#17581=CARTESIAN_POINT('Ctrl Pts',(-2.21566126416068,1.19529026260172,12.0361735846493));
#17582=CARTESIAN_POINT('Ctrl Pts',(-2.20211180975773,1.22021150702354,12.0343431311956));
#17583=CARTESIAN_POINT('Ctrl Pts',(-2.19227180478373,1.23780322277386,12.0330301104735));
#17584=CARTESIAN_POINT('Ctrl Pts',(-2.09862745198669,1.40059854144838,12.0206963188929));
#17585=CARTESIAN_POINT('Ctrl Pts',(-2.00073227821853,1.53719730463512,12.0090094862668));
#17586=CARTESIAN_POINT('Ctrl Pts',(-1.78975632717178,1.77696523595894,11.986986982023));
#17587=CARTESIAN_POINT('Ctrl Pts',(-1.67940565642236,1.88160644656731,11.9766721875944));
#17588=CARTESIAN_POINT('Ctrl Pts',(-1.53072294342952,1.99902788093899,11.9643152105487));
#17589=CARTESIAN_POINT('Ctrl Pts',(-1.50063967009827,2.02170869046113,11.9618837438889));
#17590=CARTESIAN_POINT('Ctrl Pts',(-1.45698744941406,2.05310813846939,11.9584502701666));
#17591=CARTESIAN_POINT('Ctrl Pts',(-1.44382744411486,2.06238400577086,11.9574270700946));
#17592=CARTESIAN_POINT('Ctrl Pts',(-1.42084297667296,2.07825683821559,11.9556602249378));
#17593=CARTESIAN_POINT('Ctrl Pts',(-1.41105943497202,2.08491187551337,11.9549144013992));
#17594=CARTESIAN_POINT('Ctrl Pts',(-1.39211855634074,2.09760159120119,11.9534823155637));
#17595=CARTESIAN_POINT('Ctrl Pts',(-1.38296801366096,2.10364588027217,11.9527957054004));
#17596=CARTESIAN_POINT('Ctrl Pts',(-1.35873721185581,2.11942482822684,11.9509911208822));
#17597=CARTESIAN_POINT('Ctrl Pts',(-1.34359166138221,2.12905845078916,11.9498768913881));
#17598=CARTESIAN_POINT('Ctrl Pts',(-1.28903641282525,2.16294535374278,11.9459107727317));
#17599=CARTESIAN_POINT('Ctrl Pts',(-1.24906136172821,2.18627390772019,11.943092297764));
#17600=CARTESIAN_POINT('Ctrl Pts',(-1.03619038619005,2.30275488909154,11.928490026143));
#17601=CARTESIAN_POINT('Ctrl Pts',(-0.853483432444309,2.37653967113284,
11.9173951817837));
#17602=CARTESIAN_POINT('Ctrl Pts',(-0.549542208086691,2.45965488016427,
11.8991886437835));
#17603=CARTESIAN_POINT('Ctrl Pts',(-0.432977306254001,2.48282542438193,
11.8922420461293));
#17604=CARTESIAN_POINT('Ctrl Pts',(-0.300339401330266,2.49956551554975,
11.883954204494));
#17605=CARTESIAN_POINT('Ctrl Pts',(-0.285432359299889,2.50131162899133,
11.8830172981414));
#17606=CARTESIAN_POINT('Ctrl Pts',(-0.262696777090993,2.50376884495363,
11.8815788692959));
#17607=CARTESIAN_POINT('Ctrl Pts',(-0.254878747263481,2.50457677979402,
11.8810825320049));
#17608=CARTESIAN_POINT('Ctrl Pts',(-0.240580866398312,2.50598672129961,
11.8801714830977));
#17609=CARTESIAN_POINT('Ctrl Pts',(-0.234102332032966,2.50660022660675,
11.8797574124748));
#17610=CARTESIAN_POINT('Ctrl Pts',(-0.219499358210026,2.50792599452817,
11.8788212279609));
#17611=CARTESIAN_POINT('Ctrl Pts',(-0.211373855558783,2.50862389588986,
11.8782983454335));
#17612=CARTESIAN_POINT('Ctrl Pts',(-0.190415326690593,2.51032148140501,
11.8769448352744));
#17613=CARTESIAN_POINT('Ctrl Pts',(-0.177577943914144,2.51126223125455,
11.8761111444935));
#17614=CARTESIAN_POINT('Ctrl Pts',(-0.0932844055489619,2.51678988008789,
11.8706088792076));
#17615=CARTESIAN_POINT('Ctrl Pts',(-0.0216737556048522,2.51842442015186,
11.865803100985));
#17616=CARTESIAN_POINT('Ctrl Pts',(0.210711685160005,2.51381718642206,11.8499739571947));
#17617=CARTESIAN_POINT('Ctrl Pts',(0.370847228036938,2.4952258230688,11.8387296494322));
#17618=CARTESIAN_POINT('Ctrl Pts',(0.605543147010275,2.44487096587333,11.8223839959206));
#17619=CARTESIAN_POINT('Ctrl Pts',(0.682144917858804,2.4246147732719,11.8170652946829));
#17620=CARTESIAN_POINT('Ctrl Pts',(0.790124429806865,2.39053713573412,11.8096113396093));
#17621=CARTESIAN_POINT('Ctrl Pts',(0.822368541463098,2.3796374880917,11.807390847196));
#17622=CARTESIAN_POINT('Ctrl Pts',(0.879654885388384,2.35896912522589,11.8034547681283));
#17623=CARTESIAN_POINT('Ctrl Pts',(0.90477991607114,2.34944705110204,11.8017315766919));
#17624=CARTESIAN_POINT('Ctrl Pts',(0.942841717193832,2.33432094043054,11.799125008086));
#17625=CARTESIAN_POINT('Ctrl Pts',(0.955891209509325,2.32900767824665,11.7982320454753));
#17626=CARTESIAN_POINT('Ctrl Pts',(0.978557491738719,2.31955622231094,11.7966820251234));
#17627=CARTESIAN_POINT('Ctrl Pts',(0.988194247505063,2.31546711650916,11.7960233413012));
#17628=CARTESIAN_POINT('Ctrl Pts',(1.00985878932688,2.30611444599358,11.7945431320623));
#17629=CARTESIAN_POINT('Ctrl Pts',(1.02187153075751,2.30081663706743,11.7937227850175));
#17630=CARTESIAN_POINT('Ctrl Pts',(1.05420796992306,2.28625254385818,11.791515287711));
#17631=CARTESIAN_POINT('Ctrl Pts',(1.07445098825068,2.27680922816071,11.7901341816849));
#17632=CARTESIAN_POINT('Ctrl Pts',(1.1719490907979,2.22973665045761,11.7834823499358));
#17633=CARTESIAN_POINT('Ctrl Pts',(1.2473732837918,2.18843605192168,11.7783394901813));
#17634=CARTESIAN_POINT('Ctrl Pts',(1.47325578203325,2.0492674530745,11.7627389764816));
#17635=CARTESIAN_POINT('Ctrl Pts',(1.6154678040361,1.93913398330687,11.7526594674976));
#17636=CARTESIAN_POINT('Ctrl Pts',(1.7879213438161,1.77333785295166,11.7386881385616));
#17637=CARTESIAN_POINT('Ctrl Pts',(1.82957964465381,1.73032576995872,11.735148398652));
#17638=CARTESIAN_POINT('Ctrl Pts',(1.88532101746347,1.66850761226299,11.7301071947024));
#17639=CARTESIAN_POINT('Ctrl Pts',(1.900736108857,1.65092554495815,11.7286782693222));
#17640=CARTESIAN_POINT('Ctrl Pts',(1.92720737005179,1.61987087061507,11.7261575781324));
#17641=CARTESIAN_POINT('Ctrl Pts',(1.93837289870792,1.60649318428139,11.7250727163868));
#17642=CARTESIAN_POINT('Ctrl Pts',(1.95467852464292,1.58653955128484,11.7234541977783));
#17643=CARTESIAN_POINT('Ctrl Pts',(1.95992650285732,1.58005189192766,11.7229278992065));
#17644=CARTESIAN_POINT('Ctrl Pts',(1.9688284828509,1.56893449215492,11.7220256883112));
#17645=CARTESIAN_POINT('Ctrl Pts',(1.97249861878599,1.56431781732018,11.7216509274027));
#17646=CARTESIAN_POINT('Ctrl Pts',(1.98077255356866,1.55383459544008,11.7207996534618));
#17647=CARTESIAN_POINT('Ctrl Pts',(1.98536643734936,1.54796058249875,11.7203224770519));
#17648=CARTESIAN_POINT('Ctrl Pts',(1.99776668440484,1.53195888810345,11.7190222725349));
#17649=CARTESIAN_POINT('Ctrl Pts',(2.00552196937138,1.52179215869184,11.7181958552676));
#17650=CARTESIAN_POINT('Ctrl Pts',(2.04383477821429,1.4707647702427,11.7140482184999));
#17651=CARTESIAN_POINT('Ctrl Pts',(2.07322046900851,1.42904362688158,11.7106578205151));
#17652=CARTESIAN_POINT('Ctrl Pts',(2.18455839123274,1.26030034281833,11.6970353900391));
#17653=CARTESIAN_POINT('Ctrl Pts',(2.25626729808039,1.12690223291128,11.6864831710867));
#17654=CARTESIAN_POINT('Ctrl Pts',(2.3318083941289,0.949835152145914,11.673258922542));
#17655=CARTESIAN_POINT('Ctrl Pts',(2.34709396730031,0.911408123072879,11.6704314740495));
#17656=CARTESIAN_POINT('Ctrl Pts',(2.36142193605295,0.872635485141376,11.6676249231292));
#17657=CARTESIAN_POINT('Origin',(0.,0.,10.));
#17658=CARTESIAN_POINT('',(2.3614219719961,0.872635387876314,10.6673175101421));
#17659=CARTESIAN_POINT('',(2.36142200728636,0.872635292378011,10.9438346412346));
#17660=CARTESIAN_POINT('',(2.36142200728636,0.87263529237802,10.));
#17661=CARTESIAN_POINT('',(2.51749968066629,-0.00126800833144993,11.8874166975493));
#17662=CARTESIAN_POINT('Ctrl Pts',(2.36142200728636,0.872635292378011,10.9438346412346));
#17663=CARTESIAN_POINT('Ctrl Pts',(2.33271572526319,0.95031682406596,10.9490804874489));
#17664=CARTESIAN_POINT('Ctrl Pts',(2.30013331963894,1.02668572932892,10.9543263336633));
#17665=CARTESIAN_POINT('Ctrl Pts',(2.26381902291199,1.10133086831425,10.9595721798777));
#17666=CARTESIAN_POINT('Ctrl Pts',(2.22754127086672,1.17590088859732,10.9648127469651));
#17667=CARTESIAN_POINT('Ctrl Pts',(2.1875392926656,1.24875017705897,10.9700533140526));
#17668=CARTESIAN_POINT('Ctrl Pts',(2.14400555146569,1.31948719026912,10.9752938811401));
#17669=CARTESIAN_POINT('Ctrl Pts',(2.10049529828321,1.39018603831924,10.9805316207533));
#17670=CARTESIAN_POINT('Ctrl Pts',(2.05345730675966,1.45877448166034,10.9857693603666));
#17671=CARTESIAN_POINT('Ctrl Pts',(2.00312957846779,1.52488627178143,10.9910070999799));
#17672=CARTESIAN_POINT('Ctrl Pts',(1.95281382251523,1.59098233473161,10.9962435936001));
#17673=CARTESIAN_POINT('Ctrl Pts',(1.89921016379548,1.65460254786909,11.0014800872204));
#17674=CARTESIAN_POINT('Ctrl Pts',(1.84259864664381,1.71541146008367,11.0067165808407));
#17675=CARTESIAN_POINT('Ctrl Pts',(1.78598352026102,1.77622424913162,11.0119534083103));
#17676=CARTESIAN_POINT('Ctrl Pts',(1.72636047011587,1.8342250446018,11.0171902357799));
#17677=CARTESIAN_POINT('Ctrl Pts',(1.66404741004881,1.88911420171197,11.0224270632495));
#17678=CARTESIAN_POINT('Ctrl Pts',(1.60167005533702,1.9440599934803,11.0276692940801));
#17679=CARTESIAN_POINT('Ctrl Pts',(1.53659749523301,1.99588743011063,11.0329115249107));
#17680=CARTESIAN_POINT('Ctrl Pts',(1.46918144404333,2.04433660009274,11.0381537557414));
#17681=CARTESIAN_POINT('Ctrl Pts',(1.40172945738266,2.09281159543413,11.0433987808922));
#17682=CARTESIAN_POINT('Ctrl Pts',(1.33193187978792,2.1379044875086,11.048643806043));
#17683=CARTESIAN_POINT('Ctrl Pts',(1.2601681220195,2.17939958572214,11.0538888311939));
#17684=CARTESIAN_POINT('Ctrl Pts',(1.18828032022182,2.22096640842917,11.059142922398));
#17685=CARTESIAN_POINT('Ctrl Pts',(1.11441996076285,2.258922804603,11.0643970136022));
#17686=CARTESIAN_POINT('Ctrl Pts',(1.03898945011338,2.29309990461669,11.0696511048063));
#17687=CARTESIAN_POINT('Ctrl Pts',(0.982025108734673,2.31891009701432,11.0736189401346));
#17688=CARTESIAN_POINT('Ctrl Pts',(0.924165769894775,2.34256589081392,11.0775867754629));
#17689=CARTESIAN_POINT('Ctrl Pts',(0.865590384616456,2.36401343821467,11.0815546107913));
#17690=CARTESIAN_POINT('Ctrl Pts',(0.788009478833835,2.39241991213302,11.0868098601986));
#17691=CARTESIAN_POINT('Ctrl Pts',(0.708885477546035,2.41705578739816,11.0920651096059));
#17692=CARTESIAN_POINT('Ctrl Pts',(0.628619422757704,2.43775385782317,11.0973203590132));
#17693=CARTESIAN_POINT('Ctrl Pts',(0.548467167000818,2.45842258308636,11.1025681576707));
#17694=CARTESIAN_POINT('Ctrl Pts',(0.467176516969301,2.47516447854801,11.1078159563282));
#17695=CARTESIAN_POINT('Ctrl Pts',(0.385166524084973,2.48786112930853,11.1130637549857));
#17696=CARTESIAN_POINT('Ctrl Pts',(0.302562298101252,2.5006497782496,11.1183495784686));
#17697=CARTESIAN_POINT('Ctrl Pts',(0.219228705756461,2.50933414962652,11.1236354019515));
#17698=CARTESIAN_POINT('Ctrl Pts',(0.135607525172923,2.51384503283645,11.1289212254344));
#17699=CARTESIAN_POINT('Ctrl Pts',(0.0527361699436561,2.51831546726799,
11.134159651303));
#17700=CARTESIAN_POINT('Ctrl Pts',(-0.0304171673727481,2.51868693520644,
11.1393980771716));
#17701=CARTESIAN_POINT('Ctrl Pts',(-0.113416093058638,2.51494394367654,
11.1446365030402));
#17702=CARTESIAN_POINT('Ctrl Pts',(-0.196387721779181,2.51120218315426,
11.1498732060777));
#17703=CARTESIAN_POINT('Ctrl Pts',(-0.279204579139248,2.50334867141901,
11.1551099091152));
#17704=CARTESIAN_POINT('Ctrl Pts',(-0.361431247096957,2.49142001750446,
11.1603466121527));
#17705=CARTESIAN_POINT('Ctrl Pts',(-0.443655675241373,2.47949168852048,
11.165583172545));
#17706=CARTESIAN_POINT('Ctrl Pts',(-0.525289489454989,2.46348850532878,
11.1708197329373));
#17707=CARTESIAN_POINT('Ctrl Pts',(-0.605904746066285,2.44349865739565,
11.1760562933297));
#17708=CARTESIAN_POINT('Ctrl Pts',(-0.687839457124779,2.42318162953576,
11.1813785621001));
#17709=CARTESIAN_POINT('Ctrl Pts',(-0.768721487248743,2.39874636322141,
11.1867008308706));
#17710=CARTESIAN_POINT('Ctrl Pts',(-0.848116588526167,2.37033847841753,
11.1920230996411));
#17711=CARTESIAN_POINT('Ctrl Pts',(-0.926345317708214,2.34234792621466,
11.1972671803914));
#17712=CARTESIAN_POINT('Ctrl Pts',(-1.00313010739058,2.31050093807348,11.2025112611417));
#17713=CARTESIAN_POINT('Ctrl Pts',(-1.07807656706871,2.27498509127804,11.2077553418921));
#17714=CARTESIAN_POINT('Ctrl Pts',(-1.15469917808144,2.23867494500185,11.2131167046726));
#17715=CARTESIAN_POINT('Ctrl Pts',(-1.22939978860919,2.19853009672522,11.2184780674532));
#17716=CARTESIAN_POINT('Ctrl Pts',(-1.30178609528692,2.15479911177763,11.2238394302337));
#17717=CARTESIAN_POINT('Ctrl Pts',(-1.37417240196464,2.11106812683003,11.2292007930143));
#17718=CARTESIAN_POINT('Ctrl Pts',(-1.44424402108168,2.06375134491811,11.2345621557948));
#17719=CARTESIAN_POINT('Ctrl Pts',(-1.51164419791891,2.0131413434973,11.2399235185753));
#17720=CARTESIAN_POINT('Ctrl Pts',(-1.57771037435095,1.96353302731782,11.2451787679827));
#17721=CARTESIAN_POINT('Ctrl Pts',(-1.6414539424788,1.91057746621052,11.25043401739));
#17722=CARTESIAN_POINT('Ctrl Pts',(-1.70251630309735,1.85452001544543,11.2556892667973));
#17723=CARTESIAN_POINT('Ctrl Pts',(-1.76349209116024,1.79854204141082,11.2609370654547));
#17724=CARTESIAN_POINT('Ctrl Pts',(-1.82179388522027,1.73947122242578,11.2661848641122));
#17725=CARTESIAN_POINT('Ctrl Pts',(-1.87709420657246,1.67759458441308,11.2714326627697));
#17726=CARTESIAN_POINT('Ctrl Pts',(-1.9327952264274,1.61526959681397,11.2767184862526));
#17727=CARTESIAN_POINT('Ctrl Pts',(-1.98545071457912,1.55009824201138,11.2820043097356));
#17728=CARTESIAN_POINT('Ctrl Pts',(-2.03476209091959,1.48241339826532,11.2872901332185));
#17729=CARTESIAN_POINT('Ctrl Pts',(-2.08363129555214,1.41533547984118,11.2925285590871));
#17730=CARTESIAN_POINT('Ctrl Pts',(-2.12921584430058,1.34578934831197,11.2977669849556));
#17731=CARTESIAN_POINT('Ctrl Pts',(-2.171265146536,1.27413261218682,11.3030054108242));
#17732=CARTESIAN_POINT('Ctrl Pts',(-2.21330061945572,1.20249944276962,11.3082421138617));
#17733=CARTESIAN_POINT('Ctrl Pts',(-2.2518029216706,1.12875744500906,11.3134788168993));
#17734=CARTESIAN_POINT('Ctrl Pts',(-2.28656569652305,1.05329177604502,11.3187155199368));
#17735=CARTESIAN_POINT('Ctrl Pts',(-2.32132752445488,0.977828162728087,
11.3239520803291));
#17736=CARTESIAN_POINT('Ctrl Pts',(-2.35234983543744,0.900641391085434,
11.3291886407214));
#17737=CARTESIAN_POINT('Ctrl Pts',(-2.37947360751471,0.82213843185982,11.3344252011138));
#17738=CARTESIAN_POINT('Ctrl Pts',(-2.40704132262709,0.742350590801221,
11.3397474698842));
#17739=CARTESIAN_POINT('Ctrl Pts',(-2.43058155731725,0.661203549034004,
11.3450697386547));
#17740=CARTESIAN_POINT('Ctrl Pts',(-2.44998002953474,0.579140833373839,
11.3503920074252));
#17741=CARTESIAN_POINT('Ctrl Pts',(-2.46909352401022,0.498283679015128,
11.3556360881755));
#17742=CARTESIAN_POINT('Ctrl Pts',(-2.4841861146577,0.416538047402362,11.3608801689259));
#17743=CARTESIAN_POINT('Ctrl Pts',(-2.49520041333004,0.334336876993229,
11.3661242496762));
#17744=CARTESIAN_POINT('Ctrl Pts',(-2.5064610429365,0.250297306183437,11.3714856124568));
#17745=CARTESIAN_POINT('Ctrl Pts',(-2.51345871792463,0.165782085062312,
11.3768469752373));
#17746=CARTESIAN_POINT('Ctrl Pts',(-2.51618834279567,0.081255606447549,
11.3822083380179));
#17747=CARTESIAN_POINT('Ctrl Pts',(-2.51891796766671,-0.00327087216720202,
11.3875697007985));
#17748=CARTESIAN_POINT('Ctrl Pts',(-2.51737961845211,-0.0878081014682281,
11.392931063579));
#17749=CARTESIAN_POINT('Ctrl Pts',(-2.51162447120054,-0.171897544097102,
11.3982924263596));
#17750=CARTESIAN_POINT('Ctrl Pts',(-2.50598323119857,-0.254322668384312,
11.4035476757669));
#17751=CARTESIAN_POINT('Ctrl Pts',(-2.4962698002576,-0.336622019470591,
11.4088029251742));
#17752=CARTESIAN_POINT('Ctrl Pts',(-2.4824947405883,-0.418361223049447,
11.4140581745815));
#17753=CARTESIAN_POINT('Ctrl Pts',(-2.46873921082429,-0.499984539006543,
11.419305973239));
#17754=CARTESIAN_POINT('Ctrl Pts',(-2.45093356636752,-0.581048833684736,
11.4245537718965));
#17755=CARTESIAN_POINT('Ctrl Pts',(-2.42914026605553,-0.661123148760993,
11.429801570554));
#17756=CARTESIAN_POINT('Ctrl Pts',(-2.40718905449474,-0.741777671282183,
11.4350873940369));
#17757=CARTESIAN_POINT('Ctrl Pts',(-2.38119218759287,-0.821427334373664,
11.4403732175198));
#17758=CARTESIAN_POINT('Ctrl Pts',(-2.35126631866039,-0.899640455255999,
11.4456590410027));
#17759=CARTESIAN_POINT('Ctrl Pts',(-2.32160879292897,-0.977152244482109,
11.4508974668713));
#17760=CARTESIAN_POINT('Ctrl Pts',(-2.28809261306326,-1.05325271217118,
11.4561358927399));
#17761=CARTESIAN_POINT('Ctrl Pts',(-2.25088130386272,-1.1275369643259,11.4613743186085));
#17762=CARTESIAN_POINT('Ctrl Pts',(-2.21368223284249,-1.20179678562636,
11.466611021646));
#17763=CARTESIAN_POINT('Ctrl Pts',(-2.17279065257139,-1.27424116548086,
11.4718477246835));
#17764=CARTESIAN_POINT('Ctrl Pts',(-2.1284172786826,-1.34448731411098,11.477084427721));
#17765=CARTESIAN_POINT('Ctrl Pts',(-2.08404511350235,-1.41473154927109,
11.4823209881133));
#17766=CARTESIAN_POINT('Ctrl Pts',(-2.03619159057178,-1.4827772827042,11.4875575485057));
#17767=CARTESIAN_POINT('Ctrl Pts',(-1.985111494058,-1.54826955216423,11.492794108898));
#17768=CARTESIAN_POINT('Ctrl Pts',(-1.93319535405385,-1.61483375353685,
11.4981163776685));
#17769=CARTESIAN_POINT('Ctrl Pts',(-1.87794635897837,-1.67875975435015,
11.503438646439));
#17770=CARTESIAN_POINT('Ctrl Pts',(-1.81967431466205,-1.73971021683474,
11.5087609152094));
#17771=CARTESIAN_POINT('Ctrl Pts',(-1.76225832928815,-1.79976527245543,
11.5140049959598));
#17772=CARTESIAN_POINT('Ctrl Pts',(-1.70190790868205,-1.85693135779365,
11.5192490767101));
#17773=CARTESIAN_POINT('Ctrl Pts',(-1.63895495321572,-1.9109246220952,11.5244931574604));
#17774=CARTESIAN_POINT('Ctrl Pts',(-1.57459407693794,-1.96612542685175,
11.529854520241));
#17775=CARTESIAN_POINT('Ctrl Pts',(-1.50751325655198,-2.01800946671689,
11.5352158830216));
#17776=CARTESIAN_POINT('Ctrl Pts',(-1.43809924691837,-2.06631962823103,
11.5405772458021));
#17777=CARTESIAN_POINT('Ctrl Pts',(-1.36868523728477,-2.11462978974516,
11.5459386085827));
#17778=CARTESIAN_POINT('Ctrl Pts',(-1.29693850490505,-2.15936586075083,
11.5512999713632));
#17779=CARTESIAN_POINT('Ctrl Pts',(-1.22327153025753,-2.20032111594226,
11.5566613341438));
#17780=CARTESIAN_POINT('Ctrl Pts',(-1.15106258997488,-2.24046577493673,
11.5619165835511));
#17781=CARTESIAN_POINT('Ctrl Pts',(-1.07674203656927,-2.2771262341722,11.5671718329584));
#17782=CARTESIAN_POINT('Ctrl Pts',(-1.00067997046994,-2.31007485738023,
11.5724270823657));
#17783=CARTESIAN_POINT('Ctrl Pts',(-0.924725743101172,-2.34297676692555,
11.5776748810232));
#17784=CARTESIAN_POINT('Ctrl Pts',(-0.847035327201545,-2.37217711150453,
11.5829226796807));
#17785=CARTESIAN_POINT('Ctrl Pts',(-0.768004213099251,-2.39749364517652,
11.5881704783382));
#17786=CARTESIAN_POINT('Ctrl Pts',(-0.68840045044239,-2.4229936189604,11.5934563018211));
#17787=CARTESIAN_POINT('Ctrl Pts',(-0.607436892756986,-2.44455303097054,
11.598742125304));
#17788=CARTESIAN_POINT('Ctrl Pts',(-0.525539144305069,-2.46203469874068,
11.6040279487869));
#17789=CARTESIAN_POINT('Ctrl Pts',(-0.444375767310484,-2.4793596096026,
11.6092663746555));
#17790=CARTESIAN_POINT('Ctrl Pts',(-0.362295345666159,-2.49267951493152,
11.6145048005241));
#17791=CARTESIAN_POINT('Ctrl Pts',(-0.279726532665681,-2.50191113289878,
11.6197432263927));
#17792=CARTESIAN_POINT('Ctrl Pts',(-0.197184875173657,-2.51113971474052,
11.6249799294302));
#17793=CARTESIAN_POINT('Ctrl Pts',(-0.114155603534914,-2.51628262838045,
11.6302166324677));
#17794=CARTESIAN_POINT('Ctrl Pts',(-0.0310745233178724,-2.51730820997362,
11.6354533355052));
#17795=CARTESIAN_POINT('Ctrl Pts',(0.0520042938120662,-2.51833376363045,
11.6406898958975));
#17796=CARTESIAN_POINT('Ctrl Pts',(0.135134455316132,-2.51524220356714,
11.6459264562899));
#17797=CARTESIAN_POINT('Ctrl Pts',(0.217879503963259,-2.50805398102846,
11.6511630166822));
#17798=CARTESIAN_POINT('Ctrl Pts',(0.30197886601233,-2.50074810666313,11.6564852854527));
#17799=CARTESIAN_POINT('Ctrl Pts',(0.385679903931784,-2.48921028676347,
11.6618075542231));
#17800=CARTESIAN_POINT('Ctrl Pts',(0.468530987135125,-2.47351671999487,
11.6671298229936));
#17801=CARTESIAN_POINT('Ctrl Pts',(0.550164927341342,-2.45805370319803,
11.672373903744));
#17802=CARTESIAN_POINT('Ctrl Pts',(0.630973279405442,-2.43855640038696,
11.6776179844943));
#17803=CARTESIAN_POINT('Ctrl Pts',(0.710537247829024,-2.41514866404691,
11.6828620652446));
#17804=CARTESIAN_POINT('Ctrl Pts',(0.791880636553999,-2.39121742187779,
11.6882234280252));
#17805=CARTESIAN_POINT('Ctrl Pts',(0.871922826291916,-2.36319889375187,
11.6935847908057));
#17806=CARTESIAN_POINT('Ctrl Pts',(0.950237582968915,-2.33127750083798,
11.6989461535863));
#17807=CARTESIAN_POINT('Ctrl Pts',(1.02855233964591,-2.2993561079241,11.7043075163668));
#17808=CARTESIAN_POINT('Ctrl Pts',(1.10513923131845,-2.26353212601067,11.7096688791474));
#17809=CARTESIAN_POINT('Ctrl Pts',(1.17960028275458,-2.22403898862527,11.7150302419279));
#17810=CARTESIAN_POINT('Ctrl Pts',(1.25258758326828,-2.18532750885186,11.7202854913353));
#17811=CARTESIAN_POINT('Ctrl Pts',(1.32380203496519,-2.14294784628386,11.7255407407426));
#17812=CARTESIAN_POINT('Ctrl Pts',(1.39285119654308,-2.09708650138436,11.7307959901499));
#17813=CARTESIAN_POINT('Ctrl Pts',(1.46180246209593,-2.0512901774535,11.7360437888074));
#17814=CARTESIAN_POINT('Ctrl Pts',(1.52859415406778,-2.00202222915312,11.7412915874649));
#17815=CARTESIAN_POINT('Ctrl Pts',(1.59285808064306,-1.94951516663249,11.7465393861223));
#17816=CARTESIAN_POINT('Ctrl Pts',(1.65758765476843,-1.89662764517746,11.7518252096052));
#17817=CARTESIAN_POINT('Ctrl Pts',(1.71975225860469,-1.84045409313397,11.7571110330882));
#17818=CARTESIAN_POINT('Ctrl Pts',(1.77900510365261,-1.78127681486566,11.7623968565711));
#17819=CARTESIAN_POINT('Ctrl Pts',(1.83772663252895,-1.72263017516685,11.7676352824396));
#17820=CARTESIAN_POINT('Ctrl Pts',(1.89358808005317,-1.66103379397625,11.7728737083082));
#17821=CARTESIAN_POINT('Ctrl Pts',(1.94628620911509,-1.59680187944793,11.7781121341768));
#17822=CARTESIAN_POINT('Ctrl Pts',(1.99896700663935,-1.53259108972735,11.7833488372143));
#17823=CARTESIAN_POINT('Ctrl Pts',(2.04848625947948,-1.465746844592,11.7885855402518));
#17824=CARTESIAN_POINT('Ctrl Pts',(2.09458013322459,-1.39661745496069,11.7938222432893));
#17825=CARTESIAN_POINT('Ctrl Pts',(2.14067275139564,-1.32748994837936,11.7990588036816));
#17826=CARTESIAN_POINT('Ctrl Pts',(2.18333992086565,-1.25607780554123,11.804295364074));
#17827=CARTESIAN_POINT('Ctrl Pts',(2.22236116616019,-1.18275825811665,11.8095319244663));
#17828=CARTESIAN_POINT('Ctrl Pts',(2.26202108405602,-1.10823866733811,11.8148541932368));
#17829=CARTESIAN_POINT('Ctrl Pts',(2.29791441049217,-1.0317490984141,11.8201764620073));
#17830=CARTESIAN_POINT('Ctrl Pts',(2.32985916934349,-0.953709862078643,
11.8254987307777));
#17831=CARTESIAN_POINT('Ctrl Pts',(2.36133463632767,-0.87681707919117,11.8307428115281));
#17832=CARTESIAN_POINT('Ctrl Pts',(2.38897668257414,-0.79842031994992,11.8359868922784));
#17833=CARTESIAN_POINT('Ctrl Pts',(2.41266118072916,-0.718938298466948,
11.8412309730287));
#17834=CARTESIAN_POINT('Ctrl Pts',(2.43687537439436,-0.637678689397213,
11.8465923358093));
#17835=CARTESIAN_POINT('Ctrl Pts',(2.45695274431194,-0.555285186779717,
11.8519536985898));
#17836=CARTESIAN_POINT('Ctrl Pts',(2.47281591772864,-0.472215720860557,
11.8573150613704));
#17837=CARTESIAN_POINT('Ctrl Pts',(2.48867909114535,-0.389146254941386,
11.8626764241509));
#17838=CARTESIAN_POINT('Ctrl Pts',(2.50032806421805,-0.305401338184903,
11.8680377869315));
#17839=CARTESIAN_POINT('Ctrl Pts',(2.5077419609525,-0.221441882393838,11.8733991497121));
#17840=CARTESIAN_POINT('Ctrl Pts',(2.51420329401791,-0.148269834375331,
11.878071665644));
#17841=CARTESIAN_POINT('Ctrl Pts',(2.51746263872295,-0.0748109262769095,
11.882744181576));
#17842=CARTESIAN_POINT('Ctrl Pts',(2.51749968066596,-0.00126800898217133,
11.887416697508));
#17843=CARTESIAN_POINT('Ctrl Pts',(2.51749968066629,-0.00126800833143484,
11.8874166975493));
#17844=CARTESIAN_POINT('Ctrl Pts',(2.51754083200788,0.080433733485191,11.8926075807009));
#17845=CARTESIAN_POINT('Ctrl Pts',(2.5136004923615,0.162294866749569,11.8977984638525));
#17846=CARTESIAN_POINT('Ctrl Pts',(2.50565840018274,0.243889793951418,11.9029893470041));
#17847=CARTESIAN_POINT('Ctrl Pts',(2.4977254437868,0.325390862568187,11.9081742590866));
#17848=CARTESIAN_POINT('Ctrl Pts',(2.48579990932845,0.406625865579958,11.9133591711691));
#17849=CARTESIAN_POINT('Ctrl Pts',(2.46991353201475,0.487168753483251,11.9185440832516));
#17850=CARTESIAN_POINT('Ctrl Pts',(2.45404174318634,0.567637678725842,11.9237242340212));
#17851=CARTESIAN_POINT('Ctrl Pts',(2.43421642376982,0.647415288567381,11.9289043847908));
#17852=CARTESIAN_POINT('Ctrl Pts',(2.41052097744956,0.726081859899853,11.9340845355604));
#17853=CARTESIAN_POINT('Ctrl Pts',(2.3956646756842,0.775403333180655,11.9373323276459));
#17854=CARTESIAN_POINT('Ctrl Pts',(2.37928809884128,0.824288196918462,11.9405801197315));
#17855=CARTESIAN_POINT('Ctrl Pts',(2.36142200728635,0.872635292378036,11.9438279118171));
#17856=CARTESIAN_POINT('Ctrl Pts',(2.36142193605295,0.872635485141379,11.6676249231292));
#17857=CARTESIAN_POINT('Ctrl Pts',(2.39733462200457,0.775452863264637,11.6605903752774));
#17858=CARTESIAN_POINT('Ctrl Pts',(2.42723136146153,0.676098638326863,11.653692497531));
#17859=CARTESIAN_POINT('Ctrl Pts',(2.45717869013096,0.548478592359361,11.6452161982623));
#17860=CARTESIAN_POINT('Ctrl Pts',(2.46299857004445,0.521722169439311,11.6434595024517));
#17861=CARTESIAN_POINT('Ctrl Pts',(2.47117118202385,0.480958117282357,11.6408130912722));
#17862=CARTESIAN_POINT('Ctrl Pts',(2.47384366205525,0.46701742000365,11.6399133359408));
#17863=CARTESIAN_POINT('Ctrl Pts',(2.47848523789497,0.441646550732813,11.6382852051423));
#17864=CARTESIAN_POINT('Ctrl Pts',(2.48049350670077,0.43022403548439,11.637555613152));
#17865=CARTESIAN_POINT('Ctrl Pts',(2.48466051193079,0.405523539298904,11.6359851326879));
#17866=CARTESIAN_POINT('Ctrl Pts',(2.48679190989915,0.392241263101315,11.6351451240798));
#17867=CARTESIAN_POINT('Ctrl Pts',(2.49230918754642,0.356004896870224,11.6328652520794));
#17868=CARTESIAN_POINT('Ctrl Pts',(2.49548442162297,0.33301971352108,11.6314319972977));
#17869=CARTESIAN_POINT('Ctrl Pts',(2.51117835423709,0.206536973781483,11.6236108013769));
#17870=CARTESIAN_POINT('Ctrl Pts',(2.51757761128408,0.102376427559413,11.6174167833035));
#17871=CARTESIAN_POINT('Ctrl Pts',(2.51741793553497,-0.110195921914664,
11.6050150424096));
#17872=CARTESIAN_POINT('Ctrl Pts',(2.51034757727641,-0.218384835402626,
11.5988290301993));
#17873=CARTESIAN_POINT('Ctrl Pts',(2.47987381666146,-0.451892398911848,
11.5852728567677));
#17874=CARTESIAN_POINT('Ctrl Pts',(2.45388512266596,-0.576559517709645,
11.5779033120999));
#17875=CARTESIAN_POINT('Ctrl Pts',(2.41264106487878,-0.719325857023597,
11.5687779373222));
#17876=CARTESIAN_POINT('Ctrl Pts',(2.40642315928923,-0.739860868354321,
11.5674481663356));
#17877=CARTESIAN_POINT('Ctrl Pts',(2.3973976420479,-0.768350097330235,11.5655760144903));
#17878=CARTESIAN_POINT('Ctrl Pts',(2.39481117317985,-0.776374114851892,
11.5650456829381));
#17879=CARTESIAN_POINT('Ctrl Pts',(2.39027949798047,-0.790194630478281,
11.5641267496927));
#17880=CARTESIAN_POINT('Ctrl Pts',(2.38835336851684,-0.795997372913695,
11.5637392446933));
#17881=CARTESIAN_POINT('Ctrl Pts',(2.38424507238018,-0.808225047074561,
11.5629190278164));
#17882=CARTESIAN_POINT('Ctrl Pts',(2.38205804528001,-0.814648241501571,
11.5624860244296));
#17883=CARTESIAN_POINT('Ctrl Pts',(2.37656669829816,-0.830564882332221,
11.5614078535492));
#17884=CARTESIAN_POINT('Ctrl Pts',(2.37323145959659,-0.840047454778009,
11.560760920611));
#17885=CARTESIAN_POINT('Ctrl Pts',(2.36043783596484,-0.875737263985224,
11.5583093432993));
#17886=CARTESIAN_POINT('Ctrl Pts',(2.35060177888145,-0.901805776198298,
11.5564845892203));
#17887=CARTESIAN_POINT('Ctrl Pts',(2.32422938779747,-0.968335856941044,
11.5517490492363));
#17888=CARTESIAN_POINT('Ctrl Pts',(2.30706862046077,-1.00853880933508,11.5488117769722));
#17889=CARTESIAN_POINT('Ctrl Pts',(2.23719436430341,-1.16110715123365,11.5374223580444));
#17890=CARTESIAN_POINT('Ctrl Pts',(2.17724603866038,-1.26996339033412,11.5287901057939));
#17891=CARTESIAN_POINT('Ctrl Pts',(2.02121642999805,-1.50952551202223,11.5091054489021));
#17892=CARTESIAN_POINT('Ctrl Pts',(1.92003972523376,-1.63629079817126,11.4981768932803));
#17893=CARTESIAN_POINT('Ctrl Pts',(1.79189727919847,-1.76844700605937,11.4863043246929));
#17894=CARTESIAN_POINT('Ctrl Pts',(1.77620740872702,-1.78420513546298,11.4848792754598));
#17895=CARTESIAN_POINT('Ctrl Pts',(1.75002419347935,-1.80981452017164,11.4825471305605));
#17896=CARTESIAN_POINT('Ctrl Pts',(1.73965175660351,-1.81978709054911,11.4816347860533));
#17897=CARTESIAN_POINT('Ctrl Pts',(1.72075658209769,-1.8376446386457,11.4799932226271));
#17898=CARTESIAN_POINT('Ctrl Pts',(1.7122637789379,-1.84556056291702,11.4792626900262));
#17899=CARTESIAN_POINT('Ctrl Pts',(1.6939217423108,-1.86242110709247,11.4777003369487));
#17900=CARTESIAN_POINT('Ctrl Pts',(1.68405571748575,-1.87134700160352,11.476869317981));
#17901=CARTESIAN_POINT('Ctrl Pts',(1.65683321967711,-1.89558582892479,11.4746014197013));
#17902=CARTESIAN_POINT('Ctrl Pts',(1.63933533477002,-1.91073851369584,11.4731711762786));
#17903=CARTESIAN_POINT('Ctrl Pts',(1.53480737469414,-1.99876380054203,11.4647823789306));
#17904=CARTESIAN_POINT('Ctrl Pts',(1.44313315820741,-2.06592877438447,11.4580577881623));
#17905=CARTESIAN_POINT('Ctrl Pts',(1.1965231600097,-2.22215329813713,11.4410757238237));
#17906=CARTESIAN_POINT('Ctrl Pts',(1.03610900383154,-2.30132636198947,11.4310638935683));
#17907=CARTESIAN_POINT('Ctrl Pts',(0.81113045191687,-2.38403736244201,11.4168612471783));
#17908=CARTESIAN_POINT('Ctrl Pts',(0.752824858510689,-2.40308555374831,
11.4131629968456));
#17909=CARTESIAN_POINT('Ctrl Pts',(0.680896920898376,-2.42370960772331,
11.408514393824));
#17910=CARTESIAN_POINT('Ctrl Pts',(0.667876892133936,-2.42732966809544,
11.407669521155));
#17911=CARTESIAN_POINT('Ctrl Pts',(0.647468050691093,-2.43282746694381,
11.4063389615243));
#17912=CARTESIAN_POINT('Ctrl Pts',(0.640098561790641,-2.4347768251201,11.4058572420002));
#17913=CARTESIAN_POINT('Ctrl Pts',(0.626402612903218,-2.43833316486429,
11.4049594453866));
#17914=CARTESIAN_POINT('Ctrl Pts',(0.620078646068015,-2.4399490416106,11.4045438789916));
#17915=CARTESIAN_POINT('Ctrl Pts',(0.605543715173644,-2.44360279735802,
11.4035864441435));
#17916=CARTESIAN_POINT('Ctrl Pts',(0.597328735560597,-2.44562388747316,
11.4030436467284));
#17917=CARTESIAN_POINT('Ctrl Pts',(0.571575479221172,-2.45182233543792,
11.4013371488221));
#17918=CARTESIAN_POINT('Ctrl Pts',(0.554002861577968,-2.45585261741511,
11.400165667376));
#17919=CARTESIAN_POINT('Ctrl Pts',(0.394372290485779,-2.49066349475816,
11.3894692705354));
#17920=CARTESIAN_POINT('Ctrl Pts',(0.249954017534687,-2.50927257987244,
11.3794176445737));
#17921=CARTESIAN_POINT('Ctrl Pts',(-0.0805325957285195,-2.52303614343129,
11.3565662917518));
#17922=CARTESIAN_POINT('Ctrl Pts',(-0.266136949880176,-2.51025724267252,
11.3438738372159));
#17923=CARTESIAN_POINT('Ctrl Pts',(-0.480685334711145,-2.47139757840306,
11.329711268035));
#17924=CARTESIAN_POINT('Ctrl Pts',(-0.512579264337335,-2.46498012993331,
11.3276175328131));
#17925=CARTESIAN_POINT('Ctrl Pts',(-0.559016808301207,-2.45469598871661,
11.3245847813435));
#17926=CARTESIAN_POINT('Ctrl Pts',(-0.573663345725554,-2.45131445774044,
11.3236305380125));
#17927=CARTESIAN_POINT('Ctrl Pts',(-0.599661484538509,-2.4450663382755,
11.3219405577085));
#17928=CARTESIAN_POINT('Ctrl Pts',(-0.611024919818703,-2.44225138948572,
11.3212032003458));
#17929=CARTESIAN_POINT('Ctrl Pts',(-0.634750652159168,-2.4361980950605,
11.3196662445311));
#17930=CARTESIAN_POINT('Ctrl Pts',(-0.647108784969866,-2.4329446723663,
11.3188671521334));
#17931=CARTESIAN_POINT('Ctrl Pts',(-0.679448917233236,-2.42416690688252,
11.3167795342191));
#17932=CARTESIAN_POINT('Ctrl Pts',(-0.699388645794815,-2.41848952559864,
11.3154959481257));
#17933=CARTESIAN_POINT('Ctrl Pts',(-0.792103332307921,-2.39084857161893,
11.3095413578145));
#17934=CARTESIAN_POINT('Ctrl Pts',(-0.863933568668204,-2.36584129036096,
11.3049694816425));
#17935=CARTESIAN_POINT('Ctrl Pts',(-1.05805885687285,-2.28823438307753,
11.2926070363392));
#17936=CARTESIAN_POINT('Ctrl Pts',(-1.17748619293803,-2.22913296196636,
11.2850029314329));
#17937=CARTESIAN_POINT('Ctrl Pts',(-1.40834098265433,-2.0911368230332,11.2695360682195));
#17938=CARTESIAN_POINT('Ctrl Pts',(-1.51914471610405,-2.01208043210366,
11.2616924757929));
#17939=CARTESIAN_POINT('Ctrl Pts',(-1.63938845857399,-1.91067280944356,
11.2520329516163));
#17940=CARTESIAN_POINT('Ctrl Pts',(-1.65558590818234,-1.89665503805232,
11.2507052973716));
#17941=CARTESIAN_POINT('Ctrl Pts',(-1.67790151135174,-1.87683876426748,
11.2488356608478));
#17942=CARTESIAN_POINT('Ctrl Pts',(-1.68417290717555,-1.87121320079613,
11.2483056857276));
#17943=CARTESIAN_POINT('Ctrl Pts',(-1.69494553626937,-1.8614519181657,11.2473872008259));
#17944=CARTESIAN_POINT('Ctrl Pts',(-1.69946020833582,-1.85733104559618,
11.2469997852196));
#17945=CARTESIAN_POINT('Ctrl Pts',(-1.70895589800082,-1.84860002514801,
11.2461795496073));
#17946=CARTESIAN_POINT('Ctrl Pts',(-1.71393333407742,-1.84398612717605,
11.2457464368011));
#17947=CARTESIAN_POINT('Ctrl Pts',(-1.72624217894296,-1.83248339593527,
11.2446676352453));
#17948=CARTESIAN_POINT('Ctrl Pts',(-1.73355100987166,-1.82557069015936,
11.2440201767197));
#17949=CARTESIAN_POINT('Ctrl Pts',(-1.76098721499923,-1.79930814723009,
11.2415642753773));
#17950=CARTESIAN_POINT('Ctrl Pts',(-1.78083282619967,-1.77966852873953,
11.2397356338672));
#17951=CARTESIAN_POINT('Ctrl Pts',(-1.83098620619575,-1.72835678738393,
11.2349875958374));
#17952=CARTESIAN_POINT('Ctrl Pts',(-1.86080008709392,-1.69621645878455,
11.232041549607));
#17953=CARTESIAN_POINT('Ctrl Pts',(-1.97166599481848,-1.57025740253802,
11.2206516318227));
#17954=CARTESIAN_POINT('Ctrl Pts',(-2.04658622852537,-1.47127795249396,
11.2120287854528));
#17955=CARTESIAN_POINT('Ctrl Pts',(-2.20173726091226,-1.23138706119628,
11.1923582977563));
#17956=CARTESIAN_POINT('Ctrl Pts',(-2.27628894104925,-1.08742203938476,
11.1814345814186));
#17957=CARTESIAN_POINT('Ctrl Pts',(-2.34479744928971,-0.916638196542017,
11.1695664337921));
#17958=CARTESIAN_POINT('Ctrl Pts',(-2.35280220109205,-0.89589202244469,
11.1681414005325));
#17959=CARTESIAN_POINT('Ctrl Pts',(-2.36553239402975,-0.861550791216074,
11.1658092762604));
#17960=CARTESIAN_POINT('Ctrl Pts',(-2.37041786212139,-0.848016772228323,
11.1648969365664));
#17961=CARTESIAN_POINT('Ctrl Pts',(-2.3790351887848,-0.82348807105769,11.1632553783208));
#17962=CARTESIAN_POINT('Ctrl Pts',(-2.38280749935209,-0.812508129783064,
11.1625248461243));
#17963=CARTESIAN_POINT('Ctrl Pts',(-2.39073944839949,-0.788890448991829,
11.1609624901581));
#17964=CARTESIAN_POINT('Ctrl Pts',(-2.39487514639262,-0.77624499652189,
11.160131467926));
#17965=CARTESIAN_POINT('Ctrl Pts',(-2.40593058696488,-0.741511951926544,
11.157863551125));
#17966=CARTESIAN_POINT('Ctrl Pts',(-2.41264638393,-0.719360441749694,11.1564332926306));
#17967=CARTESIAN_POINT('Ctrl Pts',(-2.45048890550599,-0.588043993508652,
11.1480441559588));
#17968=CARTESIAN_POINT('Ctrl Pts',(-2.47451096153681,-0.476960922333004,
11.1413192644936));
#17969=CARTESIAN_POINT('Ctrl Pts',(-2.51680047774478,-0.188057131813012,
11.1243341222338));
#17970=CARTESIAN_POINT('Ctrl Pts',(-2.52379800329334,-0.00925704089722142,
11.1143197143108));
#17971=CARTESIAN_POINT('Ctrl Pts',(-2.50772903572159,0.229904090897192,
11.1001166369944));
#17972=CARTESIAN_POINT('Ctrl Pts',(-2.50139100619104,0.290865149549083,
11.0964212088506));
#17973=CARTESIAN_POINT('Ctrl Pts',(-2.49094988651444,0.364907471250643,
11.0917757793895));
#17974=CARTESIAN_POINT('Ctrl Pts',(-2.48895565364245,0.37827045234536,11.0909310880515));
#17975=CARTESIAN_POINT('Ctrl Pts',(-2.48566829091056,0.399145960708781,
11.0896007531878));
#17976=CARTESIAN_POINT('Ctrl Pts',(-2.48444840247935,0.406669991729693,
11.0891190749371));
#17977=CARTESIAN_POINT('Ctrl Pts',(-2.48212046505666,0.420626740013686,
11.0882213136764));
#17978=CARTESIAN_POINT('Ctrl Pts',(-2.48102154900441,0.427060800681334,
11.0878057409841));
#17979=CARTESIAN_POINT('Ctrl Pts',(-2.47844071959789,0.441825121633087,
11.086848236874));
#17980=CARTESIAN_POINT('Ctrl Pts',(-2.47694182798876,0.450152212577691,
11.0863053759864));
#17981=CARTESIAN_POINT('Ctrl Pts',(-2.47211676075218,0.476203947033921,
11.0845984807209));
#17982=CARTESIAN_POINT('Ctrl Pts',(-2.4686421711388,0.493900055581935,11.0834266603707));
#17983=CARTESIAN_POINT('Ctrl Pts',(-2.43459210165735,0.657973106557688,
11.0724560828398));
#17984=CARTESIAN_POINT('Ctrl Pts',(-2.39122432622761,0.801376946139549,
11.0621010601758));
#17985=CARTESIAN_POINT('Ctrl Pts',(-2.26783491396871,1.10791068269773,11.0392753885434));
#17986=CARTESIAN_POINT('Ctrl Pts',(-2.18236567500239,1.26800756912656,11.0269078797221));
#17987=CARTESIAN_POINT('Ctrl Pts',(-2.06224972480371,1.4442913120166,11.0130495986418));
#17988=CARTESIAN_POINT('Ctrl Pts',(-2.04353289230858,1.47065454750975,11.0109683170281));
#17989=CARTESIAN_POINT('Ctrl Pts',(-2.01526406930795,1.50888987314861,11.007935401561));
#17990=CARTESIAN_POINT('Ctrl Pts',(-2.0061044420944,1.5210466469932,11.006968890362));
#17991=CARTESIAN_POINT('Ctrl Pts',(-1.98968887780072,1.5424273454487,11.0052648430355));
#17992=CARTESIAN_POINT('Ctrl Pts',(-1.98247771263297,1.55168491417507,11.0045255930391));
#17993=CARTESIAN_POINT('Ctrl Pts',(-1.9673339409232,1.57084832248744,11.0029921847298));
#17994=CARTESIAN_POINT('Ctrl Pts',(-1.95939061750972,1.58074530041335,11.0021984785472));
#17995=CARTESIAN_POINT('Ctrl Pts',(-1.93853216285496,1.6063350657589,11.0001413023145));
#17996=CARTESIAN_POINT('Ctrl Pts',(-1.92550107584605,1.62193246909921,10.998882505291));
#17997=CARTESIAN_POINT('Ctrl Pts',(-1.86582361245943,1.69162966811375,10.9932325047161));
#17998=CARTESIAN_POINT('Ctrl Pts',(-1.81707406750394,1.74388987759326,10.98892805379));
#17999=CARTESIAN_POINT('Ctrl Pts',(-1.59931214699988,1.95827182051405,10.9708135544456));
#18000=CARTESIAN_POINT('Ctrl Pts',(-1.41038339110225,2.09843488773873,10.9578827249366));
#18001=CARTESIAN_POINT('Ctrl Pts',(-1.15736137022779,2.23634607259549,10.9407222320724));
#18002=CARTESIAN_POINT('Ctrl Pts',(-1.10907399511331,2.26068198556832,10.9374478455764));
#18003=CARTESIAN_POINT('Ctrl Pts',(-1.04822098560862,2.28893183547811,10.933276444192));
#18004=CARTESIAN_POINT('Ctrl Pts',(-1.03635498831175,2.29432876968182,10.9324609656707));
#18005=CARTESIAN_POINT('Ctrl Pts',(-1.0175840439003,2.30269090978864,10.9311668635687));
#18006=CARTESIAN_POINT('Ctrl Pts',(-1.01070662764098,2.30571785389678,10.9306918635515));
#18007=CARTESIAN_POINT('Ctrl Pts',(-0.998416234301015,2.31106164802894,
10.9298413003156));
#18008=CARTESIAN_POINT('Ctrl Pts',(-0.993008552306173,2.31339035410235,
10.9294664598037));
#18009=CARTESIAN_POINT('Ctrl Pts',(-0.979995838311128,2.31893997709558,
10.9285630565051));
#18010=CARTESIAN_POINT('Ctrl Pts',(-0.972383134094452,2.32214243671705,
10.9280334079455));
#18011=CARTESIAN_POINT('Ctrl Pts',(-0.949066919331147,2.33181618311478,
10.9264080287004));
#18012=CARTESIAN_POINT('Ctrl Pts',(-0.93331392864005,2.33816590575514,10.925305507615));
#18013=CARTESIAN_POINT('Ctrl Pts',(-0.896431707738855,2.35260031146914,
10.9227160173604));
#18014=CARTESIAN_POINT('Ctrl Pts',(-0.875255593514787,2.36056044247229,
10.9212230562769));
#18015=CARTESIAN_POINT('Ctrl Pts',(-0.800407435936451,2.3875503964935,10.9159312862508));
#18016=CARTESIAN_POINT('Ctrl Pts',(-0.746202203458642,2.40504270691928,
10.9120727230693));
#18017=CARTESIAN_POINT('Ctrl Pts',(-0.530005995903139,2.46679796291472,
10.8966922480688));
#18018=CARTESIAN_POINT('Ctrl Pts',(-0.364333165218001,2.49665110955337,
10.8849616127632));
#18019=CARTESIAN_POINT('Ctrl Pts',(-0.0971860332738022,2.51761187361939,
10.866838087092));
#18020=CARTESIAN_POINT('Ctrl Pts',(0.0029367541128548,2.51948614030987,
10.8602112423803));
#18021=CARTESIAN_POINT('Ctrl Pts',(0.125871810457664,2.51445627167282,10.8522872724182));
#18022=CARTESIAN_POINT('Ctrl Pts',(0.148813271983063,2.51320288119465,10.8508173992024));
#18023=CARTESIAN_POINT('Ctrl Pts',(0.185103973421996,2.51072147680859,10.8485056218221));
#18024=CARTESIAN_POINT('Ctrl Pts',(0.198465641319012,2.50970062270158,10.8476573374664));
#18025=CARTESIAN_POINT('Ctrl Pts',(0.223378689272948,2.50759701636848,10.8460808623983));
#18026=CARTESIAN_POINT('Ctrl Pts',(0.234931911116423,2.50654101097681,10.8453518607697));
#18027=CARTESIAN_POINT('Ctrl Pts',(0.260668769256758,2.50400906183424,10.8437323230351));
#18028=CARTESIAN_POINT('Ctrl Pts',(0.274848067041515,2.50249238605967,10.8428430794495));
#18029=CARTESIAN_POINT('Ctrl Pts',(0.316533743979677,2.49767493737318,10.8402371409028));
#18030=CARTESIAN_POINT('Ctrl Pts',(0.343999959172452,2.49404046174496,10.8385308553767));
#18031=CARTESIAN_POINT('Ctrl Pts',(0.541732976115757,2.46454660348116,10.8263130586518));
#18032=CARTESIAN_POINT('Ctrl Pts',(0.70901385228238,2.42172946050181,10.8163732311916));
#18033=CARTESIAN_POINT('Ctrl Pts',(1.02260130307539,2.30614951468294,10.7971682262028));
#18034=CARTESIAN_POINT('Ctrl Pts',(1.16879242719175,2.23560930750595,10.787928182996));
#18035=CARTESIAN_POINT('Ctrl Pts',(1.32462344639371,2.1409333916849,10.7767165001997));
#18036=CARTESIAN_POINT('Ctrl Pts',(1.34194134790884,2.13012122190247,10.7754499427391));
#18037=CARTESIAN_POINT('Ctrl Pts',(1.36668613976552,2.11425067801649,10.7736074856101));
#18038=CARTESIAN_POINT('Ctrl Pts',(1.37422094001165,2.10936097820178,10.773042021912));
#18039=CARTESIAN_POINT('Ctrl Pts',(1.3871751458298,2.10085549422045,10.7720618764836));
#18040=CARTESIAN_POINT('Ctrl Pts',(1.39260706592421,2.09725874701013,10.7716484427858));
#18041=CARTESIAN_POINT('Ctrl Pts',(1.39826045702336,2.09348370533714,10.7712155386713));
#18042=CARTESIAN_POINT('Ctrl Pts',(1.39849592741285,2.09332641296019,10.7711975029857));
#18043=CARTESIAN_POINT('Ctrl Pts',(1.3989147409203,2.09304654660976,10.7711654158756));
#18044=CARTESIAN_POINT('Ctrl Pts',(1.39909809453178,2.09292398823192,10.771151365503));
#18045=CARTESIAN_POINT('Ctrl Pts',(1.39940806169558,2.0927167390894,10.7711276079094));
#18046=CARTESIAN_POINT('Ctrl Pts',(1.39953468372102,2.09263206089017,10.7711179015345));
#18047=CARTESIAN_POINT('Ctrl Pts',(1.39975277896695,2.09248618152838,10.7711011808126));
#18048=CARTESIAN_POINT('Ctrl Pts',(1.39984425588037,2.09242498584577,10.7710941668344));
#18049=CARTESIAN_POINT('Ctrl Pts',(1.40005856813296,2.09228159616287,10.771077732808));
#18050=CARTESIAN_POINT('Ctrl Pts',(1.40018140022948,2.09219939735575,10.7710683124367));
#18051=CARTESIAN_POINT('Ctrl Pts',(1.40042015178547,2.09203959521152,10.7710499993511));
#18052=CARTESIAN_POINT('Ctrl Pts',(1.4005360720393,2.09196199305253,10.7710411067161));
#18053=CARTESIAN_POINT('Ctrl Pts',(1.4007619906409,2.09181072592668,10.7710237735085));
#18054=CARTESIAN_POINT('Ctrl Pts',(1.40087198962762,2.09173706191837,10.7710153330003));
#18055=CARTESIAN_POINT('Ctrl Pts',(1.40108687499705,2.09159313315217,10.7709988422774));
#18056=CARTESIAN_POINT('Ctrl Pts',(1.40119176190284,2.09152286918262,10.7709907921157));
#18057=CARTESIAN_POINT('Ctrl Pts',(1.40139709362752,2.09138529462943,10.7709750308952));
#18058=CARTESIAN_POINT('Ctrl Pts',(1.40149753890377,2.09131798468491,10.7709673198786));
#18059=CARTESIAN_POINT('Ctrl Pts',(1.40169455003112,2.0911859438912,10.77095219398));
#18060=CARTESIAN_POINT('Ctrl Pts',(1.4017911162457,2.09112121359085,10.7709447791348));
#18061=CARTESIAN_POINT('Ctrl Pts',(1.40198084665936,2.09099401438221,10.7709302091109));
#18062=CARTESIAN_POINT('Ctrl Pts',(1.40207401116765,2.09093154593597,10.7709230539632));
#18063=CARTESIAN_POINT('Ctrl Pts',(1.40225734739891,2.09080859799612,10.7709089720652));
#18064=CARTESIAN_POINT('Ctrl Pts',(1.40234751939106,2.09074811889104,10.7709020453409));
#18065=CARTESIAN_POINT('Ctrl Pts',(1.40252522467712,2.09062891380924,10.7708883932264));
#18066=CARTESIAN_POINT('Ctrl Pts',(1.40261275819615,2.09057018816786,10.7708816678587));
#18067=CARTESIAN_POINT('Ctrl Pts',(1.40278549554194,2.09045428412731,10.7708683948329));
#18068=CARTESIAN_POINT('Ctrl Pts',(1.40287069955756,2.09039710601884,10.7708618471943));
#18069=CARTESIAN_POINT('Ctrl Pts',(1.40303904969481,2.09028411587032,10.77084890884));
#18070=CARTESIAN_POINT('Ctrl Pts',(1.40312219598932,2.09022830407359,10.7708425181405));
#18071=CARTESIAN_POINT('Ctrl Pts',(1.40328667162243,2.09011788587227,10.770829875232));
#18072=CARTESIAN_POINT('Ctrl Pts',(1.40336800109619,2.09006327968691,10.7708236230379));
#18073=CARTESIAN_POINT('Ctrl Pts',(1.40352905813526,2.08995512922967,10.7708112406832));
#18074=CARTESIAN_POINT('Ctrl Pts',(1.40360878582183,2.08990158514396,10.7708051105351));
#18075=CARTESIAN_POINT('Ctrl Pts',(1.40376683255596,2.08979542987289,10.7707929574762));
#18076=CARTESIAN_POINT('Ctrl Pts',(1.40384515171288,2.08974281884495,10.7707869345759));
#18077=CARTESIAN_POINT('Ctrl Pts',(1.4040005562267,2.08963841291741,10.7707749826228));
#18078=CARTESIAN_POINT('Ctrl Pts',(1.40407764167998,2.08958661815184,10.7707690535787));
#18079=CARTESIAN_POINT('Ctrl Pts',(1.4042307379417,2.08948373839258,10.7707572771445));
#18080=CARTESIAN_POINT('Ctrl Pts',(1.40430674883701,2.08943265351103,10.7707514297614));
#18081=CARTESIAN_POINT('Ctrl Pts',(1.40445784177767,2.08933109603385,10.7707398054744));
#18082=CARTESIAN_POINT('Ctrl Pts',(1.40453292388654,2.08928062354092,10.7707340285773));
#18083=CARTESIAN_POINT('Ctrl Pts',(1.40468229360237,2.08918020095291,10.7707225349601));
#18084=CARTESIAN_POINT('Ctrl Pts',(1.40475658125238,2.08913025095176,10.7707168182468));
#18085=CARTESIAN_POINT('Ctrl Pts',(1.40490448650718,2.08903079002271,10.7707054354491));
#18086=CARTESIAN_POINT('Ctrl Pts',(1.40497810417176,2.0889812791571,10.7706997693685));
#18087=CARTESIAN_POINT('Ctrl Pts',(1.40512478550771,2.08888261874761,10.7706884789288));
#18088=CARTESIAN_POINT('Ctrl Pts',(1.40519784922212,2.08883346925874,10.7706828545733));
#18089=CARTESIAN_POINT('Ctrl Pts',(1.40534353145249,2.08873545866046,10.7706716392288));
#18090=CARTESIAN_POINT('Ctrl Pts',(1.40541614999251,2.08868659760173,10.7706660482435));
#18091=CARTESIAN_POINT('Ctrl Pts',(1.40556104440565,2.08858909506851,10.7706548917615));
#18092=CARTESIAN_POINT('Ctrl Pts',(1.40563332029845,2.08854045363181,10.7706493262674));
#18093=CARTESIAN_POINT('Ctrl Pts',(1.40577762657922,2.08844332509855,10.7706382132981));
#18094=CARTESIAN_POINT('Ctrl Pts',(1.40584965698744,2.08839483802457,10.7706326658242));
#18095=CARTESIAN_POINT('Ctrl Pts',(1.40599356487939,2.08829795599818,10.7706215817738));
#18096=CARTESIAN_POINT('Ctrl Pts',(1.40606544237672,2.08824956105883,10.7706160451979));
#18097=CARTESIAN_POINT('Ctrl Pts',(1.41311305219985,2.08350389414276,10.7700731392783));
#18098=CARTESIAN_POINT('Ctrl Pts',(1.42006508721248,2.07877178123098,10.7695334630535));
#18099=CARTESIAN_POINT('Ctrl Pts',(1.44210436950111,2.06360792915573,10.7678097296066));
#18100=CARTESIAN_POINT('Ctrl Pts',(1.45710098439732,2.05304636405247,10.7666175248755));
#18101=CARTESIAN_POINT('Ctrl Pts',(1.59466926886422,1.95389560105135,10.7555112935215));
#18102=CARTESIAN_POINT('Ctrl Pts',(1.70912892953977,1.85460180676072,10.7450314383921));
#18103=CARTESIAN_POINT('Ctrl Pts',(1.93782765136039,1.61695171134747,10.7222502874169));
#18104=CARTESIAN_POINT('Ctrl Pts',(2.0476515188536,1.47541627528143,10.7100490039289));
#18105=CARTESIAN_POINT('Ctrl Pts',(2.15712861659806,1.29825940628082,10.6965184917753));
#18106=CARTESIAN_POINT('Ctrl Pts',(2.17223541240657,1.27282158573549,10.6946123108767));
#18107=CARTESIAN_POINT('Ctrl Pts',(2.19425209414119,1.23421424707339,10.6917727875705));
#18108=CARTESIAN_POINT('Ctrl Pts',(2.20149899958331,1.22124085691834,10.6908274979365));
#18109=CARTESIAN_POINT('Ctrl Pts',(2.21387391582671,1.19861916037615,10.6891943154352));
#18110=CARTESIAN_POINT('Ctrl Pts',(2.21905470931688,1.1890003406038,10.6885045666132));
#18111=CARTESIAN_POINT('Ctrl Pts',(2.22972998983283,1.16886746299885,10.6870704807308));
#18112=CARTESIAN_POINT('Ctrl Pts',(2.23521311664045,1.15834766134119,10.6863265561475));
#18113=CARTESIAN_POINT('Ctrl Pts',(2.24804292293344,1.13330234869151,10.684568005527));
#18114=CARTESIAN_POINT('Ctrl Pts',(2.2553235457549,1.11874345602014,10.683555697073));
#18115=CARTESIAN_POINT('Ctrl Pts',(2.27945219422264,1.06930098011352,10.6801503480015));
#18116=CARTESIAN_POINT('Ctrl Pts',(2.29563663540643,1.03409843624873,10.6777800458454));
#18117=CARTESIAN_POINT('Ctrl Pts',(2.32894184405087,0.957017070062897,10.6726957809908));
#18118=CARTESIAN_POINT('Ctrl Pts',(2.34575361275732,0.915035235837583,10.6699926192476));
#18119=CARTESIAN_POINT('Ctrl Pts',(2.3614219719961,0.872635387876314,10.6673175101421));
#18120=CARTESIAN_POINT('Origin',(0.,0.,10.));
#18121=CARTESIAN_POINT('',(2.36142200350084,0.872635302621937,9.67114329893353));
#18122=CARTESIAN_POINT('',(2.36142200728636,0.872635292378023,9.94365014611287));
#18123=CARTESIAN_POINT('',(2.36142200728636,0.87263529237802,10.));
#18124=CARTESIAN_POINT('',(2.51749898433573,0.00226138642591275,10.8874166974549));
#18125=CARTESIAN_POINT('Ctrl Pts',(2.36142200728636,0.872635292378024,9.94365014611287));
#18126=CARTESIAN_POINT('Ctrl Pts',(2.33166846731732,0.953150789162594,9.94908273018793));
#18127=CARTESIAN_POINT('Ctrl Pts',(2.29783002319381,1.0320428527644,9.95451531426299));
#18128=CARTESIAN_POINT('Ctrl Pts',(2.26012095724572,1.10890013464634,9.95994789833805));
#18129=CARTESIAN_POINT('Ctrl Pts',(2.22998573573739,1.17032067519298,9.96428935099269));
#18130=CARTESIAN_POINT('Ctrl Pts',(2.19737952459186,1.23044212633847,9.96863080364734));
#18131=CARTESIAN_POINT('Ctrl Pts',(2.1624315142936,1.28906795631179,9.97297225630198));
#18132=CARTESIAN_POINT('Ctrl Pts',(2.12012758401584,1.36003345627881,9.97822750570929));
#18133=CARTESIAN_POINT('Ctrl Pts',(2.07424846759199,1.42904534370428,9.98348275511659));
#18134=CARTESIAN_POINT('Ctrl Pts',(2.02500000847369,1.49572096852373,9.98873800452389));
#18135=CARTESIAN_POINT('Ctrl Pts',(1.97582137248252,1.56230206245406,9.99398580318139));
#18136=CARTESIAN_POINT('Ctrl Pts',(1.92328315409526,1.626553104896,9.99923360183888));
#18137=CARTESIAN_POINT('Ctrl Pts',(1.8676359396016,1.68811796006928,10.0044814004964));
#18138=CARTESIAN_POINT('Ctrl Pts',(1.81158551306532,1.75012890569351,10.0097672239793));
#18139=CARTESIAN_POINT('Ctrl Pts',(1.75238108825255,1.80941416526022,10.0150530474622));
#18140=CARTESIAN_POINT('Ctrl Pts',(1.69032191607646,1.86564146341992,10.0203388709451));
#18141=CARTESIAN_POINT('Ctrl Pts',(1.62881922421362,1.92136457527812,10.0255772968137));
#18142=CARTESIAN_POINT('Ctrl Pts',(1.56451312482682,1.97408403161953,10.0308157226823));
#18143=CARTESIAN_POINT('Ctrl Pts',(1.49773256054321,2.02351264564585,10.0360541485509));
#18144=CARTESIAN_POINT('Ctrl Pts',(1.43097395927577,2.07292500342366,10.0412908515884));
#18145=CARTESIAN_POINT('Ctrl Pts',(1.36174287997103,2.11904839410426,10.0465275546259));
#18146=CARTESIAN_POINT('Ctrl Pts',(1.29040036014567,2.16163668560097,10.0517642576634));
#18147=CARTESIAN_POINT('Ctrl Pts',(1.21905978365487,2.20422381701391,10.0570008180557));
#18148=CARTESIAN_POINT('Ctrl Pts',(1.1456082777219,2.24327580507479,10.0622373784481));
#18149=CARTESIAN_POINT('Ctrl Pts',(1.07043360185148,2.27859126523983,10.0674739388404));
#18150=CARTESIAN_POINT('Ctrl Pts',(0.994028519175117,2.31448474429274,10.0727962076109));
#18151=CARTESIAN_POINT('Ctrl Pts',(0.915843789831386,2.34651805717603,10.0781184763814));
#18152=CARTESIAN_POINT('Ctrl Pts',(0.836308278399151,2.37453041957374,10.0834407451518));
#18153=CARTESIAN_POINT('Ctrl Pts',(0.757941201790199,2.40213125988379,10.0886848259022));
#18154=CARTESIAN_POINT('Ctrl Pts',(0.678263233698535,2.42582843231022,10.0939289066525));
#18155=CARTESIAN_POINT('Ctrl Pts',(0.597698758546328,2.44551884965792,10.0991729874028));
#18156=CARTESIAN_POINT('Ctrl Pts',(0.515332487110007,2.4656496362967,10.1045343501834));
#18157=CARTESIAN_POINT('Ctrl Pts',(0.432040080192264,2.48159218961263,10.1098957129639));
#18158=CARTESIAN_POINT('Ctrl Pts',(0.348282757392841,2.49329207492882,10.1152570757445));
#18159=CARTESIAN_POINT('Ctrl Pts',(0.264525434593406,2.504991960245,10.1206184385251));
#18160=CARTESIAN_POINT('Ctrl Pts',(0.180303707930422,2.51244919928504,10.1259798013056));
#18161=CARTESIAN_POINT('Ctrl Pts',(0.0960789567655814,2.51566593252499,
10.1313411640862));
#18162=CARTESIAN_POINT('Ctrl Pts',(0.0135212020012339,2.51881899941202,
10.1365964134935));
#18163=CARTESIAN_POINT('Ctrl Pts',(-0.0693443933132752,2.51790958034371,
10.1418516629008));
#18164=CARTESIAN_POINT('Ctrl Pts',(-0.152084793467355,2.5129020007943,10.1471069123081));
#18165=CARTESIAN_POINT('Ctrl Pts',(-0.234707886530317,2.50790152085511,
10.1523547109656));
#18166=CARTESIAN_POINT('Ctrl Pts',(-0.317205680260735,2.49881444895049,
10.1576025096231));
#18167=CARTESIAN_POINT('Ctrl Pts',(-0.399143018617033,2.48565707624549,
10.1628503082806));
#18168=CARTESIAN_POINT('Ctrl Pts',(-0.481674063628092,2.47240436703224,
10.1681361317635));
#18169=CARTESIAN_POINT('Ctrl Pts',(-0.563636023487413,2.45502210436827,
10.1734219552464));
#18170=CARTESIAN_POINT('Ctrl Pts',(-0.64458726056848,2.43358038977816,10.1787077787293));
#18171=CARTESIAN_POINT('Ctrl Pts',(-0.724812613494356,2.41233094156275,
10.1839462045979));
#18172=CARTESIAN_POINT('Ctrl Pts',(-0.804044842948055,2.38709467180907,
10.1891846304665));
#18173=CARTESIAN_POINT('Ctrl Pts',(-0.881863965531894,2.35799113575441,
10.1944230563351));
#18174=CARTESIAN_POINT('Ctrl Pts',(-0.959657494701511,2.32889717136837,
10.1996597593726));
#18175=CARTESIAN_POINT('Ctrl Pts',(-1.03603840817081,2.29593862820907,10.2048964624101));
#18176=CARTESIAN_POINT('Ctrl Pts',(-1.11060368480479,2.25928433476135,10.2101331654476));
#18177=CARTESIAN_POINT('Ctrl Pts',(-1.18516693031777,2.22263103975832,10.21536972584));
#18178=CARTESIAN_POINT('Ctrl Pts',(-1.25791422369005,2.18228239910813,10.2206062862323));
#18179=CARTESIAN_POINT('Ctrl Pts',(-1.32846552885232,2.13845401836259,10.2258428466246));
#18180=CARTESIAN_POINT('Ctrl Pts',(-1.4001715687047,2.09390828516636,10.2311651153951));
#18181=CARTESIAN_POINT('Ctrl Pts',(-1.46960866236063,2.04576812457827,10.2364873841656));
#18182=CARTESIAN_POINT('Ctrl Pts',(-1.53640844918686,1.99430572562665,10.2418096529361));
#18183=CARTESIAN_POINT('Ctrl Pts',(-1.60222689829722,1.94359934694754,10.2470537336864));
#18184=CARTESIAN_POINT('Ctrl Pts',(-1.66548469781701,1.88966804453302,10.2522978144367));
#18185=CARTESIAN_POINT('Ctrl Pts',(-1.72586432224112,1.83281166277804,10.257541895187));
#18186=CARTESIAN_POINT('Ctrl Pts',(-1.78759431582885,1.77468370794838,10.2629032579676));
#18187=CARTESIAN_POINT('Ctrl Pts',(-1.84631548752542,1.71349862765125,10.2682646207481));
#18188=CARTESIAN_POINT('Ctrl Pts',(-1.90173106621274,1.64961365228388,10.2736259835287));
#18189=CARTESIAN_POINT('Ctrl Pts',(-1.95714664490007,1.5857286769165,10.2789873463093));
#18190=CARTESIAN_POINT('Ctrl Pts',(-2.00925637003065,1.51914424778319,10.2843487090898));
#18191=CARTESIAN_POINT('Ctrl Pts',(-2.05781083830561,1.4502485317186,10.2897100718704));
#18192=CARTESIAN_POINT('Ctrl Pts',(-2.10540430494241,1.38271641612896,10.2949653212777));
#18193=CARTESIAN_POINT('Ctrl Pts',(-2.14975779396929,1.31271425944068,10.300220570685));
#18194=CARTESIAN_POINT('Ctrl Pts',(-2.19060561490065,1.24058586561581,10.3054758200923));
#18195=CARTESIAN_POINT('Ctrl Pts',(-2.23139552290147,1.16855973346774,10.3107236187498));
#18196=CARTESIAN_POINT('Ctrl Pts',(-2.26868940967179,1.09441375005823,10.3159714174073));
#18197=CARTESIAN_POINT('Ctrl Pts',(-2.30226401872903,1.01852179066805,10.3212192160648));
#18198=CARTESIAN_POINT('Ctrl Pts',(-2.33608190477361,0.942079928605546,
10.3265050395477));
#18199=CARTESIAN_POINT('Ctrl Pts',(-2.36612611394324,0.863867068955288,
10.3317908630306));
#18200=CARTESIAN_POINT('Ctrl Pts',(-2.39221499656075,0.784291820835746,
10.3370766865135));
#18201=CARTESIAN_POINT('Ctrl Pts',(-2.41806994196864,0.705430118473343,
10.3423151123821));
#18202=CARTESIAN_POINT('Ctrl Pts',(-2.4400400646031,0.625230809207545,10.3475535382507));
#18203=CARTESIAN_POINT('Ctrl Pts',(-2.45799698585833,0.544111263907802,
10.3527919641193));
#18204=CARTESIAN_POINT('Ctrl Pts',(-2.47594800138103,0.463018397476416,
10.3580286671568));
#18205=CARTESIAN_POINT('Ctrl Pts',(-2.48988833722006,0.381006346250531,
10.3632653701943));
#18206=CARTESIAN_POINT('Ctrl Pts',(-2.49974017991993,0.298505080181056,
10.3685020732318));
#18207=CARTESIAN_POINT('Ctrl Pts',(-2.50959175426053,0.216006061404777,
10.3737386336242));
#18208=CARTESIAN_POINT('Ctrl Pts',(-2.51535500320341,0.133018312568195,
10.3789751940165));
#18209=CARTESIAN_POINT('Ctrl Pts',(-2.51700386379089,0.0499779917736052,
10.3842117544088));
#18210=CARTESIAN_POINT('Ctrl Pts',(-2.51867971178158,-0.0344214752318402,
10.3895340231793));
#18211=CARTESIAN_POINT('Ctrl Pts',(-2.51610525050777,-0.118874759276741,
10.3948562919498));
#18212=CARTESIAN_POINT('Ctrl Pts',(-2.50930823550473,-0.202924688562398,
10.4001785607203));
#18213=CARTESIAN_POINT('Ctrl Pts',(-2.5026110736224,-0.285739862925326,
10.4054226414706));
#18214=CARTESIAN_POINT('Ctrl Pts',(-2.49181472092364,-0.368162998928606,
10.4106667222209));
#18215=CARTESIAN_POINT('Ctrl Pts',(-2.47699780731677,-0.449764507879297,
10.4159108029712));
#18216=CARTESIAN_POINT('Ctrl Pts',(-2.46184951862394,-0.533191006012003,
10.4212721657518));
#18217=CARTESIAN_POINT('Ctrl Pts',(-2.44249877889863,-0.615758184287968,
10.4266335285323));
#18218=CARTESIAN_POINT('Ctrl Pts',(-2.41908365274357,-0.697022618735462,
10.4319948913129));
#18219=CARTESIAN_POINT('Ctrl Pts',(-2.3956685265885,-0.778287053182968,
10.4373562540934));
#18220=CARTESIAN_POINT('Ctrl Pts',(-2.36818924231083,-0.858248284987959,
10.442717616874));
#18221=CARTESIAN_POINT('Ctrl Pts',(-2.33683560324142,-0.936485778548348,
10.4480789796545));
#18222=CARTESIAN_POINT('Ctrl Pts',(-2.30610252288839,-1.01317477694144,
10.4533342290618));
#18223=CARTESIAN_POINT('Ctrl Pts',(-2.27153358025029,-1.08849092484316,
10.4585894784692));
#18224=CARTESIAN_POINT('Ctrl Pts',(-2.23327249983845,-1.1620241785201,10.4638447278765));
#18225=CARTESIAN_POINT('Ctrl Pts',(-2.19506566494669,-1.23545317874822,
10.469092526534));
#18226=CARTESIAN_POINT('Ctrl Pts',(-2.15317730095472,-1.3071038996678,10.4743403251915));
#18227=CARTESIAN_POINT('Ctrl Pts',(-2.10779945922323,-1.37658551848342,
10.479588123849));
#18228=CARTESIAN_POINT('Ctrl Pts',(-2.06209281590818,-1.44657059152742,
10.4848739473319));
#18229=CARTESIAN_POINT('Ctrl Pts',(-2.01284608921402,-1.51435455592319,
10.4901597708148));
#18230=CARTESIAN_POINT('Ctrl Pts',(-1.96030311786669,-1.57956257745052,
10.4954455942977));
#18231=CARTESIAN_POINT('Ctrl Pts',(-1.90823129571664,-1.64418588314981,
10.5006840201663));
#18232=CARTESIAN_POINT('Ctrl Pts',(-1.85292240139207,-1.70627889164405,
10.5059224460349));
#18233=CARTESIAN_POINT('Ctrl Pts',(-1.794656626426,-1.76550668172772,10.5111608719034));
#18234=CARTESIAN_POINT('Ctrl Pts',(-1.73641001410357,-1.82471499277701,
10.5163975749409));
#18235=CARTESIAN_POINT('Ctrl Pts',(-1.67520877585225,-1.88105962824554,
10.5216342779784));
#18236=CARTESIAN_POINT('Ctrl Pts',(-1.61137120149243,-1.93424122099619,
10.526870981016));
#18237=CARTESIAN_POINT('Ctrl Pts',(-1.54753536603621,-1.98742136510686,
10.5321075414083));
#18238=CARTESIAN_POINT('Ctrl Pts',(-1.48106369243104,-2.03743834325886,
10.5373441018006));
#18239=CARTESIAN_POINT('Ctrl Pts',(-1.41230783671028,-2.08403282708472,
10.542580662193));
#18240=CARTESIAN_POINT('Ctrl Pts',(-1.34242663296713,-2.13138993701242,
10.5479029309634));
#18241=CARTESIAN_POINT('Ctrl Pts',(-1.27018620039252,-2.17521122109056,
10.5532251997339));
#18242=CARTESIAN_POINT('Ctrl Pts',(-1.19598512270871,-2.21527105254852,
10.5585474685044));
#18243=CARTESIAN_POINT('Ctrl Pts',(-1.12287411311555,-2.25474237578864,
10.5637915492547));
#18244=CARTESIAN_POINT('Ctrl Pts',(-1.04786013143497,-2.29056188349954,
10.569035630005));
#18245=CARTESIAN_POINT('Ctrl Pts',(-0.971346323524718,-2.32256163960723,
10.5742797107554));
#18246=CARTESIAN_POINT('Ctrl Pts',(-0.893121311085303,-2.35527705905829,
10.5796410735359));
#18247=CARTESIAN_POINT('Ctrl Pts',(-0.813329058487404,-2.38399963696703,
10.5850024363165));
#18248=CARTESIAN_POINT('Ctrl Pts',(-0.732416675826054,-2.40860375798343,
10.590363799097));
#18249=CARTESIAN_POINT('Ctrl Pts',(-0.651504293164715,-2.43320787899983,
10.5957251618776));
#18250=CARTESIAN_POINT('Ctrl Pts',(-0.56947228959179,-2.45369348482417,
10.6010865246581));
#18251=CARTESIAN_POINT('Ctrl Pts',(-0.486776745845734,-2.46999081976104,
10.6064478874387));
#18252=CARTESIAN_POINT('Ctrl Pts',(-0.405717932061537,-2.48596559395061,
10.611703136846));
#18253=CARTESIAN_POINT('Ctrl Pts',(-0.323722213469202,-2.49797542585534,
10.6169583862533));
#18254=CARTESIAN_POINT('Ctrl Pts',(-0.241211782623407,-2.5059176215358,
10.6222136356606));
#18255=CARTESIAN_POINT('Ctrl Pts',(-0.158818332824435,-2.51384855698703,
10.6274614343181));
#18256=CARTESIAN_POINT('Ctrl Pts',(-0.0759120757247375,-2.51772326728586,
10.6327092329755));
#18257=CARTESIAN_POINT('Ctrl Pts',(0.00707460686686389,-2.51749005955092,
10.637957031633));
#18258=CARTESIAN_POINT('Ctrl Pts',(0.0906625995169013,-2.51725516202489,
10.6432428551159));
#18259=CARTESIAN_POINT('Ctrl Pts',(0.174331723135915,-2.51285247283202,
10.6485286785989));
#18260=CARTESIAN_POINT('Ctrl Pts',(0.25763481129679,-2.50428244293811,10.6538145020818));
#18261=CARTESIAN_POINT('Ctrl Pts',(0.340190926416144,-2.49578925991071,
10.6590529279504));
#18262=CARTESIAN_POINT('Ctrl Pts',(0.422387076759307,-2.48320322145356,
10.664291353819));
#18263=CARTESIAN_POINT('Ctrl Pts',(0.503789782285385,-2.46657700168976,
10.6695297796875));
#18264=CARTESIAN_POINT('Ctrl Pts',(0.585165715816503,-2.44995625001291,
10.6747664827251));
#18265=CARTESIAN_POINT('Ctrl Pts',(0.665748271062474,-2.42929804826106,
10.6800031857626));
#18266=CARTESIAN_POINT('Ctrl Pts',(0.745113047788698,-2.40470638457485,
10.6852398888001));
#18267=CARTESIAN_POINT('Ctrl Pts',(0.824475662657691,-2.38011539075338,
10.6904764491924));
#18268=CARTESIAN_POINT('Ctrl Pts',(0.902620124518652,-2.35159128558361,
10.6957130095847));
#18269=CARTESIAN_POINT('Ctrl Pts',(0.979137451061313,-2.31928784369883,
10.700949569977));
#18270=CARTESIAN_POINT('Ctrl Pts',(1.05690715998257,-2.2864556815462,10.7062718387475));
#18271=CARTESIAN_POINT('Ctrl Pts',(1.1329955312796,-2.24971953054739,10.711594107518));
#18272=CARTESIAN_POINT('Ctrl Pts',(1.20699630142809,-2.20929087680616,10.7169163762885));
#18273=CARTESIAN_POINT('Ctrl Pts',(1.27990994615004,-2.16945614955183,10.7221604570388));
#18274=CARTESIAN_POINT('Ctrl Pts',(1.35079655230279,-2.12603698732614,10.7274045377892));
#18275=CARTESIAN_POINT('Ctrl Pts',(1.41929576301148,-2.07928011270672,10.7326486185395));
#18276=CARTESIAN_POINT('Ctrl Pts',(1.4893269345886,-2.03147753695431,10.7380099813201));
#18277=CARTESIAN_POINT('Ctrl Pts',(1.55686222783487,-1.98018646343722,10.7433713441006));
#18278=CARTESIAN_POINT('Ctrl Pts',(1.62155284777459,-1.92571353318039,10.7487327068812));
#18279=CARTESIAN_POINT('Ctrl Pts',(1.6862434677143,-1.87124060292358,10.7540940696618));
#18280=CARTESIAN_POINT('Ctrl Pts',(1.74808908823758,-1.8135862112583,10.7594554324423));
#18281=CARTESIAN_POINT('Ctrl Pts',(1.80678288493526,-1.75309493659215,10.7648167952229));
#18282=CARTESIAN_POINT('Ctrl Pts',(1.86353796867841,-1.69460174731883,10.7700010669979));
#18283=CARTESIAN_POINT('Ctrl Pts',(1.91756794793396,-1.63322734809474,10.7751853387729));
#18284=CARTESIAN_POINT('Ctrl Pts',(1.96856067929309,-1.56925941193326,10.7803696105479));
#18285=CARTESIAN_POINT('Ctrl Pts',(2.0194881038542,-1.50537340001815,10.7855472427847));
#18286=CARTESIAN_POINT('Ctrl Pts',(2.06738570241999,-1.43890080617497,10.7907248750215));
#18287=CARTESIAN_POINT('Ctrl Pts',(2.11197797192582,-1.37016615638399,10.7959025072582));
#18288=CARTESIAN_POINT('Ctrl Pts',(2.15652744873156,-1.30149746738145,10.8010751708117));
#18289=CARTESIAN_POINT('Ctrl Pts',(2.19777763273926,-1.230571425196,10.8062478343652));
#18290=CARTESIAN_POINT('Ctrl Pts',(2.23549414426048,-1.15774443681543,10.8114204979187));
#18291=CARTESIAN_POINT('Ctrl Pts',(2.27318656404733,-1.08496396727738,10.8165898573905));
#18292=CARTESIAN_POINT('Ctrl Pts',(2.30734957417607,-1.01028538234413,10.8217592168623));
#18293=CARTESIAN_POINT('Ctrl Pts',(2.33779370789917,-0.934091445901874,
10.8269285763341));
#18294=CARTESIAN_POINT('Ctrl Pts',(2.36823897829908,-0.857894664646169,
10.8320981288115));
#18295=CARTESIAN_POINT('Ctrl Pts',(2.39496490115964,-0.780182852656203,
10.837267681289));
#18296=CARTESIAN_POINT('Ctrl Pts',(2.41782980818633,-0.701359585837148,
10.8424372337665));
#18297=CARTESIAN_POINT('Ctrl Pts',(2.44069380324846,-0.622539462876305,
10.8476065800568));
#18298=CARTESIAN_POINT('Ctrl Pts',(2.45969696387435,-0.542608431845676,
10.8527759263472));
#18299=CARTESIAN_POINT('Ctrl Pts',(2.47474785657928,-0.461984086691589,
10.8579452726376));
#18300=CARTESIAN_POINT('Ctrl Pts',(2.48981318905341,-0.381282390847459,
10.8631195783791));
#18301=CARTESIAN_POINT('Ctrl Pts',(2.50091860016248,-0.299886521460539,
10.8682938841207));
#18302=CARTESIAN_POINT('Ctrl Pts',(2.50802417071427,-0.218222384536952,
10.8734681898622));
#18303=CARTESIAN_POINT('Ctrl Pts',(2.51440905980166,-0.144841020876706,
10.8781176923931));
#18304=CARTESIAN_POINT('Ctrl Pts',(2.51756501124576,-0.0712433790694381,
10.882767194924));
#18305=CARTESIAN_POINT('Ctrl Pts',(2.51749898433573,0.00226138642592499,
10.8874166974549));
#18306=CARTESIAN_POINT('Ctrl Pts',(2.51749898433498,0.00226138726554988,
10.887416697508));
#18307=CARTESIAN_POINT('Ctrl Pts',(2.5173983212915,0.114324948237316,10.8945052149239));
#18308=CARTESIAN_POINT('Ctrl Pts',(2.50981145266277,0.226062019317946,10.9015937323398));
#18309=CARTESIAN_POINT('Ctrl Pts',(2.49489001405865,0.336645314463777,10.9086822497556));
#18310=CARTESIAN_POINT('Ctrl Pts',(2.48471334971823,0.412064924208791,10.9135167341728));
#18311=CARTESIAN_POINT('Ctrl Pts',(2.4711260222801,0.486948560768708,10.9183512185899));
#18312=CARTESIAN_POINT('Ctrl Pts',(2.4541882701679,0.561040270007676,10.923185703007));
#18313=CARTESIAN_POINT('Ctrl Pts',(2.4357768697415,0.64157823738605,10.9284408058016));
#18314=CARTESIAN_POINT('Ctrl Pts',(2.41336280308272,0.721357675404119,10.9336959085962));
#18315=CARTESIAN_POINT('Ctrl Pts',(2.38702415962054,0.799951193128594,10.9389510113908));
#18316=CARTESIAN_POINT('Ctrl Pts',(2.37886522088455,0.824297158291176,10.9405788880054));
#18317=CARTESIAN_POINT('Ctrl Pts',(2.37033006201922,0.848529372445582,10.94220676462));
#18318=CARTESIAN_POINT('Ctrl Pts',(2.36142200728636,0.872635292378011,10.9438346412346));
#18319=CARTESIAN_POINT('',(2.51749997867612,-0.000327667110924752,10.6149188233509));
#18320=CARTESIAN_POINT('Ctrl Pts',(2.3614219719961,0.872635387876314,10.6673175101421));
#18321=CARTESIAN_POINT('Ctrl Pts',(2.38753013195813,0.801984594384251,10.6628599804557));
#18322=CARTESIAN_POINT('Ctrl Pts',(2.41046358840151,0.730173114338968,10.6584813167228));
#18323=CARTESIAN_POINT('Ctrl Pts',(2.47566938108042,0.489138520415815,10.6440744556866));
#18324=CARTESIAN_POINT('Ctrl Pts',(2.50358581879094,0.316608122570416,10.6342474256015));
#18325=CARTESIAN_POINT('Ctrl Pts',(2.51540284035079,0.108321598130534,10.621654531346));
#18326=CARTESIAN_POINT('Ctrl Pts',(2.51664606178224,0.0740091890297152,
10.6195555519703));
#18327=CARTESIAN_POINT('Ctrl Pts',(2.5173298295721,0.0306372799154144,10.6168595333047));
#18328=CARTESIAN_POINT('Ctrl Pts',(2.51742367915042,0.0215899944366838,
10.6162947943949));
#18329=CARTESIAN_POINT('Ctrl Pts',(2.51749012946065,0.00825247343740583,
10.6154585264606));
#18330=CARTESIAN_POINT('Ctrl Pts',(2.51750053705118,0.00396238565652019,
10.6151889674799));
#18331=CARTESIAN_POINT('Ctrl Pts',(2.51749997867612,-0.000327667110924752,
10.6149188233509));
#18332=CARTESIAN_POINT('Ctrl Pts',(2.51749997858344,-0.000328378448568064,
10.6149187785581));
#18333=CARTESIAN_POINT('Ctrl Pts',(2.51749957459957,-0.00342550428806741,
10.6147237528536));
#18334=CARTESIAN_POINT('Ctrl Pts',(2.51749345531221,-0.0065226102894847,
10.6145284222777));
#18335=CARTESIAN_POINT('Ctrl Pts',(2.51745918050036,-0.0154923684534925,
10.6139618040555));
#18336=CARTESIAN_POINT('Ctrl Pts',(2.51741619102707,-0.0213648877897438,
10.6135897120455));
#18337=CARTESIAN_POINT('Ctrl Pts',(2.51728166745765,-0.033798035259292,
10.6127994435243));
#18338=CARTESIAN_POINT('Ctrl Pts',(2.51718503287258,-0.0403584823729039,
10.6123809765192));
#18339=CARTESIAN_POINT('Ctrl Pts',(2.51689072622532,-0.0561473645042193,
10.6113704201091));
#18340=CARTESIAN_POINT('Ctrl Pts',(2.51666794237783,-0.0653751923519982,
10.6107769720843));
#18341=CARTESIAN_POINT('Ctrl Pts',(2.51574187936881,-0.0966123993385475,
10.6087589821041));
#18342=CARTESIAN_POINT('Ctrl Pts',(2.51480059563153,-0.118613009291447,
10.6073223942329));
#18343=CARTESIAN_POINT('Ctrl Pts',(2.51235677467159,-0.162303085450508,
10.6044427754474));
#18344=CARTESIAN_POINT('Ctrl Pts',(2.51086160499253,-0.183991283202461,
10.603000168833));
#18345=CARTESIAN_POINT('Ctrl Pts',(2.49519664982502,-0.37510942135449,10.5901868837444));
#18346=CARTESIAN_POINT('Ctrl Pts',(2.46417812493984,-0.542712628507912,
10.5782847751557));
#18347=CARTESIAN_POINT('Ctrl Pts',(2.38190687746773,-0.824349383005594,
10.5581486165164));
#18348=CARTESIAN_POINT('Ctrl Pts',(2.33864240964159,-0.940101723006075,
10.5498223723753));
#18349=CARTESIAN_POINT('Ctrl Pts',(2.27083938297377,-1.08747416594008,10.5392326526807));
#18350=CARTESIAN_POINT('Ctrl Pts',(2.25380968384517,-1.12234297212867,10.5367268024903));
#18351=CARTESIAN_POINT('Ctrl Pts',(2.2284959682926,-1.17127163318593,10.5332082794644));
#18352=CARTESIAN_POINT('Ctrl Pts',(2.22087161105699,-1.18566471944585,10.5321729519042));
#18353=CARTESIAN_POINT('Ctrl Pts',(2.20745270224278,-1.21041297998127,10.5303919238626));
#18354=CARTESIAN_POINT('Ctrl Pts',(2.20172370535086,-1.22080291113549,10.5296439474443));
#18355=CARTESIAN_POINT('Ctrl Pts',(2.19057971398888,-1.24067968268403,10.5282123526258));
#18356=CARTESIAN_POINT('Ctrl Pts',(2.18517602014863,-1.25017251823079,10.527528354568));
#18357=CARTESIAN_POINT('Ctrl Pts',(2.17228005079754,-1.2724881836021,10.5259195527403));
#18358=CARTESIAN_POINT('Ctrl Pts',(2.16473570378715,-1.28528057016568,10.5249966324264));
#18359=CARTESIAN_POINT('Ctrl Pts',(2.14184472128715,-1.32332173346476,10.5222494223788));
#18360=CARTESIAN_POINT('Ctrl Pts',(2.12616602175079,-1.34836841364802,10.5204370824753));
#18361=CARTESIAN_POINT('Ctrl Pts',(2.01207723793185,-1.52368485441108,10.5077113295619));
#18362=CARTESIAN_POINT('Ctrl Pts',(1.898273111502,-1.663321474057,10.4974126751653));
#18363=CARTESIAN_POINT('Ctrl Pts',(1.69275831288387,-1.86664256412825,10.4807984124612));
#18364=CARTESIAN_POINT('Ctrl Pts',(1.61002111632048,-1.93845652730022,10.4745039220776));
#18365=CARTESIAN_POINT('Ctrl Pts',(1.48253288465022,-2.03530588075346,10.4649391348528));
#18366=CARTESIAN_POINT('Ctrl Pts',(1.44127115883748,-2.0647301136129,10.4618614093995));
#18367=CARTESIAN_POINT('Ctrl Pts',(1.39159715120258,-2.09793856647254,10.4581411117589));
#18368=CARTESIAN_POINT('Ctrl Pts',(1.38401397268012,-2.10294892416184,10.457572769733));
#18369=CARTESIAN_POINT('Ctrl Pts',(1.36955623184223,-2.11238937277149,10.456488090803));
#18370=CARTESIAN_POINT('Ctrl Pts',(1.36268686844723,-2.11682725523524,10.4559722541331));
#18371=CARTESIAN_POINT('Ctrl Pts',(1.35040395768513,-2.12467794131628,10.4550488382958));
#18372=CARTESIAN_POINT('Ctrl Pts',(1.34499886695179,-2.12810367458251,10.454642115582));
#18373=CARTESIAN_POINT('Ctrl Pts',(1.33310986540093,-2.13557550698314,10.4537466149593));
#18374=CARTESIAN_POINT('Ctrl Pts',(1.32662067451829,-2.13961263819215,10.4532572921579));
#18375=CARTESIAN_POINT('Ctrl Pts',(1.30875323543977,-2.15061600772809,10.4519087068624));
#18376=CARTESIAN_POINT('Ctrl Pts',(1.29733802407315,-2.15752132710056,10.4510457058427));
#18377=CARTESIAN_POINT('Ctrl Pts',(1.2340925713079,-2.19509653468859,10.4462588279196));
#18378=CARTESIAN_POINT('Ctrl Pts',(1.18123353221974,-2.22398726496045,10.4422383422976));
#18379=CARTESIAN_POINT('Ctrl Pts',(0.923549427309861,-2.35304891759812,
10.4227171027183));
#18380=CARTESIAN_POINT('Ctrl Pts',(0.70677037352199,-2.426990624531,10.4066489729991));
#18381=CARTESIAN_POINT('Ctrl Pts',(0.436908130361662,-2.47974193477186,
10.3883259121943));
#18382=CARTESIAN_POINT('Ctrl Pts',(0.3906037965418,-2.48745611209794,10.3852335239401));
#18383=CARTESIAN_POINT('Ctrl Pts',(0.309949773739372,-2.49858488164457,
10.3799365676373));
#18384=CARTESIAN_POINT('Ctrl Pts',(0.275696671197079,-2.50259601431372,
10.3777146410588));
#18385=CARTESIAN_POINT('Ctrl Pts',(0.225893044645415,-2.50739313981557,
10.3745225096445));
#18386=CARTESIAN_POINT('Ctrl Pts',(0.210401799524816,-2.5087405457031,10.3735349822504));
#18387=CARTESIAN_POINT('Ctrl Pts',(0.183189937584401,-2.51085356409409,
10.3718094453232));
#18388=CARTESIAN_POINT('Ctrl Pts',(0.171474722907431,-2.51168083173649,
10.3710695399124));
#18389=CARTESIAN_POINT('Ctrl Pts',(0.147117431978758,-2.51322960338131,
10.3695371897336));
#18390=CARTESIAN_POINT('Ctrl Pts',(0.134474816605329,-2.51393776994115,
10.3687451797638));
#18391=CARTESIAN_POINT('Ctrl Pts',(0.101656131209017,-2.5155277991798,10.3666976082304));
#18392=CARTESIAN_POINT('Ctrl Pts',(0.081473586061596,-2.5162623410592,10.365446636789));
#18393=CARTESIAN_POINT('Ctrl Pts',(-0.00205060046043071,-2.51829618693438,
10.3603012112854));
#18394=CARTESIAN_POINT('Ctrl Pts',(-0.0654241703440023,-2.51744723027823,
10.3564731484526));
#18395=CARTESIAN_POINT('Ctrl Pts',(-0.354587084316347,-2.50264496794959,
10.3392413479069));
#18396=CARTESIAN_POINT('Ctrl Pts',(-0.577860692956225,-2.46069716787177,
10.326692380744));
#18397=CARTESIAN_POINT('Ctrl Pts',(-0.83695234210536,-2.37476492721169,
10.3105936322072));
#18398=CARTESIAN_POINT('Ctrl Pts',(-0.880962771817687,-2.35879243945169,
10.3077980953124));
#18399=CARTESIAN_POINT('Ctrl Pts',(-0.951722428837876,-2.33085547876292,
10.303165253962));
#18400=CARTESIAN_POINT('Ctrl Pts',(-0.978754299980336,-2.31963417241312,
10.301361768732));
#18401=CARTESIAN_POINT('Ctrl Pts',(-1.01497268533276,-2.30385364134825,
10.2988917297993));
#18402=CARTESIAN_POINT('Ctrl Pts',(-1.02433708987833,-2.29970534428829,
10.2982481857628));
#18403=CARTESIAN_POINT('Ctrl Pts',(-1.03989884412982,-2.29269780477186,
10.2971701267101));
#18404=CARTESIAN_POINT('Ctrl Pts',(-1.04611045999065,-2.28987024376169,
10.2967375065194));
#18405=CARTESIAN_POINT('Ctrl Pts',(-1.05783496463517,-2.28447552399394,
10.295916425885));
#18406=CARTESIAN_POINT('Ctrl Pts',(-1.06335020373665,-2.2819135773415,10.2955282948099));
#18407=CARTESIAN_POINT('Ctrl Pts',(-1.07637049324967,-2.27580792146334,
10.2946076129807));
#18408=CARTESIAN_POINT('Ctrl Pts',(-1.0838673544966,-2.27224705685503,10.2940740377422));
#18409=CARTESIAN_POINT('Ctrl Pts',(-1.1099791569752,-2.25968582896782,10.2922038149076));
#18410=CARTESIAN_POINT('Ctrl Pts',(-1.12850013939999,-2.2504935336932,10.2908563148761));
#18411=CARTESIAN_POINT('Ctrl Pts',(-1.28754299472856,-2.16910085451562,
10.2791161168946));
#18412=CARTESIAN_POINT('Ctrl Pts',(-1.42108173315797,-2.0840547403687,10.2681331159879));
#18413=CARTESIAN_POINT('Ctrl Pts',(-1.64239481745146,-1.91189303956432,
10.2487801092099));
#18414=CARTESIAN_POINT('Ctrl Pts',(-1.73342657162677,-1.82976330741955,
10.2403986447282));
#18415=CARTESIAN_POINT('Ctrl Pts',(-1.84902955455047,-1.7090617178523,10.2292833192714));
#18416=CARTESIAN_POINT('Ctrl Pts',(-1.8790689352992,-1.67597809748634,10.2263441803925));
#18417=CARTESIAN_POINT('Ctrl Pts',(-1.92987233512501,-1.61694205003993,
10.221282307625));
#18418=CARTESIAN_POINT('Ctrl Pts',(-1.95103197319459,-1.59134635906815,
10.2191442233013));
#18419=CARTESIAN_POINT('Ctrl Pts',(-1.98120479631392,-1.5533410660387,10.2160494120328));
#18420=CARTESIAN_POINT('Ctrl Pts',(-1.99062016236569,-1.54125672698266,
10.2150768087034));
#18421=CARTESIAN_POINT('Ctrl Pts',(-2.00703784409035,-1.51978369797835,
10.2133683308657));
#18422=CARTESIAN_POINT('Ctrl Pts',(-2.01408596744621,-1.51043077281748,
10.212630677117));
#18423=CARTESIAN_POINT('Ctrl Pts',(-2.02867908161984,-1.49078179319963,
10.2110943309542));
#18424=CARTESIAN_POINT('Ctrl Pts',(-2.03621156347878,-1.48047683178363,
10.2102961357227));
#18425=CARTESIAN_POINT('Ctrl Pts',(-2.05573188399112,-1.45334085388171,
10.2082135834458));
#18426=CARTESIAN_POINT('Ctrl Pts',(-2.06759160317454,-1.43641853867961,
10.2069341211091));
#18427=CARTESIAN_POINT('Ctrl Pts',(-2.11728903364949,-1.36361559741499,
10.2015083685032));
#18428=CARTESIAN_POINT('Ctrl Pts',(-2.15308182660201,-1.30636908079411,
10.1974381523756));
#18429=CARTESIAN_POINT('Ctrl Pts',(-2.28446057396817,-1.0761433446066,10.1817007121886));
#18430=CARTESIAN_POINT('Ctrl Pts',(-2.36184108735325,-0.89361573269217,
10.1706262664755));
#18431=CARTESIAN_POINT('Ctrl Pts',(-2.43448126368547,-0.644187755481913,
10.1554761063338));
#18432=CARTESIAN_POINT('Ctrl Pts',(-2.44965576886291,-0.583834296811531,
10.1518033369345));
#18433=CARTESIAN_POINT('Ctrl Pts',(-2.46998643302507,-0.488103353977006,
10.1458814130446));
#18434=CARTESIAN_POINT('Ctrl Pts',(-2.47665197046114,-0.453070174549224,
10.1436942312045));
#18435=CARTESIAN_POINT('Ctrl Pts',(-2.48439939026788,-0.407046992703168,
10.1407809192934));
#18436=CARTESIAN_POINT('Ctrl Pts',(-2.48615658184325,-0.396172973255005,
10.1400896759648));
#18437=CARTESIAN_POINT('Ctrl Pts',(-2.48891246160676,-0.378377988306357,
10.1389532155672));
#18438=CARTESIAN_POINT('Ctrl Pts',(-2.48995379559916,-0.371463640900195,
10.1385103410759));
#18439=CARTESIAN_POINT('Ctrl Pts',(-2.49193211997425,-0.357945591364488,
10.1376418013031));
#18440=CARTESIAN_POINT('Ctrl Pts',(-2.49287169276949,-0.351342364016672,
10.1372162821138));
#18441=CARTESIAN_POINT('Ctrl Pts',(-2.49491356548371,-0.336571648608706,
10.1362617404116));
#18442=CARTESIAN_POINT('Ctrl Pts',(-2.49600201870287,-0.328402332515074,
10.1357319646937));
#18443=CARTESIAN_POINT('Ctrl Pts',(-2.49963744276939,-0.300054286493891,
10.1338875669656));
#18444=CARTESIAN_POINT('Ctrl Pts',(-2.50197989940242,-0.279850748376581,
10.1325624699713));
#18445=CARTESIAN_POINT('Ctrl Pts',(-2.52092357286169,-0.0971372093117507,
10.1204962948171));
#18446=CARTESIAN_POINT('Ctrl Pts',(-2.52191378982063,0.0665877779835312,
10.1091228666568));
#18447=CARTESIAN_POINT('Ctrl Pts',(-2.49129956622154,0.401395038494172,
10.0859288283872));
#18448=CARTESIAN_POINT('Ctrl Pts',(-2.45786506292514,0.571498928622087,
10.0741941900692));
#18449=CARTESIAN_POINT('Ctrl Pts',(-2.39948689554551,0.762215295139084,
10.0613076607371));
#18450=CARTESIAN_POINT('Ctrl Pts',(-2.39132445884022,0.787449641823742,
10.0596071326662));
#18451=CARTESIAN_POINT('Ctrl Pts',(-2.37824015787482,0.825818684746376,
10.0570275551696));
#18452=CARTESIAN_POINT('Ctrl Pts',(-2.37360495124534,0.839048447328103,
10.0561392224297));
#18453=CARTESIAN_POINT('Ctrl Pts',(-2.36531792395057,0.862082833196594,
10.0545942805152));
#18454=CARTESIAN_POINT('Ctrl Pts',(-2.36171507343008,0.871904587620782,
10.0539360796937));
#18455=CARTESIAN_POINT('Ctrl Pts',(-2.35343463355426,0.894050008575098,
10.052453135533));
#18456=CARTESIAN_POINT('Ctrl Pts',(-2.34872124634027,0.906360033174254,
10.0516295986676));
#18457=CARTESIAN_POINT('Ctrl Pts',(-2.33567290266129,0.939653167424983,
10.049404075569));
#18458=CARTESIAN_POINT('Ctrl Pts',(-2.32715188697292,0.960562402589358,
10.0480083076319));
#18459=CARTESIAN_POINT('Ctrl Pts',(-2.28341828692826,1.06387857650208,10.0411171406873));
#18460=CARTESIAN_POINT('Ctrl Pts',(-2.24410256816616,1.14448367673421,10.0357616948804));
#18461=CARTESIAN_POINT('Ctrl Pts',(-2.11500515130242,1.37680401994983,10.0201601264924));
#18462=CARTESIAN_POINT('Ctrl Pts',(-2.01352260459123,1.52136775236244,10.0102564927425));
#18463=CARTESIAN_POINT('Ctrl Pts',(-1.85885721426075,1.6988131419265,9.99650366605367));
#18464=CARTESIAN_POINT('Ctrl Pts',(-1.81836755050526,1.74208346018455,9.99299895726296));
#18465=CARTESIAN_POINT('Ctrl Pts',(-1.75993658156716,1.80026908820957,9.98800366674946));
#18466=CARTESIAN_POINT('Ctrl Pts',(-1.74325552388882,1.81642661851913,9.98658420739711));
#18467=CARTESIAN_POINT('Ctrl Pts',(-1.71373816425295,1.84423647881634,9.9840787237502));
#18468=CARTESIAN_POINT('Ctrl Pts',(-1.70100035531801,1.8559914973267,9.98299948974418));
#18469=CARTESIAN_POINT('Ctrl Pts',(-1.68196532890022,1.8731973249436,9.98138778796064));
#18470=CARTESIAN_POINT('Ctrl Pts',(-1.67576050226168,1.87875020164524,9.98086258934892));
#18471=CARTESIAN_POINT('Ctrl Pts',(-1.66511554724683,1.88818198920309,9.97996161212716));
#18472=CARTESIAN_POINT('Ctrl Pts',(-1.66068916591767,1.89207624142267,9.97958697611093));
#18473=CARTESIAN_POINT('Ctrl Pts',(-1.65062432977439,1.90086857857118,9.97873507813718));
#18474=CARTESIAN_POINT('Ctrl Pts',(-1.64497784619459,1.90575704462086,9.97825714630172));
#18475=CARTESIAN_POINT('Ctrl Pts',(-1.62956708164645,1.91897946139476,9.9769529222285));
#18476=CARTESIAN_POINT('Ctrl Pts',(-1.61976082684076,1.92726383617347,9.97612320684488));
#18477=CARTESIAN_POINT('Ctrl Pts',(-1.57035020650584,1.96836271573562,9.97194535575163));
#18478=CARTESIAN_POINT('Ctrl Pts',(-1.52981286797455,2.00003082825864,9.96852694758394));
#18479=CARTESIAN_POINT('Ctrl Pts',(-1.3666869264535,2.11960458498591,9.95489462403589));
#18480=CARTESIAN_POINT('Ctrl Pts',(-1.23727226613267,2.1976607084222,9.94436476990255));
#18481=CARTESIAN_POINT('Ctrl Pts',(-0.971402086897258,2.32705124523744,
9.92405367907568));
#18482=CARTESIAN_POINT('Ctrl Pts',(-0.835906816978862,2.37908838904751,
9.91429771706695));
#18483=CARTESIAN_POINT('Ctrl Pts',(-0.670357757058067,2.4267625166531,9.90315799669041));
#18484=CARTESIAN_POINT('Ctrl Pts',(-0.643925756265351,2.43390952003248,
9.90140135674121));
#18485=CARTESIAN_POINT('Ctrl Pts',(-0.603621092038556,2.44410500874085,
9.89875501193101));
#18486=CARTESIAN_POINT('Ctrl Pts',(-0.589831219859135,2.4474694813251,9.8978552678731));
#18487=CARTESIAN_POINT('Ctrl Pts',(-0.564723631774981,2.45337073630171,
9.89622714899279));
#18488=CARTESIAN_POINT('Ctrl Pts',(-0.553415516372069,2.45594625827215,
9.89549755773439));
#18489=CARTESIAN_POINT('Ctrl Pts',(-0.52895349010041,2.4613401653427,9.89392706945352));
#18490=CARTESIAN_POINT('Ctrl Pts',(-0.515793925170151,2.46413145796284,
9.89308705236989));
#18491=CARTESIAN_POINT('Ctrl Pts',(-0.47987712673323,2.4714494825323,9.89080713412552));
#18492=CARTESIAN_POINT('Ctrl Pts',(-0.457078328765627,2.47576736752077,
9.88937384203083));
#18493=CARTESIAN_POINT('Ctrl Pts',(-0.331523446930536,2.49775277893056,
9.88155187993226));
#18494=CARTESIAN_POINT('Ctrl Pts',(-0.227799753290429,2.50934009742363,
9.87535718135092));
#18495=CARTESIAN_POINT('Ctrl Pts',(0.0417160593748585,2.52259327000825,
9.8596143634522));
#18496=CARTESIAN_POINT('Ctrl Pts',(0.207468441432837,2.51439261681814,9.85029044450562));
#18497=CARTESIAN_POINT('Ctrl Pts',(0.452363150396881,2.47788338317032,9.83578656165403));
#18498=CARTESIAN_POINT('Ctrl Pts',(0.532868130982717,2.46182598414749,9.83089158469095));
#18499=CARTESIAN_POINT('Ctrl Pts',(0.626101070168777,2.43844256994088,9.82492410392657));
#18500=CARTESIAN_POINT('Ctrl Pts',(0.639736303658354,2.43490085168376,9.8240437431648));
#18501=CARTESIAN_POINT('Ctrl Pts',(0.660743542832745,2.4292556431424,9.82267459670275));
#18502=CARTESIAN_POINT('Ctrl Pts',(0.668137117730192,2.42723253878861,9.82219025841161));
#18503=CARTESIAN_POINT('Ctrl Pts',(0.681804255258157,2.42342562231827,9.82129019244053));
#18504=CARTESIAN_POINT('Ctrl Pts',(0.688080238292918,2.42165116641887,9.82087499924405));
#18505=CARTESIAN_POINT('Ctrl Pts',(0.702423293231371,2.41753558915091,9.81992184103611));
#18506=CARTESIAN_POINT('Ctrl Pts',(0.710485562041883,2.41517847559543,9.81938297856681));
#18507=CARTESIAN_POINT('Ctrl Pts',(0.731654057910166,2.4088744138878,9.81796026731902));
#18508=CARTESIAN_POINT('Ctrl Pts',(0.744739953539584,2.40486090750032,9.81707282940518));
#18509=CARTESIAN_POINT('Ctrl Pts',(0.856428648585164,2.36960645332421,9.80943414743815));
#18510=CARTESIAN_POINT('Ctrl Pts',(0.953042214726981,2.332425895425,9.80239952620401));
#18511=CARTESIAN_POINT('Ctrl Pts',(1.197221327585,2.22074845323684,9.78393008628809));
#18512=CARTESIAN_POINT('Ctrl Pts',(1.34025663832435,2.13747145108765,9.77244171894969));
#18513=CARTESIAN_POINT('Ctrl Pts',(1.54318947344083,1.99088768942309,9.75563412759824));
#18514=CARTESIAN_POINT('Ctrl Pts',(1.60969452066259,1.93751228449982,9.75002316110792));
#18515=CARTESIAN_POINT('Ctrl Pts',(1.68940639355854,1.86659394952443,9.74316482921825));
#18516=CARTESIAN_POINT('Ctrl Pts',(1.70525942239742,1.85212237282638,9.74179363094978));
#18517=CARTESIAN_POINT('Ctrl Pts',(1.73036941159569,1.82860475742239,9.73960949664));
#18518=CARTESIAN_POINT('Ctrl Pts',(1.73974478878245,1.81968726420496,9.73879118575063));
#18519=CARTESIAN_POINT('Ctrl Pts',(1.75744201355821,1.80259255514466,9.73724093439485));
#18520=CARTESIAN_POINT('Ctrl Pts',(1.7657765525782,1.79442902467809,9.73650843539827));
#18521=CARTESIAN_POINT('Ctrl Pts',(1.78467661374134,1.77565756192688,9.73484163468123));
#18522=CARTESIAN_POINT('Ctrl Pts',(1.79520492260039,1.76501266114465,9.73390898213249));
#18523=CARTESIAN_POINT('Ctrl Pts',(1.82747476225071,1.73179799026465,9.73103671347212));
#18524=CARTESIAN_POINT('Ctrl Pts',(1.84889081714552,1.70891520124081,9.72911106393133));
#18525=CARTESIAN_POINT('Ctrl Pts',(2.00449919592539,1.53629911474618,9.71495430327224));
#18526=CARTESIAN_POINT('Ctrl Pts',(2.12074928845023,1.37137273952955,9.7035194184664));
#18527=CARTESIAN_POINT('Ctrl Pts',(2.27205578341547,1.0906218481476,9.6851564163805));
#18528=CARTESIAN_POINT('Ctrl Pts',(2.32059591720706,0.983114007988647,9.67832658896893));
#18529=CARTESIAN_POINT('Ctrl Pts',(2.36142200350084,0.872635302621939,9.67114329893353));
#18530=CARTESIAN_POINT('Origin',(0.,0.,10.));
#18531=CARTESIAN_POINT('',(2.36142186693781,0.872635672172493,8.66836043115426));
#18532=CARTESIAN_POINT('',(2.36142200728636,0.872635292378026,8.94380698639026));
#18533=CARTESIAN_POINT('',(2.36142200728636,0.87263529237802,10.));
#18534=CARTESIAN_POINT('',(2.51749994136415,-0.000543352107728946,9.88741669745326));
#18535=CARTESIAN_POINT('Ctrl Pts',(2.36142200728635,0.872635292378026,8.94380698639026));
#18536=CARTESIAN_POINT('Ctrl Pts',(2.33302028921955,0.949492649252658,8.94896806576715));
#18537=CARTESIAN_POINT('Ctrl Pts',(2.30085777760834,1.02497408410551,8.95412914514404));
#18538=CARTESIAN_POINT('Ctrl Pts',(2.26510290562476,1.09868788877018,8.95929022452092));
#18539=CARTESIAN_POINT('Ctrl Pts',(2.22846148870633,1.17422943316732,8.96457927327726));
#18540=CARTESIAN_POINT('Ctrl Pts',(2.18804739574404,1.24791403963753,8.96986832203359));
#18541=CARTESIAN_POINT('Ctrl Pts',(2.14409230335549,1.31934621865974,8.97515737078992));
#18542=CARTESIAN_POINT('Ctrl Pts',(2.10114674343037,1.3891377890576,8.98032494405548));
#18543=CARTESIAN_POINT('Ctrl Pts',(2.05482143374227,1.45677892969738,8.98549251732103));
#18544=CARTESIAN_POINT('Ctrl Pts',(2.00537560108398,1.52193132189894,8.99066009058658));
#18545=CARTESIAN_POINT('Ctrl Pts',(1.95418626432411,1.58938104548163,8.99600987708831));
#18546=CARTESIAN_POINT('Ctrl Pts',(1.89965259770243,1.6541628068661,9.00135966359003));
#18547=CARTESIAN_POINT('Ctrl Pts',(1.84210502463234,1.71594152820668,9.00670945009175));
#18548=CARTESIAN_POINT('Ctrl Pts',(1.78455745156225,1.77772024954727,9.01205923659348));
#18549=CARTESIAN_POINT('Ctrl Pts',(1.72399642618433,1.8364955984303,9.0174090230952));
#18550=CARTESIAN_POINT('Ctrl Pts',(1.66078955074694,1.89197894230612,9.02275880959693));
#18551=CARTESIAN_POINT('Ctrl Pts',(1.59869961602288,1.9464818294633,9.02801405900423));
#18552=CARTESIAN_POINT('Ctrl Pts',(1.53380920573821,1.99802568053148,9.03326930841153));
#18553=CARTESIAN_POINT('Ctrl Pts',(1.46643193098255,2.04630976193606,9.03852455781883));
#18554=CARTESIAN_POINT('Ctrl Pts',(1.39915018189616,2.09452538748206,9.04377235647632));
#18555=CARTESIAN_POINT('Ctrl Pts',(1.32938894355375,2.13949015670334,9.04902015513382));
#18556=CARTESIAN_POINT('Ctrl Pts',(1.25749623897869,2.18094233278976,9.05426795379132));
#18557=CARTESIAN_POINT('Ctrl Pts',(1.18508260978013,2.22269486562794,9.05955377727422));
#18558=CARTESIAN_POINT('Ctrl Pts',(1.11050685153594,2.2608833743918,9.06483960075713));
#18559=CARTESIAN_POINT('Ctrl Pts',(1.0341559473649,2.2952838008686,9.07012542424004));
#18560=CARTESIAN_POINT('Ctrl Pts',(0.958489676481416,2.32937576109568,9.07536385010863));
#18561=CARTESIAN_POINT('Ctrl Pts',(0.881080395831208,2.3597471088514,9.08060227597723));
#18562=CARTESIAN_POINT('Ctrl Pts',(0.802329463704639,2.38622582369553,9.08584070184582));
#18563=CARTESIAN_POINT('Ctrl Pts',(0.723604431449088,2.41269583013101,9.09107740488332));
#18564=CARTESIAN_POINT('Ctrl Pts',(0.64353906107271,2.43527559930725,9.09631410792082));
#18565=CARTESIAN_POINT('Ctrl Pts',(0.562552613965812,2.45384205003505,9.10155081095832));
#18566=CARTESIAN_POINT('Ctrl Pts',(0.4815683728892,2.47240799502203,9.10678737135065));
#18567=CARTESIAN_POINT('Ctrl Pts',(0.39966355495031,2.4869607368158,9.11202393174299));
#18568=CARTESIAN_POINT('Ctrl Pts',(0.317269076047917,2.49742799363339,9.11726049213532));
#18569=CARTESIAN_POINT('Ctrl Pts',(0.233526021625283,2.50806657122995,9.1225827609058));
#18570=CARTESIAN_POINT('Ctrl Pts',(0.149277618914341,2.51448464551231,9.12790502967628));
#18571=CARTESIAN_POINT('Ctrl Pts',(0.0649813996984492,2.51666121432608,
9.13322729844677));
#18572=CARTESIAN_POINT('Ctrl Pts',(-0.018076446415588,2.51880580775237,
9.1384713791971));
#18573=CARTESIAN_POINT('Ctrl Pts',(-0.101180247008542,2.51683276258221,
9.14371545994744));
#18574=CARTESIAN_POINT('Ctrl Pts',(-0.183894488815157,2.51077459501713,
9.14895954069778));
#18575=CARTESIAN_POINT('Ctrl Pts',(-0.268458605684501,2.5045809386552,9.15432090347833));
#18576=CARTESIAN_POINT('Ctrl Pts',(-0.352615020686498,2.49411729347784,
9.15968226625889));
#18577=CARTESIAN_POINT('Ctrl Pts',(-0.435908145371969,2.47947380280542,
9.16504362903945));
#18578=CARTESIAN_POINT('Ctrl Pts',(-0.519201270057435,2.46483031213301,
9.17040499182));
#18579=CARTESIAN_POINT('Ctrl Pts',(-0.601630623941684,2.44600715420398,
9.17576635460055));
#18580=CARTESIAN_POINT('Ctrl Pts',(-0.682757877074033,2.42314835107002,
9.18112771738111));
#18581=CARTESIAN_POINT('Ctrl Pts',(-0.762279440227115,2.40074197482977,
9.18638296678842));
#18582=CARTESIAN_POINT('Ctrl Pts',(-0.840843710027793,2.3743755294766,9.19163821619573));
#18583=CARTESIAN_POINT('Ctrl Pts',(-0.918027687426472,2.34414833470888,
9.19689346560304));
#18584=CARTESIAN_POINT('Ctrl Pts',(-0.995102235479325,2.31396399523653,
9.20214126426054));
#18585=CARTESIAN_POINT('Ctrl Pts',(-1.07079995212278,2.27992994550431,9.20738906291804));
#18586=CARTESIAN_POINT('Ctrl Pts',(-1.14471181286138,2.24219560152445,9.21263686157554));
#18587=CARTESIAN_POINT('Ctrl Pts',(-1.2191592287505,2.20418783969166,9.21792268505845));
#18588=CARTESIAN_POINT('Ctrl Pts',(-1.29179434327592,2.16242606222498,9.22320850854136));
#18589=CARTESIAN_POINT('Ctrl Pts',(-1.36221852457427,2.11711287873526,9.22849433202426));
#18590=CARTESIAN_POINT('Ctrl Pts',(-1.43201121710003,2.07220601543409,9.23373275789286));
#18591=CARTESIAN_POINT('Ctrl Pts',(-1.49963207297705,2.02381143571954,9.23897118376145));
#18592=CARTESIAN_POINT('Ctrl Pts',(-1.56471828263945,1.97217213903195,9.24420960963005));
#18593=CARTESIAN_POINT('Ctrl Pts',(-1.62978308653067,1.92054982564965,9.24944631266755));
#18594=CARTESIAN_POINT('Ctrl Pts',(-1.69231453860351,1.86568520124345,9.25468301570506));
#18595=CARTESIAN_POINT('Ctrl Pts',(-1.75198113178758,1.80786292728743,9.25991971874256));
#18596=CARTESIAN_POINT('Ctrl Pts',(-1.81164609968345,1.75004222838129,9.26515627913489));
#18597=CARTESIAN_POINT('Ctrl Pts',(-1.8684460332117,1.68926436196184,9.27039283952722));
#18598=CARTESIAN_POINT('Ctrl Pts',(-1.92208569013667,1.62585142303097,9.27562939991955));
#18599=CARTESIAN_POINT('Ctrl Pts',(-1.97660328365647,1.56140058522333,9.28095166869003));
#18600=CARTESIAN_POINT('Ctrl Pts',(-2.02785588922117,1.49422800555234,9.2862739374605));
#18601=CARTESIAN_POINT('Ctrl Pts',(-2.07557678649202,1.42470602349237,9.29159620623098));
#18602=CARTESIAN_POINT('Ctrl Pts',(-2.12259662888613,1.35620537018672,9.29684028698132));
#18603=CARTESIAN_POINT('Ctrl Pts',(-2.16618764778015,1.28542431585706,9.30208436773166));
#18604=CARTESIAN_POINT('Ctrl Pts',(-2.20614000163594,1.21274586916706,9.30732844848199));
#18605=CARTESIAN_POINT('Ctrl Pts',(-2.24698587589978,1.13844199445904,9.31268981126254));
#18606=CARTESIAN_POINT('Ctrl Pts',(-2.28402814256931,1.06215529485584,9.31805117404309));
#18607=CARTESIAN_POINT('Ctrl Pts',(-2.31709436732389,0.984316993105329,
9.32341253682364));
#18608=CARTESIAN_POINT('Ctrl Pts',(-2.35016059207846,0.906478691354823,
9.32877389960418));
#18609=CARTESIAN_POINT('Ctrl Pts',(-2.37925066282246,0.827089287526063,
9.33413526238473));
#18610=CARTESIAN_POINT('Ctrl Pts',(-2.40424673471584,0.746594862430907,
9.33949662516528));
#18611=CARTESIAN_POINT('Ctrl Pts',(-2.42874807838152,0.66769360223127,9.34475187457258));
#18612=CARTESIAN_POINT('Ctrl Pts',(-2.44940654676642,0.58743924649994,9.35000712397989));
#18613=CARTESIAN_POINT('Ctrl Pts',(-2.4660751459744,0.506240678341169,9.35526237338719));
#18614=CARTESIAN_POINT('Ctrl Pts',(-2.48272011289535,0.425157231306012,
9.36051017204468));
#18615=CARTESIAN_POINT('Ctrl Pts',(-2.49538635454002,0.343132679074537,
9.36575797070217));
#18616=CARTESIAN_POINT('Ctrl Pts',(-2.50397650588169,0.26059145801906,9.37100576935966));
#18617=CARTESIAN_POINT('Ctrl Pts',(-2.51262890027544,0.177452154657975,
9.37629159284257));
#18618=CARTESIAN_POINT('Ctrl Pts',(-2.51714574501048,0.0937891160271414,
9.38157741632548));
#18619=CARTESIAN_POINT('Ctrl Pts',(-2.51747995172501,0.0100470225771085,
9.38686323980839));
#18620=CARTESIAN_POINT('Ctrl Pts',(-2.51781116163099,-0.072944161301374,
9.39210166567699));
#18621=CARTESIAN_POINT('Ctrl Pts',(-2.51403444206278,-0.156012517999937,
9.39734009154558));
#18622=CARTESIAN_POINT('Ctrl Pts',(-2.50615608684176,-0.238721424229121,
9.40257851741418));
#18623=CARTESIAN_POINT('Ctrl Pts',(-2.49828032268067,-0.321403128875424,
9.40781522045169));
#18624=CARTESIAN_POINT('Ctrl Pts',(-2.48630564569439,-0.403725158859143,
9.41305192348919));
#18625=CARTESIAN_POINT('Ctrl Pts',(-2.4702903381893,-0.485254464223237,
9.41828862652669));
#18626=CARTESIAN_POINT('Ctrl Pts',(-2.45427546693321,-0.566781548769688,
9.42352518691902));
#18627=CARTESIAN_POINT('Ctrl Pts',(-2.43422027394709,-0.647515499060678,
9.42876174731134));
#18628=CARTESIAN_POINT('Ctrl Pts',(-2.41023418493754,-0.727033303060081,
9.43399830770367));
#18629=CARTESIAN_POINT('Ctrl Pts',(-2.38585550830685,-0.807852599165939,
9.43932057647415));
#18630=CARTESIAN_POINT('Ctrl Pts',(-2.35741622780999,-0.887415105170079,
9.44464284524463));
#18631=CARTESIAN_POINT('Ctrl Pts',(-2.32508344262074,-0.965294377302017,
9.44996511401511));
#18632=CARTESIAN_POINT('Ctrl Pts',(-2.29322564968929,-1.04202954597707,
9.45520919476545));
#18633=CARTESIAN_POINT('Ctrl Pts',(-2.25758824566464,-1.11713021185032,
9.46045327551578));
#18634=CARTESIAN_POINT('Ctrl Pts',(-2.21837824670601,-1.19021183179364,
9.46569735626611));
#18635=CARTESIAN_POINT('Ctrl Pts',(-2.17829132984662,-1.26492789658387,
9.47105871904667));
#18636=CARTESIAN_POINT('Ctrl Pts',(-2.13447035466995,-1.33753307677758,
9.47642008182723));
#18637=CARTESIAN_POINT('Ctrl Pts',(-2.08718314535509,-1.40764795589865,
9.48178144460779));
#18638=CARTESIAN_POINT('Ctrl Pts',(-2.03989593604022,-1.47776283501973,
9.48714280738834));
#18639=CARTESIAN_POINT('Ctrl Pts',(-1.98914285101059,-1.54538704677986,
9.4925041701689));
#18640=CARTESIAN_POINT('Ctrl Pts',(-1.93523389860261,-1.61017887444201,
9.49786553294946));
#18641=CARTESIAN_POINT('Ctrl Pts',(-1.88239192506227,-1.67368832676902,
9.50312078235677));
#18642=CARTESIAN_POINT('Ctrl Pts',(-1.82632272598332,-1.73471109993205,
9.50837603176407));
#18643=CARTESIAN_POINT('Ctrl Pts',(-1.76728923830295,-1.79290127954067,
9.51363128117138));
#18644=CARTESIAN_POINT('Ctrl Pts',(-1.70833944669725,-1.85100895869389,
9.51887907982888));
#18645=CARTESIAN_POINT('Ctrl Pts',(-1.64643404012571,-1.90629169997373,
9.52412687848638));
#18646=CARTESIAN_POINT('Ctrl Pts',(-1.58187602200219,-1.95843674930147,
9.52937467714388));
#18647=CARTESIAN_POINT('Ctrl Pts',(-1.51685022538183,-2.01095963446589,
9.53466050062678));
#18648=CARTESIAN_POINT('Ctrl Pts',(-1.4491335171903,-2.06029880096679,9.53994632410969));
#18649=CARTESIAN_POINT('Ctrl Pts',(-1.37907325462678,-2.10617264448409,
9.5452321475926));
#18650=CARTESIAN_POINT('Ctrl Pts',(-1.30964121760168,-2.15163514041306,
9.55047057346119));
#18651=CARTESIAN_POINT('Ctrl Pts',(-1.23790787999561,-2.19369395365338,
9.55570899932979));
#18652=CARTESIAN_POINT('Ctrl Pts',(-1.16424290473617,-2.23211664318231,
9.56094742519839));
#18653=CARTESIAN_POINT('Ctrl Pts',(-1.09060215666123,-2.27052669612806,
9.56618412823589));
#18654=CARTESIAN_POINT('Ctrl Pts',(-1.0150314414322,-2.3053027871869,9.57142083127339));
#18655=CARTESIAN_POINT('Ctrl Pts',(-0.937925729904853,-2.33625802838266,
9.57665753431089));
#18656=CARTESIAN_POINT('Ctrl Pts',(-0.860822118698498,-2.36721242637315,
9.58189409470322));
#18657=CARTESIAN_POINT('Ctrl Pts',(-0.782184022913733,-2.39434601048332,
9.58713065509555));
#18658=CARTESIAN_POINT('Ctrl Pts',(-0.702425838779753,-2.41752025658826,
9.59236721548788));
#18659=CARTESIAN_POINT('Ctrl Pts',(-0.621362228164636,-2.44107380263432,
9.59768948425836));
#18660=CARTESIAN_POINT('Ctrl Pts',(-0.539142001277231,-2.46053708415148,
9.60301175302884));
#18661=CARTESIAN_POINT('Ctrl Pts',(-0.456213833268316,-2.47581808466103,
9.60833402179932));
#18662=CARTESIAN_POINT('Ctrl Pts',(-0.374503940688586,-2.49087459609889,
9.61357810254966));
#18663=CARTESIAN_POINT('Ctrl Pts',(-0.292107241289309,-2.50187089130879,
9.6188221833));
#18664=CARTESIAN_POINT('Ctrl Pts',(-0.209458997150726,-2.50877124874162,
9.62406626405033));
#18665=CARTESIAN_POINT('Ctrl Pts',(-0.124962353964239,-2.51582593025287,
9.62942762683089));
#18666=CARTESIAN_POINT('Ctrl Pts',(-0.0402032906123846,-2.51859923804143,
9.63478898961143));
#18667=CARTESIAN_POINT('Ctrl Pts',(0.0443541239994344,-2.51710924706979,
9.64015035239199));
#18668=CARTESIAN_POINT('Ctrl Pts',(0.128911538611253,-2.51561925609815,
9.64551171517254));
#18669=CARTESIAN_POINT('Ctrl Pts',(0.213266802099033,-2.50986606758288,
9.65087307795309));
#18670=CARTESIAN_POINT('Ctrl Pts',(0.296964500577313,-2.49992366591399,
9.65623444073364));
#18671=CARTESIAN_POINT('Ctrl Pts',(0.37900563420771,-2.49017804663468,9.66148969014094));
#18672=CARTESIAN_POINT('Ctrl Pts',(0.460718028521943,-2.47637157911841,
9.66674493954823));
#18673=CARTESIAN_POINT('Ctrl Pts',(0.541668376772104,-2.45853647920975,
9.67200018895553));
#18674=CARTESIAN_POINT('Ctrl Pts',(0.622503955817923,-2.44072666542116,
9.677247987613));
#18675=CARTESIAN_POINT('Ctrl Pts',(0.70257918795143,-2.41889966276629,9.68249578627047));
#18676=CARTESIAN_POINT('Ctrl Pts',(0.78146676678254,-2.39313934872469,9.68774358492795));
#18677=CARTESIAN_POINT('Ctrl Pts',(0.860925954131833,-2.36719237899971,
9.69302940841086));
#18678=CARTESIAN_POINT('Ctrl Pts',(0.939179733833506,-2.33725491281245,
9.69831523189377));
#18679=CARTESIAN_POINT('Ctrl Pts',(1.01580277918708,-2.30346499079014,9.70360105537668));
#18680=CARTESIAN_POINT('Ctrl Pts',(1.09173875098174,-2.2699780606663,9.70883948124527));
#18681=CARTESIAN_POINT('Ctrl Pts',(1.16607268668969,-2.23270767701616,9.71407790711385));
#18682=CARTESIAN_POINT('Ctrl Pts',(1.2384083530163,-2.19183735737382,9.71931633298244));
#18683=CARTESIAN_POINT('Ctrl Pts',(1.3107202293462,-2.15098047929938,9.72455303601994));
#18684=CARTESIAN_POINT('Ctrl Pts',(1.38103474011051,-2.10652624344335,9.72978973905744));
#18685=CARTESIAN_POINT('Ctrl Pts',(1.44898008261764,-2.05870419686204,9.73502644209495));
#18686=CARTESIAN_POINT('Ctrl Pts',(1.51692357432748,-2.01088345292947,9.74026300248727));
#18687=CARTESIAN_POINT('Ctrl Pts',(1.58249764935552,-1.95969534708922,9.74549956287959));
#18688=CARTESIAN_POINT('Ctrl Pts',(1.64536049606058,-1.90541205202531,9.75073612327192));
#18689=CARTESIAN_POINT('Ctrl Pts',(1.70925223811573,-1.85024028574499,9.75605839204241));
#18690=CARTESIAN_POINT('Ctrl Pts',(1.77034281937465,-1.79187140775071,9.7613806608129));
#18691=CARTESIAN_POINT('Ctrl Pts',(1.82831077523864,-1.73063166478205,9.76670292958339));
#18692=CARTESIAN_POINT('Ctrl Pts',(1.88542713944182,-1.67029157841926,9.77194701033372));
#18693=CARTESIAN_POINT('Ctrl Pts',(1.93951175864186,-1.60716481273136,9.77719109108406));
#18694=CARTESIAN_POINT('Ctrl Pts',(1.9902976907599,-1.54159701354011,9.78243517183439));
#18695=CARTESIAN_POINT('Ctrl Pts',(2.04221943247161,-1.47456281347266,9.78779653461496));
#18696=CARTESIAN_POINT('Ctrl Pts',(2.0906928660034,-1.40497749678828,9.79315789739553));
#18697=CARTESIAN_POINT('Ctrl Pts',(2.13548048945439,-1.33324016184618,9.7985192601761));
#18698=CARTESIAN_POINT('Ctrl Pts',(2.18026811290537,-1.26150282690409,9.80388062295667));
#18699=CARTESIAN_POINT('Ctrl Pts',(2.22136973765147,-1.18761395020763,9.80924198573724));
#18700=CARTESIAN_POINT('Ctrl Pts',(2.2585994704274,-1.11199581032712,9.81460334851781));
#18701=CARTESIAN_POINT('Ctrl Pts',(2.29771370768164,-1.0325500114058,9.82023609418019));
#18702=CARTESIAN_POINT('Ctrl Pts',(2.33268319210186,-0.950935265153575,
9.82586883984257));
#18703=CARTESIAN_POINT('Ctrl Pts',(2.36328009289161,-0.867590601921324,
9.83150158550495));
#18704=CARTESIAN_POINT('Ctrl Pts',(2.39377456178312,-0.784524958846109,
9.83711547393619));
#18705=CARTESIAN_POINT('Ctrl Pts',(2.41992549446168,-0.699741274925882,
9.84272936236742));
#18706=CARTESIAN_POINT('Ctrl Pts',(2.44155272692805,-0.613699056240259,
9.84834325079866));
#18707=CARTESIAN_POINT('Ctrl Pts',(2.46313411560376,-0.527839223417836,
9.85394523932886));
#18708=CARTESIAN_POINT('Ctrl Pts',(2.48021080455436,-0.440726511693493,
9.85954722785906));
#18709=CARTESIAN_POINT('Ctrl Pts',(2.49265158327791,-0.352837546729558,
9.86514921638926));
#18710=CARTESIAN_POINT('Ctrl Pts',(2.50505613088035,-0.265204539676687,
9.87073489031975));
#18711=CARTESIAN_POINT('Ctrl Pts',(2.51285161508252,-0.176800136802324,
9.87632056425024));
#18712=CARTESIAN_POINT('Ctrl Pts',(2.51595758515505,-0.0881117455323095,
9.88190623818073));
#18713=CARTESIAN_POINT('Ctrl Pts',(2.51697896722398,-0.058947030338859,
9.88374305793824));
#18714=CARTESIAN_POINT('Ctrl Pts',(2.51749363732466,-0.0297517030242967,
9.88557987769575));
#18715=CARTESIAN_POINT('Ctrl Pts',(2.51749994136415,-0.000543352107749378,
9.88741669745326));
#18716=CARTESIAN_POINT('Ctrl Pts',(2.51749994136434,-0.000543351237068014,
9.88741669750801));
#18717=CARTESIAN_POINT('Ctrl Pts',(2.51751848517122,0.0853753502565315,
9.89281984980827));
#18718=CARTESIAN_POINT('Ctrl Pts',(2.51313426321878,0.171241900920938,9.89822300210852));
#18719=CARTESIAN_POINT('Ctrl Pts',(2.50438935504415,0.256593469015731,9.90362615440877));
#18720=CARTESIAN_POINT('Ctrl Pts',(2.49563786110501,0.342009315124396,9.90903337580707));
#18721=CARTESIAN_POINT('Ctrl Pts',(2.48251919619281,0.42690899151922,9.91444059720537));
#18722=CARTESIAN_POINT('Ctrl Pts',(2.46512689921235,0.51083815517218,9.91984781860366));
#18723=CARTESIAN_POINT('Ctrl Pts',(2.4477056995384,0.594906793150723,9.92526402577668));
#18724=CARTESIAN_POINT('Ctrl Pts',(2.42599678269746,0.678001290366767,9.93068023294971));
#18725=CARTESIAN_POINT('Ctrl Pts',(2.40014405502514,0.759680699456999,9.93609644012273));
#18726=CARTESIAN_POINT('Ctrl Pts',(2.38812556449347,0.797652058503759,9.93861434211945));
#18727=CARTESIAN_POINT('Ctrl Pts',(2.37521222142059,0.835317852404866,9.94113224411616));
#18728=CARTESIAN_POINT('Ctrl Pts',(2.36142200728636,0.872635292378024,9.94365014611287));
#18729=CARTESIAN_POINT('Ctrl Pts',(2.36142200350084,0.872635302621937,9.67114329893353));
#18730=CARTESIAN_POINT('Ctrl Pts',(2.36647528649717,0.858960708411047,9.67025418119806));
#18731=CARTESIAN_POINT('Ctrl Pts',(2.37141038618732,0.84524060304922,9.66935958559407));
#18732=CARTESIAN_POINT('Ctrl Pts',(2.38200567353762,0.814960969193715,9.6673781273229));
#18733=CARTESIAN_POINT('Ctrl Pts',(2.38761217568937,0.798386165365412,9.66628884452266));
#18734=CARTESIAN_POINT('Ctrl Pts',(2.39564083768089,0.773809467664475,9.66466497258941));
#18735=CARTESIAN_POINT('Ctrl Pts',(2.3981967744251,0.765851383638769,9.66413781212311));
#18736=CARTESIAN_POINT('Ctrl Pts',(2.40267549959039,0.751664280709686,9.6631954002981));
#18737=CARTESIAN_POINT('Ctrl Pts',(2.40461378500539,0.745440333393591,9.66278105239958));
#18738=CARTESIAN_POINT('Ctrl Pts',(2.40878758851222,0.731852326300868,9.66187442319204));
#18739=CARTESIAN_POINT('Ctrl Pts',(2.41101348838801,0.724485630730547,9.66138162264118));
#18740=CARTESIAN_POINT('Ctrl Pts',(2.41714673468343,0.70384611189657,9.6599975922119));
#18741=CARTESIAN_POINT('Ctrl Pts',(2.42097841878177,0.69055134609642,9.65910223427123));
#18742=CARTESIAN_POINT('Ctrl Pts',(2.4427062790222,0.612758194322319,9.65384342587154));
#18743=CARTESIAN_POINT('Ctrl Pts',(2.45813246720599,0.547603584611023,9.64936074260902));
#18744=CARTESIAN_POINT('Ctrl Pts',(2.47571367516164,0.457459342572544,9.6431191754587));
#18745=CARTESIAN_POINT('Ctrl Pts',(2.48012050084405,0.43293129079698,9.64141681910491));
#18746=CARTESIAN_POINT('Ctrl Pts',(2.50623205226357,0.274080932159291,9.63038017599378));
#18747=CARTESIAN_POINT('Ctrl Pts',(2.51738163120652,0.138244323610536,9.62090456378432));
#18748=CARTESIAN_POINT('Ctrl Pts',(2.51760485864111,-0.120416906853857,
9.60326323783957));
#18749=CARTESIAN_POINT('Ctrl Pts',(2.50875650327208,-0.24286425338847,9.59508204491669));
#18750=CARTESIAN_POINT('Ctrl Pts',(2.48785268672985,-0.38584171060584,9.5857661484294));
#18751=CARTESIAN_POINT('Ctrl Pts',(2.48440587041795,-0.407446115295201,
9.5843645552423));
#18752=CARTESIAN_POINT('Ctrl Pts',(2.47824452681829,-0.443073589627441,
9.58206271849662));
#18753=CARTESIAN_POINT('Ctrl Pts',(2.47569155695518,-0.457123034891203,
9.58115745827956));
#18754=CARTESIAN_POINT('Ctrl Pts',(2.47084778377868,-0.482547502159364,
9.57952348346087));
#18755=CARTESIAN_POINT('Ctrl Pts',(2.4685976286522,-0.493929769828765,9.57879350981291));
#18756=CARTESIAN_POINT('Ctrl Pts',(2.46358221713985,-0.518409178853658,
9.57722672792726));
#18757=CARTESIAN_POINT('Ctrl Pts',(2.46079102065578,-0.531500687649627,
9.5763907644777));
#18758=CARTESIAN_POINT('Ctrl Pts',(2.45280735150639,-0.567534699657773,
9.57409477361229));
#18759=CARTESIAN_POINT('Ctrl Pts',(2.44739746577319,-0.59042801509282,9.57264166551865));
#18760=CARTESIAN_POINT('Ctrl Pts',(2.41190258342717,-0.731753281365565,
9.56370021676248));
#18761=CARTESIAN_POINT('Ctrl Pts',(2.37354752347173,-0.847947262627435,
9.55648609280943));
#18762=CARTESIAN_POINT('Ctrl Pts',(2.25344748185044,-1.13877712308217,9.53823408636118));
#18763=CARTESIAN_POINT('Ctrl Pts',(2.15985212332765,-1.30761718702181,9.52746597225172));
#18764=CARTESIAN_POINT('Ctrl Pts',(2.02411131459663,-1.49748476011527,9.51342044063668));
#18765=CARTESIAN_POINT('Ctrl Pts',(1.99945698954969,-1.53024786608671,9.51091667554503));
#18766=CARTESIAN_POINT('Ctrl Pts',(1.96655721170996,-1.57181532065612,9.50761382938489));
#18767=CARTESIAN_POINT('Ctrl Pts',(1.95903182517084,-1.58118467097132,9.50686081084206));
#18768=CARTESIAN_POINT('Ctrl Pts',(1.94688227215881,-1.5960913846239,9.50564833237535));
#18769=CARTESIAN_POINT('Ctrl Pts',(1.94230077535962,-1.60166350543643,9.50519184247834));
#18770=CARTESIAN_POINT('Ctrl Pts',(1.93346296805035,-1.61231856456575,9.50431247896849));
#18771=CARTESIAN_POINT('Ctrl Pts',(1.92921045667836,-1.61740446772248,9.5038898703138));
#18772=CARTESIAN_POINT('Ctrl Pts',(1.91899165868033,-1.62952827332452,9.50287566674407));
#18773=CARTESIAN_POINT('Ctrl Pts',(1.91300670647945,-1.63655024801305,9.5022827436402));
#18774=CARTESIAN_POINT('Ctrl Pts',(1.89237474955293,-1.66048932011846,9.50024289352669));
#18775=CARTESIAN_POINT('Ctrl Pts',(1.87754133671617,-1.67724339985583,9.49878340026861));
#18776=CARTESIAN_POINT('Ctrl Pts',(1.84065176452078,-1.71780691631435,9.49517552673694));
#18777=CARTESIAN_POINT('Ctrl Pts',(1.81835510221512,-1.74139140984504,9.49301330961599));
#18778=CARTESIAN_POINT('Ctrl Pts',(1.72456112953382,-1.83683705395011,9.48401518329662));
#18779=CARTESIAN_POINT('Ctrl Pts',(1.64921433424445,-1.90477591919613,9.4770169628648));
#18780=CARTESIAN_POINT('Ctrl Pts',(1.42058328305293,-2.08716902275808,9.45681124159363));
#18781=CARTESIAN_POINT('Ctrl Pts',(1.25807071934463,-2.18897577772168,9.44371043134116));
#18782=CARTESIAN_POINT('Ctrl Pts',(1.0565366857585,-2.28529482016103,9.42920589262093));
#18783=CARTESIAN_POINT('Ctrl Pts',(1.02723239650116,-2.29861609313234,9.42713464951643));
#18784=CARTESIAN_POINT('Ctrl Pts',(0.983936707440413,-2.31730422255812,
9.42412808951916));
#18785=CARTESIAN_POINT('Ctrl Pts',(0.970140987699629,-2.32311359685462,
9.42317791603781));
#18786=CARTESIAN_POINT('Ctrl Pts',(0.945473031784617,-2.33324320098661,
9.42149257642528));
#18787=CARTESIAN_POINT('Ctrl Pts',(0.934621051643274,-2.33761129918285,
9.42075582081989));
#18788=CARTESIAN_POINT('Ctrl Pts',(0.91182235817537,-2.34660400016268,9.41921755632303));
#18789=CARTESIAN_POINT('Ctrl Pts',(0.899869973409208,-2.35121338611812,
9.41841657206057));
#18790=CARTESIAN_POINT('Ctrl Pts',(0.868350149360071,-2.36309330922198,
9.41631827705893));
#18791=CARTESIAN_POINT('Ctrl Pts',(0.84872630732279,-2.37021215628358,9.41502600050449));
#18792=CARTESIAN_POINT('Ctrl Pts',(0.755643087744054,-2.40267519880789,
9.408959491603));
#18793=CARTESIAN_POINT('Ctrl Pts',(0.68112061180335,-2.4248548493827,9.40428917165514));
#18794=CARTESIAN_POINT('Ctrl Pts',(0.471279965914689,-2.47686822272979,
9.39151656271789));
#18795=CARTESIAN_POINT('Ctrl Pts',(0.334354027909021,-2.49903792946427,
9.38361897000609));
#18796=CARTESIAN_POINT('Ctrl Pts',(0.0682992559190702,-2.51984613277134,
9.36825909323298));
#18797=CARTESIAN_POINT('Ctrl Pts',(-0.0602596597745309,-2.52004962292166,
9.36082403409335));
#18798=CARTESIAN_POINT('Ctrl Pts',(-0.209695469693848,-2.5088436209334,
9.35162236078788));
#18799=CARTESIAN_POINT('Ctrl Pts',(-0.231113078438273,-2.50696134362511,
9.35028989132003));
#18800=CARTESIAN_POINT('Ctrl Pts',(-0.260898589216307,-2.50395874093345,
9.34841453336676));
#18801=CARTESIAN_POINT('Ctrl Pts',(-0.269289608415433,-2.50307022517838,
9.34788374802464));
#18802=CARTESIAN_POINT('Ctrl Pts',(-0.283754538422571,-2.50146497423133,
9.34696424379794));
#18803=CARTESIAN_POINT('Ctrl Pts',(-0.289830659632837,-2.50076825039936,
9.34657662481538));
#18804=CARTESIAN_POINT('Ctrl Pts',(-0.302640411658805,-2.49925209708182,
9.34575643084977));
#18805=CARTESIAN_POINT('Ctrl Pts',(-0.30937334052923,-2.4984275847554,9.3453235659978));
#18806=CARTESIAN_POINT('Ctrl Pts',(-0.326065202312927,-2.49631499905286,
9.34424619443894));
#18807=CARTESIAN_POINT('Ctrl Pts',(-0.336019840392307,-2.4949945389553,
9.34359992777618));
#18808=CARTESIAN_POINT('Ctrl Pts',(-0.373490671937523,-2.489795805394,9.34115382234958));
#18809=CARTESIAN_POINT('Ctrl Pts',(-0.40094879961149,-2.48552174476235,
9.33933398619751));
#18810=CARTESIAN_POINT('Ctrl Pts',(-0.471241468160891,-2.47338514778306,
9.3346142417374));
#18811=CARTESIAN_POINT('Ctrl Pts',(-0.513951969853503,-2.46486420674446,
9.33168805280143));
#18812=CARTESIAN_POINT('Ctrl Pts',(-0.678094326570187,-2.42766553885441,
9.32026622024919));
#18813=CARTESIAN_POINT('Ctrl Pts',(-0.797549924505594,-2.39108445777432,
9.31158751774704));
#18814=CARTESIAN_POINT('Ctrl Pts',(-1.06418579753438,-2.28721729995606,
9.29188638077167));
#18815=CARTESIAN_POINT('Ctrl Pts',(-1.20861318502091,-2.21430021351207,
9.28098607830016));
#18816=CARTESIAN_POINT('Ctrl Pts',(-1.36387873701221,-2.11616053669732,
9.26913929669441));
#18817=CARTESIAN_POINT('Ctrl Pts',(-1.38251586653006,-2.10403197621247,
9.26771431510549));
#18818=CARTESIAN_POINT('Ctrl Pts',(-1.41294464344692,-2.08365081064173,
9.26538225755767));
#18819=CARTESIAN_POINT('Ctrl Pts',(-1.42483025333498,-2.07554138222043,
9.2644699334336));
#18820=CARTESIAN_POINT('Ctrl Pts',(-1.4461794875036,-2.06070520020931,9.26282839194581));
#18821=CARTESIAN_POINT('Ctrl Pts',(-1.45566726714951,-2.05401408146994,
9.26209786105712));
#18822=CARTESIAN_POINT('Ctrl Pts',(-1.47592777422095,-2.03951476105089,
9.2605354957455));
#18823=CARTESIAN_POINT('Ctrl Pts',(-1.48668561076329,-2.0316862850355,9.25970446295303));
#18824=CARTESIAN_POINT('Ctrl Pts',(-1.51598794405718,-2.01000561064165,
9.25743648623442));
#18825=CARTESIAN_POINT('Ctrl Pts',(-1.53440454389709,-1.99598215220301,
9.25600617898162));
#18826=CARTESIAN_POINT('Ctrl Pts',(-1.64199400105456,-1.91168805488362,
9.24761594437005));
#18827=CARTESIAN_POINT('Ctrl Pts',(-1.72652968751229,-1.83570023815874,
9.24089007994945));
#18828=CARTESIAN_POINT('Ctrl Pts',(-1.93011070794262,-1.62615445052017,
9.2238949945278));
#18829=CARTESIAN_POINT('Ctrl Pts',(-2.04057104403988,-1.48518259249948,
9.21387226123886));
#18830=CARTESIAN_POINT('Ctrl Pts',(-2.16755882729801,-1.28188547036864,
9.19966778960911));
#18831=CARTESIAN_POINT('Ctrl Pts',(-2.19803665636954,-1.22889185391841,
9.19598147762745));
#18832=CARTESIAN_POINT('Ctrl Pts',(-2.23285443790405,-1.16290567150141,
9.19134629950591));
#18833=CARTESIAN_POINT('Ctrl Pts',(-2.23905890469332,-1.15091430795047,
9.19050219506075));
#18834=CARTESIAN_POINT('Ctrl Pts',(-2.2486137045485,-1.13207805610502,9.18917258768684));
#18835=CARTESIAN_POINT('Ctrl Pts',(-2.25203002396736,-1.12526667280146,
9.18869104303722));
#18836=CARTESIAN_POINT('Ctrl Pts',(-2.25831535986996,-1.11259183735401,
9.18779339612274));
#18837=CARTESIAN_POINT('Ctrl Pts',(-2.26119254661947,-1.10673263479187,
9.18737780295553));
#18838=CARTESIAN_POINT('Ctrl Pts',(-2.26774814163521,-1.09325031810593,
9.18642007424008));
#18839=CARTESIAN_POINT('Ctrl Pts',(-2.27141090503754,-1.08561981718363,
9.18587700757643));
#18840=CARTESIAN_POINT('Ctrl Pts',(-2.28276421040053,-1.06165890845496,
9.18416882368802));
#18841=CARTESIAN_POINT('Ctrl Pts',(-2.2903174427038,-1.045264581713,9.18299590420926));
#18842=CARTESIAN_POINT('Ctrl Pts',(-2.30769523368822,-1.006453164976,9.18021182397249));
#18843=CARTESIAN_POINT('Ctrl Pts',(-2.31737033072852,-0.983971504344939,
9.17859343360965));
#18844=CARTESIAN_POINT('Ctrl Pts',(-2.35122667259248,-0.902030675932925,
9.17268311619013));
#18845=CARTESIAN_POINT('Ctrl Pts',(-2.37345837403282,-0.841795996271935,
9.16831702166189));
#18846=CARTESIAN_POINT('Ctrl Pts',(-2.46056393453768,-0.57478775683513,
9.14904439575039));
#18847=CARTESIAN_POINT('Ctrl Pts',(-2.50090218333311,-0.360934568481369,
9.13392261081604));
#18848=CARTESIAN_POINT('Ctrl Pts',(-2.51621659285148,-0.0946480917806868,
9.11636057837711));
#18849=CARTESIAN_POINT('Ctrl Pts',(-2.51759985243393,-0.0446739804134837,
9.11311295916028));
#18850=CARTESIAN_POINT('Ctrl Pts',(-2.51745537497348,0.0238076706712868,
9.10872606252561));
#18851=CARTESIAN_POINT('Ctrl Pts',(-2.51721250838459,0.0423035177186008,
9.10754752802467));
#18852=CARTESIAN_POINT('Ctrl Pts',(-2.51649851536062,0.071860896210121,
9.10567385069298));
#18853=CARTESIAN_POINT('Ctrl Pts',(-2.51615823793766,0.0829246297629913,
9.10497467621193));
#18854=CARTESIAN_POINT('Ctrl Pts',(-2.51530563904789,0.105746364648813,
9.10353679445947));
#18855=CARTESIAN_POINT('Ctrl Pts',(-2.51478381303445,0.11750375613942,9.10279840022273));
#18856=CARTESIAN_POINT('Ctrl Pts',(-2.5133729325225,0.144946764559623,9.10108025546161));
#18857=CARTESIAN_POINT('Ctrl Pts',(-2.51241945238621,0.160628687832301,
9.10010252865361));
#18858=CARTESIAN_POINT('Ctrl Pts',(-2.50884053422694,0.211608596524839,
9.0969365402307));
#18859=CARTESIAN_POINT('Ctrl Pts',(-2.5056174318732,0.246861294623273,9.09476679857245));
#18860=CARTESIAN_POINT('Ctrl Pts',(-2.49621109839028,0.330295316195898,
9.08966948436537));
#18861=CARTESIAN_POINT('Ctrl Pts',(-2.48937477757095,0.378389317816642,
9.08676150987123));
#18862=CARTESIAN_POINT('Ctrl Pts',(-2.45705712119158,0.566503203603238,
9.07545818720507));
#18863=CARTESIAN_POINT('Ctrl Pts',(-2.42111584204072,0.704454558995143,
9.06734073357711));
#18864=CARTESIAN_POINT('Ctrl Pts',(-2.33044484490683,0.961093584693852,
9.05167764437746));
#18865=CARTESIAN_POINT('Ctrl Pts',(-2.27777380867821,1.08000569399528,9.04416119415918));
#18866=CARTESIAN_POINT('Ctrl Pts',(-2.20600614343839,1.21317873033923,9.03487128724458));
#18867=CARTESIAN_POINT('Ctrl Pts',(-2.19559681376915,1.23191732585953,9.03354273440847));
#18868=CARTESIAN_POINT('Ctrl Pts',(-2.18076376038303,1.25783412720895,9.03167203003952));
#18869=CARTESIAN_POINT('Ctrl Pts',(-2.17654100742291,1.26512707204384,9.03114190354894));
#18870=CARTESIAN_POINT('Ctrl Pts',(-2.16919200583589,1.2776735357655,9.03022322825833));
#18871=CARTESIAN_POINT('Ctrl Pts',(-2.16608305925666,1.28293717721042,9.029835774703));
#18872=CARTESIAN_POINT('Ctrl Pts',(-2.15948246982475,1.29402000265873,9.02901554712703));
#18873=CARTESIAN_POINT('Ctrl Pts',(-2.15598643163422,1.29983645431076,9.02858248085474));
#18874=CARTESIAN_POINT('Ctrl Pts',(-2.14725130437121,1.31423712621905,9.02750394744237));
#18875=CARTESIAN_POINT('Ctrl Pts',(-2.14198425381999,1.32280415644471,9.026856712368));
#18876=CARTESIAN_POINT('Ctrl Pts',(-2.12191414031491,1.35501467859251,9.02440265018545));
#18877=CARTESIAN_POINT('Ctrl Pts',(-2.10677038056677,1.37844216744733,9.02257566225857));
#18878=CARTESIAN_POINT('Ctrl Pts',(-2.06686679234994,1.43797934977472,9.01783294180737));
#18879=CARTESIAN_POINT('Ctrl Pts',(-2.04154913447083,1.47370269999305,9.01489062913552));
#18880=CARTESIAN_POINT('Ctrl Pts',(-1.94098394497538,1.60803314905606,9.00350092381855));
#18881=CARTESIAN_POINT('Ctrl Pts',(-1.85941964624749,1.70168938276722,8.99487407572329));
#18882=CARTESIAN_POINT('Ctrl Pts',(-1.65634442356775,1.90275946961818,8.97519755968456));
#18883=CARTESIAN_POINT('Ctrl Pts',(-1.53068343962811,2.00524204004788,8.96427178441155));
#18884=CARTESIAN_POINT('Ctrl Pts',(-1.3775310629047,2.10729894338544,8.95240175599791));
#18885=CARTESIAN_POINT('Ctrl Pts',(-1.35886453264704,2.11938384908532,8.95097671612602));
#18886=CARTESIAN_POINT('Ctrl Pts',(-1.32785922870589,2.13887894530634,8.9486445833152));
#18887=CARTESIAN_POINT('Ctrl Pts',(-1.31561298142216,2.14643326731657,8.94773224162875));
#18888=CARTESIAN_POINT('Ctrl Pts',(-1.29336968011474,2.15989256752792,8.94609068123867));
#18889=CARTESIAN_POINT('Ctrl Pts',(-1.28339534123931,2.16583412062632,8.94536014887469));
#18890=CARTESIAN_POINT('Ctrl Pts',(-1.26190338659983,2.17843592812391,8.94379779410433));
#18891=CARTESIAN_POINT('Ctrl Pts',(-1.25037331743632,2.1850743300599,8.94296677322355));
#18892=CARTESIAN_POINT('Ctrl Pts',(-1.21864165675435,2.20301032040406,8.94069886408962));
#18893=CARTESIAN_POINT('Ctrl Pts',(-1.19833572564897,2.21412138396209,8.93926861183428));
#18894=CARTESIAN_POINT('Ctrl Pts',(-1.07755813055978,2.27806048868268,8.93087961563217));
#18895=CARTESIAN_POINT('Ctrl Pts',(-0.97375375064002,2.32432772078794,8.92415484864632));
#18896=CARTESIAN_POINT('Ctrl Pts',(-0.699660671073356,2.42489545454157,
8.9071709802723));
#18897=CARTESIAN_POINT('Ctrl Pts',(-0.526105877073629,2.46836941257501,
8.89715763916029));
#18898=CARTESIAN_POINT('Ctrl Pts',(-0.288725520143927,2.50163963086478,
8.88295474023484));
#18899=CARTESIAN_POINT('Ctrl Pts',(-0.227738993692051,2.50792681547114,
8.8792581440627));
#18900=CARTESIAN_POINT('Ctrl Pts',(-0.153106759390012,2.51287627091878,
8.87461140114671));
#18901=CARTESIAN_POINT('Ctrl Pts',(-0.139617424933388,2.51366182860446,
8.87376663474007));
#18902=CARTESIAN_POINT('Ctrl Pts',(-0.118509703675461,2.51472062160851,
8.87243620682553));
#18903=CARTESIAN_POINT('Ctrl Pts',(-0.110895061522468,2.51506791882549,
8.87195451148787));
#18904=CARTESIAN_POINT('Ctrl Pts',(-0.0967571706041103,2.51564840685909,
8.8710567355929));
#18905=CARTESIAN_POINT('Ctrl Pts',(-0.0902344779359328,2.51589081492491,
8.87064116550925));
#18906=CARTESIAN_POINT('Ctrl Pts',(-0.0752550135229502,2.51638918190434,
8.86968369008033));
#18907=CARTESIAN_POINT('Ctrl Pts',(-0.0667978660740206,2.51662787714356,
8.86914085547557));
#18908=CARTESIAN_POINT('Ctrl Pts',(-0.0403127116606915,2.51724180138517,
8.86743412475642));
#18909=CARTESIAN_POINT('Ctrl Pts',(-0.0222822324136588,2.51746595996093,
8.86626244474766));
#18910=CARTESIAN_POINT('Ctrl Pts',(0.143554973629019,2.51774602412938,8.85540526024625));
#18911=CARTESIAN_POINT('Ctrl Pts',(0.291081968688955,2.50497823205498,8.84517579275143));
#18912=CARTESIAN_POINT('Ctrl Pts',(0.616535904009861,2.44766481881102,8.82234712184223));
#18913=CARTESIAN_POINT('Ctrl Pts',(0.792498801616777,2.39648652812175,8.80985292243285));
#18914=CARTESIAN_POINT('Ctrl Pts',(0.99125811164431,2.31435903973819,8.79588161340696));
#18915=CARTESIAN_POINT('Ctrl Pts',(1.02088323978874,2.30144475881326,8.79380125819369));
#18916=CARTESIAN_POINT('Ctrl Pts',(1.06408309181307,2.2816145618581,8.79076943099895));
#18917=CARTESIAN_POINT('Ctrl Pts',(1.07785588910503,2.27514055259541,8.78980309679165));
#18918=CARTESIAN_POINT('Ctrl Pts',(1.10214299834276,2.2634541629803,8.78809925320576));
#18919=CARTESIAN_POINT('Ctrl Pts',(1.11268105097236,2.25829245737752,8.78736003131039));
#18920=CARTESIAN_POINT('Ctrl Pts',(1.12409118435183,2.25260433488596,8.78655961864032));
#18921=CARTESIAN_POINT('Ctrl Pts',(1.12499932023364,2.25215092961444,8.78649591344023));
#18922=CARTESIAN_POINT('Ctrl Pts',(1.1263128507283,2.25149413012709,8.7864037697891));
#18923=CARTESIAN_POINT('Ctrl Pts',(1.12671846412425,2.25129117581764,8.78637531613239));
#18924=CARTESIAN_POINT('Ctrl Pts',(1.12742881301269,2.25093550280219,8.7863254853022));
#18925=CARTESIAN_POINT('Ctrl Pts',(1.12773357228416,2.25078283184539,8.78630410647829));
#18926=CARTESIAN_POINT('Ctrl Pts',(1.12826688649127,2.2505155294343,8.78626669451087));
#18927=CARTESIAN_POINT('Ctrl Pts',(1.12849545493568,2.25040092507252,8.78625066043071));
#18928=CARTESIAN_POINT('Ctrl Pts',(1.12889521767398,2.25020040756404,8.78622261704161));
#18929=CARTESIAN_POINT('Ctrl Pts',(1.12906641960202,2.25011450971181,8.78621060720375));
#18930=CARTESIAN_POINT('Ctrl Pts',(1.1294752501352,2.24990932706814,8.78618192766668));
#18931=CARTESIAN_POINT('Ctrl Pts',(1.12971286968457,2.24979002415011,8.78616525859452));
#18932=CARTESIAN_POINT('Ctrl Pts',(1.13017394099946,2.24955844014407,8.78613291428865));
#18933=CARTESIAN_POINT('Ctrl Pts',(1.1303973949333,2.24944616340684,8.78611723890492));
#18934=CARTESIAN_POINT('Ctrl Pts',(1.14249592626669,2.24336487336437,8.78526852112721));
#18935=CARTESIAN_POINT('Ctrl Pts',(1.15432374146975,2.2373018587586,8.78443874808158));
#18936=CARTESIAN_POINT('Ctrl Pts',(1.17870949822711,2.22455669715852,8.78272758794073));
#18937=CARTESIAN_POINT('Ctrl Pts',(1.19125995464662,2.21786120246362,8.78184669868728));
#18938=CARTESIAN_POINT('Ctrl Pts',(1.22305860582782,2.20054926384951,8.77961375049276));
#18939=CARTESIAN_POINT('Ctrl Pts',(1.24222597306976,2.18978631220626,8.77826678855427));
#18940=CARTESIAN_POINT('Ctrl Pts',(1.29744087969792,2.15782345617162,8.77438118290696));
#18941=CARTESIAN_POINT('Ctrl Pts',(1.33310509646883,2.13597424694994,8.77186467606242));
#18942=CARTESIAN_POINT('Ctrl Pts',(1.46011798923064,2.05374041427202,8.76285075555961));
#18943=CARTESIAN_POINT('Ctrl Pts',(1.54805083334395,1.98829961667938,8.75651649192456));
#18944=CARTESIAN_POINT('Ctrl Pts',(1.76742019693579,1.80164002657368,8.73994808503236));
#18945=CARTESIAN_POINT('Ctrl Pts',(1.89068018109402,1.67182264800081,8.72983492149918));
#18946=CARTESIAN_POINT('Ctrl Pts',(2.01094565721828,1.51468805641451,8.71764825393113));
#18947=CARTESIAN_POINT('Ctrl Pts',(2.02255368985017,1.4991527151326,8.71644364097489));
#18948=CARTESIAN_POINT('Ctrl Pts',(2.03868002113719,1.47704218623548,8.71472709788236));
#18949=CARTESIAN_POINT('Ctrl Pts',(2.04334864771464,1.47057680803253,8.71422491221487));
#18950=CARTESIAN_POINT('Ctrl Pts',(2.05182602342918,1.45871855028654,8.71330317408219));
#18951=CARTESIAN_POINT('Ctrl Pts',(2.05564446880157,1.45333260347049,8.71288427349661));
#18952=CARTESIAN_POINT('Ctrl Pts',(2.06353024875123,1.44211639502942,8.71201126415512));
#18953=CARTESIAN_POINT('Ctrl Pts',(2.06759411238707,1.43628387436127,8.71155694431904));
#18954=CARTESIAN_POINT('Ctrl Pts',(2.07819162105292,1.42093598299914,8.71036068927252));
#18955=CARTESIAN_POINT('Ctrl Pts',(2.08468453412916,1.4113928803266,8.70961613097328));
#18956=CARTESIAN_POINT('Ctrl Pts',(2.11381248734533,1.36794192493528,8.7062239307294));
#18957=CARTESIAN_POINT('Ctrl Pts',(2.13568612176331,1.33353391000531,8.70353193338342));
#18958=CARTESIAN_POINT('Ctrl Pts',(2.19605388452002,1.23327616511136,8.69570440061242));
#18959=CARTESIAN_POINT('Ctrl Pts',(2.23240280724681,1.16618994237024,8.69048738157978));
#18960=CARTESIAN_POINT('Ctrl Pts',(2.301214376549,1.0241453178954,8.67961586955767));
#18961=CARTESIAN_POINT('Ctrl Pts',(2.3331728339198,0.949079813084719,8.67396572716839));
#18962=CARTESIAN_POINT('Ctrl Pts',(2.36142186693781,0.872635672172493,8.66836043115426));
#18963=CARTESIAN_POINT('Origin',(0.,0.,10.));
#18964=CARTESIAN_POINT('',(2.36142200378576,0.872635301850924,7.66684133937673));
#18965=CARTESIAN_POINT('',(2.36142200728636,0.872635292378021,7.94384568391999));
#18966=CARTESIAN_POINT('',(2.36142200728636,0.87263529237802,10.));
#18967=CARTESIAN_POINT('',(2.51749930935125,-0.0018647830938552,8.88741669754404));
#18968=CARTESIAN_POINT('Ctrl Pts',(2.36142200728636,0.872635292378021,7.94384568391999));
#18969=CARTESIAN_POINT('Ctrl Pts',(2.33203545559993,0.952157689050145,7.94920817054382));
#18970=CARTESIAN_POINT('Ctrl Pts',(2.29859309494399,1.030287126504,7.95457065716764));
#18971=CARTESIAN_POINT('Ctrl Pts',(2.26125522707057,1.10658530988173,7.95993314379147));
#18972=CARTESIAN_POINT('Ctrl Pts',(2.22477931807968,1.18112212067366,7.96517183537179));
#18973=CARTESIAN_POINT('Ctrl Pts',(2.18458604395432,1.25391088226474,7.97041052695211));
#18974=CARTESIAN_POINT('Ctrl Pts',(2.1408736952347,1.32456259612451,7.97564921853243));
#18975=CARTESIAN_POINT('Ctrl Pts',(2.09717707316596,1.39518889119829,7.98088602535762));
#18976=CARTESIAN_POINT('Ctrl Pts',(2.04996413340203,1.46367927342139,7.98612283218281));
#18977=CARTESIAN_POINT('Ctrl Pts',(1.99947825686152,1.52967086340101,7.991359639008));
#18978=CARTESIAN_POINT('Ctrl Pts',(1.9489953151362,1.59565861719648,7.99659614141023));
#18979=CARTESIAN_POINT('Ctrl Pts',(1.89524009579892,1.65914750149198,8.00183264381245));
#18980=CARTESIAN_POINT('Ctrl Pts',(1.83849746441907,1.71980618772136,8.00706914621468));
#18981=CARTESIAN_POINT('Ctrl Pts',(1.77937255397181,1.78301156441867,8.01252549760445));
#18982=CARTESIAN_POINT('Ctrl Pts',(1.7170042125162,1.8431434499418,8.01798184899421));
#18983=CARTESIAN_POINT('Ctrl Pts',(1.65175734424917,1.89986944965146,8.02343820038398));
#18984=CARTESIAN_POINT('Ctrl Pts',(1.58905159374907,1.95438618706949,8.0286820476057));
#18985=CARTESIAN_POINT('Ctrl Pts',(1.52368778151637,2.0057571609586,8.03392589482741));
#18986=CARTESIAN_POINT('Ctrl Pts',(1.45602219672215,2.0537296834424,8.03916974204913));
#18987=CARTESIAN_POINT('Ctrl Pts',(1.38830887220202,2.10173605171473,8.04441728893338));
#18988=CARTESIAN_POINT('Ctrl Pts',(1.31829093226679,2.14633895037898,8.04966483581763));
#18989=CARTESIAN_POINT('Ctrl Pts',(1.24635127519451,2.18733050744989,8.05491238270188));
#18990=CARTESIAN_POINT('Ctrl Pts',(1.17430060942845,2.2283853177999,8.06016802697426));
#18991=CARTESIAN_POINT('Ctrl Pts',(1.10032272263448,2.26581746540645,8.06542367124664));
#18992=CARTESIAN_POINT('Ctrl Pts',(1.02482191817686,2.29946652204904,8.07067931551902));
#18993=CARTESIAN_POINT('Ctrl Pts',(1.01588625012767,2.30344895379247,8.07130133130998));
#18994=CARTESIAN_POINT('Ctrl Pts',(1.00692926837676,2.30737845228083,8.07192334710093));
#18995=CARTESIAN_POINT('Ctrl Pts',(0.997951656853134,2.31125479784988,8.07254536289189));
#18996=CARTESIAN_POINT('Ctrl Pts',(0.922102155402338,2.34400503192823,8.0778006122992));
#18997=CARTESIAN_POINT('Ctrl Pts',(0.844498702622624,2.37307800987226,8.08305586170651));
#18998=CARTESIAN_POINT('Ctrl Pts',(0.765532238206542,2.39828410374302,8.08831111111381));
#18999=CARTESIAN_POINT('Ctrl Pts',(0.686677730298033,2.4234544610988,8.09355890977131));
#19000=CARTESIAN_POINT('Ctrl Pts',(0.606464485047739,2.44476868481441,8.0988067084288));
#19001=CARTESIAN_POINT('Ctrl Pts',(0.52530418316165,2.46208484117686,8.10405450708629));
#19002=CARTESIAN_POINT('Ctrl Pts',(0.443555804919887,2.47952646802045,8.1093403305692));
#19003=CARTESIAN_POINT('Ctrl Pts',(0.360847022713483,2.49291165629838,8.11462615405211));
#19004=CARTESIAN_POINT('Ctrl Pts',(0.277614991356014,2.50214631198385,8.11991197753501));
#19005=CARTESIAN_POINT('Ctrl Pts',(0.195129295878602,2.51129816114922,8.12515040340361));
#19006=CARTESIAN_POINT('Ctrl Pts',(0.112130164601205,2.51637356285531,8.1303888292722));
#19007=CARTESIAN_POINT('Ctrl Pts',(0.0290524157150399,2.5173323592925,8.13562725514079));
#19008=CARTESIAN_POINT('Ctrl Pts',(-0.0539980102821334,2.51829084039749,
8.14086395817829));
#19009=CARTESIAN_POINT('Ctrl Pts',(-0.137126541510563,2.51513539979878,
8.14610066121579));
#19010=CARTESIAN_POINT('Ctrl Pts',(-0.219896386140231,2.50787795344241,
8.1513373642533));
#19011=CARTESIAN_POINT('Ctrl Pts',(-0.302663976160698,2.50062070477524,
8.15657392464563));
#19012=CARTESIAN_POINT('Ctrl Pts',(-0.385072439441506,2.48926171384237,
8.16181048503796));
#19013=CARTESIAN_POINT('Ctrl Pts',(-0.46668952830822,2.47386481727831,8.16704704543029));
#19014=CARTESIAN_POINT('Ctrl Pts',(-0.549642468915775,2.45821591502079,
8.17236931420076));
#19015=CARTESIAN_POINT('Ctrl Pts',(-0.631777410420044,2.438395813585,8.17769158297124));
#19016=CARTESIAN_POINT('Ctrl Pts',(-0.712652561784477,2.41452533144343,
8.18301385174172));
#19017=CARTESIAN_POINT('Ctrl Pts',(-0.792339598035419,2.39100552413982,
8.18825793249206));
#19018=CARTESIAN_POINT('Ctrl Pts',(-0.870803191428158,2.36355376477676,
8.19350201324239));
#19019=CARTESIAN_POINT('Ctrl Pts',(-0.947638970692298,2.33233501693587,
8.19874609399272));
#19020=CARTESIAN_POINT('Ctrl Pts',(-1.02619315526228,2.30041807272806,8.20410745677328));
#19021=CARTESIAN_POINT('Ctrl Pts',(-1.1030453720849,2.26456382854647,8.20946881955383));
#19022=CARTESIAN_POINT('Ctrl Pts',(-1.17778988319318,2.22499825641455,8.21483018233438));
#19023=CARTESIAN_POINT('Ctrl Pts',(-1.25253439430145,2.18543268428264,8.22019154511493));
#19024=CARTESIAN_POINT('Ctrl Pts',(-1.32517079737989,2.14215610165391,8.22555290789549));
#19025=CARTESIAN_POINT('Ctrl Pts',(-1.39532635611374,2.09544043340162,8.23091427067604));
#19026=CARTESIAN_POINT('Ctrl Pts',(-1.46409337926548,2.04964937281807,8.23616952008335));
#19027=CARTESIAN_POINT('Ctrl Pts',(-1.53073088988013,2.00038502354856,8.24142476949065));
#19028=CARTESIAN_POINT('Ctrl Pts',(-1.59486698177955,1.94787205956381,8.24668001889796));
#19029=CARTESIAN_POINT('Ctrl Pts',(-1.65891214327062,1.8954335470325,8.25192781755545));
#19030=CARTESIAN_POINT('Ctrl Pts',(-1.72046257628046,1.83975585812135,8.25717561621295));
#19031=CARTESIAN_POINT('Ctrl Pts',(-1.77917508770257,1.78110703139888,8.26242341487044));
#19032=CARTESIAN_POINT('Ctrl Pts',(-1.83831302188613,1.72203324336552,8.26770923835335));
#19033=CARTESIAN_POINT('Ctrl Pts',(-1.89457134013327,1.65994534158663,8.27299506183626));
#19034=CARTESIAN_POINT('Ctrl Pts',(-1.94763310747957,1.59515877850748,8.27828088531916));
#19035=CARTESIAN_POINT('Ctrl Pts',(-2.00021907362067,1.53095315206756,8.28351931118776));
#19036=CARTESIAN_POINT('Ctrl Pts',(-2.04966528800478,1.46409743145697,8.28875773705635));
#19037=CARTESIAN_POINT('Ctrl Pts',(-2.09570132912801,1.39493447483784,8.29399616292494));
#19038=CARTESIAN_POINT('Ctrl Pts',(-2.14172222976347,1.32579426476408,8.29923286596245));
#19039=CARTESIAN_POINT('Ctrl Pts',(-2.1843349291271,1.25434870953135,8.30446956899995));
#19040=CARTESIAN_POINT('Ctrl Pts',(-2.2233116102288,1.1809706744123,8.30970627203746));
#19041=CARTESIAN_POINT('Ctrl Pts',(-2.26228722962518,1.10759463807426,8.31494283242979));
#19042=CARTESIAN_POINT('Ctrl Pts',(-2.29762681213926,1.03228663449532,8.32017939282212));
#19043=CARTESIAN_POINT('Ctrl Pts',(-2.32914856552648,0.955443985645375,
8.32541595321445));
#19044=CARTESIAN_POINT('Ctrl Pts',(-2.36118624504783,0.877343629767864,
8.33073822198493));
#19045=CARTESIAN_POINT('Ctrl Pts',(-2.38927979398977,0.797658389323468,
8.33606049075541));
#19046=CARTESIAN_POINT('Ctrl Pts',(-2.41329002013544,0.716824615031257,
8.3413827595259));
#19047=CARTESIAN_POINT('Ctrl Pts',(-2.43694751850155,0.6371783479931,8.34662684027623));
#19048=CARTESIAN_POINT('Ctrl Pts',(-2.4566408204405,0.556417537949075,8.35187092102657));
#19049=CARTESIAN_POINT('Ctrl Pts',(-2.47228813556247,0.474971183080658,
8.3571150017769));
#19050=CARTESIAN_POINT('Ctrl Pts',(-2.4882853974096,0.391703308996976,8.36247636455746));
#19051=CARTESIAN_POINT('Ctrl Pts',(-2.50005344341738,0.307719363212413,
8.36783772733801));
#19052=CARTESIAN_POINT('Ctrl Pts',(-2.50756091250626,0.223482706424399,
8.37319909011857));
#19053=CARTESIAN_POINT('Ctrl Pts',(-2.51506838159514,0.139246049636391,
8.37856045289912));
#19054=CARTESIAN_POINT('Ctrl Pts',(-2.51831532100137,0.0547571921421189,
8.38392181567968));
#19055=CARTESIAN_POINT('Ctrl Pts',(-2.51732688234237,-0.0295231677914636,
8.38928317846023));
#19056=CARTESIAN_POINT('Ctrl Pts',(-2.5163580070975,-0.112135430702491,
8.39453842786754));
#19057=CARTESIAN_POINT('Ctrl Pts',(-2.51131634767356,-0.194852512373203,
8.39979367727485));
#19058=CARTESIAN_POINT('Ctrl Pts',(-2.50218787396462,-0.277240136676509,
8.40504892668215));
#19059=CARTESIAN_POINT('Ctrl Pts',(-2.49307234235767,-0.359510954044777,
8.41029672533965));
#19060=CARTESIAN_POINT('Ctrl Pts',(-2.47988155577698,-0.441452787045854,
8.41554452399715));
#19061=CARTESIAN_POINT('Ctrl Pts',(-2.46265349088341,-0.522631833932614,
8.42079232265464));
#19062=CARTESIAN_POINT('Ctrl Pts',(-2.44530059380733,-0.604399092998672,
8.42607814613755));
#19063=CARTESIAN_POINT('Ctrl Pts',(-2.42385166998306,-0.685391991366873,
8.43136396962046));
#19064=CARTESIAN_POINT('Ctrl Pts',(-2.39839876275192,-0.765172937857888,
8.43664979310337));
#19065=CARTESIAN_POINT('Ctrl Pts',(-2.37317408998301,-0.844238494108646,
8.44188821897196));
#19066=CARTESIAN_POINT('Ctrl Pts',(-2.34401709592337,-0.922113298716357,
8.44712664484055));
#19067=CARTESIAN_POINT('Ctrl Pts',(-2.31106813594437,-0.998383854548244,
8.45236507070915));
#19068=CARTESIAN_POINT('Ctrl Pts',(-2.27813001232996,-1.07462932626364,
8.45760177374665));
#19069=CARTESIAN_POINT('Ctrl Pts',(-2.24140258247872,-1.14927117381642,
8.46283847678415));
#19070=CARTESIAN_POINT('Ctrl Pts',(-2.2010745675889,-1.22191529899308,8.46807517982166));
#19071=CARTESIAN_POINT('Ctrl Pts',(-2.16074765121404,-1.29455744538009,
8.47331174021399));
#19072=CARTESIAN_POINT('Ctrl Pts',(-2.11682056966571,-1.36520157466179,
8.47854830060632));
#19073=CARTESIAN_POINT('Ctrl Pts',(-2.06952761647568,-1.43347887833915,
8.48378486099866));
#19074=CARTESIAN_POINT('Ctrl Pts',(-2.02146060512304,-1.50287369743199,
8.48910712976913));
#19075=CARTESIAN_POINT('Ctrl Pts',(-1.96991681677189,-1.56982310309958,
8.49442939853961));
#19076=CARTESIAN_POINT('Ctrl Pts',(-1.91518647561926,-1.6339727701541,8.49975166731009));
#19077=CARTESIAN_POINT('Ctrl Pts',(-1.86126016319972,-1.69718003169016,
8.50499574806043));
#19078=CARTESIAN_POINT('Ctrl Pts',(-1.80424066777231,-1.75766897052556,
8.51023982881076));
#19079=CARTESIAN_POINT('Ctrl Pts',(-1.74444329879661,-1.81513741278273,
8.51548390956109));
#19080=CARTESIAN_POINT('Ctrl Pts',(-1.68330858259666,-1.87389111663336,
8.52084527234165));
#19081=CARTESIAN_POINT('Ctrl Pts',(-1.61927062781268,-1.92948725322094,
8.5262066351222));
#19082=CARTESIAN_POINT('Ctrl Pts',(-1.55270102323419,-1.98164723965884,
8.53156799790275));
#19083=CARTESIAN_POINT('Ctrl Pts',(-1.48613141865571,-2.03380722609674,
8.53692936068331));
#19084=CARTESIAN_POINT('Ctrl Pts',(-1.41703061803393,-2.08253082417426,
8.54229072346386));
#19085=CARTESIAN_POINT('Ctrl Pts',(-1.34579874535832,-2.12758830298344,
8.54765208624441));
#19086=CARTESIAN_POINT('Ctrl Pts',(-1.27597671092752,-2.17175399340559,
8.55290733565172));
#19087=CARTESIAN_POINT('Ctrl Pts',(-1.20384932162568,-2.21256053261645,
8.55816258505902));
#19088=CARTESIAN_POINT('Ctrl Pts',(-1.12977320620478,-2.2497597099561,8.56341783446633));
#19089=CARTESIAN_POINT('Ctrl Pts',(-1.05580211388743,-2.28690614731295,
8.56866563312383));
#19090=CARTESIAN_POINT('Ctrl Pts',(-0.979888192187141,-2.32045517618541,
8.57391343178133));
#19091=CARTESIAN_POINT('Ctrl Pts',(-0.902415987114985,-2.35020246706519,
8.57916123043883));
#19092=CARTESIAN_POINT('Ctrl Pts',(-0.824382429128209,-2.38016530271256,
8.58444705392173));
#19093=CARTESIAN_POINT('Ctrl Pts',(-0.744768310763633,-2.40627082083289,
8.58973287740464));
#19094=CARTESIAN_POINT('Ctrl Pts',(-0.663990793267411,-2.4283579794701,
8.59501870088755));
#19095=CARTESIAN_POINT('Ctrl Pts',(-0.583937602194848,-2.45024708408039,
8.60025712675614));
#19096=CARTESIAN_POINT('Ctrl Pts',(-0.502742245948794,-2.46818948133829,
8.60549555262473));
#19097=CARTESIAN_POINT('Ctrl Pts',(-0.420827979435216,-2.48207777108705,
8.61073397849333));
#19098=CARTESIAN_POINT('Ctrl Pts',(-0.338940653160633,-2.49596149320846,
8.61597068153083));
#19099=CARTESIAN_POINT('Ctrl Pts',(-0.256335340766099,-2.50579367881355,
8.62120738456834));
#19100=CARTESIAN_POINT('Ctrl Pts',(-0.173445358343676,-2.51151805839995,
8.62644408760584));
#19101=CARTESIAN_POINT('Ctrl Pts',(-0.0905576338029299,-2.5172422820571,
8.63168064799818));
#19102=CARTESIAN_POINT('Ctrl Pts',(-0.00738571504710353,-2.51885889140939,
8.63691720839051));
#19103=CARTESIAN_POINT('Ctrl Pts',(0.0756334827210238,-2.51636361170072,
8.64215376878284));
#19104=CARTESIAN_POINT('Ctrl Pts',(0.160011480973147,-2.5138274909894,8.64747603755332));
#19105=CARTESIAN_POINT('Ctrl Pts',(0.244231221974307,-2.50704366739768,
8.6527983063238));
#19106=CARTESIAN_POINT('Ctrl Pts',(0.327837487473386,-2.49606266584137,
8.65812057509428));
#19107=CARTESIAN_POINT('Ctrl Pts',(0.41021551579522,-2.48524298322778,8.66336465584461));
#19108=CARTESIAN_POINT('Ctrl Pts',(0.49199752432431,-2.47034876753276,8.66860873659494));
#19109=CARTESIAN_POINT('Ctrl Pts',(0.572758381215893,-2.45147997885909,
8.67385281734527));
#19110=CARTESIAN_POINT('Ctrl Pts',(0.655325426400422,-2.432189196332,8.67921418012582));
#19111=CARTESIAN_POINT('Ctrl Pts',(0.736824601303901,-2.40874405725313,
8.68457554290638));
#19112=CARTESIAN_POINT('Ctrl Pts',(0.816819920653717,-2.3813045725449,8.68993690568693));
#19113=CARTESIAN_POINT('Ctrl Pts',(0.896815240003528,-2.35386508783667,
8.69529826846748));
#19114=CARTESIAN_POINT('Ctrl Pts',(0.975306256944832,-2.32243150840789,
8.70065963124803));
#19115=CARTESIAN_POINT('Ctrl Pts',(1.05188242683368,-2.28721437782261,8.70602099402858));
#19116=CARTESIAN_POINT('Ctrl Pts',(1.12694298287034,-2.25269427310095,8.71127624343589));
#19117=CARTESIAN_POINT('Ctrl Pts',(1.2004410628445,-2.2144115593781,8.7165314928432));
#19118=CARTESIAN_POINT('Ctrl Pts',(1.27197430248878,-2.17253023541864,8.72178674225051));
#19119=CARTESIAN_POINT('Ctrl Pts',(1.34340612424965,-2.13070828966226,8.72703454090801));
#19120=CARTESIAN_POINT('Ctrl Pts',(1.41287824401752,-2.08529809894302,8.7322823395655));
#19121=CARTESIAN_POINT('Ctrl Pts',(1.48000990510121,-2.03651096996857,8.737530138223));
#19122=CARTESIAN_POINT('Ctrl Pts',(1.54762799294374,-1.98737033618524,8.74281596170591));
#19123=CARTESIAN_POINT('Ctrl Pts',(1.61287113116809,-1.93480381800173,8.74810178518882));
#19124=CARTESIAN_POINT('Ctrl Pts',(1.67537711493224,-1.87907364750861,8.75338760867172));
#19125=CARTESIAN_POINT('Ctrl Pts',(1.73732261185449,-1.8238432056075,8.75862603454032));
#19126=CARTESIAN_POINT('Ctrl Pts',(1.79657949470934,-1.76550593339148,8.76386446040891));
#19127=CARTESIAN_POINT('Ctrl Pts',(1.85282723527963,-1.70435837962737,8.7691028862775));
#19128=CARTESIAN_POINT('Ctrl Pts',(1.90905647690416,-1.64323093627604,8.774339589315));
#19129=CARTESIAN_POINT('Ctrl Pts',(1.96227822961948,-1.57929538632552,8.77957629235251));
#19130=CARTESIAN_POINT('Ctrl Pts',(2.01220937537835,-1.51288455595246,8.78481299539001));
#19131=CARTESIAN_POINT('Ctrl Pts',(2.06213916103779,-1.4464755345772,8.79004955578234));
#19132=CARTESIAN_POINT('Ctrl Pts',(2.10877824149183,-1.37759173626641,8.79528611617467));
#19133=CARTESIAN_POINT('Ctrl Pts',(2.15188515194386,-1.30659731472383,8.80052267656701));
#19134=CARTESIAN_POINT('Ctrl Pts',(2.19569760632263,-1.23444090587049,8.80584494533749));
#19135=CARTESIAN_POINT('Ctrl Pts',(2.23586095688824,-1.16010457351426,8.81116721410797));
#19136=CARTESIAN_POINT('Ctrl Pts',(2.27216973926283,-1.08399765958155,8.81648948287845));
#19137=CARTESIAN_POINT('Ctrl Pts',(2.30794511907356,-1.00900881186765,8.82173356362878));
#19138=CARTESIAN_POINT('Ctrl Pts',(2.3399783080633,-0.932301515061035,8.82697764437911));
#19139=CARTESIAN_POINT('Ctrl Pts',(2.36812168829854,-0.854286789907267,
8.83222172512945));
#19140=CARTESIAN_POINT('Ctrl Pts',(2.39689448538076,-0.774527292735595,
8.83758308791));
#19141=CARTESIAN_POINT('Ctrl Pts',(2.42160123659593,-0.69340167100751,8.84294445069055));
#19142=CARTESIAN_POINT('Ctrl Pts',(2.44213878500907,-0.611362744002635,
8.8483058134711));
#19143=CARTESIAN_POINT('Ctrl Pts',(2.46267633342221,-0.529323816997754,
8.85366717625165));
#19144=CARTESIAN_POINT('Ctrl Pts',(2.47904464620288,-0.446372096142171,
8.85902853903221));
#19145=CARTESIAN_POINT('Ctrl Pts',(2.49119680399602,-0.362966573888061,
8.86438990181276));
#19146=CARTESIAN_POINT('Ctrl Pts',(2.50859444872508,-0.243559002877223,
8.87206550037784));
#19147=CARTESIAN_POINT('Ctrl Pts',(2.5174096762307,-0.12287148413771,8.87974109894292));
#19148=CARTESIAN_POINT('Ctrl Pts',(2.51749930935083,-0.00186478366189579,
8.88741669750801));
#19149=CARTESIAN_POINT('Ctrl Pts',(2.51749930935125,-0.00186478309385184,
8.88741669754404));
#19150=CARTESIAN_POINT('Ctrl Pts',(2.51755970653645,0.0796727815327686,
8.89258872199874));
#19151=CARTESIAN_POINT('Ctrl Pts',(2.51365459994446,0.161358301547571,8.89776074645344));
#19152=CARTESIAN_POINT('Ctrl Pts',(2.5057673658586,0.242767704190768,8.90293277090814));
#19153=CARTESIAN_POINT('Ctrl Pts',(2.49788815071092,0.324094338025553,8.90809953697391));
#19154=CARTESIAN_POINT('Ctrl Pts',(2.48603488288074,0.405144940630114,8.91326630303968));
#19155=CARTESIAN_POINT('Ctrl Pts',(2.47024295996914,0.485495590837766,8.91843306910546));
#19156=CARTESIAN_POINT('Ctrl Pts',(2.45446208214504,0.565790042698492,8.92359622146417));
#19157=CARTESIAN_POINT('Ctrl Pts',(2.43474810638477,0.645385047783456,8.92875937382288));
#19158=CARTESIAN_POINT('Ctrl Pts',(2.4111880499293,0.723863549212233,8.9339225261816));
#19159=CARTESIAN_POINT('Ctrl Pts',(2.39615340801751,0.773943911667475,8.93721734625115));
#19160=CARTESIAN_POINT('Ctrl Pts',(2.37955359253486,0.823569749410887,8.94051216632071));
#19161=CARTESIAN_POINT('Ctrl Pts',(2.36142200728635,0.872635292378026,8.94380698639026));
#19162=CARTESIAN_POINT('',(2.51749909420668,-0.00135787363871094,8.61075084542347));
#19163=CARTESIAN_POINT('Ctrl Pts',(2.36142186693781,0.872635672172493,8.66836043115426));
#19164=CARTESIAN_POINT('Ctrl Pts',(2.38766432837594,0.801621474313745,8.66315328780155));
#19165=CARTESIAN_POINT('Ctrl Pts',(2.4107055817133,0.729417533717104,8.65798469879897));
#19166=CARTESIAN_POINT('Ctrl Pts',(2.45152777444271,0.578228022230177,8.64746763910954));
#19167=CARTESIAN_POINT('Ctrl Pts',(2.46882533046289,0.499239322516955,8.64213924160784));
#19168=CARTESIAN_POINT('Ctrl Pts',(2.48627876218841,0.395974422567439,8.63538790124849));
#19169=CARTESIAN_POINT('Ctrl Pts',(2.48992714207542,0.372344891433137,8.63385720767189));
#19170=CARTESIAN_POINT('Ctrl Pts',(2.49512354268189,0.335186536182973,8.63147163611905));
#19171=CARTESIAN_POINT('Ctrl Pts',(2.49689929596445,0.321691505840321,8.63060968090192));
#19172=CARTESIAN_POINT('Ctrl Pts',(2.49985358529291,0.297739837343419,8.62908747963504));
#19173=CARTESIAN_POINT('Ctrl Pts',(2.50107616058215,0.287289058310349,8.62842587294413));
#19174=CARTESIAN_POINT('Ctrl Pts',(2.50343991969958,0.265923384065525,8.62707840247117));
#19175=CARTESIAN_POINT('Ctrl Pts',(2.50457532711521,0.255008067724658,8.62639273211866));
#19176=CARTESIAN_POINT('Ctrl Pts',(2.50692920549118,0.230844529274809,8.62488069701353));
#19177=CARTESIAN_POINT('Ctrl Pts',(2.5081141120614,0.217593312163377,8.62405538682484));
#19178=CARTESIAN_POINT('Ctrl Pts',(2.51142857636331,0.176891963405776,8.6215318582072));
#19179=CARTESIAN_POINT('Ctrl Pts',(2.51321297152733,0.14941522635885,8.61984422538577));
#19180=CARTESIAN_POINT('Ctrl Pts',(2.51653706826746,0.0808537709645683,
8.61566864809835));
#19181=CARTESIAN_POINT('Ctrl Pts',(2.51752185448915,0.0397499541746253,
8.6131971064922));
#19182=CARTESIAN_POINT('Ctrl Pts',(2.51749963220541,-0.00136082535489392,
8.61074973370103));
#19183=CARTESIAN_POINT('Ctrl Pts',(2.51749963382901,-0.00135781839193702,
8.6107499127091));
#19184=CARTESIAN_POINT('Ctrl Pts',(2.51737464808992,-0.233090982609691,
8.59695455967742));
#19185=CARTESIAN_POINT('Ctrl Pts',(2.4852569110145,-0.46368713501507,8.58412487491137));
#19186=CARTESIAN_POINT('Ctrl Pts',(2.41013441700624,-0.728675235698085,
8.56783566805232));
#19187=CARTESIAN_POINT('Ctrl Pts',(2.39712499375044,-0.770393956259634,
8.56521950708456));
#19188=CARTESIAN_POINT('Ctrl Pts',(2.37405534696998,-0.838118981753158,
8.56085586831821));
#19189=CARTESIAN_POINT('Ctrl Pts',(2.36463670135636,-0.864335201202673,
8.55913748803329));
#19190=CARTESIAN_POINT('Ctrl Pts',(2.35123051681317,-0.899790162408652,
8.55676663776672));
#19191=CARTESIAN_POINT('Ctrl Pts',(2.34761935723741,-0.909170294859618,
8.55613487769055));
#19192=CARTESIAN_POINT('Ctrl Pts',(2.34147656589317,-0.924845814336315,
8.55507113418019));
#19193=CARTESIAN_POINT('Ctrl Pts',(2.3389754317916,-0.931153164939045,8.55464093873036));
#19194=CARTESIAN_POINT('Ctrl Pts',(2.33417206311208,-0.943124813602679,
8.5538201231076));
#19195=CARTESIAN_POINT('Ctrl Pts',(2.33187463657746,-0.948790973615488,
8.55342980438863));
#19196=CARTESIAN_POINT('Ctrl Pts',(2.32636012689872,-0.96225043289266,8.55249837835992));
#19197=CARTESIAN_POINT('Ctrl Pts',(2.32312451342757,-0.970035992074675,
8.55195619037801));
#19198=CARTESIAN_POINT('Ctrl Pts',(2.31151513200617,-0.997579338570043,
8.55002633001605));
#19199=CARTESIAN_POINT('Ctrl Pts',(2.30292818396566,-1.01724552087722,8.54862690632044));
#19200=CARTESIAN_POINT('Ctrl Pts',(2.23938325271842,-1.15784934633412,8.53847862266113));
#19201=CARTESIAN_POINT('Ctrl Pts',(2.17518504586928,-1.27436882180376,8.52931295679336));
#19202=CARTESIAN_POINT('Ctrl Pts',(2.0276928550642,-1.49818382513107,8.51079520974065));
#19203=CARTESIAN_POINT('Ctrl Pts',(1.94429841729279,-1.60493096679138,8.5014754838603));
#19204=CARTESIAN_POINT('Ctrl Pts',(1.81831792885298,-1.74186934011822,8.4890361871044));
#19205=CARTESIAN_POINT('Ctrl Pts',(1.7827842255893,-1.77822098399486,8.48567866899807));
#19206=CARTESIAN_POINT('Ctrl Pts',(1.72804177147631,-1.83093183261729,8.48072608097172));
#19207=CARTESIAN_POINT('Ctrl Pts',(1.70964989923951,-1.84811715973801,8.47909709581625));
#19208=CARTESIAN_POINT('Ctrl Pts',(1.67555017835562,-1.87903510808308,8.47613927387552));
#19209=CARTESIAN_POINT('Ctrl Pts',(1.65992361592052,-1.89285365775568,8.47480693598427));
#19210=CARTESIAN_POINT('Ctrl Pts',(1.634617829585,-1.91467711804161,8.47268544841849));
#19211=CARTESIAN_POINT('Ctrl Pts',(1.62504758341077,-1.92280635428529,8.47189121301355));
#19212=CARTESIAN_POINT('Ctrl Pts',(1.60648814244898,-1.938333722254,8.4703662544326));
#19213=CARTESIAN_POINT('Ctrl Pts',(1.59750768697473,-1.94574175265601,8.46963514133291));
#19214=CARTESIAN_POINT('Ctrl Pts',(1.57703519686471,-1.96239234463157,8.46798352273246));
#19215=CARTESIAN_POINT('Ctrl Pts',(1.56551262079387,-1.97159680846695,8.46706455388978));
#19216=CARTESIAN_POINT('Ctrl Pts',(1.53017631787962,-1.99931904365559,8.46427783639052));
#19217=CARTESIAN_POINT('Ctrl Pts',(1.5061095338955,-2.01751094001382,8.46242285358293));
#19218=CARTESIAN_POINT('Ctrl Pts',(1.31079447398623,-2.15970479185445,8.4476911339114));
#19219=CARTESIAN_POINT('Ctrl Pts',(1.12487776398485,-2.26211520369748,8.43571270384987));
#19220=CARTESIAN_POINT('Ctrl Pts',(0.813875362275058,-2.38549275388142,
8.41642002826897));
#19221=CARTESIAN_POINT('Ctrl Pts',(0.696253449370582,-2.42243519113316,
8.40924954365842));
#19222=CARTESIAN_POINT('Ctrl Pts',(0.558894500901102,-2.45474383037895,
8.4005399526972));
#19223=CARTESIAN_POINT('Ctrl Pts',(0.541327222224817,-2.45867751677927,
8.39941981076524));
#19224=CARTESIAN_POINT('Ctrl Pts',(0.515449824455284,-2.46418124650907,
8.3977586177536));
#19225=CARTESIAN_POINT('Ctrl Pts',(0.50717112626941,-2.46589845309399,8.3972254954022));
#19226=CARTESIAN_POINT('Ctrl Pts',(0.492486662819062,-2.4688672983262,8.39627664719856));
#19227=CARTESIAN_POINT('Ctrl Pts',(0.486084471445781,-2.47013577259444,
8.39586187465994));
#19228=CARTESIAN_POINT('Ctrl Pts',(0.472190510290721,-2.4728324924096,8.39495931342163));
#19229=CARTESIAN_POINT('Ctrl Pts',(0.464697279245796,-2.47425157341053,
8.39447104429632));
#19230=CARTESIAN_POINT('Ctrl Pts',(0.443893438794687,-2.47809360376033,
8.39311148830178));
#19231=CARTESIAN_POINT('Ctrl Pts',(0.430569797360363,-2.48044329192573,
8.39223629570707));
#19232=CARTESIAN_POINT('Ctrl Pts',(0.356504087570587,-2.49289042031678,
8.38734871702509));
#19233=CARTESIAN_POINT('Ctrl Pts',(0.295431112545935,-2.50086323803604,
8.38323540522959));
#19234=CARTESIAN_POINT('Ctrl Pts',(0.056764030473468,-2.52315643000945,
8.36698759428564));
#19235=CARTESIAN_POINT('Ctrl Pts',(-0.121863623809035,-2.52085194192725,
8.35449859967775));
#19236=CARTESIAN_POINT('Ctrl Pts',(-0.411426366202344,-2.48624412087625,
8.33468096217839));
#19237=CARTESIAN_POINT('Ctrl Pts',(-0.523066232554378,-2.46517534363098,
8.32713640010854));
#19238=CARTESIAN_POINT('Ctrl Pts',(-0.655317832266786,-2.43082299089872,
8.31833734980553));
#19239=CARTESIAN_POINT('Ctrl Pts',(-0.677637339666892,-2.42469576827135,
8.31685686419236));
#19240=CARTESIAN_POINT('Ctrl Pts',(-0.712649121655435,-2.41456299752018,
8.31454092615491));
#19241=CARTESIAN_POINT('Ctrl Pts',(-0.725399115355684,-2.410763234761,8.31369890121087));
#19242=CARTESIAN_POINT('Ctrl Pts',(-0.749218013192332,-2.40345863337134,
8.31212821257802));
#19243=CARTESIAN_POINT('Ctrl Pts',(-0.760293902739406,-2.39997796288599,
8.31139878916497));
#19244=CARTESIAN_POINT('Ctrl Pts',(-0.785042307749389,-2.39201209542708,
8.30977088771807));
#19245=CARTESIAN_POINT('Ctrl Pts',(-0.798701316259831,-2.3874860231246,
8.30887376698085));
#19246=CARTESIAN_POINT('Ctrl Pts',(-0.833368841284254,-2.37566772108291,
8.30659976307365));
#19247=CARTESIAN_POINT('Ctrl Pts',(-0.854321184433942,-2.36821369576142,
8.3052281867491));
#19248=CARTESIAN_POINT('Ctrl Pts',(-1.02688164672101,-2.3042351847904,8.29394845952897));
#19249=CARTESIAN_POINT('Ctrl Pts',(-1.1728222245501,-2.23349125458446,8.28454767554206));
#19250=CARTESIAN_POINT('Ctrl Pts',(-1.41692888469482,-2.08459133975002,
8.26809879652324));
#19251=CARTESIAN_POINT('Ctrl Pts',(-1.51794929679112,-2.01222139487975,
8.26102541531852));
#19252=CARTESIAN_POINT('Ctrl Pts',(-1.64677294364045,-1.90469309904515,
8.25110154928247));
#19253=CARTESIAN_POINT('Ctrl Pts',(-1.67959341799864,-1.87581514430811,
8.24848445035755));
#19254=CARTESIAN_POINT('Ctrl Pts',(-1.73207627790999,-1.82715472862733,
8.24411939847138));
#19255=CARTESIAN_POINT('Ctrl Pts',(-1.75219200170792,-1.80787324646103,
8.24240056678593));
#19256=CARTESIAN_POINT('Ctrl Pts',(-1.77912312868682,-1.78118729876964,
8.24002918945711));
#19257=CARTESIAN_POINT('Ctrl Pts',(-1.78622107852673,-1.77406920691418,
8.23939736559858));
#19258=CARTESIAN_POINT('Ctrl Pts',(-1.79803841163796,-1.7620755267802,8.23833354479875));
#19259=CARTESIAN_POINT('Ctrl Pts',(-1.80278114649585,-1.75722293059777,
8.23790333641549));
#19260=CARTESIAN_POINT('Ctrl Pts',(-1.8117599738799,-1.7479615067211,8.23708252024665));
#19261=CARTESIAN_POINT('Ctrl Pts',(-1.81599972690298,-1.74355631451983,
8.2366922140699));
#19262=CARTESIAN_POINT('Ctrl Pts',(-1.82604727201779,-1.73304030058062,
8.23576084896937));
#19263=CARTESIAN_POINT('Ctrl Pts',(-1.83184045452337,-1.72691570941812,
8.23521870969261));
#19264=CARTESIAN_POINT('Ctrl Pts',(-1.85226731321811,-1.7051018590694,8.23328919107777));
#19265=CARTESIAN_POINT('Ctrl Pts',(-1.86673060489012,-1.68925525786975,
8.23189006568425));
#19266=CARTESIAN_POINT('Ctrl Pts',(-1.96694419050882,-1.57659826359056,
8.22197316778406));
#19267=CARTESIAN_POINT('Ctrl Pts',(-2.04531778775473,-1.47349935742758,
8.21305998009377));
#19268=CARTESIAN_POINT('Ctrl Pts',(-2.19277144766801,-1.24495675186071,
8.19427160147215));
#19269=CARTESIAN_POINT('Ctrl Pts',(-2.2598002872475,-1.11869322411117,8.18443217630014));
#19270=CARTESIAN_POINT('Ctrl Pts',(-2.34454518273031,-0.919942994800179,
8.17001376318646));
#19271=CARTESIAN_POINT('Ctrl Pts',(-2.37035589243968,-0.851235547118459,
8.16520466978328));
#19272=CARTESIAN_POINT('Ctrl Pts',(-2.39949401582388,-0.762007148649081,
8.15917738289421));
#19273=CARTESIAN_POINT('Ctrl Pts',(-2.40561907951748,-0.74244414700348,
8.15786891767906));
#19274=CARTESIAN_POINT('Ctrl Pts',(-2.41515908654987,-0.710615818501265,
8.15576057224085));
#19275=CARTESIAN_POINT('Ctrl Pts',(-2.41872103605421,-0.698395886482881,
8.1549559609172));
#19276=CARTESIAN_POINT('Ctrl Pts',(-2.42538505504475,-0.674871090933258,
8.15341610231489));
#19277=CARTESIAN_POINT('Ctrl Pts',(-2.42850113331093,-0.663570574678193,
8.15268042042152));
#19278=CARTESIAN_POINT('Ctrl Pts',(-2.43546012369153,-0.637627932097979,
8.15100048916356));
#19279=CARTESIAN_POINT('Ctrl Pts',(-2.4392501522418,-0.622971993294495,
8.15005795685465));
#19280=CARTESIAN_POINT('Ctrl Pts',(-2.45090892130213,-0.57614950877362,
8.14706680672387));
#19281=CARTESIAN_POINT('Ctrl Pts',(-2.45827551078707,-0.543860704749151,
8.14503416358954));
#19282=CARTESIAN_POINT('Ctrl Pts',(-2.49961667841714,-0.34460536143009,
8.13265669104477));
#19283=CARTESIAN_POINT('Ctrl Pts',(-2.51720653304508,-0.174688620952317,
8.12285330540817));
#19284=CARTESIAN_POINT('Ctrl Pts',(-2.51766562992915,0.0952434320171729,
8.10734351450212));
#19285=CARTESIAN_POINT('Ctrl Pts',(-2.51193289355596,0.194685999372743,
8.10163318409915));
#19286=CARTESIAN_POINT('Ctrl Pts',(-2.4950527900688,0.338476855747316,8.09308307747562));
#19287=CARTESIAN_POINT('Ctrl Pts',(-2.48856429327033,0.3832783608502,8.09037661033664));
#19288=CARTESIAN_POINT('Ctrl Pts',(-2.47601610355159,0.456033812292816,
8.08587718251499));
#19289=CARTESIAN_POINT('Ctrl Pts',(-2.47068131206139,0.48410358145907,8.08411565193481));
#19290=CARTESIAN_POINT('Ctrl Pts',(-2.46280586571477,0.522011993804842,
8.08169446565782));
#19291=CARTESIAN_POINT('Ctrl Pts',(-2.46068145006588,0.531936130489481,
8.08105667079656));
#19292=CARTESIAN_POINT('Ctrl Pts',(-2.45703238159988,0.548492880201491,
8.07998560484734));
#19293=CARTESIAN_POINT('Ctrl Pts',(-2.45554070858783,0.555132768166742,
8.07955417624436));
#19294=CARTESIAN_POINT('Ctrl Pts',(-2.45266165932137,0.567709615012644,
8.07873326517996));
#19295=CARTESIAN_POINT('Ctrl Pts',(-2.45127960323995,0.573647737657269,
8.07834409864006));
#19296=CARTESIAN_POINT('Ctrl Pts',(-2.44795081100352,0.587718475635898,
8.0774183008108));
#19297=CARTESIAN_POINT('Ctrl Pts',(-2.44598511085898,0.595846467177164,
8.07688061830548));
#19298=CARTESIAN_POINT('Ctrl Pts',(-2.43892972344113,0.624396526177035,
8.07498215129924));
#19299=CARTESIAN_POINT('Ctrl Pts',(-2.43362462574986,0.644763778933942,
8.07361009341827));
#19300=CARTESIAN_POINT('Ctrl Pts',(-2.38854986346771,0.809326728405822,
8.06239315346727));
#19301=CARTESIAN_POINT('Ctrl Pts',(-2.33625944751048,0.949770678525944,
8.0520197683175));
#19302=CARTESIAN_POINT('Ctrl Pts',(-2.21661803535369,1.20034354390598,8.03284351853884));
#19303=CARTESIAN_POINT('Ctrl Pts',(-2.15266556743567,1.31158583729764,8.02405411413298));
#19304=CARTESIAN_POINT('Ctrl Pts',(-2.05469925225694,1.4553760563597,8.01247067482682));
#19305=CARTESIAN_POINT('Ctrl Pts',(-2.02785168977947,1.49255701245392,8.00945181006693));
#19306=CARTESIAN_POINT('Ctrl Pts',(-1.97942987376889,1.55589555320451,8.00426743175082));
#19307=CARTESIAN_POINT('Ctrl Pts',(-1.95831586840964,1.5823883023995,8.00208553875647));
#19308=CARTESIAN_POINT('Ctrl Pts',(-1.92680814957182,1.6203255824475,7.99893982152219));
#19309=CARTESIAN_POINT('Ctrl Pts',(-1.91683430240607,1.63211240814546,7.99795937257309));
#19310=CARTESIAN_POINT('Ctrl Pts',(-1.89909460657724,1.65268976900617,7.99624194548377));
#19311=CARTESIAN_POINT('Ctrl Pts',(-1.89137466600175,1.66151908735217,7.99550312688755));
#19312=CARTESIAN_POINT('Ctrl Pts',(-1.87516099332643,1.67980326899045,7.99396897777136));
#19313=CARTESIAN_POINT('Ctrl Pts',(-1.86665678041011,1.6892484266645,7.99317411113845));
#19314=CARTESIAN_POINT('Ctrl Pts',(-1.84430919164595,1.7136938107486,7.99111036956656));
#19315=CARTESIAN_POINT('Ctrl Pts',(-1.83035409661777,1.72859098411185,7.98984622463906));
#19316=CARTESIAN_POINT('Ctrl Pts',(-1.77097689912881,1.79045121276967,7.98456682576103));
#19317=CARTESIAN_POINT('Ctrl Pts',(-1.72391462894867,1.83580885495681,7.98062253163847));
#19318=CARTESIAN_POINT('Ctrl Pts',(-1.52584839570059,2.01235889236698,7.96484999876149));
#19319=CARTESIAN_POINT('Ctrl Pts',(-1.36124366885512,2.1271612941855,7.95364432877833));
#19320=CARTESIAN_POINT('Ctrl Pts',(-1.12974841760269,2.25063690371914,7.9383454758762));
#19321=CARTESIAN_POINT('Ctrl Pts',(-1.07363646105424,2.27793803402906,7.93466314865816));
#19322=CARTESIAN_POINT('Ctrl Pts',(-0.98388970465471,2.31755120216156,7.92872740867969));
#19323=CARTESIAN_POINT('Ctrl Pts',(-0.950905355950302,2.3312788830228,7.92653632078502));
#19324=CARTESIAN_POINT('Ctrl Pts',(-0.907378010061243,2.34831703359879,
7.92361852470122));
#19325=CARTESIAN_POINT('Ctrl Pts',(-0.897087876634973,2.35226722005725,
7.92292683693532));
#19326=CARTESIAN_POINT('Ctrl Pts',(-0.880226635211065,2.35861320194372,
7.92178983062499));
#19327=CARTESIAN_POINT('Ctrl Pts',(-0.87367076998457,2.36104945914826,7.92134685897184));
#19328=CARTESIAN_POINT('Ctrl Pts',(-0.860844192792682,2.36575527021321,
7.92047829135203));
#19329=CARTESIAN_POINT('Ctrl Pts',(-0.854574482394941,2.36802727460356,
7.92005284264647));
#19330=CARTESIAN_POINT('Ctrl Pts',(-0.840540094581967,2.37305003259906,
7.91909863216753));
#19331=CARTESIAN_POINT('Ctrl Pts',(-0.832770801400698,2.3757876369001,7.91856911882831));
#19332=CARTESIAN_POINT('Ctrl Pts',(-0.80579443415389,2.38514450467108,7.91672649406695));
#19333=CARTESIAN_POINT('Ctrl Pts',(-0.786521347912426,2.39156916813997,
7.91540293331457));
#19334=CARTESIAN_POINT('Ctrl Pts',(-0.611055225459327,2.44771029748455,
7.90330190015009));
#19335=CARTESIAN_POINT('Ctrl Pts',(-0.450444886224806,2.48229034993314,
7.89188774136286));
#19336=CARTESIAN_POINT('Ctrl Pts',(-0.190566171215828,2.5121776452348,7.87384210604544));
#19337=CARTESIAN_POINT('Ctrl Pts',(-0.0929297295445561,2.5176812168465,
7.86714919964302));
#19338=CARTESIAN_POINT('Ctrl Pts',(0.0885422853935554,2.51733622264386,
7.85497386326368));
#19339=CARTESIAN_POINT('Ctrl Pts',(0.172245330360465,2.51299732701248,7.84946171354762));
#19340=CARTESIAN_POINT('Ctrl Pts',(0.276828897499114,2.50232452549987,7.84270486789271));
#19341=CARTESIAN_POINT('Ctrl Pts',(0.298045241888387,2.49988626723135,7.84134075284194));
#19342=CARTESIAN_POINT('Ctrl Pts',(0.33203919532441,2.49554062631197,7.83916517329379));
#19343=CARTESIAN_POINT('Ctrl Pts',(0.344837247835686,2.49380438836038,7.8383484082176));
#19344=CARTESIAN_POINT('Ctrl Pts',(0.369174734470975,2.49031172546414,7.8367993903288));
#19345=CARTESIAN_POINT('Ctrl Pts',(0.380716382724384,2.48857339008721,7.83606659262183));
#19346=CARTESIAN_POINT('Ctrl Pts',(0.407077902814832,2.48441528317325,7.83439677476896));
#19347=CARTESIAN_POINT('Ctrl Pts',(0.421889141030419,2.48194304654735,7.8334614260073));
#19348=CARTESIAN_POINT('Ctrl Pts',(0.467770520756483,2.47386211164416,7.83057211367006));
#19349=CARTESIAN_POINT('Ctrl Pts',(0.498758640351203,2.46780124039813,7.82863236254786));
#19350=CARTESIAN_POINT('Ctrl Pts',(0.723828231857169,2.41936770350154,7.81461117430008));
#19351=CARTESIAN_POINT('Ctrl Pts',(0.912401862226988,2.35473969720422,7.80330341300111));
#19352=CARTESIAN_POINT('Ctrl Pts',(1.17832828471452,2.22680211230946,7.78631724603764));
#19353=CARTESIAN_POINT('Ctrl Pts',(1.26274580993872,2.18004025600454,7.78073703524978));
#19354=CARTESIAN_POINT('Ctrl Pts',(1.37092066368093,2.11172359912494,7.77307222629464));
#19355=CARTESIAN_POINT('Ctrl Pts',(1.39725478287324,2.09439225466527,7.77116318943319));
#19356=CARTESIAN_POINT('Ctrl Pts',(1.44131402096562,2.06419462633159,7.76788293455805));
#19357=CARTESIAN_POINT('Ctrl Pts',(1.45920980659037,2.05158285910118,7.76652569597058));
#19358=CARTESIAN_POINT('Ctrl Pts',(1.48434531354932,2.03337377302988,7.76458029861017));
#19359=CARTESIAN_POINT('Ctrl Pts',(1.49172306209089,2.02796750728548,7.76400442900969));
#19360=CARTESIAN_POINT('Ctrl Pts',(1.50438656998002,2.01858145113807,7.76300726303883));
#19361=CARTESIAN_POINT('Ctrl Pts',(1.50968647758137,2.01462074977195,7.76258726930048));
#19362=CARTESIAN_POINT('Ctrl Pts',(1.52075911240334,2.00627777227604,7.76170410474754));
#19363=CARTESIAN_POINT('Ctrl Pts',(1.52652855707195,2.00189144030462,7.76124066839993));
#19364=CARTESIAN_POINT('Ctrl Pts',(1.54193500079129,1.99007306679771,7.75999455033995));
#19365=CARTESIAN_POINT('Ctrl Pts',(1.55153704097377,1.98259606431021,7.75920884922047));
#19366=CARTESIAN_POINT('Ctrl Pts',(1.59440894029345,1.94871001077266,7.75566130299178));
#19367=CARTESIAN_POINT('Ctrl Pts',(1.62705943610825,1.92153263700967,7.75285187299618));
#19368=CARTESIAN_POINT('Ctrl Pts',(1.68747338721567,1.86860173047059,7.74747002353398));
#19369=CARTESIAN_POINT('Ctrl Pts',(1.71537498394118,1.84302123966393,7.74490570707718));
#19370=CARTESIAN_POINT('Ctrl Pts',(1.78555450477,1.77570535738269,7.73827061628446));
#19371=CARTESIAN_POINT('Ctrl Pts',(1.826951155555,1.73308496705262,7.73417578307359));
#19372=CARTESIAN_POINT('Ctrl Pts',(1.96511040899497,1.58038550424474,7.71995367550269));
#19373=CARTESIAN_POINT('Ctrl Pts',(2.05375639382241,1.4633421695019,7.7098355341175));
#19374=CARTESIAN_POINT('Ctrl Pts',(2.1713043388427,1.27623673274407,7.69508160225339));
#19375=CARTESIAN_POINT('Ctrl Pts',(2.20807736402743,1.21150276350709,7.69020157538508));
#19376=CARTESIAN_POINT('Ctrl Pts',(2.25129880366988,1.12689128020244,7.6841000546184));
#19377=CARTESIAN_POINT('Ctrl Pts',(2.26044091766316,1.10843906449759,7.68278552761173));
#19378=CARTESIAN_POINT('Ctrl Pts',(2.27487489086101,1.07838444153065,7.68066985760226));
#19379=CARTESIAN_POINT('Ctrl Pts',(2.28030665785984,1.06685065901042,7.67986392266788));
#19380=CARTESIAN_POINT('Ctrl Pts',(2.29056158220675,1.04463924136709,7.67832311728845));
#19381=CARTESIAN_POINT('Ctrl Pts',(2.29539825934304,1.033968251417,7.67758779992275));
#19382=CARTESIAN_POINT('Ctrl Pts',(2.30629557412689,1.00947254200333,7.67591088872844));
#19383=CARTESIAN_POINT('Ctrl Pts',(2.31230675814033,0.99562621509304,7.67497099056746));
#19384=CARTESIAN_POINT('Ctrl Pts',(2.3310132988591,0.951453649614908,7.67199710374849));
#19385=CARTESIAN_POINT('Ctrl Pts',(2.34323965518116,0.920931657666336,7.66997882468211));
#19386=CARTESIAN_POINT('Ctrl Pts',(2.35707269506995,0.88433790948212,7.66759887766997));
#19387=CARTESIAN_POINT('Ctrl Pts',(2.35925833630511,0.878490361790436,7.66721976651879));
#19388=CARTESIAN_POINT('Ctrl Pts',(2.36142200378576,0.872635301850924,7.66684133937673));
#19389=CARTESIAN_POINT('Origin',(0.,0.,10.));
#19390=CARTESIAN_POINT('',(2.36142200703877,0.872635293048023,6.67067451578988));
#19391=CARTESIAN_POINT('',(2.36142200728636,0.872635292378025,6.9436622819569));
#19392=CARTESIAN_POINT('',(2.36142200728636,0.87263529237802,10.));
#19393=CARTESIAN_POINT('',(2.51749917428734,0.00203898566820233,7.8874166974512));
#19394=CARTESIAN_POINT('Ctrl Pts',(2.36142200728635,0.872635292378026,6.9436622819569));
#19395=CARTESIAN_POINT('Ctrl Pts',(2.33099320995247,0.954978090459999,6.94922798284441));
#19396=CARTESIAN_POINT('Ctrl Pts',(2.29629372475297,1.0356188703594,6.95479368373192));
#19397=CARTESIAN_POINT('Ctrl Pts',(2.25754798994522,1.11412895263263,6.96035938461943));
#19398=CARTESIAN_POINT('Ctrl Pts',(2.24918575763024,1.13107325760698,6.96156059254717));
#19399=CARTESIAN_POINT('Ctrl Pts',(2.24063521552867,1.14791841827325,6.96276180047491));
#19400=CARTESIAN_POINT('Ctrl Pts',(2.23189888544184,1.16466030032945,6.96396300840265));
#19401=CARTESIAN_POINT('Ctrl Pts',(2.19367769787667,1.23790554265705,6.96921825780996));
#19402=CARTESIAN_POINT('Ctrl Pts',(2.15177652201526,1.30940257330376,6.97447350721726));
#19403=CARTESIAN_POINT('Ctrl Pts',(2.1063792225828,1.37875770919747,6.97972875662457));
#19404=CARTESIAN_POINT('Ctrl Pts',(2.06104628620795,1.44801451526404,6.98497655528206));
#19405=CARTESIAN_POINT('Ctrl Pts',(2.01222732233057,1.51513507554269,6.99022435393955));
#19406=CARTESIAN_POINT('Ctrl Pts',(1.96015236693439,1.57974964738135,6.99547215259704));
#19407=CARTESIAN_POINT('Ctrl Pts',(1.9077000835924,1.64483240749739,7.00075797607995));
#19408=CARTESIAN_POINT('Ctrl Pts',(1.85194464393797,1.70737228971862,7.00604379956286));
#19409=CARTESIAN_POINT('Ctrl Pts',(1.79316602057124,1.76702062032923,7.01132962304577));
#19410=CARTESIAN_POINT('Ctrl Pts',(1.73491446106303,1.8261340884765,7.01656804891436));
#19411=CARTESIAN_POINT('Ctrl Pts',(1.67369404788882,1.88240731928882,7.02180647478295));
#19412=CARTESIAN_POINT('Ctrl Pts',(1.60981694875901,1.93553497552698,7.02704490065154));
#19413=CARTESIAN_POINT('Ctrl Pts',(1.54596085774405,1.98864515896316,7.03228160368904));
#19414=CARTESIAN_POINT('Ctrl Pts',(1.47945017054394,2.03861152762981,7.03751830672654));
#19415=CARTESIAN_POINT('Ctrl Pts',(1.41063142108491,2.08516791742247,7.04275500976405));
#19416=CARTESIAN_POINT('Ctrl Pts',(1.34181454621417,2.13172303904238,7.04799157015638));
#19417=CARTESIAN_POINT('Ctrl Pts',(1.27069011684549,2.17486810877582,7.05322813054871));
#19418=CARTESIAN_POINT('Ctrl Pts',(1.19763387775308,2.21438012654967,7.05846469094104));
#19419=CARTESIAN_POINT('Ctrl Pts',(1.12338190495437,2.25453884954737,7.06378695971153));
#19420=CARTESIAN_POINT('Ctrl Pts',(1.04713474113611,2.29094427560596,7.06910922848201));
#19421=CARTESIAN_POINT('Ctrl Pts',(0.96931146732795,2.32341161426609,7.07443149725249));
#19422=CARTESIAN_POINT('Ctrl Pts',(0.892631474320322,2.35540198397955,7.07967557800282));
#19423=CARTESIAN_POINT('Ctrl Pts',(0.814421833479111,2.38356910416803,7.08491965875315));
#19424=CARTESIAN_POINT('Ctrl Pts',(0.735100417157203,2.40778604254932,7.09016373950348));
#19425=CARTESIAN_POINT('Ctrl Pts',(0.654005005126743,2.43254458428005,7.09552510228404));
#19426=CARTESIAN_POINT('Ctrl Pts',(0.571747985256415,2.45317399867889,7.1008864650646));
#19427=CARTESIAN_POINT('Ctrl Pts',(0.488786758667984,2.46959384404619,7.10624782784515));
#19428=CARTESIAN_POINT('Ctrl Pts',(0.405825532079546,2.48601368941349,7.11160919062571));
#19429=CARTESIAN_POINT('Ctrl Pts',(0.322160611200065,2.49822395846984,7.11697055340626));
#19430=CARTESIAN_POINT('Ctrl Pts',(0.238252757484204,2.50620068501131,7.12233191618682));
#19431=CARTESIAN_POINT('Ctrl Pts',(0.15600562805885,2.51401953427504,7.12758716559413));
#19432=CARTESIAN_POINT('Ctrl Pts',(0.0732213097317949,2.51779982116763,
7.13284241500143));
#19433=CARTESIAN_POINT('Ctrl Pts',(-0.00966987373661683,2.51748142863893,
7.13809766440874));
#19434=CARTESIAN_POINT('Ctrl Pts',(-0.0924435363375321,2.51716348751851,
7.14334546306624));
#19435=CARTESIAN_POINT('Ctrl Pts',(-0.175323305567867,2.51275841106904,
7.14859326172374));
#19436=CARTESIAN_POINT('Ctrl Pts',(-0.257873800693118,2.50425784473486,
7.15384106038124));
#19437=CARTESIAN_POINT('Ctrl Pts',(-0.341022445322447,2.49569568446924,
7.15912688386415));
#19438=CARTESIAN_POINT('Ctrl Pts',(-0.423836552202102,2.48297838833264,
7.16441270734705));
#19439=CARTESIAN_POINT('Ctrl Pts',(-0.50587122499004,2.46615095923325,7.16969853082996));
#19440=CARTESIAN_POINT('Ctrl Pts',(-0.5871702985296,2.44947442052907,7.17493695669855));
#19441=CARTESIAN_POINT('Ctrl Pts',(-0.667703399917476,2.42876125862326,
7.18017538256715));
#19442=CARTESIAN_POINT('Ctrl Pts',(-0.747044454435779,2.40410707604648,
7.18541380843574));
#19443=CARTESIAN_POINT('Ctrl Pts',(-0.82635941500168,2.37946100182004,7.19065051147325));
#19444=CARTESIAN_POINT('Ctrl Pts',(-0.904482667029787,2.35087661793432,
7.19588721451076));
#19445=CARTESIAN_POINT('Ctrl Pts',(-0.98100228318559,2.31849968091105,7.20112391754826));
#19446=CARTESIAN_POINT('Ctrl Pts',(-1.05751981498533,2.28612362581935,7.2063604779406));
#19447=CARTESIAN_POINT('Ctrl Pts',(-1.13243337321921,2.24995540374432,7.21159703833294));
#19448=CARTESIAN_POINT('Ctrl Pts',(-1.20535133231742,2.21018877376585,7.21683359872527));
#19449=CARTESIAN_POINT('Ctrl Pts',(-1.27946276185111,2.16977127124811,7.22215586749575));
#19450=CARTESIAN_POINT('Ctrl Pts',(-1.35151223973342,2.12563672951816,7.22747813626623));
#19451=CARTESIAN_POINT('Ctrl Pts',(-1.4211165958319,2.07803606105648,7.23280040503671));
#19452=CARTESIAN_POINT('Ctrl Pts',(-1.48969841304116,2.03113468122247,7.23804448578704));
#19453=CARTESIAN_POINT('Ctrl Pts',(-1.55590613719537,1.98086867041449,7.24328856653737));
#19454=CARTESIAN_POINT('Ctrl Pts',(-1.61940578722062,1.92751942825912,7.24853264728771));
#19455=CARTESIAN_POINT('Ctrl Pts',(-1.68432558468972,1.87297704897861,7.25389401006826));
#19456=CARTESIAN_POINT('Ctrl Pts',(-1.74641434121004,1.81521221218204,7.25925537284881));
#19457=CARTESIAN_POINT('Ctrl Pts',(-1.80535555014973,1.75456478579264,7.26461673562936));
#19458=CARTESIAN_POINT('Ctrl Pts',(-1.86429675908941,1.69391735940324,7.26997809840991));
#19459=CARTESIAN_POINT('Ctrl Pts',(-1.92009013535083,1.63038776927758,7.27533946119046));
#19460=CARTESIAN_POINT('Ctrl Pts',(-1.97246471397379,1.564349450132,7.28070082397101));
#19461=CARTESIAN_POINT('Ctrl Pts',(-2.0238026824218,1.49961817717873,7.28595607337832));
#19462=CARTESIAN_POINT('Ctrl Pts',(-2.07204560924577,1.43223751273171,7.29121132278562));
#19463=CARTESIAN_POINT('Ctrl Pts',(-2.11690877828477,1.36253567821944,7.29646657219293));
#19464=CARTESIAN_POINT('Ctrl Pts',(-2.16170834154174,1.29293266507416,7.30171437085042));
#19465=CARTESIAN_POINT('Ctrl Pts',(-2.20313741713624,1.22101540329665,7.30696216950792));
#19466=CARTESIAN_POINT('Ctrl Pts',(-2.24095195361088,1.14714453823725,7.31220996816541));
#19467=CARTESIAN_POINT('Ctrl Pts',(-2.27904048900228,1.07273841507627,7.31749579164832));
#19468=CARTESIAN_POINT('Ctrl Pts',(-2.31346158888117,0.996350629387539,
7.32278161513123));
#19469=CARTESIAN_POINT('Ctrl Pts',(-2.34401077683183,0.918378858694077,
7.32806743861413));
#19470=CARTESIAN_POINT('Ctrl Pts',(-2.37428603232282,0.841106255486374,
7.33330586448272));
#19471=CARTESIAN_POINT('Ctrl Pts',(-2.4007583646804,0.762278398006722,7.33854429035132));
#19472=CARTESIAN_POINT('Ctrl Pts',(-2.42327598752445,0.682304725388445,
7.34378271621991));
#19473=CARTESIAN_POINT('Ctrl Pts',(-2.44578620469709,0.602357354780145,
7.34901941925741));
#19474=CARTESIAN_POINT('Ctrl Pts',(-2.46434417053717,0.521265361257688,
7.35425612229492));
#19475=CARTESIAN_POINT('Ctrl Pts',(-2.47884787001031,0.439453623657098,
7.35949282533242));
#19476=CARTESIAN_POINT('Ctrl Pts',(-2.49335117440993,0.357644114567342,
7.36472938572475));
#19477=CARTESIAN_POINT('Ctrl Pts',(-2.50380035248801,0.275115354896476,
7.36996594611708));
#19478=CARTESIAN_POINT('Ctrl Pts',(-2.51014470671314,0.192301329584641,
7.37520250650941));
#19479=CARTESIAN_POINT('Ctrl Pts',(-2.51659290091533,0.108131861908805,
7.38052477527989));
#19480=CARTESIAN_POINT('Ctrl Pts',(-2.51880063850722,0.0236681955690314,
7.38584704405037));
#19481=CARTESIAN_POINT('Ctrl Pts',(-2.51676976536495,-0.0606316595919791,
7.39116931282085));
#19482=CARTESIAN_POINT('Ctrl Pts',(-2.5147687272342,-0.143693088236424,
7.39641339357118));
#19483=CARTESIAN_POINT('Ctrl Pts',(-2.50865288393014,-0.226595024528087,
7.40165747432152));
#19484=CARTESIAN_POINT('Ctrl Pts',(-2.49847643477153,-0.308904119252801,
7.40690155507185));
#19485=CARTESIAN_POINT('Ctrl Pts',(-2.48807239288989,-0.393054028067616,
7.4122629178524));
#19486=CARTESIAN_POINT('Ctrl Pts',(-2.47342401384052,-0.476583753600546,
7.41762428063296));
#19487=CARTESIAN_POINT('Ctrl Pts',(-2.45464405368561,-0.559042770909252,
7.42298564341351));
#19488=CARTESIAN_POINT('Ctrl Pts',(-2.43586409353069,-0.641501788217963,
7.42834700619406));
#19489=CARTESIAN_POINT('Ctrl Pts',(-2.41295275425359,-0.722889626306476,
7.43370836897462));
#19490=CARTESIAN_POINT('Ctrl Pts',(-2.38607574271783,-0.802775684742356,
7.43906973175517));
#19491=CARTESIAN_POINT('Ctrl Pts',(-2.35973068741663,-0.881080619220939,
7.44432498116248));
#19492=CARTESIAN_POINT('Ctrl Pts',(-2.32947824272636,-0.958231921997537,
7.44958023056978));
#19493=CARTESIAN_POINT('Ctrl Pts',(-2.2954387040908,-1.03381207468376,7.45483547997709));
#19494=CARTESIAN_POINT('Ctrl Pts',(-2.26144742578818,-1.10928507188319,
7.46008327863458));
#19495=CARTESIAN_POINT('Ctrl Pts',(-2.22367990631756,-1.18319092631449,
7.46533107729208));
#19496=CARTESIAN_POINT('Ctrl Pts',(-2.18230577801954,-1.25512857557404,
7.47057887594957));
#19497=CARTESIAN_POINT('Ctrl Pts',(-2.14063185849326,-1.32758747512011,
7.47586469943248));
#19498=CARTESIAN_POINT('Ctrl Pts',(-2.09529899473707,-1.39804907730857,
7.48115052291539));
#19499=CARTESIAN_POINT('Ctrl Pts',(-2.04652942808554,-1.46612535275121,
7.48643634639829));
#19500=CARTESIAN_POINT('Ctrl Pts',(-1.99819717477185,-1.53359119293094,
7.49167477226689));
#19501=CARTESIAN_POINT('Ctrl Pts',(-1.94648987873685,-1.5987139311414,7.49691319813548));
#19502=CARTESIAN_POINT('Ctrl Pts',(-1.89166833403524,-1.66114333036266,
7.50215162400407));
#19503=CARTESIAN_POINT('Ctrl Pts',(-1.83686481922731,-1.7235521975935,7.50738832704157));
#19504=CARTESIAN_POINT('Ctrl Pts',(-1.77894939414191,-1.78326913862989,
7.51262503007908));
#19505=CARTESIAN_POINT('Ctrl Pts',(-1.71822290162412,-1.8399772581025,7.51786173311658));
#19506=CARTESIAN_POINT('Ctrl Pts',(-1.65749806326561,-1.8966838328743,7.52309829350892));
#19507=CARTESIAN_POINT('Ctrl Pts',(-1.59396264766415,-1.95038143486611,
7.52833485390125));
#19508=CARTESIAN_POINT('Ctrl Pts',(-1.52795307568929,-2.00079125560156,
7.53357141429358));
#19509=CARTESIAN_POINT('Ctrl Pts',(-1.46086310495409,-2.05202614921965,
7.53889368306406));
#19510=CARTESIAN_POINT('Ctrl Pts',(-1.39121763942827,-2.09986435746919,
7.54421595183454));
#19511=CARTESIAN_POINT('Ctrl Pts',(-1.31940185922458,-2.14405806448303,
7.54953822060503));
#19512=CARTESIAN_POINT('Ctrl Pts',(-1.24864110534737,-2.18760253362418,
7.55478230135536));
#19513=CARTESIAN_POINT('Ctrl Pts',(-1.17577382032524,-2.22760870007047,
7.56002638210569));
#19514=CARTESIAN_POINT('Ctrl Pts',(-1.10119300303954,-2.26388608813623,
7.56527046285603));
#19515=CARTESIAN_POINT('Ctrl Pts',(-1.02494421188322,-2.30097480728671,
7.57063182563658));
#19516=CARTESIAN_POINT('Ctrl Pts',(-0.946904789682583,-2.33416574940922,
7.57599318841714));
#19517=CARTESIAN_POINT('Ctrl Pts',(-0.867514023497643,-2.3633082044107,
7.58135455119769));
#19518=CARTESIAN_POINT('Ctrl Pts',(-0.788123257312707,-2.39245065941218,
7.58671591397825));
#19519=CARTESIAN_POINT('Ctrl Pts',(-0.707381652181406,-2.4175445402802,
7.5920772767588));
#19520=CARTESIAN_POINT('Ctrl Pts',(-0.625740611784981,-2.43849439957589,
7.59743863953936));
#19521=CARTESIAN_POINT('Ctrl Pts',(-0.54571543036819,-2.45902961425042,
7.60269388894667));
#19522=CARTESIAN_POINT('Ctrl Pts',(-0.464530522070502,-2.47565924426919,
7.60794913835397));
#19523=CARTESIAN_POINT('Ctrl Pts',(-0.382601593137168,-2.48825687398406,
7.61320438776128));
#19524=CARTESIAN_POINT('Ctrl Pts',(-0.300788820813074,-2.50083664312182,
7.61845218641877));
#19525=CARTESIAN_POINT('Ctrl Pts',(-0.21823457535389,-2.50939569697438,
7.62369998507627));
#19526=CARTESIAN_POINT('Ctrl Pts',(-0.135367621402295,-2.51385796278865,
7.62894778373376));
#19527=CARTESIAN_POINT('Ctrl Pts',(-0.0519002249295223,-2.51835256156567,
7.63423360721667));
#19528=CARTESIAN_POINT('Ctrl Pts',(0.031883971826203,-2.51869063448652,
7.63951943069957));
#19529=CARTESIAN_POINT('Ctrl Pts',(0.115538493166088,-2.51484733266195,
7.64480525418248));
#19530=CARTESIAN_POINT('Ctrl Pts',(0.19844289018743,-2.51103849345955,7.65004368005107));
#19531=CARTESIAN_POINT('Ctrl Pts',(0.281219458631735,-2.50312298893552,
7.65528210591966));
#19532=CARTESIAN_POINT('Ctrl Pts',(0.36343243265852,-2.4911288840387,7.66052053178826));
#19533=CARTESIAN_POINT('Ctrl Pts',(0.44561836820636,-2.47913872380338,7.66575723482576));
#19534=CARTESIAN_POINT('Ctrl Pts',(0.5272406212384,-2.46307269381636,7.67099393786327));
#19535=CARTESIAN_POINT('Ctrl Pts',(0.607869588007,-2.44301060455664,7.67623064090077));
#19536=CARTESIAN_POINT('Ctrl Pts',(0.688496358482866,-2.4229490617782,7.6814672012931));
#19537=CARTESIAN_POINT('Ctrl Pts',(0.76812944897189,-2.39889178856426,7.68670376168544));
#19538=CARTESIAN_POINT('Ctrl Pts',(0.846351832207465,-2.3709691744346,7.69194032207777));
#19539=CARTESIAN_POINT('Ctrl Pts',(0.925854505003288,-2.34258954237878,
7.69726259084825));
#19540=CARTESIAN_POINT('Ctrl Pts',(1.00389940744476,-2.31021705035651,7.70258485961873));
#19541=CARTESIAN_POINT('Ctrl Pts',(1.08006896158071,-2.27403986073903,7.70790712838921));
#19542=CARTESIAN_POINT('Ctrl Pts',(1.15511952926743,-2.23839414049158,7.71315120913954));
#19543=CARTESIAN_POINT('Ctrl Pts',(1.22834910012129,-2.19905504374563,7.71839528988987));
#19544=CARTESIAN_POINT('Ctrl Pts',(1.2993839357522,-2.15624851014653,7.72363937064021));
#19545=CARTESIAN_POINT('Ctrl Pts',(1.37200744061526,-2.1124846234085,7.72900073342076));
#19546=CARTESIAN_POINT('Ctrl Pts',(1.44233643204523,-2.06509661837745,7.73436209620131));
#19547=CARTESIAN_POINT('Ctrl Pts',(1.51000532505316,-2.01437091130484,7.73972345898186));
#19548=CARTESIAN_POINT('Ctrl Pts',(1.5776742180611,-1.96364520423223,7.74508482176241));
#19549=CARTESIAN_POINT('Ctrl Pts',(1.64268266469297,-1.90958217136595,7.75044618454297));
#19550=CARTESIAN_POINT('Ctrl Pts',(1.70470483693449,-1.85250848012422,7.75580754732352));
#19551=CARTESIAN_POINT('Ctrl Pts',(1.76459909663822,-1.7973929244779,7.76098496764176));
#19552=CARTESIAN_POINT('Ctrl Pts',(1.82194411214314,-1.73925298659712,7.76616238795999));
#19553=CARTESIAN_POINT('Ctrl Pts',(1.87641220836533,-1.67835737383239,7.77133980827823));
#19554=CARTESIAN_POINT('Ctrl Pts',(1.93078975802769,-1.61756299258898,7.77650862176731));
#19555=CARTESIAN_POINT('Ctrl Pts',(1.9822995759239,-1.55402238995363,7.78167743525639));
#19556=CARTESIAN_POINT('Ctrl Pts',(2.03064882854201,-1.48804287073356,7.78684624874548));
#19557=CARTESIAN_POINT('Ctrl Pts',(2.07895290625881,-1.42212499917313,7.7920102327775));
#19558=CARTESIAN_POINT('Ctrl Pts',(2.12410199614041,-1.35377311300361,7.79717421680953));
#19559=CARTESIAN_POINT('Ctrl Pts',(2.16584248281601,-1.28332871456591,7.80233820084155));
#19560=CARTESIAN_POINT('Ctrl Pts',(2.20755744793516,-1.2129273882348,7.8074990274377));
#19561=CARTESIAN_POINT('Ctrl Pts',(2.24586770342724,-1.14043649738504,7.81265985403386));
#19562=CARTESIAN_POINT('Ctrl Pts',(2.28056296879537,-1.06622642780942,7.81782068063001));
#19563=CARTESIAN_POINT('Ctrl Pts',(2.31524822027094,-0.992037777054395,
7.82298001768681));
#19564=CARTESIAN_POINT('Ctrl Pts',(2.34632035285082,-0.916131364616725,
7.82813935474361));
#19565=CARTESIAN_POINT('Ctrl Pts',(2.37361579836222,-0.838900644751972,
7.83329869180041));
#19566=CARTESIAN_POINT('Ctrl Pts',(2.40092462170801,-0.761632073159203,
7.83846055751191));
#19567=CARTESIAN_POINT('Ctrl Pts',(2.42445289854673,-0.683038346308388,
7.84362242322342));
#19568=CARTESIAN_POINT('Ctrl Pts',(2.44408620525132,-0.603530339999749,
7.84878428893492));
#19569=CARTESIAN_POINT('Ctrl Pts',(2.46372478256877,-0.524000989557537,
7.85394754036286));
#19570=CARTESIAN_POINT('Ctrl Pts',(2.47946621212717,-0.443557337995902,
7.8591107917908));
#19571=CARTESIAN_POINT('Ctrl Pts',(2.49124719851254,-0.362620526037097,
7.86427404321874));
#19572=CARTESIAN_POINT('Ctrl Pts',(2.50304227978826,-0.281586880464179,
7.86944347201251));
#19573=CARTESIAN_POINT('Ctrl Pts',(2.51086741194793,-0.200059370819776,
7.87461290080627));
#19574=CARTESIAN_POINT('Ctrl Pts',(2.51471124598385,-0.118463493627188,
7.87978232960004));
#19575=CARTESIAN_POINT('Ctrl Pts',(2.51660347587099,-0.0782957454756287,
7.88232711888376));
#19576=CARTESIAN_POINT('Ctrl Pts',(2.51753169311342,-0.0381114278833191,
7.88487190816748));
#19577=CARTESIAN_POINT('Ctrl Pts',(2.51749917428734,0.00203898566819532,
7.8874166974512));
#19578=CARTESIAN_POINT('Ctrl Pts',(2.51749917428662,0.00203898656449749,
7.88741669750801));
#19579=CARTESIAN_POINT('Ctrl Pts',(2.51739410665396,0.131764058348535,7.89563885372781));
#19580=CARTESIAN_POINT('Ctrl Pts',(2.50725905023964,0.261092140162662,7.9038610099476));
#19581=CARTESIAN_POINT('Ctrl Pts',(2.487294105771,0.388811369942864,7.91208316616739));
#19582=CARTESIAN_POINT('Ctrl Pts',(2.4855998057872,0.399650102266283,7.91278092914749));
#19583=CARTESIAN_POINT('Ctrl Pts',(2.48383473575149,0.410477266840176,7.91347869212759));
#19584=CARTESIAN_POINT('Ctrl Pts',(2.48199903094351,0.42129213189365,7.91417645510769));
#19585=CARTESIAN_POINT('Ctrl Pts',(2.46817693435167,0.502723584677579,7.91943032123432));
#19586=CARTESIAN_POINT('Ctrl Pts',(2.45031757063398,0.583624430079666,7.92468418736095));
#19587=CARTESIAN_POINT('Ctrl Pts',(2.42847467976397,0.663563847527349,7.92993805348757));
#19588=CARTESIAN_POINT('Ctrl Pts',(2.40920107270496,0.734100340594189,7.93457393029838));
#19589=CARTESIAN_POINT('Ctrl Pts',(2.38682672026174,0.803888074802876,7.93920980710918));
#19590=CARTESIAN_POINT('Ctrl Pts',(2.36142200728636,0.872635292378021,7.94384568391999));
#19591=CARTESIAN_POINT('Ctrl Pts',(2.36142200378576,0.872635301850921,7.66684133937673));
#19592=CARTESIAN_POINT('Ctrl Pts',(2.42086954617539,0.711765423710423,7.656443917513));
#19593=CARTESIAN_POINT('Ctrl Pts',(2.46373111482585,0.545222597560534,7.6466045117527));
#19594=CARTESIAN_POINT('Ctrl Pts',(2.49794968758694,0.318425823046622,7.63342394826705));
#19595=CARTESIAN_POINT('Ctrl Pts',(2.50460219122272,0.260988974035791,7.6300999936721));
#19596=CARTESIAN_POINT('Ctrl Pts',(2.51478615551483,0.135337905865415,7.62277330548585));
#19597=CARTESIAN_POINT('Ctrl Pts',(2.51753071680053,0.0671087438691356,
7.61875974364018));
#19598=CARTESIAN_POINT('Ctrl Pts',(2.5174828384576,-0.03838426666723,7.61238982392487));
#19599=CARTESIAN_POINT('Ctrl Pts',(2.51663955706866,-0.0756187800710945,
7.6101097592111));
#19600=CARTESIAN_POINT('Ctrl Pts',(2.51445058985874,-0.124415604668799,
7.6070641552816));
#19601=CARTESIAN_POINT('Ctrl Pts',(2.51385016514194,-0.13600862687656,7.60633632182352));
#19602=CARTESIAN_POINT('Ctrl Pts',(2.51275196666941,-0.154707939178105,
7.60515485894985));
#19603=CARTESIAN_POINT('Ctrl Pts',(2.51230416142923,-0.161817149623434,
7.60470393691037));
#19604=CARTESIAN_POINT('Ctrl Pts',(2.51137858811787,-0.175579999974779,
7.60382744031686));
#19605=CARTESIAN_POINT('Ctrl Pts',(2.51090453851276,-0.182233761054445,
7.60340207024887));
#19606=CARTESIAN_POINT('Ctrl Pts',(2.50969411076089,-0.198321093604625,
7.60236980833609));
#19607=CARTESIAN_POINT('Ctrl Pts',(2.50893098305654,-0.207752499849492,
7.60176146479519));
#19608=CARTESIAN_POINT('Ctrl Pts',(2.50605732921872,-0.240939165686356,
7.59961023555404));
#19609=CARTESIAN_POINT('Ctrl Pts',(2.50366250386092,-0.264667693276221,
7.59805292332056));
#19610=CARTESIAN_POINT('Ctrl Pts',(2.49688263338409,-0.323469647341974,
7.59415186332088));
#19611=CARTESIAN_POINT('Ctrl Pts',(2.49209541297209,-0.358490865017609,
7.591791389841));
#19612=CARTESIAN_POINT('Ctrl Pts',(2.46812431574152,-0.51000637690205,7.58144887362121));
#19613=CARTESIAN_POINT('Ctrl Pts',(2.44149695168975,-0.625167559692171,
7.57325977652352));
#19614=CARTESIAN_POINT('Ctrl Pts',(2.35764722451197,-0.898621273072675,
7.55351693658072));
#19615=CARTESIAN_POINT('Ctrl Pts',(2.29244872325207,-1.05390571419485,7.54207739813704));
#19616=CARTESIAN_POINT('Ctrl Pts',(2.19642386647353,-1.23070243644216,7.52900225495291));
#19617=CARTESIAN_POINT('Ctrl Pts',(2.18001894668773,-1.25953318799135,7.5268666764399));
#19618=CARTESIAN_POINT('Ctrl Pts',(2.15529873985325,-1.30104689539353,7.52378528451401));
#19619=CARTESIAN_POINT('Ctrl Pts',(2.14743161766961,-1.31399130354971,7.52282354351958));
#19620=CARTESIAN_POINT('Ctrl Pts',(2.13326912531708,-1.33682703688318,7.52112497942315));
#19621=CARTESIAN_POINT('Ctrl Pts',(2.12702064666858,-1.34674677045447,7.52038647885588));
#19622=CARTESIAN_POINT('Ctrl Pts',(2.11384651649111,-1.36734086711533,7.51885175949239));
#19623=CARTESIAN_POINT('Ctrl Pts',(2.1069087604897,-1.37800712139096,7.51805601344013));
#19624=CARTESIAN_POINT('Ctrl Pts',(2.08859499428624,-1.40570144194905,7.51598729921638));
#19625=CARTESIAN_POINT('Ctrl Pts',(2.07709141573814,-1.42264432767221,7.51471910438732));
#19626=CARTESIAN_POINT('Ctrl Pts',(2.02356866872017,-1.49944121594213,7.50895607026972));
#19627=CARTESIAN_POINT('Ctrl Pts',(1.97915849224262,-1.55759020817188,7.5045524668245));
#19628=CARTESIAN_POINT('Ctrl Pts',(1.84133275259981,-1.72262265491989,7.4918184183952));
#19629=CARTESIAN_POINT('Ctrl Pts',(1.74134649792106,-1.82363649798573,7.48372376864114));
#19630=CARTESIAN_POINT('Ctrl Pts',(1.53411076063925,-2.00033204983397,7.46805300434556));
#19631=CARTESIAN_POINT('Ctrl Pts',(1.4284257739737,-2.07711714193046,7.46050517015642));
#19632=CARTESIAN_POINT('Ctrl Pts',(1.29902481214428,-2.15657132556343,7.45118032750939));
#19633=CARTESIAN_POINT('Ctrl Pts',(1.28062391513368,-2.16754876822474,7.44985233013855));
#19634=CARTESIAN_POINT('Ctrl Pts',(1.25479533484955,-2.18251366828983,7.44798228585051));
#19635=CARTESIAN_POINT('Ctrl Pts',(1.24748377003217,-2.18670105029956,7.44745225291942));
#19636=CARTESIAN_POINT('Ctrl Pts',(1.234831706416,-2.1938628658829,7.44653369530755));
#19637=CARTESIAN_POINT('Ctrl Pts',(1.22950108523407,-2.19685472823494,7.4461462652104));
#19638=CARTESIAN_POINT('Ctrl Pts',(1.21822928731429,-2.20312725782635,7.44532603268121));
#19639=CARTESIAN_POINT('Ctrl Pts',(1.21228567728193,-2.20640335022703,7.44489293765851));
#19640=CARTESIAN_POINT('Ctrl Pts',(1.19750016516469,-2.21447528433339,7.44381423856481));
#19641=CARTESIAN_POINT('Ctrl Pts',(1.18864269717609,-2.21924220417729,7.44316686542151));
#19642=CARTESIAN_POINT('Ctrl Pts',(1.15510089447735,-2.23703535406014,7.44071166697805));
#19643=CARTESIAN_POINT('Ctrl Pts',(1.130230088021,-2.24970332421702,7.438883657464));
#19644=CARTESIAN_POINT('Ctrl Pts',(1.06578906603185,-2.28118818425783,7.43413765203379));
#19645=CARTESIAN_POINT('Ctrl Pts',(1.02592979365215,-2.29938980855323,7.43119303300765));
#19646=CARTESIAN_POINT('Ctrl Pts',(0.871522990269123,-2.36508524185316,
7.41980319646024));
#19647=CARTESIAN_POINT('Ctrl Pts',(0.754000131909261,-2.4051326827452,7.41117882048742));
#19648=CARTESIAN_POINT('Ctrl Pts',(0.477485186068167,-2.47708953127256,
7.39150602855232));
#19649=CARTESIAN_POINT('Ctrl Pts',(0.317378312306575,-2.50264912308864,
7.38058152522559));
#19650=CARTESIAN_POINT('Ctrl Pts',(0.133708044302341,-2.51404511139788,
7.36871265873431));
#19651=CARTESIAN_POINT('Ctrl Pts',(0.111497488915577,-2.51512803352212,
7.36728762298061));
#19652=CARTESIAN_POINT('Ctrl Pts',(0.0748956475640587,-2.51642681502144,
7.36495549548775));
#19653=CARTESIAN_POINT('Ctrl Pts',(0.0605120435658942,-2.51681377538387,
7.36404315504224));
#19654=CARTESIAN_POINT('Ctrl Pts',(0.0345180203202891,-2.51729011815153,
7.36240159598778));
#19655=CARTESIAN_POINT('Ctrl Pts',(0.0229088893203318,-2.51742253559902,
7.36167106372806));
#19656=CARTESIAN_POINT('Ctrl Pts',(-0.00200491774711399,-2.5175343554212,
7.36010870821292));
#19657=CARTESIAN_POINT('Ctrl Pts',(-0.0153093963244285,-2.51748860644803,
7.35927768649054));
#19658=CARTESIAN_POINT('Ctrl Pts',(-0.0517570586393679,-2.51707432731513,
7.35700977258154));
#19659=CARTESIAN_POINT('Ctrl Pts',(-0.0748968629791023,-2.51649209757656,
7.35557951644043));
#19660=CARTESIAN_POINT('Ctrl Pts',(-0.2114527605897,-2.51117087350629,7.34719043275331));
#19661=CARTESIAN_POINT('Ctrl Pts',(-0.324458229461923,-2.49908441014914,
7.34046558824129));
#19662=CARTESIAN_POINT('Ctrl Pts',(-0.61201477436361,-2.44848634141086,
7.32348092644027));
#19663=CARTESIAN_POINT('Ctrl Pts',(-0.783955939782015,-2.39896904096846,
7.31346692087066));
#19664=CARTESIAN_POINT('Ctrl Pts',(-1.00596542750272,-2.30859162573154,
7.29926391084281));
#19665=CARTESIAN_POINT('Ctrl Pts',(-1.0618571316909,-2.28342283877398,7.29556804216793));
#19666=CARTESIAN_POINT('Ctrl Pts',(-1.1288793337555,-2.25024893333476,7.29092211732648));
#19667=CARTESIAN_POINT('Ctrl Pts',(-1.14093994739004,-2.24415793334999,
7.29007739767234));
#19668=CARTESIAN_POINT('Ctrl Pts',(-1.15972674276995,-2.23447941008288,
7.28874702770951));
#19669=CARTESIAN_POINT('Ctrl Pts',(-1.16648685512989,-2.23095781339685,
7.2882653430135));
#19670=CARTESIAN_POINT('Ctrl Pts',(-1.17900602773341,-2.22436364919452,
7.28736757623295));
#19671=CARTESIAN_POINT('Ctrl Pts',(-1.18476923265915,-2.221299331308,7.2869520045249));
#19672=CARTESIAN_POINT('Ctrl Pts',(-1.19797544005754,-2.21421152583038,
7.28599451123468));
#19673=CARTESIAN_POINT('Ctrl Pts',(-1.20541010115261,-2.21017291613181,
7.2854516602621));
#19674=CARTESIAN_POINT('Ctrl Pts',(-1.22862677810239,-2.19740931307615,
7.28374482707147));
#19675=CARTESIAN_POINT('Ctrl Pts',(-1.24433509203443,-2.18855239459042,
7.28257305966513));
#19676=CARTESIAN_POINT('Ctrl Pts',(-1.38884285211712,-2.10501502151373,
7.27164523835278));
#19677=CARTESIAN_POINT('Ctrl Pts',(-1.51086285132787,-2.01922204570008,
7.26133757083595));
#19678=CARTESIAN_POINT('Ctrl Pts',(-1.76332579332913,-1.80595609454316,
7.2385080643547));
#19679=CARTESIAN_POINT('Ctrl Pts',(-1.88900737401213,-1.67405749725641,
7.22609022247482));
#19680=CARTESIAN_POINT('Ctrl Pts',(-2.01903637660224,-1.50410819492974,
7.21218873995391));
#19681=CARTESIAN_POINT('Ctrl Pts',(-2.0381669804889,-1.47808148284719,7.21010945771378));
#19682=CARTESIAN_POINT('Ctrl Pts',(-2.06556565544647,-1.4392624020203,7.20707889104254));
#19683=CARTESIAN_POINT('Ctrl Pts',(-2.07422638838818,-1.42675248207603,
7.20611276188839));
#19684=CARTESIAN_POINT('Ctrl Pts',(-2.08936444864689,-1.40445723544223,
7.20440915431779));
#19685=CARTESIAN_POINT('Ctrl Pts',(-2.09588770326426,-1.39470379231312,
7.20366996495082));
#19686=CARTESIAN_POINT('Ctrl Pts',(-2.10932501833041,-1.37430539610771,
7.2021364547265));
#19687=CARTESIAN_POINT('Ctrl Pts',(-2.11622725530086,-1.36365302333363,
7.20134258763454));
#19688=CARTESIAN_POINT('Ctrl Pts',(-2.13397743377333,-1.33579942278446,
7.19928450078525));
#19689=CARTESIAN_POINT('Ctrl Pts',(-2.14469817865072,-1.31851793534113,
7.19802496194301));
#19690=CARTESIAN_POINT('Ctrl Pts',(-2.19219451794774,-1.23984305548966,
7.19236614265402));
#19691=CARTESIAN_POINT('Ctrl Pts',(-2.22655347427037,-1.17702532900818,
7.1880539600011));
#19692=CARTESIAN_POINT('Ctrl Pts',(-2.36222514636639,-0.901714444178392,
7.16986113360819));
#19693=CARTESIAN_POINT('Ctrl Pts',(-2.43613021019673,-0.677087755563914,
7.15687005622727));
#19694=CARTESIAN_POINT('Ctrl Pts',(-2.48712479082669,-0.393460285449062,
7.13969386131856));
#19695=CARTESIAN_POINT('Ctrl Pts',(-2.49483742210367,-0.341154045320238,
7.13648987385414));
#19696=CARTESIAN_POINT('Ctrl Pts',(-2.50238203821092,-0.275786182520685,
7.13239797651873));
#19697=CARTESIAN_POINT('Ctrl Pts',(-2.50376725584618,-0.262913285256533,
7.13158793725552));
#19698=CARTESIAN_POINT('Ctrl Pts',(-2.50579735507217,-0.24257374926059,
7.13030058588439));
#19699=CARTESIAN_POINT('Ctrl Pts',(-2.50650831612172,-0.235113730497315,
7.12982683517828));
#19700=CARTESIAN_POINT('Ctrl Pts',(-2.50771868447863,-0.221783581787762,
7.12897729614917));
#19701=CARTESIAN_POINT('Ctrl Pts',(-2.50823080725063,-0.215914734671706,
7.12860221917862));
#19702=CARTESIAN_POINT('Ctrl Pts',(-2.50941388152144,-0.20178435057446,
7.12769664828832));
#19703=CARTESIAN_POINT('Ctrl Pts',(-2.51006463135081,-0.193521302954794,
7.12716505365914));
#19704=CARTESIAN_POINT('Ctrl Pts',(-2.51193561380513,-0.168164796620101,
7.1255278153761));
#19705=CARTESIAN_POINT('Ctrl Pts',(-2.51302209455952,-0.151062374675916,
7.12441524067728));
#19706=CARTESIAN_POINT('Ctrl Pts',(-2.51515149669146,-0.111098612961105,
7.12179814517295));
#19707=CARTESIAN_POINT('Ctrl Pts',(-2.51605743787149,-0.0882317652370027,
7.1202874643056));
#19708=CARTESIAN_POINT('Ctrl Pts',(-2.51815574540642,-0.00743339158061894,
7.11491008802558));
#19709=CARTESIAN_POINT('Ctrl Pts',(-2.51765970647078,0.0505210312757371,
7.11098171950916));
#19710=CARTESIAN_POINT('Ctrl Pts',(-2.50785362482535,0.278042039756813,
7.09539619441546));
#19711=CARTESIAN_POINT('Ctrl Pts',(-2.48339713259575,0.446523756409464,
7.08353462715593));
#19712=CARTESIAN_POINT('Ctrl Pts',(-2.41861731433399,0.705337811392432,
7.06551368229093));
#19713=CARTESIAN_POINT('Ctrl Pts',(-2.38965197754169,0.797984059906887,
7.05909644524408));
#19714=CARTESIAN_POINT('Ctrl Pts',(-2.34736056592555,0.91006833719209,7.05138258431398));
#19715=CARTESIAN_POINT('Ctrl Pts',(-2.33902269546803,0.931288833148569,
7.04992416233301));
#19716=CARTESIAN_POINT('Ctrl Pts',(-2.32534316838163,0.964761056583153,
7.04762629837541));
#19717=CARTESIAN_POINT('Ctrl Pts',(-2.32019040392467,0.977088147385552,
7.04678060405317));
#19718=CARTESIAN_POINT('Ctrl Pts',(-2.3103791762473,1.00004448547845,7.04520654015534));
#19719=CARTESIAN_POINT('Ctrl Pts',(-2.30574489831994,1.01068362116832,7.04447738077026));
#19720=CARTESIAN_POINT('Ctrl Pts',(-2.29523107927763,1.03437197312589,7.04285446389198));
#19721=CARTESIAN_POINT('Ctrl Pts',(-2.2893134593091,1.04740392612839,7.04196202520934));
#19722=CARTESIAN_POINT('Ctrl Pts',(-2.27150695398942,1.0857459700166,7.03933696433826));
#19723=CARTESIAN_POINT('Ctrl Pts',(-2.25930691941018,1.11090975905745,7.03761498939914));
#19724=CARTESIAN_POINT('Ctrl Pts',(-2.17751221303842,1.27269588043332,7.02653858240463));
#19725=CARTESIAN_POINT('Ctrl Pts',(-2.09597666478979,1.40292702264964,7.01762451166263));
#19726=CARTESIAN_POINT('Ctrl Pts',(-1.90128422003157,1.65866520065164,6.99912838210781));
#19727=CARTESIAN_POINT('Ctrl Pts',(-1.78635893107121,1.78184181425028,6.98960629277691));
#19728=CARTESIAN_POINT('Ctrl Pts',(-1.63787815670527,1.91207487812141,6.97758848348496));
#19729=CARTESIAN_POINT('Ctrl Pts',(-1.61537831608435,1.93112089686188,6.97577351135815));
#19730=CARTESIAN_POINT('Ctrl Pts',(-1.58433462449258,1.9564770835601,6.97326937013832));
#19731=CARTESIAN_POINT('Ctrl Pts',(-1.57607668008897,1.96313552001987,6.9726032447582));
#19732=CARTESIAN_POINT('Ctrl Pts',(-1.56291231315402,1.97361343980111,6.97154090058489));
#19733=CARTESIAN_POINT('Ctrl Pts',(-1.55803328739749,1.97746736552878,6.97114707517961));
#19734=CARTESIAN_POINT('Ctrl Pts',(-1.5478747479719,1.98543062703204,6.97032678232992));
#19735=CARTESIAN_POINT('Ctrl Pts',(-1.54259309688882,1.98953701739896,6.96990010620974));
#19736=CARTESIAN_POINT('Ctrl Pts',(-1.52971787966714,1.999465182298,6.9688596478821));
#19737=CARTESIAN_POINT('Ctrl Pts',(-1.52210740934946,2.00526477901384,6.96824435805372));
#19738=CARTESIAN_POINT('Ctrl Pts',(-1.49486506857249,2.0257805048549,6.96604142887106));
#19739=CARTESIAN_POINT('Ctrl Pts',(-1.47505205245633,2.04025232841725,6.96443845429551));
#19740=CARTESIAN_POINT('Ctrl Pts',(-1.42506245786211,2.07565698184861,6.96039837309672));
#19741=CARTESIAN_POINT('Ctrl Pts',(-1.3946339551262,2.09622297722418,6.95794307234788));
#19742=CARTESIAN_POINT('Ctrl Pts',(-1.25712482122973,2.1848431989041,6.94690011246475));
#19743=CARTESIAN_POINT('Ctrl Pts',(-1.14544277116187,2.24540895759377,6.9380810691353));
#19744=CARTESIAN_POINT('Ctrl Pts',(-0.886673841005095,2.36139230519445,
6.91853101820738));
#19745=CARTESIAN_POINT('Ctrl Pts',(-0.737979219513423,2.41200445029971,
6.90789386807265));
#19746=CARTESIAN_POINT('Ctrl Pts',(-0.553185453308542,2.45619574280637,
6.89554491724946));
#19747=CARTESIAN_POINT('Ctrl Pts',(-0.520698106691311,2.46328750391865,
6.89340401919077));
#19748=CARTESIAN_POINT('Ctrl Pts',(-0.47320454353213,2.47267336799684,6.89031645147102));
#19749=CARTESIAN_POINT('Ctrl Pts',(-0.458304082608395,2.47547844043885,
6.88935376412622));
#19750=CARTESIAN_POINT('Ctrl Pts',(-0.431836657858963,2.4802138696741,6.88765411354523));
#19751=CARTESIAN_POINT('Ctrl Pts',(-0.420279955113492,2.48219832109358,
6.8869154656276));
#19752=CARTESIAN_POINT('Ctrl Pts',(-0.39616143188712,2.48616654511661,6.88538101309589));
#19753=CARTESIAN_POINT('Ctrl Pts',(-0.383597572032591,2.48813602569373,
6.88458567710148));
#19754=CARTESIAN_POINT('Ctrl Pts',(-0.35079556229005,2.49302362545499,6.88251928125985));
#19755=CARTESIAN_POINT('Ctrl Pts',(-0.330535578046118,2.49579057483001,
6.88125297453443));
#19756=CARTESIAN_POINT('Ctrl Pts',(-0.238014243089519,2.50728000259833,
6.87551288149068));
#19757=CARTESIAN_POINT('Ctrl Pts',(-0.165425602166072,2.51311353095782,
6.87112941073162));
#19758=CARTESIAN_POINT('Ctrl Pts',(0.0478727385834268,2.52097134796037,
6.85848611970517));
#19759=CARTESIAN_POINT('Ctrl Pts',(0.188614261977942,2.51436187224441,6.85045753576906));
#19760=CARTESIAN_POINT('Ctrl Pts',(0.459028320221171,2.47881924209878,6.83476672284182));
#19761=CARTESIAN_POINT('Ctrl Pts',(0.588410568258542,2.45132948772839,6.82713045166811));
#19762=CARTESIAN_POINT('Ctrl Pts',(0.735569304664735,2.40773821142667,6.81770542617525));
#19763=CARTESIAN_POINT('Ctrl Pts',(0.756037481914017,2.40138975438664,6.81637721340887));
#19764=CARTESIAN_POINT('Ctrl Pts',(0.784436991520351,2.39218223822322,6.81450691315459));
#19765=CARTESIAN_POINT('Ctrl Pts',(0.792439420611852,2.38954326481827,6.8139768439395));
#19766=CARTESIAN_POINT('Ctrl Pts',(0.806224146581308,2.38492059506494,6.81305824069077));
#19767=CARTESIAN_POINT('Ctrl Pts',(0.812012804647827,2.38295590023679,6.81267080149711));
#19768=CARTESIAN_POINT('Ctrl Pts',(0.824212752112566,2.37876557222836,6.81185057089422));
#19769=CARTESIAN_POINT('Ctrl Pts',(0.830622266320938,2.3765350735141,6.81141748702581));
#19770=CARTESIAN_POINT('Ctrl Pts',(0.846508395869181,2.37093461524189,6.81033885220676));
#19771=CARTESIAN_POINT('Ctrl Pts',(0.855973908993297,2.36753375329956,6.80969153262531));
#19772=CARTESIAN_POINT('Ctrl Pts',(0.891622673758886,2.35448379227934,6.80723677503268));
#19773=CARTESIAN_POINT('Ctrl Pts',(0.917664189133221,2.34445669690555,6.80540916188624));
#19774=CARTESIAN_POINT('Ctrl Pts',(0.984140217100389,2.31758338921996,6.80066443109058));
#19775=CARTESIAN_POINT('Ctrl Pts',(1.02431054739924,2.3001113459173,6.79772070700575));
#19776=CARTESIAN_POINT('Ctrl Pts',(1.23269124837145,2.20293506466281,6.78211423221947));
#19777=CARTESIAN_POINT('Ctrl Pts',(1.39213918512665,2.10580309750223,6.76905649718064));
#19778=CARTESIAN_POINT('Ctrl Pts',(1.5793908308799,1.96109187594669,6.75303776944874));
#19779=CARTESIAN_POINT('Ctrl Pts',(1.61841443154039,1.929013213548,6.74965251004168));
#19780=CARTESIAN_POINT('Ctrl Pts',(1.70060695582346,1.85719705131927,6.74242575782365));
#19781=CARTESIAN_POINT('Ctrl Pts',(1.74340644117043,1.81708002357301,6.73860095886542));
#19782=CARTESIAN_POINT('Ctrl Pts',(1.79861698935554,1.76158131572853,6.73357923578153));
#19783=CARTESIAN_POINT('Ctrl Pts',(1.8123022330649,1.74749891502875,6.73232678688449));
#19784=CARTESIAN_POINT('Ctrl Pts',(1.83445584326564,1.72416219749561,6.73028610887836));
#19785=CARTESIAN_POINT('Ctrl Pts',(1.84302208823742,1.71500236608204,6.72949369709551));
#19786=CARTESIAN_POINT('Ctrl Pts',(1.85950936151041,1.69710642840791,6.72796185833734));
#19787=CARTESIAN_POINT('Ctrl Pts',(1.8674381438087,1.68837794392235,6.72722211447508));
#19788=CARTESIAN_POINT('Ctrl Pts',(1.88303595245279,1.67096263054701,6.72576053145248));
#19789=CARTESIAN_POINT('Ctrl Pts',(1.89070690629874,1.66227792876817,6.72503862251721));
#19790=CARTESIAN_POINT('Ctrl Pts',(1.91540776424453,1.63392054791466,6.72270355687474));
#19791=CARTESIAN_POINT('Ctrl Pts',(1.932193065581,1.61403633621696,6.72110038435432));
#19792=CARTESIAN_POINT('Ctrl Pts',(2.01823620896317,1.50884151779443,6.71278820706795));
#19793=CARTESIAN_POINT('Ctrl Pts',(2.08216626121359,1.41931950555954,6.70629179382278));
#19794=CARTESIAN_POINT('Ctrl Pts',(2.19361501752498,1.23943707110981,6.69399282060017));
#19795=CARTESIAN_POINT('Ctrl Pts',(2.24189448675934,1.14980892096917,6.68818467532153));
#19796=CARTESIAN_POINT('Ctrl Pts',(2.30948432068794,1.0037889419143,6.67891503959213));
#19797=CARTESIAN_POINT('Ctrl Pts',(2.33244594885261,0.949213082436155,6.67548944583528));
#19798=CARTESIAN_POINT('Ctrl Pts',(2.35614736665016,0.886810597765583,6.67156612518863));
#19799=CARTESIAN_POINT('Ctrl Pts',(2.35880073269644,0.879728674404211,6.6711207779961));
#19800=CARTESIAN_POINT('Ctrl Pts',(2.36142200703877,0.872635293048023,6.67067451578988));
#19801=CARTESIAN_POINT('Origin',(0.,0.,10.));
#19802=CARTESIAN_POINT('',(2.36142200559759,0.87263529694796,5.66918223051795));
#19803=CARTESIAN_POINT('',(2.36142200728636,0.872635292378019,5.94377298858649));
#19804=CARTESIAN_POINT('',(2.36142200728636,0.87263529237802,10.));
#19805=CARTESIAN_POINT('',(2.51749998978759,0.0002267586386634,6.8874166975502));
#19806=CARTESIAN_POINT('Ctrl Pts',(2.36142200728636,0.872635292378018,5.94377298858649));
#19807=CARTESIAN_POINT('Ctrl Pts',(2.33300945646759,0.949521963559691,5.94893586779302));
#19808=CARTESIAN_POINT('Ctrl Pts',(2.30084060580699,1.02501176309947,5.95409874699956));
#19809=CARTESIAN_POINT('Ctrl Pts',(2.26508957566429,1.09871536997394,5.95926162620609));
#19810=CARTESIAN_POINT('Ctrl Pts',(2.2293031348659,1.17249197874612,5.96442961913766));
#19811=CARTESIAN_POINT('Ctrl Pts',(2.18992764184852,1.24447843524094,5.96959761206923));
#19812=CARTESIAN_POINT('Ctrl Pts',(2.14718358488262,1.31430928734854,5.9747656050008));
#19813=CARTESIAN_POINT('Ctrl Pts',(2.10441596932025,1.38417862707248,5.979936446297));
#19814=CARTESIAN_POINT('Ctrl Pts',(2.0582763652583,1.45188960658155,5.9851072875932));
#19815=CARTESIAN_POINT('Ctrl Pts',(2.00902761483445,1.51710721204291,5.9902781288894));
#19816=CARTESIAN_POINT('Ctrl Pts',(1.95969848853396,1.58243125517357,5.99545740919976));
#19817=CARTESIAN_POINT('Ctrl Pts',(1.90725039554371,1.64525344003261,6.00063668951012));
#19818=CARTESIAN_POINT('Ctrl Pts',(1.85198488302567,1.70527365635091,6.00581596982048));
#19819=CARTESIAN_POINT('Ctrl Pts',(1.82376641798002,1.73591986406783,6.00846050044619));
#19820=CARTESIAN_POINT('Ctrl Pts',(1.79481399192534,1.7658361884047,6.0111050310719));
#19821=CARTESIAN_POINT('Ctrl Pts',(1.76517104191674,1.79498675281423,6.0137495616976));
#19822=CARTESIAN_POINT('Ctrl Pts',(1.70626414405401,1.85291517491172,6.01900481110491));
#19823=CARTESIAN_POINT('Ctrl Pts',(1.64439384420559,1.90804774175317,6.02426006051221));
#19824=CARTESIAN_POINT('Ctrl Pts',(1.57985623667156,1.96006645842685,6.02951530991952));
#19825=CARTESIAN_POINT('Ctrl Pts',(1.51541012880387,2.01201142437749,6.03476310857701));
#19826=CARTESIAN_POINT('Ctrl Pts',(1.44830458093836,2.06085102195825,6.0400109072345));
#19827=CARTESIAN_POINT('Ctrl Pts',(1.37887225049238,2.10630424365097,6.04525870589199));
#19828=CARTESIAN_POINT('Ctrl Pts',(1.30893682295451,2.1520868131202,6.0505445293749));
#19829=CARTESIAN_POINT('Ctrl Pts',(1.23664108935189,2.19443339293679,6.05583035285781));
#19830=CARTESIAN_POINT('Ctrl Pts',(1.16235873651848,2.23309838960113,6.06111617634071));
#19831=CARTESIAN_POINT('Ctrl Pts',(1.08874246841558,2.27141667990923,6.06635460220931));
#19832=CARTESIAN_POINT('Ctrl Pts',(1.01317548297763,2.30611893065896,6.07159302807789));
#19833=CARTESIAN_POINT('Ctrl Pts',(0.936048763302448,2.3370106894749,6.07683145394649));
#19834=CARTESIAN_POINT('Ctrl Pts',(0.858947409321755,2.36789228850549,6.08206815698399));
#19835=CARTESIAN_POINT('Ctrl Pts',(0.780287767893451,2.3949657131123,6.08730486002149));
#19836=CARTESIAN_POINT('Ctrl Pts',(0.700481465353148,2.41808435888757,6.092541563059));
#19837=CARTESIAN_POINT('Ctrl Pts',(0.620677336696681,2.44120237492247,6.09777812345133));
#19838=CARTESIAN_POINT('Ctrl Pts',(0.539727052516544,2.46036569891565,6.10301468384366));
#19839=CARTESIAN_POINT('Ctrl Pts',(0.458056749044402,2.47547778512651,6.10825124423598));
#19840=CARTESIAN_POINT('Ctrl Pts',(0.375049722851719,2.4908372154531,6.11357351300647));
#19841=CARTESIAN_POINT('Ctrl Pts',(0.291299376297725,2.5020114934577,6.11889578177695));
#19842=CARTESIAN_POINT('Ctrl Pts',(0.207261320091412,2.50895376505705,6.12421805054743));
#19843=CARTESIAN_POINT('Ctrl Pts',(0.124457844383674,2.51579404961007,6.12946213129776));
#19844=CARTESIAN_POINT('Ctrl Pts',(0.0413755260271846,2.51852589088098,
6.13470621204809));
#19845=CARTESIAN_POINT('Ctrl Pts',(-0.0415489796354925,2.51715711315191,
6.13995029279842));
#19846=CARTESIAN_POINT('Ctrl Pts',(-0.126328062838598,2.51575772318808,
6.14531165557898));
#19847=CARTESIAN_POINT('Ctrl Pts',(-0.210941678431173,2.51007211743798,
6.15067301835953));
#19848=CARTESIAN_POINT('Ctrl Pts',(-0.294929867698439,2.50016451921456,
6.15603438114009));
#19849=CARTESIAN_POINT('Ctrl Pts',(-0.378918056965711,2.49025692099114,
6.16139574392065));
#19850=CARTESIAN_POINT('Ctrl Pts',(-0.462280330108473,2.47612748106319,
6.16675710670121));
#19851=CARTESIAN_POINT('Ctrl Pts',(-0.544570910994263,2.45789519160172,
6.17211846948177));
#19852=CARTESIAN_POINT('Ctrl Pts',(-0.625232777039784,2.4400237599699,6.17737371888907));
#19853=CARTESIAN_POINT('Ctrl Pts',(-0.705162930103143,2.41814444185597,
6.18262896829638));
#19854=CARTESIAN_POINT('Ctrl Pts',(-0.783933429501754,2.39233246604848,
6.18788421770368));
#19855=CARTESIAN_POINT('Ctrl Pts',(-0.862592250226629,2.36655708575894,
6.19313201636117));
#19856=CARTESIAN_POINT('Ctrl Pts',(-0.940094248178497,2.33686026505975,
6.19837981501866));
#19857=CARTESIAN_POINT('Ctrl Pts',(-1.01602260056888,2.30336803944425,6.20362761367615));
#19858=CARTESIAN_POINT('Ctrl Pts',(-1.09250111933045,2.2696331337804,6.20891343715906));
#19859=CARTESIAN_POINT('Ctrl Pts',(-1.16738262880088,2.23204769166868,6.21419926064197));
#19860=CARTESIAN_POINT('Ctrl Pts',(-1.24025767266734,2.19079144497823,6.21948508412487));
#19861=CARTESIAN_POINT('Ctrl Pts',(-1.31247925104564,2.14990514020414,6.22472350999347));
#19862=CARTESIAN_POINT('Ctrl Pts',(-1.38272979443769,2.10541383039651,6.22996193586206));
#19863=CARTESIAN_POINT('Ctrl Pts',(-1.45063332633318,2.05753959926207,6.23520036173065));
#19864=CARTESIAN_POINT('Ctrl Pts',(-1.51851452588715,2.00968111316549,6.24043706476815));
#19865=CARTESIAN_POINT('Ctrl Pts',(-1.58404987014721,1.95844218107001,6.24567376780566));
#19866=CARTESIAN_POINT('Ctrl Pts',(-1.64689227786619,1.90408825297167,6.25091047084316));
#19867=CARTESIAN_POINT('Ctrl Pts',(-1.7097329737895,1.84973580544708,6.2561470312355));
#19868=CARTESIAN_POINT('Ctrl Pts',(-1.76988053070197,1.79226883325605,6.26138359162784));
#19869=CARTESIAN_POINT('Ctrl Pts',(-1.8270219562447,1.73199221170298,6.26662015202018));
#19870=CARTESIAN_POINT('Ctrl Pts',(-1.8850986328952,1.67072902433457,6.27194242079066));
#19871=CARTESIAN_POINT('Ctrl Pts',(-1.94006953799678,1.60656373286678,6.27726468956114));
#19872=CARTESIAN_POINT('Ctrl Pts',(-1.99164731274412,1.5398529902686,6.28258695833163));
#19873=CARTESIAN_POINT('Ctrl Pts',(-2.04246737226417,1.47412227726141,6.28783103908196));
#19874=CARTESIAN_POINT('Ctrl Pts',(-2.08999311757048,1.40592082483329,6.29307511983229));
#19875=CARTESIAN_POINT('Ctrl Pts',(-2.13399337392762,1.33561915605947,6.29831920058263));
#19876=CARTESIAN_POINT('Ctrl Pts',(-2.17897768061532,1.26374521507356,6.30368056336318));
#19877=CARTESIAN_POINT('Ctrl Pts',(-2.22027665347001,1.18967643016703,6.30904192614373));
#19878=CARTESIAN_POINT('Ctrl Pts',(-2.25769373727086,1.11383357764432,6.31440328892429));
#19879=CARTESIAN_POINT('Ctrl Pts',(-2.2951108210717,1.03799072512163,6.31976465170484));
#19880=CARTESIAN_POINT('Ctrl Pts',(-2.32864587561046,0.960374297908852,
6.3251260144854));
#19881=CARTESIAN_POINT('Ctrl Pts',(-2.35815600709098,0.881422995060092,
6.33048737726595));
#19882=CARTESIAN_POINT('Ctrl Pts',(-2.38708206699782,0.804034315262673,
6.33574262667326));
#19883=CARTESIAN_POINT('Ctrl Pts',(-2.41224796036822,0.725077290618015,
6.34099787608056));
#19884=CARTESIAN_POINT('Ctrl Pts',(-2.43348379555695,0.644951832900536,
6.34625312548787));
#19885=CARTESIAN_POINT('Ctrl Pts',(-2.45468952315561,0.564939974879646,
6.35150092414538));
#19886=CARTESIAN_POINT('Ctrl Pts',(-2.47197614282722,0.483763416523515,
6.35674872280288));
#19887=CARTESIAN_POINT('Ctrl Pts',(-2.48522243235339,0.40184040579251,6.36199652146039));
#19888=CARTESIAN_POINT('Ctrl Pts',(-2.49856470266681,0.319323792222941,
6.36728234494329));
#19889=CARTESIAN_POINT('Ctrl Pts',(-2.50780767851238,0.23605030714626,6.3725681684262));
#19890=CARTESIAN_POINT('Ctrl Pts',(-2.51287918846666,0.152461254655519,
6.3778539919091));
#19891=CARTESIAN_POINT('Ctrl Pts',(-2.51790522254124,0.0696217394286344,
6.3830924177777));
#19892=CARTESIAN_POINT('Ctrl Pts',(-2.5188342731305,-0.0135272374760142,
6.38833084364629));
#19893=CARTESIAN_POINT('Ctrl Pts',(-2.51564792133638,-0.0965493960413684,
6.39356926951489));
#19894=CARTESIAN_POINT('Ctrl Pts',(-2.51246261748033,-0.179544250000486,
6.39880597255239));
#19895=CARTESIAN_POINT('Ctrl Pts',(-2.50516461702319,-0.262411907738021,
6.4040426755899));
#19896=CARTESIAN_POINT('Ctrl Pts',(-2.4937876084469,-0.34471671551679,6.40927937862741));
#19897=CARTESIAN_POINT('Ctrl Pts',(-2.48241090977468,-0.427019281353452,
6.41451593901973));
#19898=CARTESIAN_POINT('Ctrl Pts',(-2.46695548810174,-0.50875857078144,
6.41975249941204));
#19899=CARTESIAN_POINT('Ctrl Pts',(-2.44750666130293,-0.589506058389383,
6.42498905980436));
#19900=CARTESIAN_POINT('Ctrl Pts',(-2.42773950963489,-0.671575164709831,
6.43031132857484));
#19901=CARTESIAN_POINT('Ctrl Pts',(-2.40384715326946,-0.752619228922703,
6.43563359734532));
#19902=CARTESIAN_POINT('Ctrl Pts',(-2.37597229701536,-0.832203036413311,
6.4409558661158));
#19903=CARTESIAN_POINT('Ctrl Pts',(-2.34850694278311,-0.910617699576286,
6.44619994686614));
#19904=CARTESIAN_POINT('Ctrl Pts',(-2.31717555686965,-0.987614315326444,
6.45144402761647));
#19905=CARTESIAN_POINT('Ctrl Pts',(-2.2821630677264,-1.06279724421248,6.45668810836681));
#19906=CARTESIAN_POINT('Ctrl Pts',(-2.24636753652009,-1.13966161298417,
6.46204947114736));
#19907=CARTESIAN_POINT('Ctrl Pts',(-2.20672450140766,-1.21462973836723,
6.46741083392791));
#19908=CARTESIAN_POINT('Ctrl Pts',(-2.16347989151026,-1.287307659043,6.47277219670846));
#19909=CARTESIAN_POINT('Ctrl Pts',(-2.12023528161285,-1.35998557971878,
6.47813355948902));
#19910=CARTESIAN_POINT('Ctrl Pts',(-2.07338943405647,-1.43037290970729,
6.48349492226957));
#19911=CARTESIAN_POINT('Ctrl Pts',(-2.02323252747283,-1.49811094040992,
6.48885628505012));
#19912=CARTESIAN_POINT('Ctrl Pts',(-1.9740683383692,-1.56450828382301,6.49411153445743));
#19913=CARTESIAN_POINT('Ctrl Pts',(-1.92154140516665,-1.62860551635464,
6.49936678386474));
#19914=CARTESIAN_POINT('Ctrl Pts',(-1.86589467300489,-1.69004240161363,
6.50462203327205));
#19915=CARTESIAN_POINT('Ctrl Pts',(-1.81032683526795,-1.75139218332606,
6.50986983192955));
#19916=CARTESIAN_POINT('Ctrl Pts',(-1.75164829144652,-1.81008877046015,
6.51511763058705));
#19917=CARTESIAN_POINT('Ctrl Pts',(-1.69014386507699,-1.8658027669994,6.52036542924455));
#19918=CARTESIAN_POINT('Ctrl Pts',(-1.62819378611535,-1.92192045947471,
6.52565125272745));
#19919=CARTESIAN_POINT('Ctrl Pts',(-1.56337698190049,-1.97501177524926,
6.53093707621036));
#19920=CARTESIAN_POINT('Ctrl Pts',(-1.49602432105693,-2.02477590878747,
6.53622289969326));
#19921=CARTESIAN_POINT('Ctrl Pts',(-1.42927560687406,-2.07409381077528,
6.54146132556186));
#19922=CARTESIAN_POINT('Ctrl Pts',(-1.36003670956918,-2.12014368151662,
6.54669975143045));
#19923=CARTESIAN_POINT('Ctrl Pts',(-1.28866354925699,-2.16267253804555,
6.55193817729905));
#19924=CARTESIAN_POINT('Ctrl Pts',(-1.21731386238938,-2.20518740754137,
6.55717488033656));
#19925=CARTESIAN_POINT('Ctrl Pts',(-1.14383170264659,-2.24418332667548,
6.56241158337407));
#19926=CARTESIAN_POINT('Ctrl Pts',(-1.06860083476897,-2.27945136072939,
6.56764828641158));
#19927=CARTESIAN_POINT('Ctrl Pts',(-0.993372016142759,-2.31471843409959,
6.5728848468039));
#19928=CARTESIAN_POINT('Ctrl Pts',(-0.916395002317771,-2.34625762936338,
6.57812140719623));
#19929=CARTESIAN_POINT('Ctrl Pts',(-0.838075688553231,-2.37390719916681,
6.58335796758855));
#19930=CARTESIAN_POINT('Ctrl Pts',(-0.758474498736846,-2.40200931789683,
6.58868023635903));
#19931=CARTESIAN_POINT('Ctrl Pts',(-0.677487132195189,-2.42609316097627,
6.59400250512951));
#19932=CARTESIAN_POINT('Ctrl Pts',(-0.59555633944533,-2.44604147482141,
6.59932477389999));
#19933=CARTESIAN_POINT('Ctrl Pts',(-0.514829169952893,-2.46569673334895,
6.60456885465032));
#19934=CARTESIAN_POINT('Ctrl Pts',(-0.433186580706483,-2.4813371362005,
6.60981293540065));
#19935=CARTESIAN_POINT('Ctrl Pts',(-0.351061115609648,-2.49290239341754,
6.61505701615098));
#19936=CARTESIAN_POINT('Ctrl Pts',(-0.267098943234972,-2.50472630356368,
6.62041837893153));
#19937=CARTESIAN_POINT('Ctrl Pts',(-0.182632545677713,-2.5122905444431,
6.62577974171208));
#19938=CARTESIAN_POINT('Ctrl Pts',(-0.0981262711465387,-2.51558690665039,
6.63114110449264));
#19939=CARTESIAN_POINT('Ctrl Pts',(-0.0136199966153704,-2.51888326885768,
6.63650246727319));
#19940=CARTESIAN_POINT('Ctrl Pts',(0.070925647583907,-2.51791182502412,
6.64186383005375));
#19941=CARTESIAN_POINT('Ctrl Pts',(0.155051791237123,-2.51272067529086,
6.6472251928343));
#19942=CARTESIAN_POINT('Ctrl Pts',(0.237512890153206,-2.50763227003354,
6.6524804422416));
#19943=CARTESIAN_POINT('Ctrl Pts',(0.319875525080888,-2.49847092200906,
6.6577356916489));
#19944=CARTESIAN_POINT('Ctrl Pts',(0.401705260653849,-2.48524428046078,
6.66299094105621));
#19945=CARTESIAN_POINT('Ctrl Pts',(0.483418980251289,-2.47203639128548,
6.6682387397137));
#19946=CARTESIAN_POINT('Ctrl Pts',(0.564600849488969,-2.4547747299151,6.6734865383712));
#19947=CARTESIAN_POINT('Ctrl Pts',(0.644819500910465,-2.43351886395926,
6.67873433702869));
#19948=CARTESIAN_POINT('Ctrl Pts',(0.725619405618183,-2.41210898092985,
6.6840201605116));
#19949=CARTESIAN_POINT('Ctrl Pts',(0.80544160193643,-2.38664679535527,6.68930598399451));
#19950=CARTESIAN_POINT('Ctrl Pts',(0.883853634563512,-2.35724606324178,
6.69459180747741));
#19951=CARTESIAN_POINT('Ctrl Pts',(0.961562551906455,-2.32810896546375,
6.69983023334601));
#19952=CARTESIAN_POINT('Ctrl Pts',(1.03788605394017,-2.29510383658063,6.7050686592146));
#19953=CARTESIAN_POINT('Ctrl Pts',(1.1124181592425,-2.25839148266803,6.71030708508319));
#19954=CARTESIAN_POINT('Ctrl Pts',(1.18692575217586,-2.22169120283763,6.7155437881207));
#19955=CARTESIAN_POINT('Ctrl Pts',(1.25964270487964,-2.18128632319353,6.72078049115821));
#19956=CARTESIAN_POINT('Ctrl Pts',(1.33018482321191,-2.13738498780559,6.72601719419572));
#19957=CARTESIAN_POINT('Ctrl Pts',(1.40072502001207,-2.09348484826812,6.73125375458805));
#19958=CARTESIAN_POINT('Ctrl Pts',(1.46909010902144,-2.04608868703051,6.73649031498038));
#19959=CARTESIAN_POINT('Ctrl Pts',(1.53492342749988,-1.99544890230545,6.74172687537271));
#19960=CARTESIAN_POINT('Ctrl Pts',(1.601834259944,-1.94398028080713,6.74704914414319));
#19961=CARTESIAN_POINT('Ctrl Pts',(1.66612929985463,-1.8891611885151,6.75237141291367));
#19962=CARTESIAN_POINT('Ctrl Pts',(1.72746913962016,-1.83129916225066,6.75769368168415));
#19963=CARTESIAN_POINT('Ctrl Pts',(1.78790785228484,-1.7742871714636,6.76293776243449));
#19964=CARTESIAN_POINT('Ctrl Pts',(1.84547733669641,-1.71432143920906,6.76818184318483));
#19965=CARTESIAN_POINT('Ctrl Pts',(1.8998915228993,-1.6517319550143,6.77342592393516));
#19966=CARTESIAN_POINT('Ctrl Pts',(1.95552266332814,-1.58774267891589,6.77878728671571));
#19967=CARTESIAN_POINT('Ctrl Pts',(2.00785535222641,-1.52101127904257,6.78414864949626));
#19968=CARTESIAN_POINT('Ctrl Pts',(2.05662988850108,-1.4519227774658,6.78951001227682));
#19969=CARTESIAN_POINT('Ctrl Pts',(2.10540442477576,-1.38283427588904,6.79487137505737));
#19970=CARTESIAN_POINT('Ctrl Pts',(2.15062059314599,-1.31138913767725,6.80023273783792));
#19971=CARTESIAN_POINT('Ctrl Pts',(2.19206890703465,-1.23799844782291,6.80559410061847));
#19972=CARTESIAN_POINT('Ctrl Pts',(2.23446890777386,-1.16292264829979,6.81107856462994));
#19973=CARTESIAN_POINT('Ctrl Pts',(2.27307163741378,-1.08555429773617,6.81656302864142));
#19974=CARTESIAN_POINT('Ctrl Pts',(2.30763425924484,-1.00629537192593,6.82204749265289));
#19975=CARTESIAN_POINT('Ctrl Pts',(2.3421071209173,-0.927242283907316,6.82751771334793));
#19976=CARTESIAN_POINT('Ctrl Pts',(2.37256061323794,-0.846308768248659,
6.83298793404297));
#19977=CARTESIAN_POINT('Ctrl Pts',(2.39879783154463,-0.76392094707293,6.83845815473802));
#19978=CARTESIAN_POINT('Ctrl Pts',(2.42499481295722,-0.681659474277432,
6.84391998640766));
#19979=CARTESIAN_POINT('Ctrl Pts',(2.44698825905869,-0.597948514162592,
6.8493818180773));
#19980=CARTESIAN_POINT('Ctrl Pts',(2.46462916087108,-0.513234205196725,
6.85484364974695));
#19981=CARTESIAN_POINT('Ctrl Pts',(2.48223686891343,-0.428679297792125,
6.86029520423312));
#19982=CARTESIAN_POINT('Ctrl Pts',(2.49550826265312,-0.343125195357741,
6.8657467587193));
#19983=CARTESIAN_POINT('Ctrl Pts',(2.50434439920537,-0.257031866056912,
6.87119831320548));
#19984=CARTESIAN_POINT('Ctrl Pts',(2.51310690653042,-0.171655930072285,
6.87660444130632));
#19985=CARTESIAN_POINT('Ctrl Pts',(2.51750773395471,-0.0857501128064433,
6.88201056940717));
#19986=CARTESIAN_POINT('Ctrl Pts',(2.51749998978765,0.000226757967686038,
6.88741669750801));
#19987=CARTESIAN_POINT('Ctrl Pts',(2.51749998978759,0.000226758638666253,
6.8874166975502));
#19988=CARTESIAN_POINT('Ctrl Pts',(2.51749207334366,0.0881160122807311,
6.89294307411638));
#19989=CARTESIAN_POINT('Ctrl Pts',(2.51287736989993,0.175904347014042,6.89846945068255));
#19990=CARTESIAN_POINT('Ctrl Pts',(2.50371314433435,0.263109750650595,6.90399582724873));
#19991=CARTESIAN_POINT('Ctrl Pts',(2.49453499561041,0.350447644985407,6.90953060000895));
#19992=CARTESIAN_POINT('Ctrl Pts',(2.48079359631616,0.43720046548662,6.91506537276916));
#19993=CARTESIAN_POINT('Ctrl Pts',(2.46259736788571,0.522896216932551,6.92060014552938));
#19994=CARTESIAN_POINT('Ctrl Pts',(2.44435527462668,0.60880797033544,6.92614886905993));
#19995=CARTESIAN_POINT('Ctrl Pts',(2.42163600591916,0.693656960244299,6.93169759259049));
#19996=CARTESIAN_POINT('Ctrl Pts',(2.39459808317596,0.776985373124874,6.93724631612104));
#19997=CARTESIAN_POINT('Ctrl Pts',(2.38417680414139,0.809102805014325,6.93938497139966));
#19998=CARTESIAN_POINT('Ctrl Pts',(2.37311446244257,0.840994558653117,6.94152362667828));
#19999=CARTESIAN_POINT('Ctrl Pts',(2.36142200728635,0.872635292378026,6.9436622819569));
#20000=CARTESIAN_POINT('',(2.51749891107627,0.00228349541106654,6.61240052779172));
#20001=CARTESIAN_POINT('Ctrl Pts',(2.36142200703877,0.872635293048023,6.67067451578988));
#20002=CARTESIAN_POINT('Ctrl Pts',(2.38467103606877,0.809721531444391,6.66671645507875));
#20003=CARTESIAN_POINT('Ctrl Pts',(2.40539555026188,0.745906400452688,6.66268671174773));
#20004=CARTESIAN_POINT('Ctrl Pts',(2.42706372989967,0.66883240968557,6.65771882192992));
#20005=CARTESIAN_POINT('Ctrl Pts',(2.43048394040097,0.656294857644221,6.65690755437749));
#20006=CARTESIAN_POINT('Ctrl Pts',(2.4359017972833,0.6358111417721,6.65557615329902));
#20007=CARTESIAN_POINT('Ctrl Pts',(2.43795803848093,0.627880539714219,6.65505922957548));
#20008=CARTESIAN_POINT('Ctrl Pts',(2.44157840260655,0.613631423224701,6.65412762765142));
#20009=CARTESIAN_POINT('Ctrl Pts',(2.44315677540427,0.607316711904609,6.65371376685591));
#20010=CARTESIAN_POINT('Ctrl Pts',(2.4465792908925,0.593394718934433,6.65279907558092));
#20011=CARTESIAN_POINT('Ctrl Pts',(2.44841242767532,0.58578502809641,6.65229765308281));
#20012=CARTESIAN_POINT('Ctrl Pts',(2.45214370450115,0.569972276258733,6.65125286516005));
#20013=CARTESIAN_POINT('Ctrl Pts',(2.45403623661321,0.561768001886577,6.65070920448268));
#20014=CARTESIAN_POINT('Ctrl Pts',(2.45885124073767,0.540405862953337,6.64928978862847));
#20015=CARTESIAN_POINT('Ctrl Pts',(2.46170922010563,0.527233931585121,6.64841079322574));
#20016=CARTESIAN_POINT('Ctrl Pts',(2.46993370875743,0.487803278738433,6.64576947173143));
#20017=CARTESIAN_POINT('Ctrl Pts',(2.47498664686636,0.46148189809904,6.6439930735918));
#20018=CARTESIAN_POINT('Ctrl Pts',(2.50469517508788,0.292168690199933,6.63250235207536));
#20019=CARTESIAN_POINT('Ctrl Pts',(2.51736734102002,0.147362881071231,6.6224012180816));
#20020=CARTESIAN_POINT('Ctrl Pts',(2.51749896391893,0.00228400243197625,
6.61240047030075));
#20021=CARTESIAN_POINT('Ctrl Pts',(2.51749896437308,0.00228350180114051,
6.61240043579068));
#20022=CARTESIAN_POINT('Ctrl Pts',(2.51764262912045,-0.156102995878949,
6.60148235182255));
#20023=CARTESIAN_POINT('Ctrl Pts',(2.50283907664945,-0.314178187571748,
6.59073840743485));
#20024=CARTESIAN_POINT('Ctrl Pts',(2.46917070021309,-0.491410592718018,
6.57903055701159));
#20025=CARTESIAN_POINT('Ctrl Pts',(2.4647909428422,-0.512926871148302,6.57761434418599));
#20026=CARTESIAN_POINT('Ctrl Pts',(2.4571129791369,-0.548273741161353,6.57529586558297));
#20027=CARTESIAN_POINT('Ctrl Pts',(2.45397817822452,-0.562138240850671,
6.57438851837946));
#20028=CARTESIAN_POINT('Ctrl Pts',(2.44763110369328,-0.589144486888082,
6.57262494229146));
#20029=CARTESIAN_POINT('Ctrl Pts',(2.44442999896002,-0.602288334602156,
6.57176839110694));
#20030=CARTESIAN_POINT('Ctrl Pts',(2.43857323921963,-0.625520269782588,
6.57025737715399));
#20031=CARTESIAN_POINT('Ctrl Pts',(2.43596055922672,-0.635618761611592,
6.56960155995007));
#20032=CARTESIAN_POINT('Ctrl Pts',(2.42979489923048,-0.65885368382676,6.56809478766277));
#20033=CARTESIAN_POINT('Ctrl Pts',(2.42619799965326,-0.671978204279829,
6.56724526228131));
#20034=CARTESIAN_POINT('Ctrl Pts',(2.41599242172552,-0.708066263611893,
6.56491332556017));
#20035=CARTESIAN_POINT('Ctrl Pts',(2.40916284800644,-0.730966242373608,
6.56343804479047));
#20036=CARTESIAN_POINT('Ctrl Pts',(2.36612829424863,-0.868103401182656,
6.55462425740325));
#20037=CARTESIAN_POINT('Ctrl Pts',(2.32212847682084,-0.979740342680465,
6.5475475943634));
#20038=CARTESIAN_POINT('Ctrl Pts',(2.2260048061575,-1.18035375868838,6.53463937488682));
#20039=CARTESIAN_POINT('Ctrl Pts',(2.17605756268362,-1.27008110973878,6.52878496287698));
#20040=CARTESIAN_POINT('Ctrl Pts',(2.0702389931808,-1.43551830349322,6.51745801455129));
#20041=CARTESIAN_POINT('Ctrl Pts',(2.01533173785899,-1.51163403156109,6.51200350096616));
#20042=CARTESIAN_POINT('Ctrl Pts',(1.93166392045488,-1.61493478907269,6.50398640288852));
#20043=CARTESIAN_POINT('Ctrl Pts',(1.90631064602362,-1.64478545996722,6.50159045911177));
#20044=CARTESIAN_POINT('Ctrl Pts',(1.87265745955274,-1.68258475532417,6.49843395943529));
#20045=CARTESIAN_POINT('Ctrl Pts',(1.86498363084858,-1.69108647461973,6.49771572571102));
#20046=CARTESIAN_POINT('Ctrl Pts',(1.85246658510197,-1.70476510224588,6.4965460787577));
#20047=CARTESIAN_POINT('Ctrl Pts',(1.84765894056843,-1.70997454341697,6.49609727528917));
#20048=CARTESIAN_POINT('Ctrl Pts',(1.83832436401742,-1.72000392664656,6.49522656451627));
#20049=CARTESIAN_POINT('Ctrl Pts',(1.83380035822558,-1.72482643106998,6.49480487203248));
#20050=CARTESIAN_POINT('Ctrl Pts',(1.82374968607531,-1.73545602069929,6.49386878388667));
#20051=CARTESIAN_POINT('Ctrl Pts',(1.81821417438852,-1.74125464224175,6.4933537272423));
#20052=CARTESIAN_POINT('Ctrl Pts',(1.79846577836947,-1.76174485810495,6.49151832115046));
#20053=CARTESIAN_POINT('Ctrl Pts',(1.78410219566875,-1.77628922011353,6.4901872096681));
#20054=CARTESIAN_POINT('Ctrl Pts',(1.64937474330208,-1.90942966451447,6.47775040913707));
#20055=CARTESIAN_POINT('Ctrl Pts',(1.51754305519328,-2.0157910269683,6.46596740877383));
#20056=CARTESIAN_POINT('Ctrl Pts',(1.27947782164855,-2.17118556082261,6.44636657095683));
#20057=CARTESIAN_POINT('Ctrl Pts',(1.17866325968881,-2.22752511464358,6.438492154302));
#20058=CARTESIAN_POINT('Ctrl Pts',(1.03531313466283,-2.29516760162362,6.42796476353293));
#20059=CARTESIAN_POINT('Ctrl Pts',(0.995826835890043,-2.31257364836771,
6.42512964081845));
#20060=CARTESIAN_POINT('Ctrl Pts',(0.926007551901459,-2.34123068113191,
6.42022828307746));
#20061=CARTESIAN_POINT('Ctrl Pts',(0.89586974705452,-2.3529276749184,6.41814798903026));
#20062=CARTESIAN_POINT('Ctrl Pts',(0.851281326778832,-2.36925221730586,
6.41512051641313));
#20063=CARTESIAN_POINT('Ctrl Pts',(0.83700179633168,-2.37433442796945,6.414158424086));
#20064=CARTESIAN_POINT('Ctrl Pts',(0.811629527554386,-2.38310729875188,
6.41246186480738));
#20065=CARTESIAN_POINT('Ctrl Pts',(0.800555456859901,-2.38685019540337,
6.41172570031532));
#20066=CARTESIAN_POINT('Ctrl Pts',(0.777261056146578,-2.39454305135542,
6.41018604902812));
#20067=CARTESIAN_POINT('Ctrl Pts',(0.765035734341543,-2.39847691444072,
6.40938310591206));
#20068=CARTESIAN_POINT('Ctrl Pts',(0.732720663011623,-2.40860303836279,
6.40727376137095));
#20069=CARTESIAN_POINT('Ctrl Pts',(0.712582265283442,-2.41463759662118,
6.40597249293455));
#20070=CARTESIAN_POINT('Ctrl Pts',(0.624223997608043,-2.43991281517091,
6.40031796042861));
#20071=CARTESIAN_POINT('Ctrl Pts',(0.555281092223001,-2.45652079187197,
6.39604924512552));
#20072=CARTESIAN_POINT('Ctrl Pts',(0.271994146491859,-2.51222454296997,
6.37894128547761));
#20073=CARTESIAN_POINT('Ctrl Pts',(0.0537343956660501,-2.52633247150004,
6.36683508631061));
#20074=CARTESIAN_POINT('Ctrl Pts',(-0.209791046977706,-2.50917040783561,
6.35125327565513));
#20075=CARTESIAN_POINT('Ctrl Pts',(-0.255882464528519,-2.50488963686466,
6.34848813789867));
#20076=CARTESIAN_POINT('Ctrl Pts',(-0.330648633776396,-2.49586068039505,
6.34390077324298));
#20077=CARTESIAN_POINT('Ctrl Pts',(-0.359406554799883,-2.49188198282343,
6.34211154031295));
#20078=CARTESIAN_POINT('Ctrl Pts',(-0.39817651573996,-2.48583305398359,
6.3396580874016));
#20079=CARTESIAN_POINT('Ctrl Pts',(-0.40825536533137,-2.48419766891451,
6.33901648352339));
#20080=CARTESIAN_POINT('Ctrl Pts',(-0.425047333157644,-2.48136807111227,
6.33794078620589));
#20081=CARTESIAN_POINT('Ctrl Pts',(-0.43176617225622,-2.48020779574439,
6.33750856988267));
#20082=CARTESIAN_POINT('Ctrl Pts',(-0.444473562776449,-2.47796015846696,
6.33668755472791));
#20083=CARTESIAN_POINT('Ctrl Pts',(-0.450463048201784,-2.47687834486623,
6.33629908076239));
#20084=CARTESIAN_POINT('Ctrl Pts',(-0.464631096237097,-2.47426623983085,
6.3353766983061));
#20085=CARTESIAN_POINT('Ctrl Pts',(-0.472806052021689,-2.47271711153767,
6.334841756449));
#20086=CARTESIAN_POINT('Ctrl Pts',(-0.501618220916195,-2.46710919515326,
6.33294711116231));
#20087=CARTESIAN_POINT('Ctrl Pts',(-0.522211451640957,-2.46283246529598,
6.3315761218241));
#20088=CARTESIAN_POINT('Ctrl Pts',(-0.690659741181082,-2.42564212631217,
6.32023669481753));
#20089=CARTESIAN_POINT('Ctrl Pts',(-0.835309564179003,-2.37970602818354,
6.30972613747561));
#20090=CARTESIAN_POINT('Ctrl Pts',(-1.04112724916594,-2.29325400895412,
6.2943107460072));
#20091=CARTESIAN_POINT('Ctrl Pts',(-1.10609724884355,-2.26263331728389,
6.28936833769292));
#20092=CARTESIAN_POINT('Ctrl Pts',(-1.238742405954,-2.19303616263861,6.27917404651769));
#20093=CARTESIAN_POINT('Ctrl Pts',(-1.30609616516309,-2.15360280351311,
6.27393809799044));
#20094=CARTESIAN_POINT('Ctrl Pts',(-1.39977026599398,-2.0927457440425,6.26658696488886));
#20095=CARTESIAN_POINT('Ctrl Pts',(-1.42765487181711,-2.07382335057029,
6.26438912432197));
#20096=CARTESIAN_POINT('Ctrl Pts',(-1.47690468943093,-2.03893829110284,
6.26048920128261));
#20097=CARTESIAN_POINT('Ctrl Pts',(-1.49841161713251,-2.02318549110424,
6.2587797136444));
#20098=CARTESIAN_POINT('Ctrl Pts',(-1.5308633246844,-1.99861477623512,6.2561894618137));
#20099=CARTESIAN_POINT('Ctrl Pts',(-1.54199068744078,-1.99004227982961,
6.25529929537964));
#20100=CARTESIAN_POINT('Ctrl Pts',(-1.56128157608125,-1.97492166610264,
6.25375234563691));
#20101=CARTESIAN_POINT('Ctrl Pts',(-1.5694770150833,-1.96841500997854,6.2530939570433));
#20102=CARTESIAN_POINT('Ctrl Pts',(-1.5878872597679,-1.9536103727868,6.25161211527055));
#20103=CARTESIAN_POINT('Ctrl Pts',(-1.59807809883172,-1.9452829714154,6.25078985732198));
#20104=CARTESIAN_POINT('Ctrl Pts',(-1.62549896937443,-1.92251520663694,
6.24857156387508));
#20105=CARTESIAN_POINT('Ctrl Pts',(-1.64260189478767,-1.90792313388635,
6.24718167660706));
#20106=CARTESIAN_POINT('Ctrl Pts',(-1.72578199286055,-1.83500689183502,
6.24038661615886));
#20107=CARTESIAN_POINT('Ctrl Pts',(-1.78896419196649,-1.77346646891228,
6.23511647398662));
#20108=CARTESIAN_POINT('Ctrl Pts',(-1.96922831725502,-1.57842657059376,
6.21951580690794));
#20109=CARTESIAN_POINT('Ctrl Pts',(-2.07554382487315,-1.43575955508333,
6.20954189931697));
#20110=CARTESIAN_POINT('Ctrl Pts',(-2.19629948248837,-1.23191507266479,
6.19570149942029));
#20111=CARTESIAN_POINT('Ctrl Pts',(-2.2247975460239,-1.17966992406611,6.19218250646721));
#20112=CARTESIAN_POINT('Ctrl Pts',(-2.26183683041802,-1.10564132577336,
6.1871684904197));
#20113=CARTESIAN_POINT('Ctrl Pts',(-2.27196736898275,-1.08467173988065,
6.18574516567033));
#20114=CARTESIAN_POINT('Ctrl Pts',(-2.28914374284474,-1.04782103196951,
6.18323347093917));
#20115=CARTESIAN_POINT('Ctrl Pts',(-2.29631892846367,-1.03200161361778,
6.18215193758628));
#20116=CARTESIAN_POINT('Ctrl Pts',(-2.30669339976604,-1.00848463871386,
6.18053745030711));
#20117=CARTESIAN_POINT('Ctrl Pts',(-2.31001925158052,-1.00084302449772,
6.18001180189886));
#20118=CARTESIAN_POINT('Ctrl Pts',(-2.31587817315683,-0.987196541443809,
6.17907100691467));
#20119=CARTESIAN_POINT('Ctrl Pts',(-2.31842594640675,-0.981198172534568,
6.17865675112962));
#20120=CARTESIAN_POINT('Ctrl Pts',(-2.32393861334242,-0.968078033439025,
6.17774902075387));
#20121=CARTESIAN_POINT('Ctrl Pts',(-2.32689403170536,-0.960952610090968,
6.17725501668204));
#20122=CARTESIAN_POINT('Ctrl Pts',(-2.33508972099295,-0.940933553534841,
6.17586446101935));
#20123=CARTESIAN_POINT('Ctrl Pts',(-2.34025579114612,-0.928010112279348,
6.17496372115736));
#20124=CARTESIAN_POINT('Ctrl Pts',(-2.37021276929685,-0.851228598166221,
6.16959693924877));
#20125=CARTESIAN_POINT('Ctrl Pts',(-2.39249394915815,-0.786428408410698,
6.16500603894688));
#20126=CARTESIAN_POINT('Ctrl Pts',(-2.47510092030687,-0.50999306334675,
6.14538475903113));
#20127=CARTESIAN_POINT('Ctrl Pts',(-2.51019960579048,-0.291785896529965,
6.12991464126099));
#20128=CARTESIAN_POINT('Ctrl Pts',(-2.51779611652691,-0.0255264967127382,
6.11217455402732));
#20129=CARTESIAN_POINT('Ctrl Pts',(-2.51783990854284,0.0207731010988608,
6.10912587337467));
#20130=CARTESIAN_POINT('Ctrl Pts',(-2.51569820002282,0.101158395823247,
6.103895795856));
#20131=CARTESIAN_POINT('Ctrl Pts',(-2.51409609117507,0.135246017962943,
6.10169762598872));
#20132=CARTESIAN_POINT('Ctrl Pts',(-2.51076017542635,0.184741330002574,
6.09853302560837));
#20133=CARTESIAN_POINT('Ctrl Pts',(-2.50957637538775,0.200181045749964,
6.09754968826761));
#20134=CARTESIAN_POINT('Ctrl Pts',(-2.50724518243701,0.227300559581401,
6.09582895586437));
#20135=CARTESIAN_POINT('Ctrl Pts',(-2.50615844354016,0.238984963220055,
6.09508969775372));
#20136=CARTESIAN_POINT('Ctrl Pts',(-2.50372654916484,0.263288141369486,
6.09355630303063));
#20137=CARTESIAN_POINT('Ctrl Pts',(-2.50236759773365,0.275905225729157,
6.09276261833018));
#20138=CARTESIAN_POINT('Ctrl Pts',(-2.49858436198463,0.308699546120931,
6.09070556367505));
#20139=CARTESIAN_POINT('Ctrl Pts',(-2.49601103316484,0.328858911285989,
6.08944686569461));
#20140=CARTESIAN_POINT('Ctrl Pts',(-2.48425174869456,0.412868665011913,
6.08422338922226));
#20141=CARTESIAN_POINT('Ctrl Pts',(-2.47285718629996,0.476388141691041,
6.08032764246175));
#20142=CARTESIAN_POINT('Ctrl Pts',(-2.41598692254536,0.735648212729541,
6.06454189794592));
#20143=CARTESIAN_POINT('Ctrl Pts',(-2.34960640922154,0.926023061614967,
6.05328600561617));
#20144=CARTESIAN_POINT('Ctrl Pts',(-2.23386081771046,1.16257094251553,6.03793050442848));
#20145=CARTESIAN_POINT('Ctrl Pts',(-2.20434065542979,1.21761512791022,6.03424483181116));
#20146=CARTESIAN_POINT('Ctrl Pts',(-2.15475215657273,1.3023545222563,6.02830425705274));
#20147=CARTESIAN_POINT('Ctrl Pts',(-2.13604310721858,1.33281795542462,6.02611180328649));
#20148=CARTESIAN_POINT('Ctrl Pts',(-2.11072452865471,1.37214057700311,6.02319243929303));
#20149=CARTESIAN_POINT('Ctrl Pts',(-2.10469538990937,1.38137073377817,6.02250059629575));
#20150=CARTESIAN_POINT('Ctrl Pts',(-2.09474246671518,1.39639148221189,6.02136339930581));
#20151=CARTESIAN_POINT('Ctrl Pts',(-2.09085475665357,1.4022059610428,6.02092039371176));
#20152=CARTESIAN_POINT('Ctrl Pts',(-2.08321336271889,1.41353203121619,6.02005181629774));
#20153=CARTESIAN_POINT('Ctrl Pts',(-2.07946193210531,1.41904502649759,6.01962639214683));
#20154=CARTESIAN_POINT('Ctrl Pts',(-2.0710282168807,1.43133371708985,6.01867229712303));
#20155=CARTESIAN_POINT('Ctrl Pts',(-2.06633449916899,1.43810146298348,6.01814287525579));
#20156=CARTESIAN_POINT('Ctrl Pts',(-2.04995275398882,1.46147608833569,6.01630086828549));
#20157=CARTESIAN_POINT('Ctrl Pts',(-2.03809740475567,1.47796399063211,6.01497784278345));
#20158=CARTESIAN_POINT('Ctrl Pts',(-1.92862734988289,1.62638819521802,6.00286387292814));
#20159=CARTESIAN_POINT('Ctrl Pts',(-1.81853600395081,1.74861676855274,5.99143463933209));
#20160=CARTESIAN_POINT('Ctrl Pts',(-1.60987589763608,1.93910631497473,5.97194476242831));
#20161=CARTESIAN_POINT('Ctrl Pts',(-1.51687216290424,2.01269417510598,5.96384920749629));
#20162=CARTESIAN_POINT('Ctrl Pts',(-1.38282625343039,2.10416686797863,5.9530645614086));
#20163=CARTESIAN_POINT('Ctrl Pts',(-1.34598830421661,2.12791976276554,5.95018339347335));
#20164=CARTESIAN_POINT('Ctrl Pts',(-1.28059835777471,2.1677048679725,5.94521088331135));
#20165=CARTESIAN_POINT('Ctrl Pts',(-1.25231975275721,2.18416390178316,5.94310491752272));
#20166=CARTESIAN_POINT('Ctrl Pts',(-1.21041859692883,2.20747026888751,5.94004750529565));
#20167=CARTESIAN_POINT('Ctrl Pts',(-1.19704283174079,2.2147520500952,5.93908072092514));
#20168=CARTESIAN_POINT('Ctrl Pts',(-1.17327642486921,2.22741229707972,5.93737885179961));
#20169=CARTESIAN_POINT('Ctrl Pts',(-1.16291292804173,2.23284048682187,5.93664203307494));
#20170=CARTESIAN_POINT('Ctrl Pts',(-1.14112599277617,2.24405920807533,5.93510391053287));
#20171=CARTESIAN_POINT('Ctrl Pts',(-1.12969542403539,2.2498352204772,5.934303129359));
#20172=CARTESIAN_POINT('Ctrl Pts',(-1.099533123351,2.26478878496928,5.93220598024121));
#20173=CARTESIAN_POINT('Ctrl Pts',(-1.08073029840269,2.27382131937554,5.93091463628026));
#20174=CARTESIAN_POINT('Ctrl Pts',(-0.998858166881356,2.31190616977218,
5.92535786513149));
#20175=CARTESIAN_POINT('Ctrl Pts',(-0.934711121816948,2.33857738123311,
5.92117334385899));
#20176=CARTESIAN_POINT('Ctrl Pts',(-0.705050342623193,2.42310374368821,
5.90666017056631));
#20177=CARTESIAN_POINT('Ctrl Pts',(-0.534693677424592,2.46629915494052,
5.89676193790825));
#20178=CARTESIAN_POINT('Ctrl Pts',(-0.251619936255753,2.50734128341228,
5.8801981352094));
#20179=CARTESIAN_POINT('Ctrl Pts',(-0.141094987856981,2.51598071206995,
5.8736904597384));
#20180=CARTESIAN_POINT('Ctrl Pts',(-0.0155015312881966,2.5174962230828,
5.86590237217017));
#20181=CARTESIAN_POINT('Ctrl Pts',(-0.000626224857081857,2.51754386530644,
5.8649736600194));
#20182=CARTESIAN_POINT('Ctrl Pts',(0.0220799689617035,2.51741535376739,
5.86354525662034));
#20183=CARTESIAN_POINT('Ctrl Pts',(0.0299113531311938,2.51733448223364,
5.86305064050257));
#20184=CARTESIAN_POINT('Ctrl Pts',(0.0442503720644473,2.51711948894187,
5.86214121999668));
#20185=CARTESIAN_POINT('Ctrl Pts',(0.0507579945147347,2.51699667068455,
5.86172704153836));
#20186=CARTESIAN_POINT('Ctrl Pts',(0.0654506991158243,2.5166623720372,5.8607886591277));
#20187=CARTESIAN_POINT('Ctrl Pts',(0.0736352119455181,2.51643619825982,
5.86026366945199));
#20188=CARTESIAN_POINT('Ctrl Pts',(0.0947900643359271,2.51574830563656,
5.85890109550621));
#20189=CARTESIAN_POINT('Ctrl Pts',(0.107758015593976,2.51522620989445,5.85806038132969));
#20190=CARTESIAN_POINT('Ctrl Pts',(0.194849099336523,2.51104514390699,5.85238016261128));
#20191=CARTESIAN_POINT('Ctrl Pts',(0.268776644480801,2.50421062328309,5.84739338082318));
#20192=CARTESIAN_POINT('Ctrl Pts',(0.402265388164401,2.48589099178223,5.83820729703165));
#20193=CARTESIAN_POINT('Ctrl Pts',(0.461926122795771,2.47549900149968,5.83403467532624));
#20194=CARTESIAN_POINT('Ctrl Pts',(0.62173698506213,2.4416837658413,5.82275368068259));
#20195=CARTESIAN_POINT('Ctrl Pts',(0.720928165416151,2.41425784866357,5.81564385606498));
#20196=CARTESIAN_POINT('Ctrl Pts',(0.926184677678503,2.34372220155681,5.80089070620759));
#20197=CARTESIAN_POINT('Ctrl Pts',(1.03156194926637,2.29929079358061,5.7932945120028));
#20198=CARTESIAN_POINT('Ctrl Pts',(1.15426592261674,2.23741226971139,5.78444470955402));
#20199=CARTESIAN_POINT('Ctrl Pts',(1.17481702349848,2.22669003337826,5.78296196079747));
#20200=CARTESIAN_POINT('Ctrl Pts',(1.20693309826492,2.20936550523106,5.78064329816586));
#20201=CARTESIAN_POINT('Ctrl Pts',(1.21859837794703,2.20295289185225,5.7798007859347));
#20202=CARTESIAN_POINT('Ctrl Pts',(1.24034085962375,2.19077510671482,5.77822965190946));
#20203=CARTESIAN_POINT('Ctrl Pts',(1.25043006066988,2.18503219355857,5.77750026638291));
#20204=CARTESIAN_POINT('Ctrl Pts',(1.27292575132958,2.1720204931856,5.77587304062748));
#20205=CARTESIAN_POINT('Ctrl Pts',(1.28531048293538,2.16471475424095,5.77497655249754));
#20206=CARTESIAN_POINT('Ctrl Pts',(1.31665850606506,2.14585871080158,5.77270527134266));
#20207=CARTESIAN_POINT('Ctrl Pts',(1.33553307244268,2.13416276062942,5.77133576283714));
#20208=CARTESIAN_POINT('Ctrl Pts',(1.49044716137565,2.03530745380056,5.76007220965784));
#20209=CARTESIAN_POINT('Ctrl Pts',(1.61796758928213,1.93548430355487,5.75068398696019));
#20210=CARTESIAN_POINT('Ctrl Pts',(1.82556859812181,1.73801924811472,5.73420126790117));
#20211=CARTESIAN_POINT('Ctrl Pts',(1.90954424125383,1.64531115857055,5.72708242144767));
#20212=CARTESIAN_POINT('Ctrl Pts',(2.01294746991208,1.51252489607689,5.71712629495188));
#20213=CARTESIAN_POINT('Ctrl Pts',(2.03871636746502,1.47760760512915,5.71452763058099));
#20214=CARTESIAN_POINT('Ctrl Pts',(2.07944486742211,1.41932501431833,5.71019036280101));
#20215=CARTESIAN_POINT('Ctrl Pts',(2.09494406099876,1.39634654999743,5.7084804154402));
#20216=CARTESIAN_POINT('Ctrl Pts',(2.11553174354946,1.36470961498031,5.70611941352598));
#20217=CARTESIAN_POINT('Ctrl Pts',(2.12095307622008,1.35626875348217,5.70548884757562));
#20218=CARTESIAN_POINT('Ctrl Pts',(2.12995417931019,1.3420683399604,5.7044265506527));
#20219=CARTESIAN_POINT('Ctrl Pts',(2.13356145796007,1.33632620958028,5.70399659693292));
#20220=CARTESIAN_POINT('Ctrl Pts',(2.14037890575465,1.32537610422837,5.7031757896568));
#20221=CARTESIAN_POINT('Ctrl Pts',(2.14359336835503,1.3201708779858,5.70278523464692));
#20222=CARTESIAN_POINT('Ctrl Pts',(2.15119994053834,1.30775241834254,5.70185266208054));
#20223=CARTESIAN_POINT('Ctrl Pts',(2.15557475603701,1.30052875329529,5.70130955784393));
#20224=CARTESIAN_POINT('Ctrl Pts',(2.1709795289709,1.27480123526098,5.69937337687495));
#20225=CARTESIAN_POINT('Ctrl Pts',(2.18180788290342,1.2561785677007,5.69796845186269));
#20226=CARTESIAN_POINT('Ctrl Pts',(2.25520805841346,1.12613200654281,5.688145840705));
#20227=CARTESIAN_POINT('Ctrl Pts',(2.30944999734189,1.01023324050885,5.6793424912854));
#20228=CARTESIAN_POINT('Ctrl Pts',(2.3569344417224,0.884707728550295,5.67007201361025));
#20229=CARTESIAN_POINT('Ctrl Pts',(2.35918987096009,0.878675634613511,5.6696271157682));
#20230=CARTESIAN_POINT('Ctrl Pts',(2.36142200559759,0.87263529694796,5.66918223051795));
#20231=CARTESIAN_POINT('Origin',(0.,0.,10.));
#20232=CARTESIAN_POINT('',(2.36142200727925,0.872635292397265,4.66658913197125));
#20233=CARTESIAN_POINT('',(2.36142200728636,0.872635292378022,4.94384492744144));
#20234=CARTESIAN_POINT('',(2.36142200728636,0.87263529237802,10.));
#20235=CARTESIAN_POINT('',(2.51749903524847,-0.00220397890970226,5.88741669756531));
#20236=CARTESIAN_POINT('Ctrl Pts',(2.36142200728636,0.872635292378022,4.94384492744144));
#20237=CARTESIAN_POINT('Ctrl Pts',(2.33267223382292,0.950434515437239,4.94908498406439));
#20238=CARTESIAN_POINT('Ctrl Pts',(2.30004677929906,1.02688413496855,4.95432504068734));
#20239=CARTESIAN_POINT('Ctrl Pts',(2.26369979786784,1.101575905298,4.95956509731029));
#20240=CARTESIAN_POINT('Ctrl Pts',(2.2273708295506,1.17623065931083,4.96480255702605));
#20241=CARTESIAN_POINT('Ctrl Pts',(2.1873241979168,1.2491288796774,4.97004001674182));
#20242=CARTESIAN_POINT('Ctrl Pts',(2.14376179350139,1.31988318525683,4.97527747645758));
#20243=CARTESIAN_POINT('Ctrl Pts',(2.10020783758702,1.39062376873271,4.98051392041941));
#20244=CARTESIAN_POINT('Ctrl Pts',(2.05313970549245,1.45922087074756,4.98575036438124));
#20245=CARTESIAN_POINT('Ctrl Pts',(2.00280406300176,1.52531378254562,4.99098680834306));
#20246=CARTESIAN_POINT('Ctrl Pts',(1.95246299932454,1.59141381259997,4.99622381627384));
#20247=CARTESIAN_POINT('Ctrl Pts',(1.89885400717399,1.65500875069382,5.00146082420462));
#20248=CARTESIAN_POINT('Ctrl Pts',(1.84226484542956,1.7157699406664,5.0066978321354));
#20249=CARTESIAN_POINT('Ctrl Pts',(1.78561580536273,1.77659542348254,5.01194038146738));
#20250=CARTESIAN_POINT('Ctrl Pts',(1.72598061546314,1.83458083389482,5.01718293079937));
#20251=CARTESIAN_POINT('Ctrl Pts',(1.66368442898251,1.88943387573134,5.02242548013135));
#20252=CARTESIAN_POINT('Ctrl Pts',(1.60135258097397,1.94431831825853,5.0276710305671));
#20253=CARTESIAN_POINT('Ctrl Pts',(1.53635706458887,1.99606653476143,5.03291658100284));
#20254=CARTESIAN_POINT('Ctrl Pts',(1.4690547859029,2.04442761818945,5.03816213143859));
#20255=CARTESIAN_POINT('Ctrl Pts',(1.40163917700721,2.09287013677589,5.04341651484912));
#20256=CARTESIAN_POINT('Ctrl Pts',(1.33190943726327,2.13791388323439,5.04867089825965));
#20257=CARTESIAN_POINT('Ctrl Pts',(1.2602496924962,2.17935241816536,5.05392528167019));
#20258=CARTESIAN_POINT('Ctrl Pts',(1.21655856142409,2.20461759971172,5.05712889277764));
#20259=CARTESIAN_POINT('Ctrl Pts',(1.17215044553941,2.22854349808343,5.06033250388509));
#20260=CARTESIAN_POINT('Ctrl Pts',(1.12711601958344,2.25109211903875,5.06353611499254));
#20261=CARTESIAN_POINT('Ctrl Pts',(1.05324090416664,2.28808119884167,5.06879136439984));
#20262=CARTESIAN_POINT('Ctrl Pts',(0.977406600329949,2.3214981450137,5.07404661380715));
#20263=CARTESIAN_POINT('Ctrl Pts',(0.899992693089727,2.35113151533152,5.07930186321445));
#20264=CARTESIAN_POINT('Ctrl Pts',(0.822688541183612,2.38072287226214,5.08454966187195));
#20265=CARTESIAN_POINT('Ctrl Pts',(0.743809661544648,2.40654114472748,5.08979746052945));
#20266=CARTESIAN_POINT('Ctrl Pts',(0.663759045355666,2.42842133488168,5.09504525918694));
#20267=CARTESIAN_POINT('Ctrl Pts',(0.583128393440619,2.4504600658765,5.10033108266985));
#20268=CARTESIAN_POINT('Ctrl Pts',(0.501309376583909,2.46850319198873,5.10561690615276));
#20269=CARTESIAN_POINT('Ctrl Pts',(0.418733125877458,2.48243203719516,5.11090272963567));
#20270=CARTESIAN_POINT('Ctrl Pts',(0.336897330711262,2.49623598340805,5.11614115550426));
#20271=CARTESIAN_POINT('Ctrl Pts',(0.254318290809087,2.50599905997798,5.12137958137285));
#20272=CARTESIAN_POINT('Ctrl Pts',(0.171427855908116,2.51165657290537,5.12661800724144));
#20273=CARTESIAN_POINT('Ctrl Pts',(0.088564682291696,2.51731222517091,5.13185471027894));
#20274=CARTESIAN_POINT('Ctrl Pts',(0.00539077706015141,2.51886496407217,
5.13709141331644));
#20275=CARTESIAN_POINT('Ctrl Pts',(-0.0776570934184586,2.51630197429518,
5.14232811635394));
#20276=CARTESIAN_POINT('Ctrl Pts',(-0.16070270171454,2.51373905433274,5.14756467674627));
#20277=CARTESIAN_POINT('Ctrl Pts',(-0.243621820914314,2.50706064386031,
5.15280123713859));
#20278=CARTESIAN_POINT('Ctrl Pts',(-0.325979284033456,2.49630602218178,
5.15803779753092));
#20279=CARTESIAN_POINT('Ctrl Pts',(-0.409684716824353,2.48537537633611,
5.1633600663014));
#20280=CARTESIAN_POINT('Ctrl Pts',(-0.492809452779872,2.47023393290528,
5.16868233507188));
#20281=CARTESIAN_POINT('Ctrl Pts',(-0.57490557300384,2.45097732183085,5.17400460384237));
#20282=CARTESIAN_POINT('Ctrl Pts',(-0.65579564118882,2.43200360445452,5.1792486845927));
#20283=CARTESIAN_POINT('Ctrl Pts',(-0.735686682421181,2.40903501479327,
5.18449276534303));
#20284=CARTESIAN_POINT('Ctrl Pts',(-0.814165640056451,2.38221337427013,
5.18973684609336));
#20285=CARTESIAN_POINT('Ctrl Pts',(-0.89439975210679,2.35479187714591,5.19509820887392));
#20286=CARTESIAN_POINT('Ctrl Pts',(-0.973157381352252,2.3233430951021,5.20045957165448));
#20287=CARTESIAN_POINT('Ctrl Pts',(-1.05002065499384,2.28806968296123,5.20582093443504));
#20288=CARTESIAN_POINT('Ctrl Pts',(-1.12688392863543,2.25279627082036,5.2111822972156));
#20289=CARTESIAN_POINT('Ctrl Pts',(-1.20185242704163,2.21369852276584,5.21654365999616));
#20290=CARTESIAN_POINT('Ctrl Pts',(-1.27453862635216,2.17102683998525,5.22190502277672));
#20291=CARTESIAN_POINT('Ctrl Pts',(-1.34578620303772,2.12919972534656,5.22716027218404));
#20292=CARTESIAN_POINT('Ctrl Pts',(-1.41510418478558,2.08378440484446,5.23241552159136));
#20293=CARTESIAN_POINT('Ctrl Pts',(-1.48210854983538,2.03498415141368,5.23767077099868));
#20294=CARTESIAN_POINT('Ctrl Pts',(-1.5490179179171,1.98625308565619,5.24291856965619));
#20295=CARTESIAN_POINT('Ctrl Pts',(-1.61361981483033,1.93414688869806,5.2481663683137));
#20296=CARTESIAN_POINT('Ctrl Pts',(-1.67555643247632,1.87891375309971,5.25341416697121));
#20297=CARTESIAN_POINT('Ctrl Pts',(-1.73794183431264,1.82328040581752,5.25869999045411));
#20298=CARTESIAN_POINT('Ctrl Pts',(-1.79762276074638,1.76447485387468,5.26398581393702));
#20299=CARTESIAN_POINT('Ctrl Pts',(-1.8542649372488,1.70279411335889,5.26927163741992));
#20300=CARTESIAN_POINT('Ctrl Pts',(-1.91039920726448,1.64166645978555,5.27451006328853));
#20301=CARTESIAN_POINT('Ctrl Pts',(-1.96354868775492,1.57771532047659,5.27974848915713));
#20302=CARTESIAN_POINT('Ctrl Pts',(-2.01342399262884,1.51126770491086,5.28498691502574));
#20303=CARTESIAN_POINT('Ctrl Pts',(-2.06328289434503,1.44484194286004,5.29022361806326));
#20304=CARTESIAN_POINT('Ctrl Pts',(-2.10986948229739,1.3759217039417,5.29546032110078));
#20305=CARTESIAN_POINT('Ctrl Pts',(-2.1529352089685,1.30486636709808,5.3006970241383));
#20306=CARTESIAN_POINT('Ctrl Pts',(-2.19599976255075,1.23381296576632,5.30593358453064));
#20307=CARTESIAN_POINT('Ctrl Pts',(-2.23554340725751,1.16062497728009,5.31117014492299));
#20308=CARTESIAN_POINT('Ctrl Pts',(-2.27136216292191,1.08568880202693,5.31640670531534));
#20309=CARTESIAN_POINT('Ctrl Pts',(-2.30776717506465,1.00952612358046,5.3217289740858));
#20310=CARTESIAN_POINT('Ctrl Pts',(-2.34032404138,0.931557953841109,5.32705124285626));
#20311=CARTESIAN_POINT('Ctrl Pts',(-2.36886910538294,0.852212069594317,
5.33237351162672));
#20312=CARTESIAN_POINT('Ctrl Pts',(-2.39699482152228,0.774031834408297,
5.33761759237707));
#20313=CARTESIAN_POINT('Ctrl Pts',(-2.42122574782482,0.694514560871142,
5.34286167312742));
#20314=CARTESIAN_POINT('Ctrl Pts',(-2.44145595367123,0.614083932604748,
5.34810575387777));
#20315=CARTESIAN_POINT('Ctrl Pts',(-2.46213860098934,0.531854501493749,
5.35346711665829));
#20316=CARTESIAN_POINT('Ctrl Pts',(-2.47863931941877,0.44867087120749,5.35882847943881));
#20317=CARTESIAN_POINT('Ctrl Pts',(-2.49090058276349,0.364993885960422,
5.36418984221933));
#20318=CARTESIAN_POINT('Ctrl Pts',(-2.50316184610821,0.28131690071336,5.36955120499985));
#20319=CARTESIAN_POINT('Ctrl Pts',(-2.51118367265795,0.197147072657779,
5.37491256778037));
#20320=CARTESIAN_POINT('Ctrl Pts',(-2.51496510902639,0.112945785135466,
5.38027393056089));
#20321=CARTESIAN_POINT('Ctrl Pts',(-2.51867170230267,0.0304110296152409,
5.38552917996819));
#20322=CARTESIAN_POINT('Ctrl Pts',(-2.51831796520711,-0.0524588008414003,
5.39078442937549));
#20323=CARTESIAN_POINT('Ctrl Pts',(-2.51386532026224,-0.135230919477881,
5.39603967878279));
#20324=CARTESIAN_POINT('Ctrl Pts',(-2.50941898815638,-0.217885686053684,
5.40128747744027));
#20325=CARTESIAN_POINT('Ctrl Pts',(-2.50088531575826,-0.300442559065994,
5.40653527609776));
#20326=CARTESIAN_POINT('Ctrl Pts',(-2.48827767589485,-0.38246628301505,
5.41178307475525));
#20327=CARTESIAN_POINT('Ctrl Pts',(-2.47557868281153,-0.46508433955709,
5.41706889823816));
#20328=CARTESIAN_POINT('Ctrl Pts',(-2.45874641307709,-0.547161014775412,
5.42235472172107));
#20329=CARTESIAN_POINT('Ctrl Pts',(-2.4378480052055,-0.628254210901584,
5.42764054520398));
#20330=CARTESIAN_POINT('Ctrl Pts',(-2.4171369919148,-0.708620249935456,
5.43287897107256));
#20331=CARTESIAN_POINT('Ctrl Pts',(-2.39243258725539,-0.788019921759011,
5.43811739694115));
#20332=CARTESIAN_POINT('Ctrl Pts',(-2.36385152754614,-0.866032450730203,
5.44335582280973));
#20333=CARTESIAN_POINT('Ctrl Pts',(-2.33527986767179,-0.944019322678919,
5.44859252584723));
#20334=CARTESIAN_POINT('Ctrl Pts',(-2.30283424350849,-1.02061952491235,
5.45382922888473));
#20335=CARTESIAN_POINT('Ctrl Pts',(-2.26668077725661,-1.09542891326429,
5.45906593192222));
#20336=CARTESIAN_POINT('Ctrl Pts',(-2.23052829580707,-1.17023626384591,
5.46430249231455));
#20337=CARTESIAN_POINT('Ctrl Pts',(-2.19066837478679,-1.24325248253438,
5.46953905270688));
#20338=CARTESIAN_POINT('Ctrl Pts',(-2.14731406653957,-1.31409609604523,
5.4747756130992));
#20339=CARTESIAN_POINT('Ctrl Pts',(-2.10325016513045,-1.38609922854609,
5.48009788186969));
#20340=CARTESIAN_POINT('Ctrl Pts',(-2.05557670255103,-1.45585756856753,
5.48542015064018));
#20341=CARTESIAN_POINT('Ctrl Pts',(-2.00456339163998,-1.52300093857385,
5.49074241941067));
#20342=CARTESIAN_POINT('Ctrl Pts',(-1.95429950356983,-1.58915792337601,
5.495986500161));
#20343=CARTESIAN_POINT('Ctrl Pts',(-1.90079359363922,-1.65277594112813,
5.50123058091132));
#20344=CARTESIAN_POINT('Ctrl Pts',(-1.84434337031048,-1.7135354628346,5.50647466166165));
#20345=CARTESIAN_POINT('Ctrl Pts',(-1.78663065749791,-1.77565384997461,
5.51183602444222));
#20346=CARTESIAN_POINT('Ctrl Pts',(-1.72584071206694,-1.83478398265607,
5.51719738722279));
#20347=CARTESIAN_POINT('Ctrl Pts',(-1.66232876636211,-1.89062670099759,
5.52255875000336));
#20348=CARTESIAN_POINT('Ctrl Pts',(-1.59881682065729,-1.9464694193391,5.52792011278393));
#20349=CARTESIAN_POINT('Ctrl Pts',(-1.53258331422587,-1.99902445983985,
5.5332814755645));
#20350=CARTESIAN_POINT('Ctrl Pts',(-1.46401473278279,-2.04803982192606,
5.53864283834507));
#20351=CARTESIAN_POINT('Ctrl Pts',(-1.39680327708826,-2.09608506025352,
5.54389808775238));
#20352=CARTESIAN_POINT('Ctrl Pts',(-1.32710010991282,-2.14090695686197,
5.54915333715968));
#20353=CARTESIAN_POINT('Ctrl Pts',(-1.25524724588119,-2.18223752183571,
5.55440858656699));
#20354=CARTESIAN_POINT('Ctrl Pts',(-1.18349625288774,-2.22350948945751,
5.55965638522449));
#20355=CARTESIAN_POINT('Ctrl Pts',(-1.10960201345748,-2.26129972927176,
5.56490418388198));
#20356=CARTESIAN_POINT('Ctrl Pts',(-1.03393689740224,-2.29538248276627,
5.57015198253948));
#20357=CARTESIAN_POINT('Ctrl Pts',(-0.957723522350152,-2.32971219519264,
5.57543780602239));
#20358=CARTESIAN_POINT('Ctrl Pts',(-0.879713884850836,-2.36028019114472,
5.58072362950529));
#20359=CARTESIAN_POINT('Ctrl Pts',(-0.800315366770485,-2.3869020850699,
5.5860094529882));
#20360=CARTESIAN_POINT('Ctrl Pts',(-0.721628809721245,-2.41328526230983,
5.59124787885679));
#20361=CARTESIAN_POINT('Ctrl Pts',(-0.641578625868135,-2.43579267354177,
5.59648630472538));
#20362=CARTESIAN_POINT('Ctrl Pts',(-0.560581315844548,-2.45429314433423,
5.60172473059397));
#20363=CARTESIAN_POINT('Ctrl Pts',(-0.479610644488222,-2.47278753062974,
5.60696143363148));
#20364=CARTESIAN_POINT('Ctrl Pts',(-0.397693915086651,-2.48727749107547,
5.61219813666898));
#20365=CARTESIAN_POINT('Ctrl Pts',(-0.315260566139868,-2.4976823307693,
5.61743483970649));
#20366=CARTESIAN_POINT('Ctrl Pts',(-0.232829462636283,-2.5080868870405,
5.62267140009882));
#20367=CARTESIAN_POINT('Ctrl Pts',(-0.149882225484674,-2.51440648704672,
5.62790796049115));
#20368=CARTESIAN_POINT('Ctrl Pts',(-0.0668548282142248,-2.51661214372506,
5.63314452088349));
#20369=CARTESIAN_POINT('Ctrl Pts',(0.0175315037440013,-2.51885390105774,
5.63846678965397));
#20370=CARTESIAN_POINT('Ctrl Pts',(0.102000152302478,-2.51684580555825,
5.64378905842444));
#20371=CARTESIAN_POINT('Ctrl Pts',(0.186093769824085,-2.51061254653773,
5.64911132719492));
#20372=CARTESIAN_POINT('Ctrl Pts',(0.268951990610853,-2.50447085865029,
5.65435540794526));
#20373=CARTESIAN_POINT('Ctrl Pts',(0.351445669286562,-2.49422744326407,
5.65959948869559));
#20374=CARTESIAN_POINT('Ctrl Pts',(0.433144699557753,-2.47995804788005,
5.66484356944592));
#20375=CARTESIAN_POINT('Ctrl Pts',(0.51667090004111,-2.46536952246346,5.67020493222648));
#20376=CARTESIAN_POINT('Ctrl Pts',(0.599365979841238,-2.44657287826214,
5.67556629500703));
#20377=CARTESIAN_POINT('Ctrl Pts',(0.680785599153083,-2.4237032033617,5.68092765778758));
#20378=CARTESIAN_POINT('Ctrl Pts',(0.762205218464927,-2.40083352846127,
5.68628902056813));
#20379=CARTESIAN_POINT('Ctrl Pts',(0.842348916953833,-2.37389104808713,
5.69165038334869));
#20380=CARTESIAN_POINT('Ctrl Pts',(0.920794895731843,-2.34306274136955,
5.69701174612924));
#20381=CARTESIAN_POINT('Ctrl Pts',(0.997688252953283,-2.31284459586492,
5.70226699553655));
#20382=CARTESIAN_POINT('Ctrl Pts',(1.07323451221374,-2.27878146856251,5.70752224494385));
#20383=CARTESIAN_POINT('Ctrl Pts',(1.14702267524311,-2.24101433116304,5.71277749435116));
#20384=CARTESIAN_POINT('Ctrl Pts',(1.22070622341987,-2.20330073898478,5.71802529300865));
#20385=CARTESIAN_POINT('Ctrl Pts',(1.29263621904077,-2.16189377609017,5.72327309166614));
#20386=CARTESIAN_POINT('Ctrl Pts',(1.36242056028213,-2.1169828688302,5.72852089032363));
#20387=CARTESIAN_POINT('Ctrl Pts',(1.43271054923708,-2.0717465433293,5.73380671380654));
#20388=CARTESIAN_POINT('Ctrl Pts',(1.50082321732777,-2.02295545433889,5.73909253728945));
#20389=CARTESIAN_POINT('Ctrl Pts',(1.56638210368218,-1.9708509216235,5.74437836077236));
#20390=CARTESIAN_POINT('Ctrl Pts',(1.63135312802791,-1.91921360665641,5.74961678664095));
#20391=CARTESIAN_POINT('Ctrl Pts',(1.69381561848899,-1.86432232519309,5.75485521250955));
#20392=CARTESIAN_POINT('Ctrl Pts',(1.75343278254427,-1.80645501662761,5.76009363837814));
#20393=CARTESIAN_POINT('Ctrl Pts',(1.81303033950647,-1.74860673965686,5.76533034141565));
#20394=CARTESIAN_POINT('Ctrl Pts',(1.86978409773885,-1.68778470059144,5.77056704445316));
#20395=CARTESIAN_POINT('Ctrl Pts',(1.92339256251835,-1.62430517466673,5.77580374749066));
#20396=CARTESIAN_POINT('Ctrl Pts',(1.97699956703006,-1.56082737789256,5.781040307883));
#20397=CARTESIAN_POINT('Ctrl Pts',(2.02746115151177,-1.49469259138107,5.78627686827533));
#20398=CARTESIAN_POINT('Ctrl Pts',(2.07451563537021,-1.42625072431342,5.79151342866767));
#20399=CARTESIAN_POINT('Ctrl Pts',(2.12234027429109,-1.35668864837122,5.79683569743815));
#20400=CARTESIAN_POINT('Ctrl Pts',(2.1666449868447,-1.28474368689114,5.80215796620862));
#20401=CARTESIAN_POINT('Ctrl Pts',(2.20720147859976,-1.21081290167681,5.8074802349791));
#20402=CARTESIAN_POINT('Ctrl Pts',(2.24716216583405,-1.1379682137591,5.81272431572944));
#20403=CARTESIAN_POINT('Ctrl Pts',(2.28348388016501,-1.0631961090121,5.81796839647978));
#20404=CARTESIAN_POINT('Ctrl Pts',(2.31599598596918,-0.986898598121723,
5.82321247723012));
#20405=CARTESIAN_POINT('Ctrl Pts',(2.34923521363833,-0.908894720109367,
5.82857384001067));
#20406=CARTESIAN_POINT('Ctrl Pts',(2.37849219878231,-0.829296862872776,
5.83393520279122));
#20407=CARTESIAN_POINT('Ctrl Pts',(2.40363833074468,-0.748551284131521,
5.83929656557177));
#20408=CARTESIAN_POINT('Ctrl Pts',(2.42878446270704,-0.667805705390267,
5.84465792835232));
#20409=CARTESIAN_POINT('Ctrl Pts',(2.44981967977522,-0.585912913893838,
5.85001929113287));
#20410=CARTESIAN_POINT('Ctrl Pts',(2.46667116953814,-0.503328512374697,
5.85538065391342));
#20411=CARTESIAN_POINT('Ctrl Pts',(2.49012320424341,-0.388396700541604,
5.8628420040828));
#20412=CARTESIAN_POINT('Ctrl Pts',(2.50554871649177,-0.271776010994806,
5.87030335425218));
#20413=CARTESIAN_POINT('Ctrl Pts',(2.51276111767348,-0.154394998326727,
5.87776470442156));
#20414=CARTESIAN_POINT('Ctrl Pts',(2.51587110200439,-0.103780355443389,
5.88098203545038));
#20415=CARTESIAN_POINT('Ctrl Pts',(2.51745454359309,-0.0530246346749052,
5.8841993664792));
#20416=CARTESIAN_POINT('Ctrl Pts',(2.51749903524768,-0.00220397981474928,
5.88741669750801));
#20417=CARTESIAN_POINT('Ctrl Pts',(2.51749903524847,-0.00220397890970059,
5.88741669756531));
#20418=CARTESIAN_POINT('Ctrl Pts',(2.51757053067679,0.0794618079230993,
5.89258675825598));
#20419=CARTESIAN_POINT('Ctrl Pts',(2.51366404213075,0.161254080397915,5.89775681894665));
#20420=CARTESIAN_POINT('Ctrl Pts',(2.5057692990165,0.242747749951151,5.90292687963733));
#20421=CARTESIAN_POINT('Ctrl Pts',(2.49788117536977,0.324173089896855,5.90809260541193));
#20422=CARTESIAN_POINT('Ctrl Pts',(2.48601147702744,0.405299852219512,5.91325833118653));
#20423=CARTESIAN_POINT('Ctrl Pts',(2.47020197026165,0.485704103457491,5.91842405696113));
#20424=CARTESIAN_POINT('Ctrl Pts',(2.45439918947274,0.566074147610928,5.92358758503579));
#20425=CARTESIAN_POINT('Ctrl Pts',(2.43466001342619,0.645721823650851,5.92875111311045));
#20426=CARTESIAN_POINT('Ctrl Pts',(2.41107772695427,0.724230933187066,5.93391464118511));
#20427=CARTESIAN_POINT('Ctrl Pts',(2.39606974731984,0.774194838020478,5.93720075698557));
#20428=CARTESIAN_POINT('Ctrl Pts',(2.37950628321881,0.823697772264239,5.94048687278603));
#20429=CARTESIAN_POINT('Ctrl Pts',(2.36142200728636,0.872635292378018,5.94377298858649));
#20430=CARTESIAN_POINT('Ctrl Pts',(2.36142200559759,0.872635296947961,5.66918223051795));
#20431=CARTESIAN_POINT('Ctrl Pts',(2.39783104698668,0.774109473113404,5.66192556901657));
#20432=CARTESIAN_POINT('Ctrl Pts',(2.42804248043668,0.673389919223703,5.65467850049511));
#20433=CARTESIAN_POINT('Ctrl Pts',(2.47501374093648,0.47171881947199,5.64067010978861));
#20434=CARTESIAN_POINT('Ctrl Pts',(2.49209560292995,0.371046896598681,5.63391380302999));
#20435=CARTESIAN_POINT('Ctrl Pts',(2.5054373914724,0.247180826666557,5.62589615657237));
#20436=CARTESIAN_POINT('Ctrl Pts',(2.50755126384116,0.224725603632017,5.62445411121646));
#20437=CARTESIAN_POINT('Ctrl Pts',(2.51042164432387,0.189111133098329,5.62218448477917));
#20438=CARTESIAN_POINT('Ctrl Pts',(2.51137702772495,0.175969566382344,5.62135076358077));
#20439=CARTESIAN_POINT('Ctrl Pts',(2.51298104593006,0.151220523591832,5.6197875217877));
#20440=CARTESIAN_POINT('Ctrl Pts',(2.51365253433375,0.139614927153138,5.61905731044915));
#20441=CARTESIAN_POINT('Ctrl Pts',(2.51498468159558,0.113449196171349,5.6174172010502));
#20442=CARTESIAN_POINT('Ctrl Pts',(2.51559933861532,0.0988870589969022,
5.61650875328282));
#20443=CARTESIAN_POINT('Ctrl Pts',(2.51703647558089,0.0560033358103809,
5.6138456553633));
#20444=CARTESIAN_POINT('Ctrl Pts',(2.51750737237581,0.0276716838714607,
5.61210188970108));
#20445=CARTESIAN_POINT('Ctrl Pts',(2.51747265449706,-0.104199967389831,
5.60405005134338));
#20446=CARTESIAN_POINT('Ctrl Pts',(2.51105833246633,-0.207643202004953,
5.59792487363476));
#20447=CARTESIAN_POINT('Ctrl Pts',(2.47687590215931,-0.482758338292225,
5.58179499959653));
#20448=CARTESIAN_POINT('Ctrl Pts',(2.43768600780875,-0.652418633881754,
5.5720364616246));
#20449=CARTESIAN_POINT('Ctrl Pts',(2.3599098385048,-0.879204334357425,5.55787415453548));
#20450=CARTESIAN_POINT('Ctrl Pts',(2.33601678259988,-0.940849987195239,
5.55389904250376));
#20451=CARTESIAN_POINT('Ctrl Pts',(2.30424270751658,-1.01413114795309,5.5489391888713));
#20452=CARTESIAN_POINT('Ctrl Pts',(2.29865284163117,-1.02673829875189,5.54807730597257));
#20453=CARTESIAN_POINT('Ctrl Pts',(2.28978699462535,-1.04629863674219,5.5467256699616));
#20454=CARTESIAN_POINT('Ctrl Pts',(2.2865821744531,-1.0532840422973,5.54624008944124));
#20455=CARTESIAN_POINT('Ctrl Pts',(2.28059952182967,-1.06616817726162,5.54533892952165));
#20456=CARTESIAN_POINT('Ctrl Pts',(2.27783071097401,-1.0720708978997,5.54492389581341));
#20457=CARTESIAN_POINT('Ctrl Pts',(2.27145410797361,-1.08552870991306,5.54397268782207));
#20458=CARTESIAN_POINT('Ctrl Pts',(2.26783155110192,-1.09307657358126,5.54343563055764));
#20459=CARTESIAN_POINT('Ctrl Pts',(2.25649076860869,-1.11640687884374,5.54176483477058));
#20460=CARTESIAN_POINT('Ctrl Pts',(2.24864512176733,-1.13212631077346,5.5406237595016));
#20461=CARTESIAN_POINT('Ctrl Pts',(2.22986181527336,-1.16879467666197,5.53792807393001));
#20462=CARTESIAN_POINT('Ctrl Pts',(2.21879255196787,-1.18967400472535,5.5363668114175));
#20463=CARTESIAN_POINT('Ctrl Pts',(2.17818180303355,-1.26373705706365,5.53074189303134));
#20464=CARTESIAN_POINT('Ctrl Pts',(2.14700993797586,-1.31599950790599,5.52661087654587));
#20465=CARTESIAN_POINT('Ctrl Pts',(2.01346722173593,-1.52250297695557,5.50975858512767));
#20466=CARTESIAN_POINT('Ctrl Pts',(1.89610733146566,-1.66639001829872,5.49682899394259));
#20467=CARTESIAN_POINT('Ctrl Pts',(1.70718628308946,-1.85193647878988,5.47908743713262));
#20468=CARTESIAN_POINT('Ctrl Pts',(1.64772250568898,-1.90503714795624,5.47384760369904));
#20469=CARTESIAN_POINT('Ctrl Pts',(1.56886942098742,-1.96899266999412,5.4673185314169));
#20470=CARTESIAN_POINT('Ctrl Pts',(1.55172562925484,-1.98253146639487,5.46592262179008));
#20471=CARTESIAN_POINT('Ctrl Pts',(1.52408399891509,-2.00378236723756,5.46370865119447));
#20472=CARTESIAN_POINT('Ctrl Pts',(1.51369907746407,-2.01163886526274,5.46288495309209));
#20473=CARTESIAN_POINT('Ctrl Pts',(1.49390886409483,-2.02637071292773,5.46133029742939));
#20474=CARTESIAN_POINT('Ctrl Pts',(1.48451592885888,-2.03326201575861,5.46059873439598));
#20475=CARTESIAN_POINT('Ctrl Pts',(1.46306251189895,-2.0487738012655,5.45894193223829));
#20476=CARTESIAN_POINT('Ctrl Pts',(1.45097297380197,-2.05735350550188,5.45801826834275));
#20477=CARTESIAN_POINT('Ctrl Pts',(1.41372720728206,-2.08329446596012,5.45520237251203));
#20478=CARTESIAN_POINT('Ctrl Pts',(1.38832944068451,-2.10030520075686,5.4533233096956));
#20479=CARTESIAN_POINT('Ctrl Pts',(1.26371508216894,-2.18052011764391,5.44428962807916));
#20480=CARTESIAN_POINT('Ctrl Pts',(1.16045619625476,-2.2371834521684,5.43737439906529));
#20481=CARTESIAN_POINT('Ctrl Pts',(0.887978982514378,-2.36274325372937,
5.42000525339764));
#20482=CARTESIAN_POINT('Ctrl Pts',(0.714570661034453,-2.42083425413133,
5.40976769672338));
#20483=CARTESIAN_POINT('Ctrl Pts',(0.493989579096829,-2.46894054252338,
5.39620999699039));
#20484=CARTESIAN_POINT('Ctrl Pts',(0.451319574014799,-2.4770957263316,5.39356156159059));
#20485=CARTESIAN_POINT('Ctrl Pts',(0.396365628675956,-2.48613170227601,
5.39009325859955));
#20486=CARTESIAN_POINT('Ctrl Pts',(0.384254192605346,-2.4880324061188,5.38932531531737));
#20487=CARTESIAN_POINT('Ctrl Pts',(0.36494204170022,-2.49091878066398,5.38809445220397));
#20488=CARTESIAN_POINT('Ctrl Pts',(0.357749927974798,-2.49196188805645,
5.38763466257352));
#20489=CARTESIAN_POINT('Ctrl Pts',(0.344008604780543,-2.49389414622446,
5.38675334150088));
#20490=CARTESIAN_POINT('Ctrl Pts',(0.337460301974299,-2.49478866304452,
5.38633210946532));
#20491=CARTESIAN_POINT('Ctrl Pts',(0.321886276455238,-2.49685368205619,
5.38532740676311));
#20492=CARTESIAN_POINT('Ctrl Pts',(0.312857636908472,-2.49800103632878,
5.38474267322363));
#20493=CARTESIAN_POINT('Ctrl Pts',(0.282358510436422,-2.50170890824558,
5.38276016628613));
#20494=CARTESIAN_POINT('Ctrl Pts',(0.260861986125186,-2.50404168101888,
5.38135073287078));
#20495=CARTESIAN_POINT('Ctrl Pts',(0.133269989665312,-2.51622705632052,
5.37292373061923));
#20496=CARTESIAN_POINT('Ctrl Pts',(0.0266748502186243,-2.51961177295505,
5.36563681993708));
#20497=CARTESIAN_POINT('Ctrl Pts',(-0.270519628149642,-2.51018626220693,
5.34513737730983));
#20498=CARTESIAN_POINT('Ctrl Pts',(-0.459963597470203,-2.48247262574406,
5.3319125261101));
#20499=CARTESIAN_POINT('Ctrl Pts',(-0.694773483722971,-2.42029002422557,
5.31589706063384));
#20500=CARTESIAN_POINT('Ctrl Pts',(-0.744653177009354,-2.40541187577891,
5.31251266403639));
#20501=CARTESIAN_POINT('Ctrl Pts',(-0.811868078652032,-2.38307143522336,
5.30797368071818));
#20502=CARTESIAN_POINT('Ctrl Pts',(-0.829630643553055,-2.37694599623925,
5.30677623025569));
#20503=CARTESIAN_POINT('Ctrl Pts',(-0.857798471472089,-2.36687806575736,
5.30488018697502));
#20504=CARTESIAN_POINT('Ctrl Pts',(-0.868248772877727,-2.36306455067636,
5.30417738532549));
#20505=CARTESIAN_POINT('Ctrl Pts',(-0.889675628291844,-2.35508415185207,
5.30273755970141));
#20506=CARTESIAN_POINT('Ctrl Pts',(-0.900649012105707,-2.35090949429513,
5.30200081375032));
#20507=CARTESIAN_POINT('Ctrl Pts',(-0.926063452541657,-2.34103689127228,
5.30029577581887));
#20508=CARTESIAN_POINT('Ctrl Pts',(-0.940481906354718,-2.33528179139785,
5.29932941236738));
#20509=CARTESIAN_POINT('Ctrl Pts',(-0.986621950089961,-2.3163684322425,
5.29623930884737));
#20510=CARTESIAN_POINT('Ctrl Pts',(-1.01812868814839,-2.30269401661894,
5.29413284744242));
#20511=CARTESIAN_POINT('Ctrl Pts',(-1.09177945566315,-2.26892110560911,
5.28920965306988));
#20512=CARTESIAN_POINT('Ctrl Pts',(-1.13366417879987,-2.24828629554803,
5.28641069389122));
#20513=CARTESIAN_POINT('Ctrl Pts',(-1.37379983546856,-2.12156348579047,
5.27030554327346));
#20514=CARTESIAN_POINT('Ctrl Pts',(-1.55767334296076,-1.99047711769316,
5.25783974244052));
#20515=CARTESIAN_POINT('Ctrl Pts',(-1.76803016161815,-1.79329575922209,
5.24078055354328));
#20516=CARTESIAN_POINT('Ctrl Pts',(-1.81270494747751,-1.74812461430787,
5.23695498945698));
#20517=CARTESIAN_POINT('Ctrl Pts',(-1.86484320538594,-1.69125761796496,
5.23216304485169));
#20518=CARTESIAN_POINT('Ctrl Pts',(-1.87398410878147,-1.68112344927229,
5.23130995820897));
#20519=CARTESIAN_POINT('Ctrl Pts',(-1.88812155839485,-1.66519122125636,
5.22996921899234));
#20520=CARTESIAN_POINT('Ctrl Pts',(-1.89317498215566,-1.65944367361167,
5.22948563235671));
#20521=CARTESIAN_POINT('Ctrl Pts',(-1.90248721580531,-1.64875443934342,
5.22858622295046));
#20522=CARTESIAN_POINT('Ctrl Pts',(-1.90675310206618,-1.64381915429765,
5.2281709278583));
#20523=CARTESIAN_POINT('Ctrl Pts',(-1.91647903501075,-1.63247823930534,
5.22721656550286));
#20524=CARTESIAN_POINT('Ctrl Pts',(-1.92192615375607,-1.62606179098011,
5.22667659187876));
#20525=CARTESIAN_POINT('Ctrl Pts',(-1.93879348003045,-1.60598972300047,
5.22498771447247));
#20526=CARTESIAN_POINT('Ctrl Pts',(-1.95010080566896,-1.59224054526798,
5.22383125059638));
#20527=CARTESIAN_POINT('Ctrl Pts',(-1.97633192303534,-1.55964618097085,
5.22109292579974));
#20528=CARTESIAN_POINT('Ctrl Pts',(-1.99113329443608,-1.54070509648409,
5.21950413730703));
#20529=CARTESIAN_POINT('Ctrl Pts',(-2.04339858759305,-1.47181084790265,
5.213742489502));
#20530=CARTESIAN_POINT('Ctrl Pts',(-2.07927053936707,-1.4206822273389,5.20949904134749));
#20531=CARTESIAN_POINT('Ctrl Pts',(-2.22238787113198,-1.19964805883782,
5.19144218569171));
#20532=CARTESIAN_POINT('Ctrl Pts',(-2.31101455648827,-1.01852606918758,
5.1774116300116));
#20533=CARTESIAN_POINT('Ctrl Pts',(-2.39839943693262,-0.767884266252309,
5.15977470738541));
#20534=CARTESIAN_POINT('Ctrl Pts',(-2.41728564940047,-0.706185116115677,
5.15555772546259));
#20535=CARTESIAN_POINT('Ctrl Pts',(-2.43897931291082,-0.624178737845461,
5.15011190534594));
#20536=CARTESIAN_POINT('Ctrl Pts',(-2.4439382176043,-0.604471019706533,
5.14881496257076));
#20537=CARTESIAN_POINT('Ctrl Pts',(-2.45160529217868,-0.572362441648023,
5.1467205395948));
#20538=CARTESIAN_POINT('Ctrl Pts',(-2.45445918741456,-0.559997660829141,
5.14591844311952));
#20539=CARTESIAN_POINT('Ctrl Pts',(-2.45977204724335,-0.536158023758772,
5.14438034527616));
#20540=CARTESIAN_POINT('Ctrl Pts',(-2.46224450211045,-0.524686544662356,
5.14364393290269));
#20541=CARTESIAN_POINT('Ctrl Pts',(-2.46779332284992,-0.498038299465238,
5.14194163364446));
#20542=CARTESIAN_POINT('Ctrl Pts',(-2.47081007162127,-0.482849499192106,
5.14097765538341));
#20543=CARTESIAN_POINT('Ctrl Pts',(-2.48002501804241,-0.43410430442964,
5.13790331653093));
#20544=CARTESIAN_POINT('Ctrl Pts',(-2.4856813568868,-0.400448498062643,
5.13580998245519));
#20545=CARTESIAN_POINT('Ctrl Pts',(-2.49739482298834,-0.320886960949656,
5.13092271934361));
#20546=CARTESIAN_POINT('Ctrl Pts',(-2.50287340265627,-0.274908056206649,
5.12814620071889));
#20547=CARTESIAN_POINT('Ctrl Pts',(-2.52708725807323,-0.00958669160281925,
5.11233812185545));
#20548=CARTESIAN_POINT('Ctrl Pts',(-2.51825552154817,0.211284599114498,
5.10010925068193));
#20549=CARTESIAN_POINT('Ctrl Pts',(-2.46917851291256,0.495629312918067,
5.08308886645551));
#20550=CARTESIAN_POINT('Ctrl Pts',(-2.4547925588343,0.562567934436855,5.07897784435588));
#20551=CARTESIAN_POINT('Ctrl Pts',(-2.43422362353306,0.642304621406732,
5.07386541939244));
#20552=CARTESIAN_POINT('Ctrl Pts',(-2.43063633277828,0.655749093308375,
5.07299592113837));
#20553=CARTESIAN_POINT('Ctrl Pts',(-2.42488760042545,0.676598753039767,
5.07163485508647));
#20554=CARTESIAN_POINT('Ctrl Pts',(-2.42280319906389,0.6840251473156,5.07114755319548));
#20555=CARTESIAN_POINT('Ctrl Pts',(-2.41889472268292,0.697708424927733,
5.07024485968005));
#20556=CARTESIAN_POINT('Ctrl Pts',(-2.41708044755187,0.703967920136713,
5.06983002920037));
#20557=CARTESIAN_POINT('Ctrl Pts',(-2.41289048720496,0.718216693059688,
5.06888144425261));
#20558=CARTESIAN_POINT('Ctrl Pts',(-2.41049942857921,0.726201226606091,
5.06834682639191));
#20559=CARTESIAN_POINT('Ctrl Pts',(-2.4030017259259,0.750793480825635,5.06669106566961));
#20560=CARTESIAN_POINT('Ctrl Pts',(-2.39776288664475,0.76735991920852,5.0655627692444));
#20561=CARTESIAN_POINT('Ctrl Pts',(-2.38509955493481,0.806008103160726,
5.0629023821986));
#20562=CARTESIAN_POINT('Ctrl Pts',(-2.37753927888408,0.828043383359886,
5.06136386287958));
#20563=CARTESIAN_POINT('Ctrl Pts',(-2.34957682770992,0.906001349191321,
5.05585083568419));
#20564=CARTESIAN_POINT('Ctrl Pts',(-2.32749925548017,0.96129913973336,5.05181156332078));
#20565=CARTESIAN_POINT('Ctrl Pts',(-2.23184105489407,1.17822777274019,5.03557425351062));
#20566=CARTESIAN_POINT('Ctrl Pts',(-2.14320051976757,1.33268035914081,5.02316971068235));
#20567=CARTESIAN_POINT('Ctrl Pts',(-1.98745293853806,1.54776421966146,5.00530566140899));
#20568=CARTESIAN_POINT('Ctrl Pts',(-1.9321612889552,1.61626081773016,4.99950345885724));
#20569=CARTESIAN_POINT('Ctrl Pts',(-1.85838124510524,1.69844936984479,4.99239617219218));
#20570=CARTESIAN_POINT('Ctrl Pts',(-1.84314792697643,1.71496847983924,4.9909595743883));
#20571=CARTESIAN_POINT('Ctrl Pts',(-1.81864656474489,1.74083429619041,4.98869651578299));
#20572=CARTESIAN_POINT('Ctrl Pts',(-1.80952316544436,1.75031577112604,4.98786397516013));
#20573=CARTESIAN_POINT('Ctrl Pts',(-1.79301112695942,1.7672087743431,4.98637506234196));
#20574=CARTESIAN_POINT('Ctrl Pts',(-1.78564987124667,1.77464652710094,4.98571753098342));
#20575=CARTESIAN_POINT('Ctrl Pts',(-1.76829735120659,1.79196208479789,4.98418193579814));
#20576=CARTESIAN_POINT('Ctrl Pts',(-1.75826928521604,1.8018026442891,4.98330551430559));
#20577=CARTESIAN_POINT('Ctrl Pts',(-1.72896599214416,1.83008040077963,4.98077563076421));
#20578=CARTESIAN_POINT('Ctrl Pts',(-1.70947911242897,1.84829622155621,4.97913165863776));
#20579=CARTESIAN_POINT('Ctrl Pts',(-1.66470943289628,1.88883186115741,4.97543720539586));
#20580=CARTESIAN_POINT('Ctrl Pts',(-1.63926004935121,1.91096047562378,4.97339446686066));
#20581=CARTESIAN_POINT('Ctrl Pts',(-1.5534247573338,1.98261852516899,4.96667961332971));
#20582=CARTESIAN_POINT('Ctrl Pts',(-1.49117773052985,2.02985098470629,4.96208958936225));
#20583=CARTESIAN_POINT('Ctrl Pts',(-1.29699391176685,2.16343446891779,4.94839785901126));
#20584=CARTESIAN_POINT('Ctrl Pts',(-1.1590633456091,2.24035934814638,4.93950759087748));
#20585=CARTESIAN_POINT('Ctrl Pts',(-0.980537396851379,2.31899952566037,
4.9280518150789));
#20586=CARTESIAN_POINT('Ctrl Pts',(-0.94588865729387,2.33334669678435,4.92582948336285));
#20587=CARTESIAN_POINT('Ctrl Pts',(-0.87103399495885,2.36240087034972,4.9210049780843));
#20588=CARTESIAN_POINT('Ctrl Pts',(-0.830748287170026,2.37686661068305,
4.91839436507727));
#20589=CARTESIAN_POINT('Ctrl Pts',(-0.778532670600854,2.3941265571579,4.91496913413278));
#20590=CARTESIAN_POINT('Ctrl Pts',(-0.766921661508516,2.39787118961044,
4.91420487082656));
#20591=CARTESIAN_POINT('Ctrl Pts',(-0.748364102276225,2.40370756214885,
4.91297854083794));
#20592=CARTESIAN_POINT('Ctrl Pts',(-0.741434764551357,2.40585397741949,
4.91251956454737));
#20593=CARTESIAN_POINT('Ctrl Pts',(-0.728170045990337,2.40990007676248,
4.91163874208495));
#20594=CARTESIAN_POINT('Ctrl Pts',(-0.721836350474372,2.41180477545543,
4.91121718691396));
#20595=CARTESIAN_POINT('Ctrl Pts',(-0.706740563891648,2.41627966227534,
4.91021021680694));
#20596=CARTESIAN_POINT('Ctrl Pts',(-0.697971904485111,2.41882716318682,
4.90962352338039));
#20597=CARTESIAN_POINT('Ctrl Pts',(-0.668221110241237,2.42729522366124,
4.90762740351304));
#20598=CARTESIAN_POINT('Ctrl Pts',(-0.647176655283755,2.43299072257802,
4.90620610507695));
#20599=CARTESIAN_POINT('Ctrl Pts',(-0.595697615316425,2.44620795496882,
4.9027110232013));
#20600=CARTESIAN_POINT('Ctrl Pts',(-0.565191888532306,2.45343574493739,
4.9006244390631));
#20601=CARTESIAN_POINT('Ctrl Pts',(-0.441218789015813,2.48037422811033,
4.89210297107627));
#20602=CARTESIAN_POINT('Ctrl Pts',(-0.346803498109627,2.4953267446186,4.88552086845927));
#20603=CARTESIAN_POINT('Ctrl Pts',(-0.0527297734357414,2.52488502687459,
4.86510603044115));
#20604=CARTESIAN_POINT('Ctrl Pts',(0.148028322265435,2.52109926485449,4.85136063564229));
#20605=CARTESIAN_POINT('Ctrl Pts',(0.377381707151431,2.4892523867735,4.83633409965327));
#20606=CARTESIAN_POINT('Ctrl Pts',(0.408435175550585,2.48434604097104,4.83431208699742));
#20607=CARTESIAN_POINT('Ctrl Pts',(0.454149540200648,2.47624294849541,4.83135274200616));
#20608=CARTESIAN_POINT('Ctrl Pts',(0.468885879539872,2.47349489440385,4.83040143843833));
#20609=CARTESIAN_POINT('Ctrl Pts',(0.495048174979353,2.46837389925695,4.82871701919486));
#20610=CARTESIAN_POINT('Ctrl Pts',(0.506483721125436,2.46605284811969,4.82798228952315));
#20611=CARTESIAN_POINT('Ctrl Pts',(0.530555048926457,2.46099263339741,4.82643877389073));
#20612=CARTESIAN_POINT('Ctrl Pts',(0.54318673069177,2.45823546209455,4.82563058182078));
#20613=CARTESIAN_POINT('Ctrl Pts',(0.576686211217743,2.45065256409399,4.82349164490495));
#20614=CARTESIAN_POINT('Ctrl Pts',(0.597514905203522,2.44565757167712,4.82216630136789));
#20615=CARTESIAN_POINT('Ctrl Pts',(0.700286369158245,2.41962028727449,4.8156461055526));
#20616=CARTESIAN_POINT('Ctrl Pts',(0.781200640062332,2.39472150350713,4.81057589382786));
#20617=CARTESIAN_POINT('Ctrl Pts',(1.04208450983859,2.29980768000398,4.79423109796298));
#20618=CARTESIAN_POINT('Ctrl Pts',(1.21525311579265,2.21318999624887,4.78342971419582));
#20619=CARTESIAN_POINT('Ctrl Pts',(1.44160217561186,2.06532729588902,4.76756265704338));
#20620=CARTESIAN_POINT('Ctrl Pts',(1.504391363471,2.02004897692823,4.7629382400568));
#20621=CARTESIAN_POINT('Ctrl Pts',(1.57525990343738,1.96380610075467,4.75732539260183));
#20622=CARTESIAN_POINT('Ctrl Pts',(1.58546614983903,1.95557542311832,4.75650702445257));
#20623=CARTESIAN_POINT('Ctrl Pts',(1.60197152502219,1.94205076653459,4.75516629177455));
#20624=CARTESIAN_POINT('Ctrl Pts',(1.60830995542125,1.93680485066354,4.75464721232406));
#20625=CARTESIAN_POINT('Ctrl Pts',(1.61961782581343,1.92735226133159,4.75371336168882));
#20626=CARTESIAN_POINT('Ctrl Pts',(1.62459680010945,1.92315726767796,4.75329942609349));
#20627=CARTESIAN_POINT('Ctrl Pts',(1.62960637340882,1.91890315584798,4.75288014057315));
#20628=CARTESIAN_POINT('Ctrl Pts',(1.62965322346661,1.91886336799233,4.75287621912359));
#20629=CARTESIAN_POINT('Ctrl Pts',(1.62974579673245,1.91878474343315,4.75286847005589));
#20630=CARTESIAN_POINT('Ctrl Pts',(1.62979152002562,1.91874590679733,4.75286464244233));
#20631=CARTESIAN_POINT('Ctrl Pts',(1.62988188058262,1.91866915042142,4.75285707766432));
#20632=CARTESIAN_POINT('Ctrl Pts',(1.62992651790169,1.91863123076616,4.75285334050626));
#20633=CARTESIAN_POINT('Ctrl Pts',(1.63001474534562,1.91855627575205,4.75284595342067));
#20634=CARTESIAN_POINT('Ctrl Pts',(1.63005833553188,1.9185192404651,4.75284230349837));
#20635=CARTESIAN_POINT('Ctrl Pts',(1.6301445057419,1.91844602309309,4.75283508781444));
#20636=CARTESIAN_POINT('Ctrl Pts',(1.6301870858217,1.91840984107733,4.75283152205789));
#20637=CARTESIAN_POINT('Ctrl Pts',(1.6302712711175,1.91833830060032,4.75282447177856));
#20638=CARTESIAN_POINT('Ctrl Pts',(1.63031287639333,1.91830294219848,4.75282098726));
#20639=CARTESIAN_POINT('Ctrl Pts',(1.6303951457655,1.91823302065012,4.75281409666296));
#20640=CARTESIAN_POINT('Ctrl Pts',(1.6304358099162,1.91819845756144,4.75281069058863));
#20641=CARTESIAN_POINT('Ctrl Pts',(1.6305162292395,1.91813009957854,4.75280395420877));
#20642=CARTESIAN_POINT('Ctrl Pts',(1.63055598444249,1.91809630475671,4.75280062390889));
#20643=CARTESIAN_POINT('Ctrl Pts',(1.6306346165123,1.91802945755159,4.75279403653548));
#20644=CARTESIAN_POINT('Ctrl Pts',(1.63067349345178,1.91799640519935,4.75279077946363));
#20645=CARTESIAN_POINT('Ctrl Pts',(1.63075039838825,1.91793101821943,4.75278433610682));
#20646=CARTESIAN_POINT('Ctrl Pts',(1.63078842642159,1.91789868364861,4.75278114982615));
#20647=CARTESIAN_POINT('Ctrl Pts',(1.63086366159562,1.91783470864212,4.75277484572332));
#20648=CARTESIAN_POINT('Ctrl Pts',(1.63090086877354,1.91780306825785,4.75277172790498));
#20649=CARTESIAN_POINT('Ctrl Pts',(1.63097448908139,1.91774045904306,4.75276555849799));
#20650=CARTESIAN_POINT('Ctrl Pts',(1.63101090224037,1.91770949026646,4.75276250691349));
#20651=CARTESIAN_POINT('Ctrl Pts',(1.63108296018502,1.91764820266488,4.75275646784209));
#20652=CARTESIAN_POINT('Ctrl Pts',(1.63111860500452,1.9176178838856,4.75275348035858));
#20653=CARTESIAN_POINT('Ctrl Pts',(1.63118915082847,1.91755787561133,4.75274756744943));
#20654=CARTESIAN_POINT('Ctrl Pts',(1.63122405188274,1.91752818614455,4.7527446420255));
#20655=CARTESIAN_POINT('Ctrl Pts',(1.63129313370655,1.91746941668853,4.75273885128076));
#20656=CARTESIAN_POINT('Ctrl Pts',(1.63132731452337,1.91744033672601,4.75273598596157));
#20657=CARTESIAN_POINT('Ctrl Pts',(1.6313949785099,1.91738276721824,4.75273031354528));
#20658=CARTESIAN_POINT('Ctrl Pts',(1.63142846168033,1.91735427773589,4.75272750645343));
#20659=CARTESIAN_POINT('Ctrl Pts',(1.63149475192016,1.91729787104473,4.75272194870129));
#20660=CARTESIAN_POINT('Ctrl Pts',(1.6315275590418,1.91726995385177,4.75271919804166));
#20661=CARTESIAN_POINT('Ctrl Pts',(1.63159251796458,1.91721467423563,4.75271375142668));
#20662=CARTESIAN_POINT('Ctrl Pts',(1.63162466978812,1.91718731185069,4.75271105547422));
#20663=CARTESIAN_POINT('Ctrl Pts',(1.63168833800625,1.91713312509258,4.75270571661992));
#20664=CARTESIAN_POINT('Ctrl Pts',(1.6317198544294,1.91710630074957,4.75270307372023));
#20665=CARTESIAN_POINT('Ctrl Pts',(1.63178227092494,1.91705317399953,4.75269783938514));
#20666=CARTESIAN_POINT('Ctrl Pts',(1.63181317103331,1.91702687161366,4.75269524795106));
#20667=CARTESIAN_POINT('Ctrl Pts',(1.63187437328153,1.9169747732849,4.75269011501845));
#20668=CARTESIAN_POINT('Ctrl Pts',(1.63190467542814,1.91694897738553,4.75268757352348));
#20669=CARTESIAN_POINT('Ctrl Pts',(1.63196469934903,1.91689787719699,4.75268253900554));
#20670=CARTESIAN_POINT('Ctrl Pts',(1.63199442114572,1.91687257293565,4.75268004598462));
#20671=CARTESIAN_POINT('Ctrl Pts',(1.63205330128584,1.91682244175839,4.75267510700729));
#20672=CARTESIAN_POINT('Ctrl Pts',(1.63208245965654,1.91679761486393,4.75267266105233));
#20673=CARTESIAN_POINT('Ctrl Pts',(1.63214022922484,1.91674842469169,4.75266781485241));
#20674=CARTESIAN_POINT('Ctrl Pts',(1.63216884044255,1.91672406143936,4.7526654146093));
#20675=CARTESIAN_POINT('Ctrl Pts',(1.63222553137195,1.91667578533717,4.75266065852934));
#20676=CARTESIAN_POINT('Ctrl Pts',(1.63225361109485,1.91665187251835,4.75265830269492));
#20677=CARTESIAN_POINT('Ctrl Pts',(1.63230925407908,1.91660448459212,4.75265363418023));
#20678=CARTESIAN_POINT('Ctrl Pts',(1.63233681736609,1.91658100950154,4.75265132150104));
#20679=CARTESIAN_POINT('Ctrl Pts',(1.63239144192669,1.91653448484187,4.75264673809416));
#20680=CARTESIAN_POINT('Ctrl Pts',(1.63241850324724,1.91651143526973,4.75264446736561));
#20681=CARTESIAN_POINT('Ctrl Pts',(1.63247213787864,1.91646574982922,4.75263996669418));
#20682=CARTESIAN_POINT('Ctrl Pts',(1.63249871119377,1.91644311399248,4.75263773675387));
#20683=CARTESIAN_POINT('Ctrl Pts',(1.63255138328412,1.91639824465391,4.75263331653733));
#20684=CARTESIAN_POINT('Ctrl Pts',(1.63257748205064,1.91637601119318,4.75263112626464));
#20685=CARTESIAN_POINT('Ctrl Pts',(1.63262921791013,1.91633193574613,4.75262678431195));
#20686=CARTESIAN_POINT('Ctrl Pts',(1.63265485504277,1.91631009375821,4.75262463263131));
#20687=CARTESIAN_POINT('Ctrl Pts',(1.63270568017682,1.91626679066704,4.75262036681807));
#20688=CARTESIAN_POINT('Ctrl Pts',(1.63273086817529,1.91624532959707,4.75261825268828));
#20689=CARTESIAN_POINT('Ctrl Pts',(1.63278080701975,1.91620277822712,4.75261406097898));
#20690=CARTESIAN_POINT('Ctrl Pts',(1.63280555789136,1.91618168793476,4.75261198339977));
#20691=CARTESIAN_POINT('Ctrl Pts',(1.6391588304552,1.9107678327417,4.75207867428604));
#20692=CARTESIAN_POINT('Ctrl Pts',(1.64546049089582,1.9053438404436,4.75154518615882));
#20693=CARTESIAN_POINT('Ctrl Pts',(1.66463752982013,1.88867160829619,4.74990815432789));
#20694=CARTESIAN_POINT('Ctrl Pts',(1.67742498848545,1.87732360559165,4.74879775780544));
#20695=CARTESIAN_POINT('Ctrl Pts',(1.70739940553356,1.85017259237463,4.7461521073417));
#20696=CARTESIAN_POINT('Ctrl Pts',(1.72448383043867,1.83425919316251,4.74461010133018));
#20697=CARTESIAN_POINT('Ctrl Pts',(1.78447788478779,1.7767983075371,4.73907998321365));
#20698=CARTESIAN_POINT('Ctrl Pts',(1.82612549743954,1.73396606487033,4.73502671276063));
#20699=CARTESIAN_POINT('Ctrl Pts',(1.98608829622687,1.55729300844135,4.71870252679664));
#20700=CARTESIAN_POINT('Ctrl Pts',(2.09155176009271,1.41249073707705,4.70622488586076));
#20701=CARTESIAN_POINT('Ctrl Pts',(2.22414725145006,1.18258318892851,4.68838087862704));
#20702=CARTESIAN_POINT('Ctrl Pts',(2.263583151661,1.10522767257613,4.6826600644618));
#20703=CARTESIAN_POINT('Ctrl Pts',(2.30807433911545,1.00553490477725,4.67563550199438));
#20704=CARTESIAN_POINT('Ctrl Pts',(2.31692654013989,0.98496652741267,4.67420400112456));
#20705=CARTESIAN_POINT('Ctrl Pts',(2.33053667777167,0.952143749777371,4.67194708862268));
#20706=CARTESIAN_POINT('Ctrl Pts',(2.33547492215656,0.939965863899505,4.67111565336464));
#20707=CARTESIAN_POINT('Ctrl Pts',(2.34417481929611,0.918019725400779,4.66962771806396));
#20708=CARTESIAN_POINT('Ctrl Pts',(2.34797130142708,0.90826569496149,4.66897006797735));
#20709=CARTESIAN_POINT('Ctrl Pts',(2.35499248616887,0.889888414752341,4.6677377694359));
#20710=CARTESIAN_POINT('Ctrl Pts',(2.35823090787457,0.881270666679349,4.66716267736481));
#20711=CARTESIAN_POINT('Ctrl Pts',(2.36142200727925,0.872635292397265,4.66658913197125));
#20712=CARTESIAN_POINT('Origin',(0.,0.,10.));
#20713=CARTESIAN_POINT('',(2.36142196837105,0.872635397685999,3.66998323165053));
#20714=CARTESIAN_POINT('',(2.36142200728636,0.872635292378021,3.9436931725108));
#20715=CARTESIAN_POINT('',(2.36142200728636,0.87263529237802,10.));
#20716=CARTESIAN_POINT('',(2.51749952702257,0.00154319187075679,4.88741669746642));
#20717=CARTESIAN_POINT('Ctrl Pts',(2.36142200728636,0.872635292378021,3.9436931725108));
#20718=CARTESIAN_POINT('Ctrl Pts',(2.34093516802426,0.928074344082446,3.94744670184164));
#20719=CARTESIAN_POINT('Ctrl Pts',(2.31851215292549,0.982746025527077,3.95120023117247));
#20720=CARTESIAN_POINT('Ctrl Pts',(2.29421643254441,1.03652168845771,3.95495376050331));
#20721=CARTESIAN_POINT('Ctrl Pts',(2.26020042817918,1.11181203409469,3.96020900990937));
#20722=CARTESIAN_POINT('Ctrl Pts',(2.22241142210613,1.18556516925875,3.96546425931544));
#20723=CARTESIAN_POINT('Ctrl Pts',(2.18101071131842,1.25737763902272,3.97071950872151));
#20724=CARTESIAN_POINT('Ctrl Pts',(2.13966869733361,1.32908829501817,3.97596730737775));
#20725=CARTESIAN_POINT('Ctrl Pts',(2.09472537813039,1.39886335432976,3.98121510603399));
#20726=CARTESIAN_POINT('Ctrl Pts',(2.04638950247262,1.46632065189366,3.98646290469024));
#20727=CARTESIAN_POINT('Ctrl Pts',(1.99770339171077,1.5342667357537,3.99174872817346));
#20728=CARTESIAN_POINT('Ctrl Pts',(1.94557554816624,1.5998608959182,3.99703455165667));
#20729=CARTESIAN_POINT('Ctrl Pts',(1.89026576924196,1.66273917727108,4.00232037513989));
#20730=CARTESIAN_POINT('Ctrl Pts',(1.83545194930389,1.72505363339665,4.00755880100723));
#20731=CARTESIAN_POINT('Ctrl Pts',(1.77751334019645,1.78470036898949,4.01279722687456));
#20732=CARTESIAN_POINT('Ctrl Pts',(1.71674433469282,1.84135687450861,4.0180356527419));
#20733=CARTESIAN_POINT('Ctrl Pts',(1.65599531510379,1.89799474664594,4.02327235577815));
#20734=CARTESIAN_POINT('Ctrl Pts',(1.59241808510542,1.95164402746345,4.02850905881439));
#20735=CARTESIAN_POINT('Ctrl Pts',(1.52634356492189,2.00201937348806,4.03374576185064));
#20736=CARTESIAN_POINT('Ctrl Pts',(1.46027084457531,2.05239334731339,4.03898232224171));
#20737=CARTESIAN_POINT('Ctrl Pts',(1.39170133686044,2.09949328472293,4.04421888263278));
#20738=CARTESIAN_POINT('Ctrl Pts',(1.32099756813324,2.14307528448864,4.04945544302385));
#20739=CARTESIAN_POINT('Ctrl Pts',(1.24913656926093,2.18737060413561,4.05477771179582));
#20740=CARTESIAN_POINT('Ctrl Pts',(1.17507122655244,2.22803151965106,4.06009998056779));
#20741=CARTESIAN_POINT('Ctrl Pts',(1.09920949497462,2.26484982640299,4.06542224933976));
#20742=CARTESIAN_POINT('Ctrl Pts',(1.02446222774625,2.30112724528657,4.07066633008885));
#20743=CARTESIAN_POINT('Ctrl Pts',(0.947971456517051,2.33367408067572,4.07591041083793));
#20744=CARTESIAN_POINT('Ctrl Pts',(0.870147202928374,2.36233996182512,4.08115449158702));
#20745=CARTESIAN_POINT('Ctrl Pts',(0.790582437090273,2.39164694539416,4.08651585437043));
#20746=CARTESIAN_POINT('Ctrl Pts',(0.70962431222964,2.41689713515886,4.09187721715384));
#20747=CARTESIAN_POINT('Ctrl Pts',(0.627724945719765,2.43798434008939,4.09723857993726));
#20748=CARTESIAN_POINT('Ctrl Pts',(0.545825579209892,2.45907154501993,4.10259994272067));
#20749=CARTESIAN_POINT('Ctrl Pts',(0.462985482245224,2.47599572885717,4.10796130550408));
#20750=CARTESIAN_POINT('Ctrl Pts',(0.379663322338168,2.48870689549234,4.11332266828749));
#20751=CARTESIAN_POINT('Ctrl Pts',(0.297990294582247,2.50116647967214,4.11857791769423));
#20752=CARTESIAN_POINT('Ctrl Pts',(0.21555245044207,2.50962436248483,4.12383316710096));
#20753=CARTESIAN_POINT('Ctrl Pts',(0.132776023197794,2.51399617693897,4.12908841650769));
#20754=CARTESIAN_POINT('Ctrl Pts',(0.0501169541230106,2.51836179315337,
4.1343362151646));
#20755=CARTESIAN_POINT('Ctrl Pts',(-0.0328792876339783,2.51865282369693,
4.13958401382151));
#20756=CARTESIAN_POINT('Ctrl Pts',(-0.115778491375535,2.51483629505676,
4.14483181247842));
#20757=CARTESIAN_POINT('Ctrl Pts',(-0.199278371327402,2.51099211237582,
4.15011763596147));
#20758=CARTESIAN_POINT('Ctrl Pts',(-0.282679332614184,2.50298052226196,
4.15540345944452));
#20759=CARTESIAN_POINT('Ctrl Pts',(-0.36553464539088,2.4908212848414,4.16068928292757));
#20760=CARTESIAN_POINT('Ctrl Pts',(-0.447647000285111,2.47877107846524,
4.16592770879555));
#20761=CARTESIAN_POINT('Ctrl Pts',(-0.529222988118453,2.46264737843161,
4.17116613466353));
#20762=CARTESIAN_POINT('Ctrl Pts',(-0.609831807771019,2.44252152830446,
4.1764045605315));
#20763=CARTESIAN_POINT('Ctrl Pts',(-0.690414116524153,2.4224022972345,4.18164126356838));
#20764=CARTESIAN_POINT('Ctrl Pts',(-0.77002944150669,2.39828364188206,4.18687796660525));
#20765=CARTESIAN_POINT('Ctrl Pts',(-0.848258268782068,2.37028777987882,
4.19211466964213));
#20766=CARTESIAN_POINT('Ctrl Pts',(-0.926484965143172,2.3422926804689,4.19735123003382));
#20767=CARTESIAN_POINT('Ctrl Pts',(-1.00332480479719,2.31042074083838,4.20258779042552));
#20768=CARTESIAN_POINT('Ctrl Pts',(-1.07837582723516,2.27484325289345,4.20782435081721));
#20769=CARTESIAN_POINT('Ctrl Pts',(-1.15465523262542,2.23868345736289,4.21314661958842));
#20770=CARTESIAN_POINT('Ctrl Pts',(-1.22908628631208,2.19869591822691,4.21846888835962));
#20771=CARTESIAN_POINT('Ctrl Pts',(-1.30127223613778,2.15510946762734,4.22379115713083));
#20772=CARTESIAN_POINT('Ctrl Pts',(-1.37239772155604,2.11216333387084,4.22903523788051));
#20773=CARTESIAN_POINT('Ctrl Pts',(-1.44134327579444,2.06572364040126,4.23427931863019));
#20774=CARTESIAN_POINT('Ctrl Pts',(-1.50775953210907,2.01605244062109,4.23952339937987));
#20775=CARTESIAN_POINT('Ctrl Pts',(-1.5756611647726,1.96527036182622,4.24488476216184));
#20776=CARTESIAN_POINT('Ctrl Pts',(-1.64091860658684,1.91111081651486,4.2502461249438));
#20777=CARTESIAN_POINT('Ctrl Pts',(-1.70319662932577,1.85389522137939,4.25560748772577));
#20778=CARTESIAN_POINT('Ctrl Pts',(-1.7654746520647,1.79667962624392,4.26096885050774));
#20779=CARTESIAN_POINT('Ctrl Pts',(-1.82477294699385,1.73640839032897,4.2663302132897));
#20780=CARTESIAN_POINT('Ctrl Pts',(-1.88079985551992,1.67343901994553,4.27169157607167));
#20781=CARTESIAN_POINT('Ctrl Pts',(-1.93571786607732,1.61171595439566,4.27694682547964));
#20782=CARTESIAN_POINT('Ctrl Pts',(-1.98769568587252,1.54717263420609,4.28220207488761));
#20783=CARTESIAN_POINT('Ctrl Pts',(-2.03643048514925,1.48012064682403,4.28745732429558));
#20784=CARTESIAN_POINT('Ctrl Pts',(-2.08509618955193,1.41316372392755,4.29270512295376));
#20785=CARTESIAN_POINT('Ctrl Pts',(-2.13052773711959,1.3437055686568,4.29795292161193));
#20786=CARTESIAN_POINT('Ctrl Pts',(-2.17246106323187,1.27209244111481,4.3032007202701));
#20787=CARTESIAN_POINT('Ctrl Pts',(-2.21469823243587,1.19996041473755,4.30848654375284));
#20788=CARTESIAN_POINT('Ctrl Pts',(-2.25338595601427,1.12564240909209,4.31377236723558));
#20789=CARTESIAN_POINT('Ctrl Pts',(-2.28829758584728,1.04952389615744,4.31905819071832));
#20790=CARTESIAN_POINT('Ctrl Pts',(-2.32289616551108,0.974087932661735,
4.32429661658761));
#20791=CARTESIAN_POINT('Ctrl Pts',(-2.35378590423559,0.896884049737827,
4.32953504245689));
#20792=CARTESIAN_POINT('Ctrl Pts',(-2.38079209410969,0.81831244315651,4.33477346832618));
#20793=CARTESIAN_POINT('Ctrl Pts',(-2.40778940209743,0.739766677468888,
4.34001017136439));
#20794=CARTESIAN_POINT('Ctrl Pts',(-2.4309055480264,0.659854517514087,4.34524687440259));
#20795=CARTESIAN_POINT('Ctrl Pts',(-2.45001464208563,0.578994389926193,
4.3504835774408));
#20796=CARTESIAN_POINT('Ctrl Pts',(-2.46912321562272,0.498136464927666,
4.35572013783384));
#20797=CARTESIAN_POINT('Ctrl Pts',(-2.48422484919077,0.416331072925899,
4.36095669822688));
#20798=CARTESIAN_POINT('Ctrl Pts',(-2.49524437309276,0.334008635440673,
4.36619325861992));
#20799=CARTESIAN_POINT('Ctrl Pts',(-2.50644425689397,0.250338801583255,
4.37151552738958));
#20800=CARTESIAN_POINT('Ctrl Pts',(-2.51342712092159,0.166135329894889,
4.37683779615924));
#20801=CARTESIAN_POINT('Ctrl Pts',(-2.51616889547945,0.0818556010405808,
4.3821600649289));
#20802=CARTESIAN_POINT('Ctrl Pts',(-2.51887039136492,-0.00118599699139293,
4.38740414567994));
#20803=CARTESIAN_POINT('Ctrl Pts',(-2.51745464937952,-0.0843011596064944,
4.39264822643099));
#20804=CARTESIAN_POINT('Ctrl Pts',(-2.51195126462655,-0.167054165291002,
4.39789230718203));
#20805=CARTESIAN_POINT('Ctrl Pts',(-2.50632479860254,-0.251657912942316,
4.403253669961));
#20806=CARTESIAN_POINT('Ctrl Pts',(-2.49642570589058,-0.335882600626038,
4.40861503273997));
#20807=CARTESIAN_POINT('Ctrl Pts',(-2.4823410728014,-0.419272045673439,
4.41397639551893));
#20808=CARTESIAN_POINT('Ctrl Pts',(-2.46825643971223,-0.502661490720837,
4.4193377582979));
#20809=CARTESIAN_POINT('Ctrl Pts',(-2.44998644125835,-0.585215211462834,
4.42469912107687));
#20810=CARTESIAN_POINT('Ctrl Pts',(-2.42767215699857,-0.666493922053232,
4.43006048385584));
#20811=CARTESIAN_POINT('Ctrl Pts',(-2.40579952237929,-0.746163945002343,
4.43531573326292));
#20812=CARTESIAN_POINT('Ctrl Pts',(-2.37996048847709,-0.824903250665136,
4.44057098267001));
#20813=CARTESIAN_POINT('Ctrl Pts',(-2.35025153630514,-0.902288183506419,
4.44582623207709));
#20814=CARTESIAN_POINT('Ctrl Pts',(-2.32058470467833,-0.979563402092642,
4.45107403073436));
#20815=CARTESIAN_POINT('Ctrl Pts',(-2.28705901689624,-1.05548763474825,
4.45632182939163));
#20816=CARTESIAN_POINT('Ctrl Pts',(-2.24982114286705,-1.12965086425338,
4.4615696280489));
#20817=CARTESIAN_POINT('Ctrl Pts',(-2.21231344833568,-1.20435147029651,
4.46685545153187));
#20818=CARTESIAN_POINT('Ctrl Pts',(-2.17103967004633,-1.27726498855752,
4.47214127501483));
#20819=CARTESIAN_POINT('Ctrl Pts',(-2.12619973999849,-1.34799143752116,
4.47742709849779));
#20820=CARTESIAN_POINT('Ctrl Pts',(-2.08176188651069,-1.41808368729509,
4.48266552436616));
#20821=CARTESIAN_POINT('Ctrl Pts',(-2.0338218316076,-1.48602753639573,4.48790395023452));
#20822=CARTESIAN_POINT('Ctrl Pts',(-1.98262013641925,-1.55145855396299,
4.49314237610289));
#20823=CARTESIAN_POINT('Ctrl Pts',(-1.93143528061632,-1.61686805235751,
4.49837907914017));
#20824=CARTESIAN_POINT('Ctrl Pts',(-1.87699119910284,-1.67976599745249,
4.50361578217744));
#20825=CARTESIAN_POINT('Ctrl Pts',(-1.81957032400716,-1.73981898081164,
4.50885248521472));
#20826=CARTESIAN_POINT('Ctrl Pts',(-1.76215101302744,-1.79987032835752,
4.51408904560682));
#20827=CARTESIAN_POINT('Ctrl Pts',(-1.7017553893145,-1.85707653546034,4.51932560599892));
#20828=CARTESIAN_POINT('Ctrl Pts',(-1.63870356085949,-1.91114020668982,
4.52456216639102));
#20829=CARTESIAN_POINT('Ctrl Pts',(-1.57461974392674,-1.96608875449054,
4.52988443516177));
#20830=CARTESIAN_POINT('Ctrl Pts',(-1.50779235269812,-2.01779063858759,
4.53520670393252));
#20831=CARTESIAN_POINT('Ctrl Pts',(-1.43859192976348,-2.0659766478882,4.54052897270327));
#20832=CARTESIAN_POINT('Ctrl Pts',(-1.37040811165095,-2.11345476947172,
4.54577305345338));
#20833=CARTESIAN_POINT('Ctrl Pts',(-1.29992095154826,-2.15751943604622,
4.55101713420348));
#20834=CARTESIAN_POINT('Ctrl Pts',(-1.22751204239967,-2.19795824249775,
4.55626121495359));
#20835=CARTESIAN_POINT('Ctrl Pts',(-1.15348373333534,-2.2393014487052,4.56162257773466));
#20836=CARTESIAN_POINT('Ctrl Pts',(-1.07744713857565,-2.27685442881522,
4.56698394051573));
#20837=CARTESIAN_POINT('Ctrl Pts',(-0.99983231490222,-2.31044186078708,
4.5723453032968));
#20838=CARTESIAN_POINT('Ctrl Pts',(-0.922217491228789,-2.34402929275895,
4.57770666607787));
#20839=CARTESIAN_POINT('Ctrl Pts',(-0.843024937947763,-2.37365106114631,
4.58306802885894));
#20840=CARTESIAN_POINT('Ctrl Pts',(-0.762699935624585,-2.3991863325299,
4.58842939164001));
#20841=CARTESIAN_POINT('Ctrl Pts',(-0.683964744949417,-2.42421620371794,
4.59368464104726));
#20842=CARTESIAN_POINT('Ctrl Pts',(-0.603850720472383,-2.44541235930782,
4.59893989045451));
#20843=CARTESIAN_POINT('Ctrl Pts',(-0.522765750426252,-2.46262506691158,
4.60419513986177));
#20844=CARTESIAN_POINT('Ctrl Pts',(-0.441795740447352,-2.47981337080623,
4.60944293851921));
#20845=CARTESIAN_POINT('Ctrl Pts',(-0.359857966786886,-2.49302934952906,
4.61469073717665));
#20846=CARTESIAN_POINT('Ctrl Pts',(-0.277376203386156,-2.50217279415213,
4.61993853583409));
#20847=CARTESIAN_POINT('Ctrl Pts',(-0.194296788500819,-2.5113824909142,
4.62522435931701));
#20848=CARTESIAN_POINT('Ctrl Pts',(-0.110665918879123,-2.5164602429421,
4.63051018279993));
#20849=CARTESIAN_POINT('Ctrl Pts',(-0.026927949219451,-2.51735598109422,
4.63579600628285));
#20850=CARTESIAN_POINT('Ctrl Pts',(0.0560591478451705,-2.51824368722415,
4.64103443215139));
#20851=CARTESIAN_POINT('Ctrl Pts',(0.139150962027135,-2.51502407372522,
4.64627285801992));
#20852=CARTESIAN_POINT('Ctrl Pts',(0.221910837649735,-2.50770050646675,
4.65151128388845));
#20853=CARTESIAN_POINT('Ctrl Pts',(0.304643494926548,-2.50037934780767,
4.65674798692589));
#20854=CARTESIAN_POINT('Ctrl Pts',(0.387043971197711,-2.48895695665212,
4.66198468996334));
#20855=CARTESIAN_POINT('Ctrl Pts',(0.468678835425855,-2.47348871014684,
4.66722139300078));
#20856=CARTESIAN_POINT('Ctrl Pts',(0.550311475961083,-2.45802088498886,
4.67245795339305));
#20857=CARTESIAN_POINT('Ctrl Pts',(0.631178092756059,-2.43850751051613,
4.67769451378532));
#20858=CARTESIAN_POINT('Ctrl Pts',(0.710854949522729,-2.4150551734358,4.68293107417759));
#20859=CARTESIAN_POINT('Ctrl Pts',(0.791835901662793,-2.3912189848141,4.68825334294814));
#20860=CARTESIAN_POINT('Ctrl Pts',(0.871587320643905,-2.36331385611791,
4.69357561171869));
#20861=CARTESIAN_POINT('Ctrl Pts',(0.949681651786961,-2.33150402321317,
4.69889788048924));
#20862=CARTESIAN_POINT('Ctrl Pts',(1.02662872009707,-2.30016150001554,4.70414196123951));
#20863=CARTESIAN_POINT('Ctrl Pts',(1.10196666682185,-2.26502849041801,4.70938604198977));
#20864=CARTESIAN_POINT('Ctrl Pts',(1.17530956931617,-2.22630942734245,4.71463012274004));
#20865=CARTESIAN_POINT('Ctrl Pts',(1.25029276015298,-2.18672442597381,4.71999148552073));
#20866=CARTESIAN_POINT('Ctrl Pts',(1.3231901528623,-2.14339129554255,4.72535284830142));
#20867=CARTESIAN_POINT('Ctrl Pts',(1.39362054358296,-2.09657531000046,4.73071421108212));
#20868=CARTESIAN_POINT('Ctrl Pts',(1.46405093430362,-2.04975932445837,4.73607557386281));
#20869=CARTESIAN_POINT('Ctrl Pts',(1.53201395435211,-1.99946083976464,4.7414369366435));
#20870=CARTESIAN_POINT('Ctrl Pts',(1.59716581588964,-1.94598756587846,4.74679829942419));
#20871=CARTESIAN_POINT('Ctrl Pts',(1.66018580041307,-1.89426402624049,4.75198422951874));
#20872=CARTESIAN_POINT('Ctrl Pts',(1.72082195295255,-1.83936794722174,4.7571701596133));
#20873=CARTESIAN_POINT('Ctrl Pts',(1.77873133380433,-1.7815501935513,4.76235608970785));
#20874=CARTESIAN_POINT('Ctrl Pts',(1.83691908277286,-1.72345451221237,4.76756694836446));
#20875=CARTESIAN_POINT('Ctrl Pts',(1.89235335502451,-1.66240923773946,4.77277780702107));
#20876=CARTESIAN_POINT('Ctrl Pts',(1.94471789917397,-1.5987115257708,4.77798866567767));
#20877=CARTESIAN_POINT('Ctrl Pts',(1.9966980531484,-1.53548139687862,4.78316127320647));
#20878=CARTESIAN_POINT('Ctrl Pts',(2.04565307367945,-1.4696379988575,4.78833388073526));
#20879=CARTESIAN_POINT('Ctrl Pts',(2.09131013993223,-1.40150923957591,4.79350648826406));
#20880=CARTESIAN_POINT('Ctrl Pts',(2.13693972349127,-1.33342148953955,4.79867598220716));
#20881=CARTESIAN_POINT('Ctrl Pts',(2.17927502808787,-1.26305150123698,4.80384547615025));
#20882=CARTESIAN_POINT('Ctrl Pts',(2.21808489358847,-1.19075843681018,4.80901497009335));
#20883=CARTESIAN_POINT('Ctrl Pts',(2.25688384820123,-1.11848569663618,4.8141830107006));
#20884=CARTESIAN_POINT('Ctrl Pts',(2.29215910763938,-1.04429137212952,4.81935105130785));
#20885=CARTESIAN_POINT('Ctrl Pts',(2.32372486071905,-0.968560282933497,
4.82451909191511));
#20886=CARTESIAN_POINT('Ctrl Pts',(2.35573909391718,-0.891753221060157,
4.82976055904438));
#20887=CARTESIAN_POINT('Ctrl Pts',(2.38393735988785,-0.813365831106525,
4.83500202617366));
#20888=CARTESIAN_POINT('Ctrl Pts',(2.40817655178341,-0.733820104276619,
4.84024349330293));
#20889=CARTESIAN_POINT('Ctrl Pts',(2.43209781731739,-0.655317716004383,
4.84541621224205));
#20890=CARTESIAN_POINT('Ctrl Pts',(2.45216318475617,-0.575687678729605,
4.85058893118116));
#20891=CARTESIAN_POINT('Ctrl Pts',(2.46828607655098,-0.495348457456518,
4.85576165012027));
#20892=CARTESIAN_POINT('Ctrl Pts',(2.48473039107651,-0.413407609613363,
4.86103749134463));
#20893=CARTESIAN_POINT('Ctrl Pts',(2.49707324762491,-0.330729506808876,
4.86631333256899));
#20894=CARTESIAN_POINT('Ctrl Pts',(2.50527825608034,-0.247764221813888,
4.87158917379334));
#20895=CARTESIAN_POINT('Ctrl Pts',(2.51348326453577,-0.1647989368189,4.8768650150177));
#20896=CARTESIAN_POINT('Ctrl Pts',(2.51755046013754,-0.0815469897731697,
4.88214085624206));
#20897=CARTESIAN_POINT('Ctrl Pts',(2.51749952702257,0.00154319187075648,
4.88741669746642));
#20898=CARTESIAN_POINT('Ctrl Pts',(2.51749952702217,0.00154319252581683,
4.88741669750801));
#20899=CARTESIAN_POINT('Ctrl Pts',(2.51744240569644,0.0947285262346869,
4.89333353407479));
#20900=CARTESIAN_POINT('Ctrl Pts',(2.51221164500483,0.187753544831829,4.89925037064158));
#20901=CARTESIAN_POINT('Ctrl Pts',(2.50185877901997,0.280194396519088,4.90516720720837));
#20902=CARTESIAN_POINT('Ctrl Pts',(2.49266337064657,0.362300296749366,4.91042253733531));
#20903=CARTESIAN_POINT('Ctrl Pts',(2.47940487600131,0.444104686115124,4.91567786746224));
#20904=CARTESIAN_POINT('Ctrl Pts',(2.46211260638418,0.525174031616275,4.92093319758918));
#20905=CARTESIAN_POINT('Ctrl Pts',(2.44484693031314,0.606118701674371,4.92618044561544));
#20906=CARTESIAN_POINT('Ctrl Pts',(2.42355990290171,0.686330126880152,4.9314276936417));
#20907=CARTESIAN_POINT('Ctrl Pts',(2.3983325070012,0.765380582364975,4.93667494166796));
#20908=CARTESIAN_POINT('Ctrl Pts',(2.3868420349923,0.801386163346109,4.93906493692579));
#20909=CARTESIAN_POINT('Ctrl Pts',(2.37453480876644,0.837150986090258,4.94145493218361));
#20910=CARTESIAN_POINT('Ctrl Pts',(2.36142200728636,0.872635292378022,4.94384492744144));
#20911=CARTESIAN_POINT('',(2.51749980506587,-0.00177349968566837,4.61406162840033));
#20912=CARTESIAN_POINT('Ctrl Pts',(2.36142200727925,0.872635292397265,4.66658913197125));
#20913=CARTESIAN_POINT('Ctrl Pts',(2.3631089532083,0.868070279640319,4.66628593237008));
#20914=CARTESIAN_POINT('Ctrl Pts',(2.36478267438196,0.86350034104399,4.6659831649262));
#20915=CARTESIAN_POINT('Ctrl Pts',(2.37558197045969,0.833746981502558,4.6640168308542));
#20916=CARTESIAN_POINT('Ctrl Pts',(2.38431862179719,0.808423479041231,4.6623660094523));
#20917=CARTESIAN_POINT('Ctrl Pts',(2.40319358021164,0.750743778121066,4.65865389320594));
#20918=CARTESIAN_POINT('Ctrl Pts',(2.41308584250394,0.718312241636577,4.65660045200013));
#20919=CARTESIAN_POINT('Ctrl Pts',(2.44376410437075,0.60993583797465,4.64983766640419));
#20920=CARTESIAN_POINT('Ctrl Pts',(2.46164346316683,0.533214366119594,4.64521179243));
#20921=CARTESIAN_POINT('Ctrl Pts',(2.50368455543998,0.304835965786213,4.63172626299532));
#20922=CARTESIAN_POINT('Ctrl Pts',(2.51760727523633,0.151684038986887,4.62306023742689));
#20923=CARTESIAN_POINT('Ctrl Pts',(2.51749937769237,-0.00177011822094938,
4.61406257126606));
#20924=CARTESIAN_POINT('Ctrl Pts',(2.51749937528208,-0.00177354288295418,
4.61406237046359));
#20925=CARTESIAN_POINT('Ctrl Pts',(2.51744798928901,-0.074714663546969,
4.6097855217469));
#20926=CARTESIAN_POINT('Ctrl Pts',(2.5142265643001,-0.147614065923254,4.60543620366339));
#20927=CARTESIAN_POINT('Ctrl Pts',(2.5067136734322,-0.233152702817736,4.60013979836202));
#20928=CARTESIAN_POINT('Ctrl Pts',(2.50548244364905,-0.24603116151992,4.59933719764383));
#20929=CARTESIAN_POINT('Ctrl Pts',(2.50330884937322,-0.267054823730848,
4.59801766304268));
#20930=CARTESIAN_POINT('Ctrl Pts',(2.50242583835527,-0.275206092752786,
4.59750376256807));
#20931=CARTESIAN_POINT('Ctrl Pts',(2.50078928885904,-0.289653925735625,
4.59658859503168));
#20932=CARTESIAN_POINT('Ctrl Pts',(2.50005174171018,-0.295952277669667,
4.59618818876115));
#20933=CARTESIAN_POINT('Ctrl Pts',(2.49858281402361,-0.308098861281167,
4.59541307615331));
#20934=CARTESIAN_POINT('Ctrl Pts',(2.49785469025906,-0.313947340020373,
4.59503855329779));
#20935=CARTESIAN_POINT('Ctrl Pts',(2.49615591669731,-0.327212212864726,
4.59418606597501));
#20936=CARTESIAN_POINT('Ctrl Pts',(2.49517276865825,-0.334626723071374,
4.59370742554324));
#20937=CARTESIAN_POINT('Ctrl Pts',(2.49240608059129,-0.354801618961238,
4.59239942839782));
#20938=CARTESIAN_POINT('Ctrl Pts',(2.49055762418982,-0.367552667451044,
4.59156661650582));
#20939=CARTESIAN_POINT('Ctrl Pts',(2.48075080098427,-0.431728584194256,
4.58734607722727));
#20940=CARTESIAN_POINT('Ctrl Pts',(2.47129775668273,-0.482908533398728,
4.58388640033651));
#20941=CARTESIAN_POINT('Ctrl Pts',(2.44745406651946,-0.592812672928028,
4.57630366372473));
#20942=CARTESIAN_POINT('Ctrl Pts',(2.43251963181112,-0.651387618516999,
4.57216618637696));
#20943=CARTESIAN_POINT('Ctrl Pts',(2.36635209388672,-0.876697742863623,
4.55599662172088));
#20944=CARTESIAN_POINT('Ctrl Pts',(2.29994927894316,-1.03849294306498,4.54387645177078));
#20945=CARTESIAN_POINT('Ctrl Pts',(2.19455542882569,-1.23452390324998,4.52903029996862));
#20946=CARTESIAN_POINT('Ctrl Pts',(2.17055167131663,-1.27625574720375,4.52585623893855));
#20947=CARTESIAN_POINT('Ctrl Pts',(2.12697109225534,-1.34723270256414,4.52043466639669));
#20948=CARTESIAN_POINT('Ctrl Pts',(2.10795123725415,-1.37680200726673,4.51816867482162));
#20949=CARTESIAN_POINT('Ctrl Pts',(2.07956736075055,-1.41896135419786,4.51492557004882));
#20950=CARTESIAN_POINT('Ctrl Pts',(2.0706959195927,-1.43187644693349,4.51393035071565));
#20951=CARTESIAN_POINT('Ctrl Pts',(2.05495444971835,-1.45434067759052,4.51219596546999));
#20952=CARTESIAN_POINT('Ctrl Pts',(2.04813706580728,-1.46392594217284,4.51145484323011));
#20953=CARTESIAN_POINT('Ctrl Pts',(2.03387025006481,-1.48369038244374,4.50992426356614));
#20954=CARTESIAN_POINT('Ctrl Pts',(2.02641097891935,-1.4938620748913,4.50913521028086));
#20955=CARTESIAN_POINT('Ctrl Pts',(2.00694517156414,-1.51999214853163,4.50710440826548));
#20956=CARTESIAN_POINT('Ctrl Pts',(1.99482448748306,-1.53586469228605,4.50586710620542));
#20957=CARTESIAN_POINT('Ctrl Pts',(1.94466273879563,-1.5999578856432,4.50085340107417));
#20958=CARTESIAN_POINT('Ctrl Pts',(1.90505029543186,-1.64692522077764,4.49713908020449));
#20959=CARTESIAN_POINT('Ctrl Pts',(1.74121030300414,-1.82735419379689,4.48261756620563));
#20960=CARTESIAN_POINT('Ctrl Pts',(1.6043719357939,-1.94859676368014,4.47232338479871));
#20961=CARTESIAN_POINT('Ctrl Pts',(1.39197377331506,-2.09911978196859,4.45726027364328));
#20962=CARTESIAN_POINT('Ctrl Pts',(1.32625146030379,-2.14124968082467,4.45269975540765));
#20963=CARTESIAN_POINT('Ctrl Pts',(1.23467467028978,-2.19411788625095,4.44633435250681));
#20964=CARTESIAN_POINT('Ctrl Pts',(1.21043869724606,-2.20758077371835,4.44464865928232));
#20965=CARTESIAN_POINT('Ctrl Pts',(1.16858530360595,-2.22993358740495,4.44172728066867));
#20966=CARTESIAN_POINT('Ctrl Pts',(1.15107620987603,-2.23902186667889,4.44050210802469));
#20967=CARTESIAN_POINT('Ctrl Pts',(1.12571314245084,-2.25181071511957,4.43872042207612));
#20968=CARTESIAN_POINT('Ctrl Pts',(1.11794350901209,-2.25567814220515,4.438173698644));
#20969=CARTESIAN_POINT('Ctrl Pts',(1.10434736264418,-2.26235828538219,4.43721509807269));
#20970=CARTESIAN_POINT('Ctrl Pts',(1.09852965225872,-2.26518889083171,4.43680431526626));
#20971=CARTESIAN_POINT('Ctrl Pts',(1.08612971779064,-2.27116307045286,4.43592738472692));
#20972=CARTESIAN_POINT('Ctrl Pts',(1.07954472926909,-2.27430047063708,4.43546088519819));
#20973=CARTESIAN_POINT('Ctrl Pts',(1.06174573697435,-2.28268603579702,4.4341979713399));
#20974=CARTESIAN_POINT('Ctrl Pts',(1.05050666751586,-2.28788008310356,4.43339839923334));
#20975=CARTESIAN_POINT('Ctrl Pts',(0.998485460932153,-2.31145714994828,
4.42968931897497));
#20976=CARTESIAN_POINT('Ctrl Pts',(0.957258736938432,-2.32883286562977,
4.42672691332104));
#20977=CARTESIAN_POINT('Ctrl Pts',(0.746502291969871,-2.41111821512607,
4.4115435181355));
#20978=CARTESIAN_POINT('Ctrl Pts',(0.570769684802599,-2.45865401231696,
4.39880315403903));
#20979=CARTESIAN_POINT('Ctrl Pts',(0.275834907844707,-2.5050788399438,4.37841181338006));
#20980=CARTESIAN_POINT('Ctrl Pts',(0.159076672967931,-2.51519504256211,
4.37057367471458));
#20981=CARTESIAN_POINT('Ctrl Pts',(0.0115384077442088,-2.51765818198488,
4.36100571210751));
#20982=CARTESIAN_POINT('Ctrl Pts',(-0.0189545506671911,-2.5176132972375,
4.35904562349324));
#20983=CARTESIAN_POINT('Ctrl Pts',(-0.0642470446742235,-2.51672364227029,
4.35615890513128));
#20984=CARTESIAN_POINT('Ctrl Pts',(-0.0790511865987438,-2.51630214789036,
4.35521927443884));
#20985=CARTESIAN_POINT('Ctrl Pts',(-0.105490832705892,-2.51531580686368,
4.35354787036417));
#20986=CARTESIAN_POINT('Ctrl Pts',(-0.117127656783522,-2.5148007959716,
4.3528145731037));
#20987=CARTESIAN_POINT('Ctrl Pts',(-0.141773591668861,-2.51353859718961,
4.35126627752719));
#20988=CARTESIAN_POINT('Ctrl Pts',(-0.154781355721146,-2.51277113421189,
4.35045193061832));
#20989=CARTESIAN_POINT('Ctrl Pts',(-0.189616500768391,-2.51044431749062,
4.34827829449673));
#20990=CARTESIAN_POINT('Ctrl Pts',(-0.211430795401036,-2.50870128829697,
4.34692472823319));
#20991=CARTESIAN_POINT('Ctrl Pts',(-0.313046573431349,-2.4992469893665,
4.34065150298943));
#20992=CARTESIAN_POINT('Ctrl Pts',(-0.392477531622812,-2.48801063872559,
4.33584201279791));
#20993=CARTESIAN_POINT('Ctrl Pts',(-0.634449916484938,-2.44190155405757,
4.3213171572279));
#20994=CARTESIAN_POINT('Ctrl Pts',(-0.794173080282035,-2.39472320081013,
4.31193143764029));
#20995=CARTESIAN_POINT('Ctrl Pts',(-1.03891968337528,-2.29522692923639,
4.29661534481884));
#20996=CARTESIAN_POINT('Ctrl Pts',(-1.12750998836885,-2.25302859825829,
4.29085029025559));
#20997=CARTESIAN_POINT('Ctrl Pts',(-1.231619824543,-2.19575751998811,4.28354315913374));
#20998=CARTESIAN_POINT('Ctrl Pts',(-1.2497101567384,-2.18551205400862,4.28225301975849));
#20999=CARTESIAN_POINT('Ctrl Pts',(-1.27541156447124,-2.17053262208112,
4.28038761485535));
#21000=CARTESIAN_POINT('Ctrl Pts',(-1.2831280082296,-2.16597992396813,4.2798233110935));
#21001=CARTESIAN_POINT('Ctrl Pts',(-1.29647556950908,-2.15800851336101,
4.27883951995507));
#21002=CARTESIAN_POINT('Ctrl Pts',(-1.3021178339861,-2.1546087328432,4.27842124599539));
#21003=CARTESIAN_POINT('Ctrl Pts',(-1.31401320986657,-2.1473773105845,4.27753421237516));
#21004=CARTESIAN_POINT('Ctrl Pts',(-1.32026283641549,-2.1435405452716,4.27706514263467));
#21005=CARTESIAN_POINT('Ctrl Pts',(-1.33716980493438,-2.13305904632379,
4.2757881079507));
#21006=CARTESIAN_POINT('Ctrl Pts',(-1.34779416642361,-2.12636188166849,
4.27497686695568));
#21007=CARTESIAN_POINT('Ctrl Pts',(-1.39766215347746,-2.09440324734153,
4.27112928987244));
#21008=CARTESIAN_POINT('Ctrl Pts',(-1.43624594734759,-2.06813476367657,
4.26803529049715));
#21009=CARTESIAN_POINT('Ctrl Pts',(-1.65439171066707,-1.91056845184088,
4.24995279725691));
#21010=CARTESIAN_POINT('Ctrl Pts',(-1.81665829245263,-1.75700089373511,
4.23424298515611));
#21011=CARTESIAN_POINT('Ctrl Pts',(-2.01256128725213,-1.51502489094334,
4.21330326755074));
#21012=CARTESIAN_POINT('Ctrl Pts',(-2.06478704277916,-1.44303878620737,
4.20744416857285));
#21013=CARTESIAN_POINT('Ctrl Pts',(-2.12491064956853,-1.35019739174296,
4.20033207579972));
#21014=CARTESIAN_POINT('Ctrl Pts',(-2.13648390135242,-1.3318088650073,4.19894382138404));
#21015=CARTESIAN_POINT('Ctrl Pts',(-2.15459736900602,-1.30218482590774,
4.19673909199813));
#21016=CARTESIAN_POINT('Ctrl Pts',(-2.16129091909579,-1.29104481590471,
4.19591706167645));
#21017=CARTESIAN_POINT('Ctrl Pts',(-2.17382289879586,-1.26981734099256,
4.19436378643572));
#21018=CARTESIAN_POINT('Ctrl Pts',(-2.17967810548655,-1.25974022664038,
4.19363195048458));
#21019=CARTESIAN_POINT('Ctrl Pts',(-2.19284359558402,-1.23671512100248,
4.19197213563917));
#21020=CARTESIAN_POINT('Ctrl Pts',(-2.20010961451792,-1.22374222133413,
4.19104575431238));
#21021=CARTESIAN_POINT('Ctrl Pts',(-2.22207121504036,-1.18370360610821,
4.18821288760459));
#21022=CARTESIAN_POINT('Ctrl Pts',(-2.23638576959146,-1.15643137619107,
4.18631980886489));
#21023=CARTESIAN_POINT('Ctrl Pts',(-2.34263351170426,-0.944651929046173,
4.17187998451683));
#21024=CARTESIAN_POINT('Ctrl Pts',(-2.41209127125278,-0.749748807333856,
4.16017838755981));
#21025=CARTESIAN_POINT('Ctrl Pts',(-2.48477485889716,-0.424187848460003,
4.14095889405291));
#21026=CARTESIAN_POINT('Ctrl Pts',(-2.50305361361178,-0.297918940740631,
4.13355452995335));
#21027=CARTESIAN_POINT('Ctrl Pts',(-2.51291935836652,-0.152862074446298,
4.12458054997968));
#21028=CARTESIAN_POINT('Ctrl Pts',(-2.51394843288695,-0.134884207099769,
4.12346010345837));
#21029=CARTESIAN_POINT('Ctrl Pts',(-2.51517717408223,-0.1084506160654,4.12179854246881));
#21030=CARTESIAN_POINT('Ctrl Pts',(-2.515527250423,-0.100002003188513,4.12126536174167));
#21031=CARTESIAN_POINT('Ctrl Pts',(-2.51607211081778,-0.0850293129558371,
4.12031645005344));
#21032=CARTESIAN_POINT('Ctrl Pts',(-2.51628409624932,-0.0785060283885452,
4.11990167289346));
#21033=CARTESIAN_POINT('Ctrl Pts',(-2.51668875814144,-0.0643591346285295,
4.11899914942007));
#21034=CARTESIAN_POINT('Ctrl Pts',(-2.51687216099032,-0.0567355720520758,
4.11851092304939));
#21035=CARTESIAN_POINT('Ctrl Pts',(-2.51728479638091,-0.0355874964734826,
4.11715159729157));
#21036=CARTESIAN_POINT('Ctrl Pts',(-2.51743966443228,-0.0220620218026809,
4.11627659424445));
#21037=CARTESIAN_POINT('Ctrl Pts',(-2.51769415614889,0.0529913523234178,
4.11139232549786));
#21038=CARTESIAN_POINT('Ctrl Pts',(-2.51564707031644,0.114500799560346,
4.10728229034464));
#21039=CARTESIAN_POINT('Ctrl Pts',(-2.49890169806237,0.353620788117591,
4.09103490019247));
#21040=CARTESIAN_POINT('Ctrl Pts',(-2.46761781469537,0.529551139057424,
4.07854247228994));
#21041=CARTESIAN_POINT('Ctrl Pts',(-2.38643388434348,0.809701166666007,
4.05872123340112));
#21042=CARTESIAN_POINT('Ctrl Pts',(-2.34751390807522,0.916442791962811,
4.0511763124758));
#21043=CARTESIAN_POINT('Ctrl Pts',(-2.29213875125551,1.04136536845466,4.04237690925929));
#21044=CARTESIAN_POINT('Ctrl Pts',(-2.28246824911139,1.06239382332507,4.04089640781739));
#21045=CARTESIAN_POINT('Ctrl Pts',(-2.26678421339043,1.09529565456573,4.0385804507244));
#21046=CARTESIAN_POINT('Ctrl Pts',(-2.26096436584289,1.10725940430399,4.037738422373));
#21047=CARTESIAN_POINT('Ctrl Pts',(-2.24988870012625,1.12957596935306,4.03616773063101));
#21048=CARTESIAN_POINT('Ctrl Pts',(-2.24465559573863,1.1399396024689,4.03543830748814));
#21049=CARTESIAN_POINT('Ctrl Pts',(-2.23277655353745,1.16306584057133,4.03381041078868));
#21050=CARTESIAN_POINT('Ctrl Pts',(-2.22609247742936,1.17580848059847,4.03291329449226));
#21051=CARTESIAN_POINT('Ctrl Pts',(-2.20880146406436,1.20809636548607,4.03063930969692));
#21052=CARTESIAN_POINT('Ctrl Pts',(-2.19804400544689,1.22755991072405,4.0292677478866));
#21053=CARTESIAN_POINT('Ctrl Pts',(-2.10692146373496,1.38738916238534,4.01799162421964));
#21054=CARTESIAN_POINT('Ctrl Pts',(-2.0134556447357,1.51985938665549,4.00859402375851));
#21055=CARTESIAN_POINT('Ctrl Pts',(-1.8270199675378,1.73642675999762,3.99215505830478));
#21056=CARTESIAN_POINT('Ctrl Pts',(-1.739299865033,1.82428406368276,3.9850882575277));
#21057=CARTESIAN_POINT('Ctrl Pts',(-1.61230661530876,1.9339580768998,3.97516577627883));
#21058=CARTESIAN_POINT('Ctrl Pts',(-1.57840182551127,1.9617272275819,3.9725423984803));
#21059=CARTESIAN_POINT('Ctrl Pts',(-1.52174235110174,2.00571325047913,3.9681678883919));
#21060=CARTESIAN_POINT('Ctrl Pts',(-1.49941092881506,2.02246190158252,3.9664460366982));
#21061=CARTESIAN_POINT('Ctrl Pts',(-1.46866008532416,2.04473592255081,3.96407113343376));
#21062=CARTESIAN_POINT('Ctrl Pts',(-1.46047829109749,2.05058786507156,3.96343888321199));
#21063=CARTESIAN_POINT('Ctrl Pts',(-1.44671806540844,2.06030559633666,3.96237454570308));
#21064=CARTESIAN_POINT('Ctrl Pts',(-1.44115857038415,2.06419821825453,3.9619442508103));
#21065=CARTESIAN_POINT('Ctrl Pts',(-1.43056191984243,2.07155405674072,3.96112343074273));
#21066=CARTESIAN_POINT('Ctrl Pts',(-1.42552776839172,2.07502149293185,3.960733208211));
#21067=CARTESIAN_POINT('Ctrl Pts',(-1.4135249184593,2.08322455445612,3.95980224961037));
#21068=CARTESIAN_POINT('Ctrl Pts',(-1.40654502839954,2.08794356189775,3.95926043531785));
#21069=CARTESIAN_POINT('Ctrl Pts',(-1.38173285553225,2.10453785443036,3.95733319561931));
#21070=CARTESIAN_POINT('Ctrl Pts',(-1.36377337835662,2.11622006549789,3.95593605920174));
#21071=CARTESIAN_POINT('Ctrl Pts',(-1.23519378924031,2.197541560704,3.94593014511059));
#21072=CARTESIAN_POINT('Ctrl Pts',(-1.11945610819381,2.25869524199001,3.93691735121521));
#21073=CARTESIAN_POINT('Ctrl Pts',(-0.869483556517382,2.36682791992753,
3.91810230171811));
#21074=CARTESIAN_POINT('Ctrl Pts',(-0.734930638955566,2.41200348908363,
3.90833609761946));
#21075=CARTESIAN_POINT('Ctrl Pts',(-0.526294355866242,2.46295759780508,
3.89400629362969));
#21076=CARTESIAN_POINT('Ctrl Pts',(-0.454581605793358,2.47719664283383,
3.88921622652109));
#21077=CARTESIAN_POINT('Ctrl Pts',(-0.362109163229426,2.49140569627182,
3.8832088763224));
#21078=CARTESIAN_POINT('Ctrl Pts',(-0.34183611138683,2.49426812971329,3.88190205532801));
#21079=CARTESIAN_POINT('Ctrl Pts',(-0.308911488984472,2.49850791603864,
3.87979569662749));
#21080=CARTESIAN_POINT('Ctrl Pts',(-0.296280761104125,2.50003716667972,
3.87899144427039));
#21081=CARTESIAN_POINT('Ctrl Pts',(-0.271989715869779,2.50279149953608,
3.87745184010376));
#21082=CARTESIAN_POINT('Ctrl Pts',(-0.260331400269903,2.50403100323958,
3.87671605703081));
#21083=CARTESIAN_POINT('Ctrl Pts',(-0.233589418796562,2.5066854083391,3.87503529557393));
#21084=CARTESIAN_POINT('Ctrl Pts',(-0.218500694778285,2.50804569637984,
3.87409204012157));
#21085=CARTESIAN_POINT('Ctrl Pts',(-0.170328953041776,2.51195047747566,
3.87109613906079));
#21086=CARTESIAN_POINT('Ctrl Pts',(-0.137206689401077,2.51397725426197,
3.86905954150488));
#21087=CARTESIAN_POINT('Ctrl Pts',(0.0630887435892422,2.52226290574743,
3.85686716284664));
#21088=CARTESIAN_POINT('Ctrl Pts',(0.2305083175267,2.51250165583614,3.84723060401108));
#21089=CARTESIAN_POINT('Ctrl Pts',(0.512861728766748,2.467558454867,3.83080257427056));
#21090=CARTESIAN_POINT('Ctrl Pts',(0.628513786338901,2.44066349071575,3.82400895071012));
#21091=CARTESIAN_POINT('Ctrl Pts',(0.775688520157098,2.39528055834854,3.81482386695236));
#21092=CARTESIAN_POINT('Ctrl Pts',(0.809320913102423,2.38412689409412,3.81268654724171));
#21093=CARTESIAN_POINT('Ctrl Pts',(0.865219012911848,2.36427010979438,3.80905237504293));
#21094=CARTESIAN_POINT('Ctrl Pts',(0.887617057871395,2.35595266394936,3.80757377048634));
#21095=CARTESIAN_POINT('Ctrl Pts',(0.91872139354652,2.34389567074444,3.80548448993186));
#21096=CARTESIAN_POINT('Ctrl Pts',(0.927530862207434,2.34042355294591,3.80488869226996));
#21097=CARTESIAN_POINT('Ctrl Pts',(0.942513635927006,2.3344204441844,3.80386809933771));
#21098=CARTESIAN_POINT('Ctrl Pts',(0.948696961229068,2.33191441501032,3.80344477605443));
#21099=CARTESIAN_POINT('Ctrl Pts',(0.96145908796655,2.32668291352529,3.80256651621827));
#21100=CARTESIAN_POINT('Ctrl Pts',(0.968036349294273,2.3239540833154,3.80211139472084));
#21101=CARTESIAN_POINT('Ctrl Pts',(0.985295243741117,2.31670758622374,3.8009107575322));
#21102=CARTESIAN_POINT('Ctrl Pts',(0.995957244739025,2.31214400757547,3.80016258477397));
#21103=CARTESIAN_POINT('Ctrl Pts',(1.04063556883363,2.29265430568783,3.79700135697263));
#21104=CARTESIAN_POINT('Ctrl Pts',(1.07434910270687,2.27705068431263,3.7945521714047));
#21105=CARTESIAN_POINT('Ctrl Pts',(1.27957306220259,2.17649493439499,3.7793003101533));
#21106=CARTESIAN_POINT('Ctrl Pts',(1.441275236585,2.07296008206912,3.76584384774829));
#21107=CARTESIAN_POINT('Ctrl Pts',(1.65548889862967,1.89851641530261,3.74698032153053));
#21108=CARTESIAN_POINT('Ctrl Pts',(1.7185463933416,1.84163207473074,3.74126397762998));
#21109=CARTESIAN_POINT('Ctrl Pts',(1.803819558469,1.75650494009893,3.73331900902989));
#21110=CARTESIAN_POINT('Ctrl Pts',(1.82848821148946,1.73081069762476,3.73099224160633));
#21111=CARTESIAN_POINT('Ctrl Pts',(1.87145654006031,1.68411159679977,3.72688710466982));
#21112=CARTESIAN_POINT('Ctrl Pts',(1.88996806643035,1.6633106328245,3.72510015771468));
#21113=CARTESIAN_POINT('Ctrl Pts',(1.9174515598588,1.63137669145542,3.72241783447421));
#21114=CARTESIAN_POINT('Ctrl Pts',(1.92667957399474,1.62046790362634,3.72151199976722));
#21115=CARTESIAN_POINT('Ctrl Pts',(1.94323225018751,1.60055905765305,3.71987741231498));
#21116=CARTESIAN_POINT('Ctrl Pts',(1.95058845549773,1.59158586314099,3.7191473960898));
#21117=CARTESIAN_POINT('Ctrl Pts',(1.96629256355762,1.5721573683499,3.7175809868224));
#21118=CARTESIAN_POINT('Ctrl Pts',(1.97461971784119,1.56168569732838,3.71674543498294));
#21119=CARTESIAN_POINT('Ctrl Pts',(1.99695978580558,1.53312794677522,3.7144898531122));
#21120=CARTESIAN_POINT('Ctrl Pts',(2.01081048229548,1.51491615101593,3.71307619427292));
#21121=CARTESIAN_POINT('Ctrl Pts',(2.08288641489722,1.41741556958778,3.7056331651904));
#21122=CARTESIAN_POINT('Ctrl Pts',(2.13667886061936,1.33494920078824,3.69977497513817));
#21123=CARTESIAN_POINT('Ctrl Pts',(2.254471578004,1.1289232096223,3.6858968307041));
#21124=CARTESIAN_POINT('Ctrl Pts',(2.31330030136958,1.0028565208644,3.67801546162231));
#21125=CARTESIAN_POINT('Ctrl Pts',(2.36142196837104,0.872635397686014,3.66998323165053));
#21126=CARTESIAN_POINT('Origin',(0.,0.,10.));
#21127=CARTESIAN_POINT('',(2.36142200370902,0.872635302058581,2.66999896006316));
#21128=CARTESIAN_POINT('',(2.36142200728636,0.872635292378021,2.94373350505074));
#21129=CARTESIAN_POINT('',(2.36142200728636,0.87263529237802,10.));
#21130=CARTESIAN_POINT('',(2.51749981257981,0.000971421949232871,3.88741669755218));
#21131=CARTESIAN_POINT('Ctrl Pts',(2.36142200728636,0.872635292378019,2.94373350505074));
#21132=CARTESIAN_POINT('Ctrl Pts',(2.33289170715608,0.949840602764351,2.94891972478529));
#21133=CARTESIAN_POINT('Ctrl Pts',(2.30058211384146,1.02561533123368,2.95410594451983));
#21134=CARTESIAN_POINT('Ctrl Pts',(2.2646748419411,1.09956996606812,2.95929216425438));
#21135=CARTESIAN_POINT('Ctrl Pts',(2.22875114002844,1.17355844016397,2.9644807570362));
#21136=CARTESIAN_POINT('Ctrl Pts',(2.18922670931926,1.24572474801263,2.96966934981803));
#21137=CARTESIAN_POINT('Ctrl Pts',(2.14632862703392,1.31570501054556,2.97485794259986));
#21138=CARTESIAN_POINT('Ctrl Pts',(2.10335434119307,1.38580958504156,2.9800557523256));
#21139=CARTESIAN_POINT('Ctrl Pts',(2.05699469910031,1.4537199663387,2.98525356205133));
#21140=CARTESIAN_POINT('Ctrl Pts',(2.00751934661653,1.5191024728307,2.99045137177706));
#21141=CARTESIAN_POINT('Ctrl Pts',(1.9621829145152,1.57901532675449,2.99521435245079));
#21142=CARTESIAN_POINT('Ctrl Pts',(1.91423093465632,1.63680574266011,2.99997733312453));
#21143=CARTESIAN_POINT('Ctrl Pts',(1.86389785875587,1.69224437423361,3.00474031379826));
#21144=CARTESIAN_POINT('Ctrl Pts',(1.80836270459021,1.7534127589605,3.00999556317994));
#21145=CARTESIAN_POINT('Ctrl Pts',(1.7497107152114,1.81195742573655,3.01525081256161));
#21146=CARTESIAN_POINT('Ctrl Pts',(1.68821951959702,1.86754413700229,3.02050606194329));
#21147=CARTESIAN_POINT('Ctrl Pts',(1.62681550452739,1.92305203894059,3.02575386057532));
#21148=CARTESIAN_POINT('Ctrl Pts',(1.56258061817866,1.975610008454,3.03100165920735));
#21149=CARTESIAN_POINT('Ctrl Pts',(1.49583108670036,2.02491866751749,3.03624945783939));
#21150=CARTESIAN_POINT('Ctrl Pts',(1.42859789691412,2.074584610626,3.04153528132868));
#21151=CARTESIAN_POINT('Ctrl Pts',(1.35881378520359,2.12095360559161,3.04682110481797));
#21152=CARTESIAN_POINT('Ctrl Pts',(1.28683794502615,2.16375931037648,3.05210692830727));
#21153=CARTESIAN_POINT('Ctrl Pts',(1.21550750766473,2.20618117910827,3.05734535415095));
#21154=CARTESIAN_POINT('Ctrl Pts',(1.14202489448295,2.2451031651063,3.06258377999464));
#21155=CARTESIAN_POINT('Ctrl Pts',(1.06676946087999,2.28030900698432,3.06782220583833));
#21156=CARTESIAN_POINT('Ctrl Pts',(0.991538777532885,2.31550327024865,3.0730589088512));
#21157=CARTESIAN_POINT('Ctrl Pts',(0.914536849353382,2.34698362133617,3.07829561186407));
#21158=CARTESIAN_POINT('Ctrl Pts',(0.836166348986227,2.37458040226543,3.08353231487695));
#21159=CARTESIAN_POINT('Ctrl Pts',(0.757797983387795,2.40217643147376,3.08876887524495));
#21160=CARTESIAN_POINT('Ctrl Pts',(0.678061555290332,2.42588894856972,3.09400543561296));
#21161=CARTESIAN_POINT('Ctrl Pts',(0.597377056140069,2.44559745313848,3.09924199598096));
#21162=CARTESIAN_POINT('Ctrl Pts',(0.515371968391089,2.46562853300615,3.10456426478108));
#21163=CARTESIAN_POINT('Ctrl Pts',(0.432387969400019,2.48152321851334,3.10988653358121));
#21164=CARTESIAN_POINT('Ctrl Pts',(0.348877289275957,2.49320895374364,3.11520880238133));
#21165=CARTESIAN_POINT('Ctrl Pts',(0.266593442934255,2.50472301686289,3.12045288310835));
#21166=CARTESIAN_POINT('Ctrl Pts',(0.183798759045822,2.5121509933318,3.12569696383536));
#21167=CARTESIAN_POINT('Ctrl Pts',(0.100929636214124,2.51547599045065,3.13094104456238));
#21168=CARTESIAN_POINT('Ctrl Pts',(0.0162071731961466,2.51887535001681,
3.13630240739905));
#21169=CARTESIAN_POINT('Ctrl Pts',(-0.0685925865370805,2.5179859975086,
3.14166377023573));
#21170=CARTESIAN_POINT('Ctrl Pts',(-0.153006787453389,2.51284603049872,
3.14702513307241));
#21171=CARTESIAN_POINT('Ctrl Pts',(-0.237420988369697,2.50770606348885,
3.15238649590908));
#21172=CARTESIAN_POINT('Ctrl Pts',(-0.321449132924398,2.49831560479349,
3.15774785874576));
#21173=CARTESIAN_POINT('Ctrl Pts',(-0.404639426819381,2.48476823552284,
3.16310922158244));
#21174=CARTESIAN_POINT('Ctrl Pts',(-0.486183197008939,2.47148899927115,
3.16836447094613));
#21175=CARTESIAN_POINT('Ctrl Pts',(-0.567223178648792,2.45416689838971,
3.17361972030981));
#21176=CARTESIAN_POINT('Ctrl Pts',(-0.647327860324917,2.43285282975505,
3.1788749696735));
#21177=CARTESIAN_POINT('Ctrl Pts',(-0.727318971746132,2.41156897963144,
3.18412276828653));
#21178=CARTESIAN_POINT('Ctrl Pts',(-0.806376974925999,2.38630452123467,
3.18937056689956));
#21179=CARTESIAN_POINT('Ctrl Pts',(-0.8840785840676,2.35716170577944,3.19461836551259));
#21180=CARTESIAN_POINT('Ctrl Pts',(-0.962343209180321,2.32780772519228,
3.19990418900651));
#21181=CARTESIAN_POINT('Ctrl Pts',(-1.03923123307102,2.29451902239971,3.20519001250043));
#21182=CARTESIAN_POINT('Ctrl Pts',(-1.11432368664947,2.25745187575991,3.21047583599435));
#21183=CARTESIAN_POINT('Ctrl Pts',(-1.18874279056827,2.22071710806612,3.21571426181672));
#21184=CARTESIAN_POINT('Ctrl Pts',(-1.26139797536918,2.1802715953004,3.22095268763908));
#21185=CARTESIAN_POINT('Ctrl Pts',(-1.3319013020307,2.13631579398948,3.22619111346145));
#21186=CARTESIAN_POINT('Ctrl Pts',(-1.40238144131381,2.09237444901484,3.23142781645218));
#21187=CARTESIAN_POINT('Ctrl Pts',(-1.47071073676316,2.04492535227277,3.23666451944291));
#21188=CARTESIAN_POINT('Ctrl Pts',(-1.53652764482227,1.99421389191253,3.24190122243364));
#21189=CARTESIAN_POINT('Ctrl Pts',(-1.60234276005534,1.94350381291203,3.24713778277869));
#21190=CARTESIAN_POINT('Ctrl Pts',(-1.66564525908662,1.88953182942044,3.25237434312373));
#21191=CARTESIAN_POINT('Ctrl Pts',(-1.7261054020982,1.83258462037839,3.25761090346878));
#21192=CARTESIAN_POINT('Ctrl Pts',(-1.78755511585904,1.77470533791553,3.2629331722936));
#21193=CARTESIAN_POINT('Ctrl Pts',(-1.84606822367696,1.71375288583823,3.26825544111842));
#21194=CARTESIAN_POINT('Ctrl Pts',(-1.90133764881034,1.65006708809562,3.27357770994324));
#21195=CARTESIAN_POINT('Ctrl Pts',(-1.95579512461805,1.58731688250739,3.27882179064555));
#21196=CARTESIAN_POINT('Ctrl Pts',(-2.00710334879779,1.52191351407604,3.28406587134786));
#21197=CARTESIAN_POINT('Ctrl Pts',(-2.05501055398101,1.45421383332255,3.28930995205017));
#21198=CARTESIAN_POINT('Ctrl Pts',(-2.10398918845009,1.38500007091213,3.29467131493624));
#21199=CARTESIAN_POINT('Ctrl Pts',(-2.14941256856701,1.31338647656395,3.30003267782232));
#21200=CARTESIAN_POINT('Ctrl Pts',(-2.19106064785408,1.23978203222392,3.30539404070839));
#21201=CARTESIAN_POINT('Ctrl Pts',(-2.23270872714114,1.16617758788389,3.31075540359447));
#21202=CARTESIAN_POINT('Ctrl Pts',(-2.27058133772659,1.09058277775616,3.31611676648054));
#21203=CARTESIAN_POINT('Ctrl Pts',(-2.30451099460484,1.01342751380915,3.32147812936661));
#21204=CARTESIAN_POINT('Ctrl Pts',(-2.33776910715393,0.937799326311952,
3.32673337880581));
#21205=CARTESIAN_POINT('Ctrl Pts',(-2.36736180743918,0.860392568794018,
3.331988628245));
#21206=CARTESIAN_POINT('Ctrl Pts',(-2.39309685031164,0.781596900600643,
3.3372438776842));
#21207=CARTESIAN_POINT('Ctrl Pts',(-2.41879540674197,0.702912946757253,
3.34249167637402));
#21208=CARTESIAN_POINT('Ctrl Pts',(-2.44064702728877,0.622844428524487,
3.34773947506385));
#21209=CARTESIAN_POINT('Ctrl Pts',(-2.45850702087654,0.541802065611387,
3.35298727375368));
#21210=CARTESIAN_POINT('Ctrl Pts',(-2.47649642537684,0.460172481539068,
3.35827309722856));
#21211=CARTESIAN_POINT('Ctrl Pts',(-2.490435922581,0.37755531436034,3.36355892070344));
#21212=CARTESIAN_POINT('Ctrl Pts',(-2.50022848920796,0.294387078101105,
3.36884474417831));
#21213=CARTESIAN_POINT('Ctrl Pts',(-2.5099332466421,0.211964605028515,3.37408317008008));
#21214=CARTESIAN_POINT('Ctrl Pts',(-2.51556509109816,0.129001372780505,
3.37932159598185));
#21215=CARTESIAN_POINT('Ctrl Pts',(-2.51708094996556,0.0459319204960778,
3.38456002188362));
#21216=CARTESIAN_POINT('Ctrl Pts',(-2.51859631029229,-0.037110211632046,
3.38979672495455));
#21217=CARTESIAN_POINT('Ctrl Pts',(-2.51599836509906,-0.12025803343577,
3.39503342802547));
#21218=CARTESIAN_POINT('Ctrl Pts',(-2.50929610112586,-0.203074682997528,
3.4002701310964));
#21219=CARTESIAN_POINT('Ctrl Pts',(-2.50259401971873,-0.28588907667826,
3.40550669152235));
#21220=CARTESIAN_POINT('Ctrl Pts',(-2.49178788006596,-0.368371856219138,
3.4107432519483));
#21221=CARTESIAN_POINT('Ctrl Pts',(-2.47693861889985,-0.450090355598209,
3.41597981237425));
#21222=CARTESIAN_POINT('Ctrl Pts',(-2.46184631556332,-0.533146365391441,
3.42130208110562));
#21223=CARTESIAN_POINT('Ctrl Pts',(-2.44257742174296,-0.615412364763316,
3.426624349837));
#21224=CARTESIAN_POINT('Ctrl Pts',(-2.41924979072903,-0.696445762466485,
3.43194661856838));
#21225=CARTESIAN_POINT('Ctrl Pts',(-2.39626485935617,-0.776288721402427,
3.43719069935248));
#21226=CARTESIAN_POINT('Ctrl Pts',(-2.36933986039222,-0.854934630968459,
3.44243478013658));
#21227=CARTESIAN_POINT('Ctrl Pts',(-2.33863704216953,-0.931978022805563,
3.44767886092068));
#21228=CARTESIAN_POINT('Ctrl Pts',(-2.30724756680958,-1.01074446151412,
3.4530402236257));
#21229=CARTESIAN_POINT('Ctrl Pts',(-2.27190946744169,-1.08783537264659,
3.45840158633072));
#21230=CARTESIAN_POINT('Ctrl Pts',(-2.23284599028985,-1.16284351210579,
3.46376294903574));
#21231=CARTESIAN_POINT('Ctrl Pts',(-2.19378251313801,-1.23785165156499,
3.46912431174075));
#21232=CARTESIAN_POINT('Ctrl Pts',(-2.15099397295079,-1.31077661491582,
3.47448567444577));
#21233=CARTESIAN_POINT('Ctrl Pts',(-2.10474978906033,-1.38124385082812,
3.47984703715079));
#21234=CARTESIAN_POINT('Ctrl Pts',(-2.05942088052246,-1.45031638326054,
3.48510228655188));
#21235=CARTESIAN_POINT('Ctrl Pts',(-2.01060448178666,-1.51728274144073,
3.49035753595296));
#21236=CARTESIAN_POINT('Ctrl Pts',(-1.95852276792631,-1.5817695209841,3.49561278535405));
#21237=CARTESIAN_POINT('Ctrl Pts',(-1.90651489410496,-1.64616487292335,
3.5008605840053));
#21238=CARTESIAN_POINT('Ctrl Pts',(-1.85125118814415,-1.7080872730199,3.50610838265656));
#21239=CARTESIAN_POINT('Ctrl Pts',(-1.79299738127787,-1.76719173853057,
3.51135618130781));
#21240=CARTESIAN_POINT('Ctrl Pts',(-1.73432147527304,-1.82672446693629,
3.51664200479228));
#21241=CARTESIAN_POINT('Ctrl Pts',(-1.67261221380116,-1.88339785551484,
3.52192782827674));
#21242=CARTESIAN_POINT('Ctrl Pts',(-1.60818291698439,-1.93689286113599,
3.5272136517612));
#21243=CARTESIAN_POINT('Ctrl Pts',(-1.54433135331982,-1.98990818065546,
3.53245207762355));
#21244=CARTESIAN_POINT('Ctrl Pts',(-1.47780870122699,-2.03980158942313,
3.53769050348591));
#21245=CARTESIAN_POINT('Ctrl Pts',(-1.40895599782697,-2.08630037295386,
3.54292892934826));
#21246=CARTESIAN_POINT('Ctrl Pts',(-1.34012593893504,-2.13278386380866,
3.54816563237953));
#21247=CARTESIAN_POINT('Ctrl Pts',(-1.26896773276627,-2.17587468869197,
3.55340233541081));
#21248=CARTESIAN_POINT('Ctrl Pts',(-1.19585270856544,-2.21534253545963,
3.55863903844209));
#21249=CARTESIAN_POINT('Ctrl Pts',(-1.12273967598102,-2.25480930714303,
3.56387559882821));
#21250=CARTESIAN_POINT('Ctrl Pts',(-1.04767033787355,-2.2906530786532,3.56911215921434));
#21251=CARTESIAN_POINT('Ctrl Pts',(-0.971040788257617,-2.32268939756051,
3.57434871960047));
#21252=CARTESIAN_POINT('Ctrl Pts',(-0.893157019273675,-2.35525006473628,
3.57967098837834));
#21253=CARTESIAN_POINT('Ctrl Pts',(-0.813661953682703,-2.38387731755965,
3.58499325715621));
#21254=CARTESIAN_POINT('Ctrl Pts',(-0.732990999032035,-2.40842904095969,
3.59031552593409));
#21255=CARTESIAN_POINT('Ctrl Pts',(-0.653505159898557,-2.43262008152783,
3.59555960667833));
#21256=CARTESIAN_POINT('Ctrl Pts',(-0.572878220599952,-2.45285448845586,
3.60080368742257));
#21257=CARTESIAN_POINT('Ctrl Pts',(-0.491538621220228,-2.46904759651346,
3.60604776816682));
#21258=CARTESIAN_POINT('Ctrl Pts',(-0.408379889858549,-2.48560285782704,
3.61140913096151));
#21259=CARTESIAN_POINT('Ctrl Pts',(-0.324476743563918,-2.49793380003589,
3.6167704937562));
#21260=CARTESIAN_POINT('Ctrl Pts',(-0.240292322326436,-2.5060059556655,
3.62213185655089));
#21261=CARTESIAN_POINT('Ctrl Pts',(-0.156107901088954,-2.51407811129511,
3.62749321934558));
#21262=CARTESIAN_POINT('Ctrl Pts',(-0.0716427155110961,-2.51789152415883,
3.63285458214027));
#21263=CARTESIAN_POINT('Ctrl Pts',(0.0126423778376351,-2.51746825606255,
3.63821594493496));
#21264=CARTESIAN_POINT('Ctrl Pts',(0.0952592801793968,-2.51705336539107,
3.64347119433707));
#21265=CARTESIAN_POINT('Ctrl Pts',(0.178008309290671,-2.51256648498689,
3.64872644373918));
#21266=CARTESIAN_POINT('Ctrl Pts',(0.260455292888836,-2.50399067298706,
3.65398169314129));
#21267=CARTESIAN_POINT('Ctrl Pts',(0.342785385391971,-2.49542701954066,
3.65922949179347));
#21268=CARTESIAN_POINT('Ctrl Pts',(0.424813827859746,-2.48278599672192,
3.66447729044565));
#21269=CARTESIAN_POINT('Ctrl Pts',(0.506106573643376,-2.46610267144638,
3.66972508909783));
#21270=CARTESIAN_POINT('Ctrl Pts',(0.587988355556145,-2.44929846107529,
3.67501091258205));
#21271=CARTESIAN_POINT('Ctrl Pts',(0.669123260401729,-2.42839312350843,
3.68029673606627));
#21272=CARTESIAN_POINT('Ctrl Pts',(0.749073089634344,-2.40347576571632,
3.68558255955049));
#21273=CARTESIAN_POINT('Ctrl Pts',(0.828306014163418,-2.37878184018383,
3.69082098541355));
#21274=CARTESIAN_POINT('Ctrl Pts',(0.906374582304272,-2.35014769710119,
3.69605941127661));
#21275=CARTESIAN_POINT('Ctrl Pts',(0.982864365057567,-2.31771091594702,
3.70129783713967));
#21276=CARTESIAN_POINT('Ctrl Pts',(1.05932899159329,-2.28528480271077,3.70653454017157));
#21277=CARTESIAN_POINT('Ctrl Pts',(1.13421543950595,-2.2490587152142,3.71177124320348));
#21278=CARTESIAN_POINT('Ctrl Pts',(1.20712835395856,-2.20921872775633,3.71700794623539));
#21279=CARTESIAN_POINT('Ctrl Pts',(1.28003928229874,-2.1693798255204,3.72224450662204));
#21280=CARTESIAN_POINT('Ctrl Pts',(1.35097637964091,-2.12592744120263,3.72748106700869));
#21281=CARTESIAN_POINT('Ctrl Pts',(1.41956927470519,-2.0790933899931,3.73271762739535));
#21282=CARTESIAN_POINT('Ctrl Pts',(1.48928485072602,-2.0314927914996,3.73803989617233));
#21283=CARTESIAN_POINT('Ctrl Pts',(1.5565783820882,-1.98039909625843,3.74336216494931));
#21284=CARTESIAN_POINT('Ctrl Pts',(1.62109360544763,-1.92610014598847,3.7486844337263));
#21285=CARTESIAN_POINT('Ctrl Pts',(1.68466105285133,-1.8725988871285,3.75392851447084));
#21286=CARTESIAN_POINT('Ctrl Pts',(1.74553098024876,-1.8159862868895,3.75917259521539));
#21287=CARTESIAN_POINT('Ctrl Pts',(1.80339910622492,-1.75657562139156,3.76441667595993));
#21288=CARTESIAN_POINT('Ctrl Pts',(1.8625614327859,-1.69583625694693,3.76977803875313));
#21289=CARTESIAN_POINT('Ctrl Pts',(1.91858573094579,-1.6321725458682,3.77513940154633));
#21290=CARTESIAN_POINT('Ctrl Pts',(1.971190932362,-1.5659542005352,3.78050076433954));
#21291=CARTESIAN_POINT('Ctrl Pts',(2.02379613377821,-1.49973585520219,3.78586212713274));
#21292=CARTESIAN_POINT('Ctrl Pts',(2.07298199720273,-1.43096332775857,3.79122348992594));
#21293=CARTESIAN_POINT('Ctrl Pts',(2.11851611382906,-1.36003519272356,3.79658485271914));
#21294=CARTESIAN_POINT('Ctrl Pts',(2.16415197869778,-1.28894856525233,3.80195819574346));
#21295=CARTESIAN_POINT('Ctrl Pts',(2.2062826727302,-1.21544362331868,3.80733153876778));
#21296=CARTESIAN_POINT('Ctrl Pts',(2.24465002146114,-1.1398914558652,3.81270488179211));
#21297=CARTESIAN_POINT('Ctrl Pts',(2.28295541767622,-1.06446128398889,3.81806954837331));
#21298=CARTESIAN_POINT('Ctrl Pts',(2.31750935406228,-0.986990841663087,
3.82343421495451));
#21299=CARTESIAN_POINT('Ctrl Pts',(2.34809743283373,-0.907879229809594,
3.82879888153571));
#21300=CARTESIAN_POINT('Ctrl Pts',(2.37863368176286,-0.828901668296364,
3.83415445798003));
#21301=CARTESIAN_POINT('Ctrl Pts',(2.40521729350954,-0.748288874715507,
3.83951003442434));
#21302=CARTESIAN_POINT('Ctrl Pts',(2.42768086926413,-0.666462187231165,
3.84486561086866));
#21303=CARTESIAN_POINT('Ctrl Pts',(2.45012200391775,-0.584717244566827,
3.85021583709479));
#21304=CARTESIAN_POINT('Ctrl Pts',(2.46845116965856,-0.501761234880452,
3.85556606332091));
#21305=CARTESIAN_POINT('Ctrl Pts',(2.4825500989695,-0.418032601726885,3.86091628954703));
#21306=CARTESIAN_POINT('Ctrl Pts',(2.49663704247012,-0.334375148128312,
3.86626196742801));
#21307=CARTESIAN_POINT('Ctrl Pts',(2.50650083257717,-0.249946804510473,
3.87160764530899));
#21308=CARTESIAN_POINT('Ctrl Pts',(2.51207407902142,-0.165197068704897,
3.87695332318996));
#21309=CARTESIAN_POINT('Ctrl Pts',(2.51571034773615,-0.109902041654824,
3.88044111462931));
#21310=CARTESIAN_POINT('Ctrl Pts',(2.51752120578827,-0.0544704354779488,
3.88392890606866));
#21311=CARTESIAN_POINT('Ctrl Pts',(2.51749981258008,0.000971421247064627,
3.88741669750801));
#21312=CARTESIAN_POINT('Ctrl Pts',(2.51749981257981,0.000971421949234606,
3.88741669755219));
#21313=CARTESIAN_POINT('Ctrl Pts',(2.51746490758839,0.0914298570691506,
3.89310734671633));
#21314=CARTESIAN_POINT('Ctrl Pts',(2.51255029559255,0.181738119631553,3.89879799588047));
#21315=CARTESIAN_POINT('Ctrl Pts',(2.50282942875531,0.271387362558304,3.90448864504461));
#21316=CARTESIAN_POINT('Ctrl Pts',(2.49308230922834,0.361278716996203,3.9101946626784));
#21317=CARTESIAN_POINT('Ctrl Pts',(2.47850306200983,0.450507179086973,3.91590068031219));
#21318=CARTESIAN_POINT('Ctrl Pts',(2.4592160192085,0.538574805266912,3.92160669794598));
#21319=CARTESIAN_POINT('Ctrl Pts',(2.43985725342605,0.626969929692968,3.92733393462299));
#21320=CARTESIAN_POINT('Ctrl Pts',(2.41575575171988,0.714195269642512,3.93306117130002));
#21321=CARTESIAN_POINT('Ctrl Pts',(2.38708587495822,0.799767013307601,3.93878840797704));
#21322=CARTESIAN_POINT('Ctrl Pts',(2.37890164914636,0.824194689753225,3.94042332948829));
#21323=CARTESIAN_POINT('Ctrl Pts',(2.37034544207401,0.84848775276759,3.94205825099955));
#21324=CARTESIAN_POINT('Ctrl Pts',(2.36142200728636,0.872635292378021,3.9436931725108));
#21325=CARTESIAN_POINT('Ctrl Pts',(2.36142196837104,0.872635397686016,3.66998323165053));
#21326=CARTESIAN_POINT('Ctrl Pts',(2.37171308987963,0.844786790496797,3.66826548869242));
#21327=CARTESIAN_POINT('Ctrl Pts',(2.38151450564319,0.816748213276368,3.66654020096058));
#21328=CARTESIAN_POINT('Ctrl Pts',(2.40889173926343,0.733740777454115,3.66142820138484));
#21329=CARTESIAN_POINT('Ctrl Pts',(2.42507293816446,0.678347504930899,3.65801142973578));
#21330=CARTESIAN_POINT('Ctrl Pts',(2.44497829488643,0.600340006610761,3.6531315422438));
#21331=CARTESIAN_POINT('Ctrl Pts',(2.45031934433564,0.578153977253145,3.65173604938153));
#21332=CARTESIAN_POINT('Ctrl Pts',(2.45913364056118,0.53922200803024,3.64926911247199));
#21333=CARTESIAN_POINT('Ctrl Pts',(2.46273927628498,0.52250727853566,3.64820417505802));
#21334=CARTESIAN_POINT('Ctrl Pts',(2.46783795430178,0.497645116948153,3.64660980248966));
#21335=CARTESIAN_POINT('Ctrl Pts',(2.46946158761549,0.489524558937571,3.64608741239728));
#21336=CARTESIAN_POINT('Ctrl Pts',(2.47217146575597,0.475614540417378,3.64518957261515));
#21337=CARTESIAN_POINT('Ctrl Pts',(2.47327750259242,0.469829055492997,3.64481524299538));
#21338=CARTESIAN_POINT('Ctrl Pts',(2.47574547546959,0.456669271492089,3.64396169082849));
#21339=CARTESIAN_POINT('Ctrl Pts',(2.47709474700074,0.449292881899078,3.64348178144294));
#21340=CARTESIAN_POINT('Ctrl Pts',(2.48068753908381,0.429143074010089,3.64216702075899));
#21341=CARTESIAN_POINT('Ctrl Pts',(2.48286530638019,0.416358376843797,3.64132865654332));
#21342=CARTESIAN_POINT('Ctrl Pts',(2.49346449598788,0.351092887361307,3.63702953903928));
#21343=CARTESIAN_POINT('Ctrl Pts',(2.50032050644018,0.298375384728944,3.63349369227555));
#21344=CARTESIAN_POINT('Ctrl Pts',(2.50839807836804,0.215932938583925,3.62790463997628));
#21345=CARTESIAN_POINT('Ctrl Pts',(2.51077038227164,0.186332871078375,3.62588602703367));
#21346=CARTESIAN_POINT('Ctrl Pts',(2.51582836012262,0.105229638886954,3.62033318810098));
#21347=CARTESIAN_POINT('Ctrl Pts',(2.51745592389102,0.053675300667166,3.61677955282314));
#21348=CARTESIAN_POINT('Ctrl Pts',(2.51767273534475,-0.205168317705718,
3.5989066387134));
#21349=CARTESIAN_POINT('Ctrl Pts',(2.49224625113157,-0.411717004261668,
3.58463819453919));
#21350=CARTESIAN_POINT('Ctrl Pts',(2.4343054571848,-0.6425756439213,3.56920234207048));
#21351=CARTESIAN_POINT('Ctrl Pts',(2.4262979681964,-0.67217915923025,3.56723083786128));
#21352=CARTESIAN_POINT('Ctrl Pts',(2.41361454144976,-0.715885055189095,
3.56433071215611));
#21353=CARTESIAN_POINT('Ctrl Pts',(2.40935169984168,-0.730103395954272,
3.56338891325753));
#21354=CARTESIAN_POINT('Ctrl Pts',(2.40151856909678,-0.755414171939983,
3.56171510177294));
#21355=CARTESIAN_POINT('Ctrl Pts',(2.39799657891024,-0.76652098717923,3.56098154858628));
#21356=CARTESIAN_POINT('Ctrl Pts',(2.39037887645708,-0.789977436969182,
3.55943419123705));
#21357=CARTESIAN_POINT('Ctrl Pts',(2.38626427071203,-0.802320611951452,
3.55862102752818));
#21358=CARTESIAN_POINT('Ctrl Pts',(2.375002138915,-0.835252074218305,3.55645406357455));
#21359=CARTESIAN_POINT('Ctrl Pts',(2.3676825553437,-0.85578066727183,3.55510592383193));
#21360=CARTESIAN_POINT('Ctrl Pts',(2.32882949577893,-0.960432259289628,
3.54824336988238));
#21361=CARTESIAN_POINT('Ctrl Pts',(2.29307425674893,-1.04292375489012,3.54287068636599));
#21362=CARTESIAN_POINT('Ctrl Pts',(2.14978889206595,-1.33029976436524,3.52401132456284));
#21363=CARTESIAN_POINT('Ctrl Pts',(2.01858682484259,-1.52202912021574,3.51124533961636));
#21364=CARTESIAN_POINT('Ctrl Pts',(1.83727275460247,-1.7215423723066,3.49498375102671));
#21365=CARTESIAN_POINT('Ctrl Pts',(1.81081543102841,-1.74935028689683,3.49263580341399));
#21366=CARTESIAN_POINT('Ctrl Pts',(1.77545113924399,-1.78485777812619,3.48951188901158));
#21367=CARTESIAN_POINT('Ctrl Pts',(1.76710986829707,-1.79311648723545,3.48877607258802));
#21368=CARTESIAN_POINT('Ctrl Pts',(1.75359392008409,-1.80631275399331,3.48758478064276));
#21369=CARTESIAN_POINT('Ctrl Pts',(1.74845530888824,-1.81128723055797,3.48713209471877));
#21370=CARTESIAN_POINT('Ctrl Pts',(1.73849316391186,-1.82084927474419,3.48625475489709));
#21371=CARTESIAN_POINT('Ctrl Pts',(1.73367254737565,-1.82543968859462,3.48583032499636));
#21372=CARTESIAN_POINT('Ctrl Pts',(1.72201250808263,-1.83645507190215,3.48480408717947));
#21373=CARTESIAN_POINT('Ctrl Pts',(1.71515529277909,-1.84286098881615,3.48420086870498));
#21374=CARTESIAN_POINT('Ctrl Pts',(1.6911094225939,-1.8650738544232,3.48208716537312));
#21375=CARTESIAN_POINT('Ctrl Pts',(1.67373736211122,-1.88067932200606,3.48056289556372));
#21376=CARTESIAN_POINT('Ctrl Pts',(1.63027458762246,-1.9186431471577,3.47676157242773));
#21377=CARTESIAN_POINT('Ctrl Pts',(1.60393890545098,-1.94071288771721,3.47446880780639));
#21378=CARTESIAN_POINT('Ctrl Pts',(1.48977456550939,-2.03247330753569,3.46460230041676));
#21379=CARTESIAN_POINT('Ctrl Pts',(1.39779778294782,-2.09679160269266,3.45683767390979));
#21380=CARTESIAN_POINT('Ctrl Pts',(1.151263233354,-2.24574071247285,3.4369449681719));
#21381=CARTESIAN_POINT('Ctrl Pts',(0.991534070169703,-2.32069790843866,
3.42493592058843));
#21382=CARTESIAN_POINT('Ctrl Pts',(0.794146002400204,-2.38918891138065,
3.41136014051053));
#21383=CARTESIAN_POINT('Ctrl Pts',(0.762812716553126,-2.39937668045928,
3.40923921039686));
#21384=CARTESIAN_POINT('Ctrl Pts',(0.716831965717704,-2.41333511848547,
3.4061748339182));
#21385=CARTESIAN_POINT('Ctrl Pts',(0.702337240403806,-2.4175931994747,3.40521570686261));
#21386=CARTESIAN_POINT('Ctrl Pts',(0.676533150631907,-2.4249219461005,3.40352014032761));
#21387=CARTESIAN_POINT('Ctrl Pts',(0.665239134635787,-2.42804457327948,
3.40278204330003));
#21388=CARTESIAN_POINT('Ctrl Pts',(0.641618365982783,-2.43439817942558,
3.40124656931451));
#21389=CARTESIAN_POINT('Ctrl Pts',(0.629288030963136,-2.43761465518074,
3.40044967658379));
#21390=CARTESIAN_POINT('Ctrl Pts',(0.596996005642966,-2.44577695727829,
3.39837448153957));
#21391=CARTESIAN_POINT('Ctrl Pts',(0.576996947687529,-2.45057212027743,
3.397101009265));
#21392=CARTESIAN_POINT('Ctrl Pts',(0.484673455937985,-2.47151557379813,
3.39127321743585));
#21393=CARTESIAN_POINT('Ctrl Pts',(0.411713150437736,-2.48471153322036,
3.38681276013958));
#21394=CARTESIAN_POINT('Ctrl Pts',(0.194177121897359,-2.51420890257995,
3.37381836547031));
#21395=CARTESIAN_POINT('Ctrl Pts',(0.048660402299325,-2.52122703488835,
3.36553363916592));
#21396=CARTESIAN_POINT('Ctrl Pts',(-0.142852604899192,-2.51386890608652,
3.35449845190083));
#21397=CARTESIAN_POINT('Ctrl Pts',(-0.188992894594998,-2.51082162631455,
3.35182787668881));
#21398=CARTESIAN_POINT('Ctrl Pts',(-0.263188565840582,-2.50386468497476,
3.34748090515114));
#21399=CARTESIAN_POINT('Ctrl Pts',(-0.291307966759062,-2.50074912227055,
3.34582116996553));
#21400=CARTESIAN_POINT('Ctrl Pts',(-0.382552431661657,-2.48907963642776,
3.34037919518763));
#21401=CARTESIAN_POINT('Ctrl Pts',(-0.445401720126896,-2.47860437691079,
3.33654292471539));
#21402=CARTESIAN_POINT('Ctrl Pts',(-0.521157792299076,-2.46300372564203,
3.33173895899301));
#21403=CARTESIAN_POINT('Ctrl Pts',(-0.534512312162776,-2.4601401110027,
3.33088522893934));
#21404=CARTESIAN_POINT('Ctrl Pts',(-0.555314694445819,-2.45550207676014,
3.32954369250539));
#21405=CARTESIAN_POINT('Ctrl Pts',(-0.562779112528652,-2.45380205511044,
3.32905995982354));
#21406=CARTESIAN_POINT('Ctrl Pts',(-0.57658933707655,-2.45059044729018,
3.32816042308855));
#21407=CARTESIAN_POINT('Ctrl Pts',(-0.582937135970413,-2.44908821731899,
3.32774514803687));
#21408=CARTESIAN_POINT('Ctrl Pts',(-0.597458810120976,-2.44559195448451,
3.32679102082923));
#21409=CARTESIAN_POINT('Ctrl Pts',(-0.60562854849773,-2.44358161190014,
3.3262512640499));
#21410=CARTESIAN_POINT('Ctrl Pts',(-0.631035500015342,-2.43719443774873,
3.32456373562764));
#21411=CARTESIAN_POINT('Ctrl Pts',(-0.64823608676926,-2.43267598814066,
3.32340842067298));
#21412=CARTESIAN_POINT('Ctrl Pts',(-0.688540729517259,-2.42163050087728,
3.32067328443048));
#21413=CARTESIAN_POINT('Ctrl Pts',(-0.711601855916282,-2.4149545189643,
3.319086556369));
#21414=CARTESIAN_POINT('Ctrl Pts',(-0.794170158447463,-2.38976644418621,
3.31333519381706));
#21415=CARTESIAN_POINT('Ctrl Pts',(-0.853077884324735,-2.36937692926746,
3.30910021546813));
#21416=CARTESIAN_POINT('Ctrl Pts',(-1.09672329928171,-2.2747805768987,3.2911784825484));
#21417=CARTESIAN_POINT('Ctrl Pts',(-1.2731140963201,-2.18096963974417,3.27727592078711));
#21418=CARTESIAN_POINT('Ctrl Pts',(-1.49093792685606,-2.02960248621425,
3.25963439224541));
#21419=CARTESIAN_POINT('Ctrl Pts',(-1.54375500766294,-1.98972459092971,
3.25530642923218));
#21420=CARTESIAN_POINT('Ctrl Pts',(-1.61080487683812,-1.93482147613294,
3.24974178241116));
#21421=CARTESIAN_POINT('Ctrl Pts',(-1.62650694528666,-1.92164036523148,
3.24843320757732));
#21422=CARTESIAN_POINT('Ctrl Pts',(-1.6516948543067,-1.89996641352216,3.2463247295588));
#21423=CARTESIAN_POINT('Ctrl Pts',(-1.66128009982131,-1.89159105090206,
3.24552009417809));
#21424=CARTESIAN_POINT('Ctrl Pts',(-1.67956975512852,-1.87536372195323,
3.24398021825313));
#21425=CARTESIAN_POINT('Ctrl Pts',(-1.68828362861271,-1.86752297141914,
3.24324454287149));
#21426=CARTESIAN_POINT('Ctrl Pts',(-1.70831560627555,-1.84924338367033,
3.24154841723865));
#21427=CARTESIAN_POINT('Ctrl Pts',(-1.71959341949941,-1.83876093902504,
3.24058983070305));
#21428=CARTESIAN_POINT('Ctrl Pts',(-1.75519832861889,-1.80505297681218,
3.23755092435718));
#21429=CARTESIAN_POINT('Ctrl Pts',(-1.7791571098717,-1.78144255130788,3.2354870714768));
#21430=CARTESIAN_POINT('Ctrl Pts',(-1.83434769453083,-1.72482998398978,
3.23068026805999));
#21431=CARTESIAN_POINT('Ctrl Pts',(-1.86517386625816,-1.69144811748293,
3.22795393026716));
#21432=CARTESIAN_POINT('Ctrl Pts',(-1.97805722934954,-1.5623648277117,3.21777166402914));
#21433=CARTESIAN_POINT('Ctrl Pts',(-2.05379396674959,-1.46137860112287,
3.21053271485628));
#21434=CARTESIAN_POINT('Ctrl Pts',(-2.20380360870498,-1.22651897647792,
3.19452017714683));
#21435=CARTESIAN_POINT('Ctrl Pts',(-2.27408017708267,-1.09070903769988,
3.18577779565248));
#21436=CARTESIAN_POINT('Ctrl Pts',(-2.33953929678176,-0.92994785828179,
3.17511175862017));
#21437=CARTESIAN_POINT('Ctrl Pts',(-2.34721388681938,-0.910403231290679,
3.17380971612176));
#21438=CARTESIAN_POINT('Ctrl Pts',(-2.35758517305081,-0.882987855629502,
3.17197291095029));
#21439=CARTESIAN_POINT('Ctrl Pts',(-2.36048891968801,-0.875195667738129,
3.17144967586976));
#21440=CARTESIAN_POINT('Ctrl Pts',(-2.36545060206652,-0.861676696728664,
3.17053964527978));
#21441=CARTESIAN_POINT('Ctrl Pts',(-2.36752649821355,-0.855956516928376,
3.17015389652312));
#21442=CARTESIAN_POINT('Ctrl Pts',(-2.37188486993873,-0.843809767980152,
3.16933317926256));
#21443=CARTESIAN_POINT('Ctrl Pts',(-2.3741619988306,-0.837381371283397,
3.16889789308085));
#21444=CARTESIAN_POINT('Ctrl Pts',(-2.37978555272848,-0.821298593474106,
3.16780667530516));
#21445=CARTESIAN_POINT('Ctrl Pts',(-2.38309934182735,-0.811633029811188,
3.16714888844337));
#21446=CARTESIAN_POINT('Ctrl Pts',(-2.39561913878663,-0.774377898401364,
3.16460663404196));
#21447=CARTESIAN_POINT('Ctrl Pts',(-2.40440521173164,-0.746650918215022,
3.16270014773739));
#21448=CARTESIAN_POINT('Ctrl Pts',(-2.42595743999321,-0.674307103136191,
3.15769953107164));
#21449=CARTESIAN_POINT('Ctrl Pts',(-2.43797347914089,-0.629479457219506,
3.15457534235658));
#21450=CARTESIAN_POINT('Ctrl Pts',(-2.49971753143807,-0.370737594176667,
3.13648773307066));
#21451=CARTESIAN_POINT('Ctrl Pts',(-2.52252971298457,-0.151331259863748,
3.12104593521538));
#21452=CARTESIAN_POINT('Ctrl Pts',(-2.51469800671796,0.137449642934256,
3.10179872673477));
#21453=CARTESIAN_POINT('Ctrl Pts',(-2.50996770517658,0.206548040190508,
3.09726400102883));
#21454=CARTESIAN_POINT('Ctrl Pts',(-2.50011539984802,0.296079994589264,
3.0914780765001));
#21455=CARTESIAN_POINT('Ctrl Pts',(-2.49757927136606,0.316762058377484,
3.09014768627992));
#21456=CARTESIAN_POINT('Ctrl Pts',(-2.49307084906653,0.350096950074888,
3.0880128489194));
#21457=CARTESIAN_POINT('Ctrl Pts',(-2.49125832461962,0.362770041155054,
3.08720344927099));
#21458=CARTESIAN_POINT('Ctrl Pts',(-2.48760437230363,0.386998229362491,
3.08566010392745));
#21459=CARTESIAN_POINT('Ctrl Pts',(-2.48577890713357,0.398555359898262,
3.08492567946336));
#21460=CARTESIAN_POINT('Ctrl Pts',(-2.48139045791008,0.42513512914044,3.08324048269309));
#21461=CARTESIAN_POINT('Ctrl Pts',(-2.47877148966601,0.440148157713901,
3.08229149444509));
#21462=CARTESIAN_POINT('Ctrl Pts',(-2.47009157229782,0.487368289417942,
3.07931497634118));
#21463=CARTESIAN_POINT('Ctrl Pts',(-2.46353783886127,0.519482139296874,
3.07730295206085));
#21464=CARTESIAN_POINT('Ctrl Pts',(-2.44673793709007,0.594313643730848,
3.07263681950008));
#21465=CARTESIAN_POINT('Ctrl Pts',(-2.435997030405,0.636909746295945,3.06999798211615));
#21466=CARTESIAN_POINT('Ctrl Pts',(-2.39207015336152,0.793688945211835,
3.06031716401303));
#21467=CARTESIAN_POINT('Ctrl Pts',(-2.35192235723,0.905762509449909,3.05346794087905));
#21468=CARTESIAN_POINT('Ctrl Pts',(-2.2381278782979,1.16417677531396,3.03724161255528));
#21469=CARTESIAN_POINT('Ctrl Pts',(-2.1578496306127,1.30697907522442,3.02792262634101));
#21470=CARTESIAN_POINT('Ctrl Pts',(-2.05267611894614,1.45764898203386,3.01662309222682));
#21471=CARTESIAN_POINT('Ctrl Pts',(-2.04083492552195,1.47418199365801,3.01536139924901));
#21472=CARTESIAN_POINT('Ctrl Pts',(-2.02391577071154,1.49721044572789,3.01357034872952));
#21473=CARTESIAN_POINT('Ctrl Pts',(-2.01900385365688,1.50382764976125,3.01305172188164));
#21474=CARTESIAN_POINT('Ctrl Pts',(-2.01005804303024,1.51575637809767,3.01210935373858));
#21475=CARTESIAN_POINT('Ctrl Pts',(-2.00603531737064,1.52107627623965,3.01168637542339));
#21476=CARTESIAN_POINT('Ctrl Pts',(-1.99775186904073,1.53194080040577,3.01081685069875));
#21477=CARTESIAN_POINT('Ctrl Pts',(-1.9934891235286,1.53748374226118,3.0103701713089));
#21478=CARTESIAN_POINT('Ctrl Pts',(-1.98245150853844,1.55171312430389,3.00921574652804));
#21479=CARTESIAN_POINT('Ctrl Pts',(-1.97564269978716,1.56037287724135,3.00850569441227));
#21480=CARTESIAN_POINT('Ctrl Pts',(-1.94654819574101,1.59688088240674,3.00548133484038));
#21481=CARTESIAN_POINT('Ctrl Pts',(-1.92372998622106,1.62429709914944,3.00313333120025));
#21482=CARTESIAN_POINT('Ctrl Pts',(-1.85951898013077,1.69819568486777,2.99661106303427));
#21483=CARTESIAN_POINT('Ctrl Pts',(-1.81697393802239,1.7436410594951,2.99238198517743));
#21484=CARTESIAN_POINT('Ctrl Pts',(-1.63229961464143,1.92679988488511,2.97454762553986));
#21485=CARTESIAN_POINT('Ctrl Pts',(-1.47584473239446,2.04911224221236,2.96072737486786));
#21486=CARTESIAN_POINT('Ctrl Pts',(-1.24922388776033,2.18672429166329,2.94308313956118));
#21487=CARTESIAN_POINT('Ctrl Pts',(-1.19039802918825,2.21929659168274,2.93868396082205));
#21488=CARTESIAN_POINT('Ctrl Pts',(-1.11190695324792,2.25873736342474,2.93304258489894));
#21489=CARTESIAN_POINT('Ctrl Pts',(-1.0933662242406,2.26777024644018,2.93172602637423));
#21490=CARTESIAN_POINT('Ctrl Pts',(-1.06318155788361,2.28201970226479,2.92960790181943));
#21491=CARTESIAN_POINT('Ctrl Pts',(-1.0516055990162,2.2873772361348,2.92880152340266));
#21492=CARTESIAN_POINT('Ctrl Pts',(-1.02932188052382,2.29748556560566,2.92726039813304));
#21493=CARTESIAN_POINT('Ctrl Pts',(-1.01862073081102,2.30225004552018,2.92652520025176));
#21494=CARTESIAN_POINT('Ctrl Pts',(-0.993831707052291,2.31308020454868,
2.92483317086968));
#21495=CARTESIAN_POINT('Ctrl Pts',(-0.979720784149016,2.31909221380158,
2.9238781732613));
#21496=CARTESIAN_POINT('Ctrl Pts',(-0.934793678844641,2.33775031374205,
2.9208626950068));
#21497=CARTESIAN_POINT('Ctrl Pts',(-0.903780261914417,2.34991428532921,
2.91881831672342));
#21498=CARTESIAN_POINT('Ctrl Pts',(-0.83045466926891,2.37700728712604,2.9140644857403));
#21499=CARTESIAN_POINT('Ctrl Pts',(-0.787966269845653,2.39142804494661,
2.91137113266122));
#21500=CARTESIAN_POINT('Ctrl Pts',(-0.627332967009044,2.44120128131698,
2.90138049976519));
#21501=CARTESIAN_POINT('Ctrl Pts',(-0.507024909679662,2.46899552152921,
2.89429073882447));
#21502=CARTESIAN_POINT('Ctrl Pts',(-0.373100388752179,2.48972915813977,
2.88650397502014));
#21503=CARTESIAN_POINT('Ctrl Pts',(-0.361026919649716,2.4915085277924,2.88580281368281));
#21504=CARTESIAN_POINT('Ctrl Pts',(-0.206630451209501,2.5131174066636,2.87684243796109));
#21505=CARTESIAN_POINT('Ctrl Pts',(-0.0628934766570935,2.52081119644265,
2.86857856377841));
#21506=CARTESIAN_POINT('Ctrl Pts',(0.101947062899903,2.51552484072547,2.85844853305551));
#21507=CARTESIAN_POINT('Ctrl Pts',(0.123190319662389,2.51457402046924,2.8571303815876));
#21508=CARTESIAN_POINT('Ctrl Pts',(0.152803218266471,2.51287245353318,2.85527204210989));
#21509=CARTESIAN_POINT('Ctrl Pts',(0.161185666735311,2.51234869541708,2.85474367295009));
#21510=CARTESIAN_POINT('Ctrl Pts',(0.175657399741574,2.51137173910912,2.85382720652775));
#21511=CARTESIAN_POINT('Ctrl Pts',(0.18174800831294,2.51093830940743,2.85344019210531));
#21512=CARTESIAN_POINT('Ctrl Pts',(0.194612585022782,2.50997576853738,2.85261986285461));
#21513=CARTESIAN_POINT('Ctrl Pts',(0.201386063150256,2.50944138547143,2.85218624937463));
#21514=CARTESIAN_POINT('Ctrl Pts',(0.21821934900887,2.50804475838059,2.85110457204126));
#21515=CARTESIAN_POINT('Ctrl Pts',(0.228276208659745,2.50714940892081,2.85045471865989));
#21516=CARTESIAN_POINT('Ctrl Pts',(0.26638712461251,2.503525240354,2.84797903568993));
#21517=CARTESIAN_POINT('Ctrl Pts',(0.294398890518322,2.50038594327313,2.84613259776715));
#21518=CARTESIAN_POINT('Ctrl Pts',(0.366401059950976,2.49108998215924,2.84132720683863));
#21519=CARTESIAN_POINT('Ctrl Pts',(0.410290872402409,2.4842383116301,2.83834084816532));
#21520=CARTESIAN_POINT('Ctrl Pts',(0.548304915399368,2.45893582690046,2.82881274187096));
#21521=CARTESIAN_POINT('Ctrl Pts',(0.641567526632519,2.43626632422023,2.82217353630221));
#21522=CARTESIAN_POINT('Ctrl Pts',(0.901082493008442,2.35724738529896,2.80343855349362));
#21523=CARTESIAN_POINT('Ctrl Pts',(1.06308842496709,2.28876121845641,2.79146798812186));
#21524=CARTESIAN_POINT('Ctrl Pts',(1.24504301358969,2.18831531239108,2.77796172802742));
#21525=CARTESIAN_POINT('Ctrl Pts',(1.27310407652904,2.1721100759696,2.77587520841093));
#21526=CARTESIAN_POINT('Ctrl Pts',(1.31389599146097,2.1474906109862,2.77283545736936));
#21527=CARTESIAN_POINT('Ctrl Pts',(1.32687481053861,2.13949570097053,2.77186727856046));
#21528=CARTESIAN_POINT('Ctrl Pts',(1.34934163025603,2.12537313255695,2.77018928761137));
#21529=CARTESIAN_POINT('Ctrl Pts',(1.35886238252501,2.11929866224996,2.76947755954944));
#21530=CARTESIAN_POINT('Ctrl Pts',(1.37746306078472,2.10725409985954,2.76808564045312));
#21531=CARTESIAN_POINT('Ctrl Pts',(1.38654583490639,2.10128888514113,2.76740529007627));
#21532=CARTESIAN_POINT('Ctrl Pts',(1.41048381300153,2.08534455405227,2.76561022065557));
#21533=CARTESIAN_POINT('Ctrl Pts',(1.4252718980391,2.07526541394443,2.76449925106208));
#21534=CARTESIAN_POINT('Ctrl Pts',(1.48067372532626,2.03663354087659,2.76032794016278));
#21535=CARTESIAN_POINT('Ctrl Pts',(1.52054891479112,2.00703820567017,2.75730705847066));
#21536=CARTESIAN_POINT('Ctrl Pts',(1.61993872037049,1.92860763391846,2.74970116868446));
#21537=CARTESIAN_POINT('Ctrl Pts',(1.67813746788893,1.87818657481302,2.74517492606913));
#21538=CARTESIAN_POINT('Ctrl Pts',(1.80775107238824,1.75505210947985,2.73478374756119));
#21539=CARTESIAN_POINT('Ctrl Pts',(1.87724313439426,1.68051492397956,2.72896981967822));
#21540=CARTESIAN_POINT('Ctrl Pts',(1.97971512538996,1.55629091919991,2.71969270406915));
#21541=CARTESIAN_POINT('Ctrl Pts',(2.01577470029517,1.50929297108582,2.71626548606949));
#21542=CARTESIAN_POINT('Ctrl Pts',(2.09345290729549,1.40029650535367,2.70839880870442));
#21543=CARTESIAN_POINT('Ctrl Pts',(2.13403574625664,1.33763395736447,2.70393206790445));
#21544=CARTESIAN_POINT('Ctrl Pts',(2.17834447459626,1.26205803152608,2.69849599581683));
#21545=CARTESIAN_POINT('Ctrl Pts',(2.18482995186509,1.25079702184486,2.69768476671425));
#21546=CARTESIAN_POINT('Ctrl Pts',(2.19526147742054,1.23235563727955,2.69635341592008));
#21547=CARTESIAN_POINT('Ctrl Pts',(2.19926025732571,1.22520516121395,2.69583650361944));
#21548=CARTESIAN_POINT('Ctrl Pts',(2.20637332013503,1.21233881061133,2.69490491367588));
#21549=CARTESIAN_POINT('Ctrl Pts',(2.20950042246204,1.20663022537022,2.69449105334225));
#21550=CARTESIAN_POINT('Ctrl Pts',(2.2163393576788,1.19402988783534,2.69357635275449));
#21551=CARTESIAN_POINT('Ctrl Pts',(2.22004115315811,1.18713301520003,2.69307492039927));
#21552=CARTESIAN_POINT('Ctrl Pts',(2.23067482018304,1.16709758389474,2.69161629212046));
#21553=CARTESIAN_POINT('Ctrl Pts',(2.23752250331571,1.15391505135971,2.69065413464249));
#21554=CARTESIAN_POINT('Ctrl Pts',(2.28848054339192,1.05365606101378,2.68332246710814));
#21555=CARTESIAN_POINT('Ctrl Pts',(2.32760090953802,0.964157929869422,2.67670089885606));
#21556=CARTESIAN_POINT('Ctrl Pts',(2.36142200370902,0.872635302058581,2.66999896006316));
#21557=CARTESIAN_POINT('Origin',(0.,0.,10.));
#21558=CARTESIAN_POINT('',(2.36142200724207,0.872635292497862,1.66658329180866));
#21559=CARTESIAN_POINT('',(2.36142200728636,0.872635292378021,1.94383454073647));
#21560=CARTESIAN_POINT('',(2.36142200728636,0.87263529237802,10.));
#21561=CARTESIAN_POINT('',(2.51749898697345,-0.00225844805835542,2.88741669746852));
#21562=CARTESIAN_POINT('Ctrl Pts',(2.36142200728636,0.872635292378021,1.94383454073647));
#21563=CARTESIAN_POINT('Ctrl Pts',(2.33265413141813,0.950483502015518,1.94907292625409));
#21564=CARTESIAN_POINT('Ctrl Pts',(2.30001172667712,1.02696408405365,1.95431131177171));
#21565=CARTESIAN_POINT('Ctrl Pts',(2.26365383506435,1.10167035223721,1.95954969728933));
#21566=CARTESIAN_POINT('Ctrl Pts',(2.2273076844016,1.1763524957391,1.96478639119009));
#21567=CARTESIAN_POINT('Ctrl Pts',(2.18724863159326,1.24926104878193,1.97002308509085));
#21568=CARTESIAN_POINT('Ctrl Pts',(2.14368314884031,1.32001091184054,1.97525977899161));
#21569=CARTESIAN_POINT('Ctrl Pts',(2.10011859343222,1.39075926890134,1.9804963614229));
#21570=CARTESIAN_POINT('Ctrl Pts',(2.05304799935803,1.45934863501175,1.9857329438542));
#21571=CARTESIAN_POINT('Ctrl Pts',(2.00272220913907,1.52542125428392,1.99096952628549));
#21572=CARTESIAN_POINT('Ctrl Pts',(1.95182111346055,1.5922491908284,1.9962659713528));
#21573=CARTESIAN_POINT('Ctrl Pts',(1.89759020054139,1.65650207795797,2.00156241642011));
#21574=CARTESIAN_POINT('Ctrl Pts',(1.8403309830746,1.71784403329746,2.00685886148742));
#21575=CARTESIAN_POINT('Ctrl Pts',(1.7836372765285,1.77858015525019,2.01210299711603));
#21576=CARTESIAN_POINT('Ctrl Pts',(1.72397519722586,1.83646231030203,2.01734713274463));
#21577=CARTESIAN_POINT('Ctrl Pts',(1.66167330739977,1.89120281024408,2.02259126837324));
#21578=CARTESIAN_POINT('Ctrl Pts',(1.59843924005638,1.94676235216823,2.0279138681599));
#21579=CARTESIAN_POINT('Ctrl Pts',(1.53248610333258,1.99908514507073,2.03323646794657));
#21580=CARTESIAN_POINT('Ctrl Pts',(1.4641892332896,2.04791507126609,2.03855906773323));
#21581=CARTESIAN_POINT('Ctrl Pts',(1.39589236324662,2.09674499746146,2.04388166751989));
#21582=CARTESIAN_POINT('Ctrl Pts',(1.32525220718384,2.14208184682114,2.04920426730656));
#21583=CARTESIAN_POINT('Ctrl Pts',(1.25266969650984,2.18371813232522,2.05452686709322));
#21584=CARTESIAN_POINT('Ctrl Pts',(1.18100561291598,2.22482757063473,2.05978211704952));
#21585=CARTESIAN_POINT('Ctrl Pts',(1.10718338004907,2.26248143958662,2.06503736700583));
#21586=CARTESIAN_POINT('Ctrl Pts',(1.03157001246663,2.29644716015405,2.07029261696213));
#21587=CARTESIAN_POINT('Ctrl Pts',(0.956063846954617,2.33036472527377,2.07554041620312));
#21588=CARTESIAN_POINT('Ctrl Pts',(0.878772008130202,2.36060434069963,2.08078821544411));
#21589=CARTESIAN_POINT('Ctrl Pts',(0.800087506862563,2.38697847316696,2.08603601468509));
#21590=CARTESIAN_POINT('Ctrl Pts',(0.720832879483858,2.41354370529602,2.09132183802644));
#21591=CARTESIAN_POINT('Ctrl Pts',(0.640165733872132,2.43618696587407,2.09660766136779));
#21592=CARTESIAN_POINT('Ctrl Pts',(0.558509796253283,2.45476537727929,2.10189348470913));
#21593=CARTESIAN_POINT('Ctrl Pts',(0.477586049366593,2.47317720017856,2.10713191124168));
#21594=CARTESIAN_POINT('Ctrl Pts',(0.395691630223132,2.48759667489879,2.11237033777423));
#21595=CARTESIAN_POINT('Ctrl Pts',(0.313254036815387,2.49793477865593,2.11760876430678));
#21596=CARTESIAN_POINT('Ctrl Pts',(0.230843555302572,2.50826948244018,2.1228454680371));
#21597=CARTESIAN_POINT('Ctrl Pts',(0.147890711783706,2.51452542371834,2.12808217176742));
#21598=CARTESIAN_POINT('Ctrl Pts',(0.0648308480982068,2.51666509713447,
2.13331887549774));
#21599=CARTESIAN_POINT('Ctrl Pts',(-0.0182267535231641,2.51880471227844,
2.13855543661092));
#21600=CARTESIAN_POINT('Ctrl Pts',(-0.101390908222088,2.51682827159825,
2.14379199772411));
#21601=CARTESIAN_POINT('Ctrl Pts',(-0.184224923671929,2.51075037140256,
2.1490285588373));
#21602=CARTESIAN_POINT('Ctrl Pts',(-0.268414684946125,2.50457299410477,
2.15435082684063));
#21603=CARTESIAN_POINT('Ctrl Pts',(-0.352262911315727,2.4941587115898,2.15967309484397));
#21604=CARTESIAN_POINT('Ctrl Pts',(-0.435316991251371,2.47957765902338,
2.16499536284731));
#21605=CARTESIAN_POINT('Ctrl Pts',(-0.517150970037226,2.46521080856497,
2.17023944438088));
#21606=CARTESIAN_POINT('Ctrl Pts',(-0.598213537433156,2.44679896233672,
2.17548352591445));
#21607=CARTESIAN_POINT('Ctrl Pts',(-0.678084274595561,2.42446034542663,
2.18072760744801));
#21608=CARTESIAN_POINT('Ctrl Pts',(-0.759741257148187,2.40162214315027,
2.18608896868624));
#21609=CARTESIAN_POINT('Ctrl Pts',(-0.840151972029443,2.37467957529194,
2.19145032992447));
#21610=CARTESIAN_POINT('Ctrl Pts',(-0.918887750789561,2.34381133017334,
2.19681169116269));
#21611=CARTESIAN_POINT('Ctrl Pts',(-0.997623529549678,2.31294308505473,
2.20217305240092));
#21612=CARTESIAN_POINT('Ctrl Pts',(-1.07468393658661,2.27814943264632,2.20753441363915));
#21613=CARTESIAN_POINT('Ctrl Pts',(-1.14966790242312,2.23965844809829,2.21289577487737));
#21614=CARTESIAN_POINT('Ctrl Pts',(-1.22316775138176,2.20192929468543,2.21815102160681));
#21615=CARTESIAN_POINT('Ctrl Pts',(-1.29494410802143,2.1605085163771,2.22340626833624));
#21616=CARTESIAN_POINT('Ctrl Pts',(-1.36460206538526,2.11557733329375,2.22866151506568));
#21617=CARTESIAN_POINT('Ctrl Pts',(-1.43416126292787,2.07070985284792,2.23390931099915));
#21618=CARTESIAN_POINT('Ctrl Pts',(-1.50160764236144,2.02234210140636,2.23915710693263));
#21619=CARTESIAN_POINT('Ctrl Pts',(-1.56656992694817,1.97070162987237,2.2444049028661));
#21620=CARTESIAN_POINT('Ctrl Pts',(-1.63200296161448,1.91868694495843,2.24969072702424));
#21621=CARTESIAN_POINT('Ctrl Pts',(-1.69491532586794,1.86335212458742,2.25497655118239));
#21622=CARTESIAN_POINT('Ctrl Pts',(-1.75495647585527,1.80497479701343,2.26026237534053));
#21623=CARTESIAN_POINT('Ctrl Pts',(-1.81445920139815,1.74712097340586,2.26550079839233));
#21624=CARTESIAN_POINT('Ctrl Pts',(-1.87114166523572,1.6862793195283,2.27073922144413));
#21625=CARTESIAN_POINT('Ctrl Pts',(-1.9246964437954,1.62275994812583,2.27597764449592));
#21626=CARTESIAN_POINT('Ctrl Pts',(-1.9782336087776,1.5592614675458,2.28121434468801));
#21627=CARTESIAN_POINT('Ctrl Pts',(-2.02864483426583,1.49308737099406,2.28645104488009));
#21628=CARTESIAN_POINT('Ctrl Pts',(-2.07566163847028,1.42458239936582,2.29168774507218));
#21629=CARTESIAN_POINT('Ctrl Pts',(-2.12267716173675,1.35607929410476,2.29692430259425));
#21630=CARTESIAN_POINT('Ctrl Pts',(-2.16629818733523,1.28524582104953,2.30216086011633));
#21631=CARTESIAN_POINT('Ctrl Pts',(-2.20629920064349,1.21245622075187,2.3073974176384));
#21632=CARTESIAN_POINT('Ctrl Pts',(-2.24695497031956,1.13847516427939,2.31271968972366));
#21633=CARTESIAN_POINT('Ctrl Pts',(-2.28387090180366,1.06247378967159,2.31804196180892));
#21634=CARTESIAN_POINT('Ctrl Pts',(-2.31685939799245,0.984869930464954,
2.32336423389419));
#21635=CARTESIAN_POINT('Ctrl Pts',(-2.3493632308149,0.908406218642723,2.32860831174196));
#21636=CARTESIAN_POINT('Ctrl Pts',(-2.37805416120823,0.830387257136895,
2.33385238958973));
#21637=CARTESIAN_POINT('Ctrl Pts',(-2.4028024577348,0.751230057374981,2.33909646743751));
#21638=CARTESIAN_POINT('Ctrl Pts',(-2.42810428556819,0.670302392798165,
2.34445783664152));
#21639=CARTESIAN_POINT('Ctrl Pts',(-2.44928485791634,0.588185454647371,
2.34981920584553));
#21640=CARTESIAN_POINT('Ctrl Pts',(-2.46626066743033,0.505336096361721,
2.35518057504954));
#21641=CARTESIAN_POINT('Ctrl Pts',(-2.48323647694432,0.422486738076075,
2.36054194425355));
#21642=CARTESIAN_POINT('Ctrl Pts',(-2.49600751290881,0.338905472027392,
2.36590331345755));
#21643=CARTESIAN_POINT('Ctrl Pts',(-2.50454672006448,0.255052890621214,
2.37126468266156));
#21644=CARTESIAN_POINT('Ctrl Pts',(-2.51291690935513,0.172860016495573,
2.37651993344498));
#21645=CARTESIAN_POINT('Ctrl Pts',(-2.51725222683093,0.0901028851533855,
2.38177518422839));
#21646=CARTESIAN_POINT('Ctrl Pts',(-2.51748967139839,0.0072114077971777,
2.38703043501181));
#21647=CARTESIAN_POINT('Ctrl Pts',(-2.51772677932425,-0.0755625485714478,
2.39227823506227));
#21648=CARTESIAN_POINT('Ctrl Pts',(-2.5138775530656,-0.158470015052679,
2.39752603511273));
#21649=CARTESIAN_POINT('Ctrl Pts',(-2.5059307189532,-0.241075676514023,
2.40277383516319));
#21650=CARTESIAN_POINT('Ctrl Pts',(-2.49792630582551,-0.324279859673127,
2.40805965829996));
#21651=CARTESIAN_POINT('Ctrl Pts',(-2.48576460762758,-0.407177374436601,
2.41334548143673));
#21652=CARTESIAN_POINT('Ctrl Pts',(-2.46948764310001,-0.489323032951007,
2.41863130457351));
#21653=CARTESIAN_POINT('Ctrl Pts',(-2.45335662754912,-0.570732124473509,
2.4238697318659));
#21654=CARTESIAN_POINT('Ctrl Pts',(-2.43318394130393,-0.651402327969849,
2.42910815915829));
#21655=CARTESIAN_POINT('Ctrl Pts',(-2.40906232782647,-0.730906937063328,
2.43434658645068));
#21656=CARTESIAN_POINT('Ctrl Pts',(-2.38494864750538,-0.810385398548718,
2.43958329092039));
#21657=CARTESIAN_POINT('Ctrl Pts',(-2.35688875315938,-0.888698585773644,
2.4448199953901));
#21658=CARTESIAN_POINT('Ctrl Pts',(-2.32502563597652,-0.965433603129697,
2.45005669985981));
#21659=CARTESIAN_POINT('Ctrl Pts',(-2.29316338668939,-1.04216653035772,
2.45529326169082));
#21660=CARTESIAN_POINT('Ctrl Pts',(-2.25749829843715,-1.11732094743798,
2.46052982352183));
#21661=CARTESIAN_POINT('Ctrl Pts',(-2.21822150001762,-1.19050393819575,
2.46576638535285));
#21662=CARTESIAN_POINT('Ctrl Pts',(-2.17830186984482,-1.26488469333735,
2.47108865244392));
#21663=CARTESIAN_POINT('Ctrl Pts',(-2.13465146028981,-1.3372284689841,2.47641091953499));
#21664=CARTESIAN_POINT('Ctrl Pts',(-2.08751860851424,-1.40715042163473,
2.48173318662607));
#21665=CARTESIAN_POINT('Ctrl Pts',(-2.04107814539084,-1.47604521032795,
2.4869772688164));
#21666=CARTESIAN_POINT('Ctrl Pts',(-1.99125720574241,-1.54258851974971,
2.49222135100673));
#21667=CARTESIAN_POINT('Ctrl Pts',(-1.93833494345258,-1.60644448923412,
2.49746543319706));
#21668=CARTESIAN_POINT('Ctrl Pts',(-1.88422914083846,-1.67172851775383,
2.50282679273851));
#21669=CARTESIAN_POINT('Ctrl Pts',(-1.82688197361883,-1.73420318074725,
2.50818815227995));
#21670=CARTESIAN_POINT('Ctrl Pts',(-1.7666311789406,-1.79354970034147,2.51354951182139));
#21671=CARTESIAN_POINT('Ctrl Pts',(-1.70638038426236,-1.85289621993568,
2.51891087136284));
#21672=CARTESIAN_POINT('Ctrl Pts',(-1.64322638605859,-1.90911430818517,
2.52427223090428));
#21673=CARTESIAN_POINT('Ctrl Pts',(-1.57754079279172,-1.96193050261167,
2.52963359044573));
#21674=CARTESIAN_POINT('Ctrl Pts',(-1.51315522620229,-2.01370137707772,
2.53488883980251));
#21675=CARTESIAN_POINT('Ctrl Pts',(-1.44609957370261,-2.06239504521322,
2.54014408915929));
#21676=CARTESIAN_POINT('Ctrl Pts',(-1.37670014015963,-2.10772459635609,
2.54539933851607));
#21677=CARTESIAN_POINT('Ctrl Pts',(-1.30739909920855,-2.1529898805187,2.55064713712609));
#21678=CARTESIAN_POINT('Ctrl Pts',(-1.23576126065028,-2.19490027118673,
2.5558949357361));
#21679=CARTESIAN_POINT('Ctrl Pts',(-1.16214562522365,-2.23320930406747,
2.56114273434611));
#21680=CARTESIAN_POINT('Ctrl Pts',(-1.08799658021141,-2.2717959193563,2.56642855784127));
#21681=CARTESIAN_POINT('Ctrl Pts',(-1.01184132497023,-2.30672846972519,
2.57171438133643));
#21682=CARTESIAN_POINT('Ctrl Pts',(-0.934076156963984,-2.33779981670617,
2.57700020483159));
#21683=CARTESIAN_POINT('Ctrl Pts',(-0.857008304613156,-2.36859254875914,
2.58223863066055));
#21684=CARTESIAN_POINT('Ctrl Pts',(-0.778359732224536,-2.39559287208768,
2.58747705648951));
#21685=CARTESIAN_POINT('Ctrl Pts',(-0.698538851910779,-2.41864625821371,
2.59271548231847));
#21686=CARTESIAN_POINT('Ctrl Pts',(-0.618744223309859,-2.44169206247807,
2.59795218531939));
#21687=CARTESIAN_POINT('Ctrl Pts',(-0.537778495463607,-2.4607933796665,
2.60318888832031));
#21688=CARTESIAN_POINT('Ctrl Pts',(-0.456065853583791,-2.47584534799629,
2.60842559132124));
#21689=CARTESIAN_POINT('Ctrl Pts',(-0.374355437466878,-2.49089690632695,
2.6136621516801));
#21690=CARTESIAN_POINT('Ctrl Pts',(-0.291898601740537,-2.50189925252725,
2.61889871203897));
#21691=CARTESIAN_POINT('Ctrl Pts',(-0.209128981627125,-2.50879878010246,
2.62413527239784));
#21692=CARTESIAN_POINT('Ctrl Pts',(-0.12500464463323,-2.51581123445517,
2.62945754121718));
#21693=CARTESIAN_POINT('Ctrl Pts',(-0.0405576809259553,-2.51858530024611,
2.63477981003652));
#21694=CARTESIAN_POINT('Ctrl Pts',(0.0437538975583074,-2.51711975210725,
2.64010207885586));
#21695=CARTESIAN_POINT('Ctrl Pts',(0.126826876137409,-2.51567573396247,
2.64534615958083));
#21696=CARTESIAN_POINT('Ctrl Pts',(0.209767958040033,-2.51011593374228,
2.6505902403058));
#21697=CARTESIAN_POINT('Ctrl Pts',(0.292143440366348,-2.50049164370748,
2.65583432103077));
#21698=CARTESIAN_POINT('Ctrl Pts',(0.376361223275997,-2.49065210958979,
2.66119568389729));
#21699=CARTESIAN_POINT('Ctrl Pts',(0.459987297506857,-2.47656417495975,
2.66655704676382));
#21700=CARTESIAN_POINT('Ctrl Pts',(0.542570392136683,-2.45833757233962,
2.67191840963034));
#21701=CARTESIAN_POINT('Ctrl Pts',(0.625153486766509,-2.44011096971949,
2.67727977249686));
#21702=CARTESIAN_POINT('Ctrl Pts',(0.706693129455465,-2.41774589792986,
2.68264113536339));
#21703=CARTESIAN_POINT('Ctrl Pts',(0.78675761828311,-2.39140517271195,2.68800249822991));
#21704=CARTESIAN_POINT('Ctrl Pts',(0.865237445155743,-2.36558579154721,
2.69325774728885));
#21705=CARTESIAN_POINT('Ctrl Pts',(0.942589867960649,-2.33585137359311,
2.69851299634779));
#21706=CARTESIAN_POINT('Ctrl Pts',(1.01839657108159,-2.30231941181263,2.70376824540673));
#21707=CARTESIAN_POINT('Ctrl Pts',(1.09409579741994,-2.2688349907801,2.70901604370951));
#21708=CARTESIAN_POINT('Ctrl Pts',(1.16825323853503,-2.23156390533443,2.71426384201229));
#21709=CARTESIAN_POINT('Ctrl Pts',(1.24046670358489,-2.19067309457555,2.71951164031506));
#21710=CARTESIAN_POINT('Ctrl Pts',(1.31320342357032,-2.14948599117189,2.72479746388586));
#21711=CARTESIAN_POINT('Ctrl Pts',(1.38396742657179,-2.10462663253549,2.73008328745665));
#21712=CARTESIAN_POINT('Ctrl Pts',(1.45236920159089,-2.05631465303106,2.73536911102744));
#21713=CARTESIAN_POINT('Ctrl Pts',(1.52015761673026,-2.00843588786837,2.74060753652839));
#21714=CARTESIAN_POINT('Ctrl Pts',(1.58562561464942,-1.95716644436069,2.74584596202934));
#21715=CARTESIAN_POINT('Ctrl Pts',(1.64842121744586,-1.90276476209602,2.75108438753029));
#21716=CARTESIAN_POINT('Ctrl Pts',(1.71119616776366,-1.84838097168254,2.75632109019611));
#21717=CARTESIAN_POINT('Ctrl Pts',(1.77130012004533,-1.79086729032705,2.76155779286192));
#21718=CARTESIAN_POINT('Ctrl Pts',(1.828414168735,-1.73052242908582,2.76679449552774));
#21719=CARTESIAN_POINT('Ctrl Pts',(1.88552666162767,-1.67017921164952,2.77203105554483));
#21720=CARTESIAN_POINT('Ctrl Pts',(1.93964909643247,-1.60700530349576,2.77726761556192));
#21721=CARTESIAN_POINT('Ctrl Pts',(1.99050041505611,-1.54133524830305,2.78250417557901));
#21722=CARTESIAN_POINT('Ctrl Pts',(2.04218404059567,-1.47459034111862,2.78782644478193));
#21723=CARTESIAN_POINT('Ctrl Pts',(2.09048819269342,-1.40526721925857,2.79314871398485));
#21724=CARTESIAN_POINT('Ctrl Pts',(2.13516247809648,-1.33374939255053,2.79847098318777));
#21725=CARTESIAN_POINT('Ctrl Pts',(2.17918045881088,-1.26328222584898,2.80371506355789));
#21726=CARTESIAN_POINT('Ctrl Pts',(2.21967434238095,-1.19068484919091,2.808959143928));
#21727=CARTESIAN_POINT('Ctrl Pts',(2.25645102213422,-1.11634897532512,2.81420322429812));
#21728=CARTESIAN_POINT('Ctrl Pts',(2.29405020806441,-1.0403505882626,2.81956458791744));
#21729=CARTESIAN_POINT('Ctrl Pts',(2.32776371056333,-0.962535472885557,
2.82492595153677));
#21730=CARTESIAN_POINT('Ctrl Pts',(2.35743787716961,-0.883341896032365,
2.8302873151561));
#21731=CARTESIAN_POINT('Ctrl Pts',(2.38711204377589,-0.804148319179173,
2.83564867877542));
#21732=CARTESIAN_POINT('Ctrl Pts',(2.4127467840924,-0.723576785293608,2.84101004239475));
#21733=CARTESIAN_POINT('Ctrl Pts',(2.43424362587157,-0.642078048140283,
2.84637140601408));
#21734=CARTESIAN_POINT('Ctrl Pts',(2.4616727216149,-0.538088974428746,2.85321228792315));
#21735=CARTESIAN_POINT('Ctrl Pts',(2.48245069282632,-0.432277824801234,
2.86005316983222));
#21736=CARTESIAN_POINT('Ctrl Pts',(2.49638302074693,-0.325389095893594,
2.8668940517413));
#21737=CARTESIAN_POINT('Ctrl Pts',(2.51031534866753,-0.21850036698595,2.87373493365037));
#21738=CARTESIAN_POINT('Ctrl Pts',(2.5174018532492,-0.110533708811776,2.88057581555944));
#21739=CARTESIAN_POINT('Ctrl Pts',(2.51749898697345,-0.00225844805835206,
2.88741669746852));
#21740=CARTESIAN_POINT('Ctrl Pts',(2.51749898697402,-0.00225844743326701,
2.88741669750801));
#21741=CARTESIAN_POINT('Ctrl Pts',(2.51757261561498,0.0798156475007308,
2.89260217743504));
#21742=CARTESIAN_POINT('Ctrl Pts',(2.51362838985468,0.161986453160739,2.89778765736208));
#21743=CARTESIAN_POINT('Ctrl Pts',(2.50566466175838,0.243825455634248,2.90297313728911));
#21744=CARTESIAN_POINT('Ctrl Pts',(2.49770584428074,0.325613994288886,2.90815541972948));
#21745=CARTESIAN_POINT('Ctrl Pts',(2.4857324912812,0.407070667135054,2.91333770216984));
#21746=CARTESIAN_POINT('Ctrl Pts',(2.46979497608291,0.487769439505618,2.9185199846102));
#21747=CARTESIAN_POINT('Ctrl Pts',(2.4538590637285,0.568460095960229,2.92370174586582));
#21748=CARTESIAN_POINT('Ctrl Pts',(2.4339598626489,0.648392538286256,2.92888350712144));
#21749=CARTESIAN_POINT('Ctrl Pts',(2.41019910481231,0.72714958926064,2.93406526837706));
#21750=CARTESIAN_POINT('Ctrl Pts',(2.39542133466959,0.776131764173706,2.93728801393495));
#21751=CARTESIAN_POINT('Ctrl Pts',(2.37915089320259,0.824659486525423,2.94051075949285));
#21752=CARTESIAN_POINT('Ctrl Pts',(2.36142200728636,0.872635292378019,2.94373350505074));
#21753=CARTESIAN_POINT('',(2.51749999784475,0.000104171493018674,2.61023257544742));
#21754=CARTESIAN_POINT('Ctrl Pts',(2.36142200370902,0.872635302058581,2.66999896006316));
#21755=CARTESIAN_POINT('Ctrl Pts',(2.36560483263882,0.861316227240872,2.66917009677071));
#21756=CARTESIAN_POINT('Ctrl Pts',(2.36970660561097,0.849966189911584,2.66833995597539));
#21757=CARTESIAN_POINT('Ctrl Pts',(2.44966690857208,0.623628147166383,2.65180981247241));
#21758=CARTESIAN_POINT('Ctrl Pts',(2.49607367105078,0.399296602080148,2.63599979237781));
#21759=CARTESIAN_POINT('Ctrl Pts',(2.51373507564165,0.141034278453407,2.61920134346827));
#21760=CARTESIAN_POINT('Ctrl Pts',(2.51527232959309,0.110272133569269,2.61722005897344));
#21761=CARTESIAN_POINT('Ctrl Pts',(2.51670862159752,0.0648055824669632,
2.61431949278353));
#21762=CARTESIAN_POINT('Ctrl Pts',(2.51704393563378,0.0501187643659415,
2.61338680522547));
#21763=CARTESIAN_POINT('Ctrl Pts',(2.51735379166243,0.0281036860631062,
2.61199492973371));
#21764=CARTESIAN_POINT('Ctrl Pts',(2.51742492146047,0.0207773004703606,
2.61153275554957));
#21765=CARTESIAN_POINT('Ctrl Pts',(2.51748783676618,0.00900187890311291,
2.61079154030412));
#21766=CARTESIAN_POINT('Ctrl Pts',(2.51749981375532,0.00455303872383315,
2.6105118753073));
#21767=CARTESIAN_POINT('Ctrl Pts',(2.51749999784475,0.000104171493018674,
2.61023257544742));
#21768=CARTESIAN_POINT('Ctrl Pts',(2.51749999784015,0.000104282475506742,
2.6102325824149));
#21769=CARTESIAN_POINT('Ctrl Pts',(2.51750022479702,-0.00537471984685295,
2.60988861067223));
#21770=CARTESIAN_POINT('Ctrl Pts',(2.51748256528205,-0.0108537515103197,
2.60954519348913));
#21771=CARTESIAN_POINT('Ctrl Pts',(2.51738144358299,-0.0264401591722797,
2.60856981810447));
#21772=CARTESIAN_POINT('Ctrl Pts',(2.51725499699461,-0.0365472206500459,
2.60793919480463));
#21773=CARTESIAN_POINT('Ctrl Pts',(2.51664876752044,-0.0692548427430348,
2.60590424622283));
#21774=CARTESIAN_POINT('Ctrl Pts',(2.51592544507136,-0.0918501948059999,
2.60450745476016));
#21775=CARTESIAN_POINT('Ctrl Pts',(2.51055257667226,-0.209929573437987,
2.59725081006728));
#21776=CARTESIAN_POINT('Ctrl Pts',(2.50077135808014,-0.30510696611966,2.59155198304949));
#21777=CARTESIAN_POINT('Ctrl Pts',(2.45882025594135,-0.566113290107611,
2.5760757995714));
#21778=CARTESIAN_POINT('Ctrl Pts',(2.41536020766425,-0.729598243129649,
2.56657451789204));
#21779=CARTESIAN_POINT('Ctrl Pts',(2.33486495002623,-0.943272842912999,
2.55323697219275));
#21780=CARTESIAN_POINT('Ctrl Pts',(2.31188277138799,-0.99827607715766,2.54971235222533));
#21781=CARTESIAN_POINT('Ctrl Pts',(2.27722642761517,-1.07358724792391,2.54469096161048));
#21782=CARTESIAN_POINT('Ctrl Pts',(2.2671870395028,-1.09462899172694,2.54326611708904));
#21783=CARTESIAN_POINT('Ctrl Pts',(2.24915360344967,-1.13111297926263,2.54075198124741));
#21784=CARTESIAN_POINT('Ctrl Pts',(2.24128895854769,-1.14661775202205,2.53966954485422));
#21785=CARTESIAN_POINT('Ctrl Pts',(2.22941641910484,-1.16943498521629,2.53805396455376));
#21786=CARTESIAN_POINT('Ctrl Pts',(2.22553157132549,-1.17681135903904,2.53752814049659));
#21787=CARTESIAN_POINT('Ctrl Pts',(2.21883643611925,-1.18937205870896,2.53662646318241));
#21788=CARTESIAN_POINT('Ctrl Pts',(2.21604446192654,-1.1945660158331,2.53625175754563));
#21789=CARTESIAN_POINT('Ctrl Pts',(2.20967806856464,-1.20631039347719,2.53540022030728));
#21790=CARTESIAN_POINT('Ctrl Pts',(2.20609283085704,-1.21285462867864,2.53492272254882));
#21791=CARTESIAN_POINT('Ctrl Pts',(2.19627463015713,-1.23058850053314,2.53362080340586));
#21792=CARTESIAN_POINT('Ctrl Pts',(2.18998537718652,-1.24174648784717,2.53279297834645));
#21793=CARTESIAN_POINT('Ctrl Pts',(2.15819618128822,-1.29715211045029,2.52864078190378));
#21794=CARTESIAN_POINT('Ctrl Pts',(2.1314408507088,-1.34066156928266,2.5252471349779));
#21795=CARTESIAN_POINT('Ctrl Pts',(2.09086086841776,-1.4023645892814,2.52027059419372));
#21796=CARTESIAN_POINT('Ctrl Pts',(2.0780807328474,-1.42123398151892,2.51872567664879));
#21797=CARTESIAN_POINT('Ctrl Pts',(1.9516489097758,-1.60255402837902,2.5036721197753));
#21798=CARTESIAN_POINT('Ctrl Pts',(1.81941891068677,-1.75124001647328,2.48976241523873));
#21799=CARTESIAN_POINT('Ctrl Pts',(1.60717857832517,-1.93961095658286,2.4707071243353));
#21800=CARTESIAN_POINT('Ctrl Pts',(1.54039068661423,-1.99306622145591,2.46507782694509));
#21801=CARTESIAN_POINT('Ctrl Pts',(1.45357079845143,-2.05557771053364,2.45820069727876));
#21802=CARTESIAN_POINT('Ctrl Pts',(1.43597592865269,-2.06790738893567,2.45682820446374));
#21803=CARTESIAN_POINT('Ctrl Pts',(1.40914459195788,-2.08620194459258,2.454766484838));
#21804=CARTESIAN_POINT('Ctrl Pts',(1.40002369501289,-2.09233379131881,2.45407099804921));
#21805=CARTESIAN_POINT('Ctrl Pts',(1.38213431595182,-2.10419120814286,2.45271720478694));
#21806=CARTESIAN_POINT('Ctrl Pts',(1.37336969813707,-2.10992217518418,2.45205870628358));
#21807=CARTESIAN_POINT('Ctrl Pts',(1.35352424940092,-2.12272256961129,2.4505782673358));
#21808=CARTESIAN_POINT('Ctrl Pts',(1.34242324566254,-2.12976027786114,2.44975751034793));
#21809=CARTESIAN_POINT('Ctrl Pts',(1.312082295444,-2.14866406178501,2.44753378448082));
#21810=CARTESIAN_POINT('Ctrl Pts',(1.29273654710529,-2.16035864414496,2.44613706835385));
#21811=CARTESIAN_POINT('Ctrl Pts',(1.19033445768652,-2.22039294032427,2.43884968431189));
#21812=CARTESIAN_POINT('Ctrl Pts',(1.10471341295377,-2.26421117102594,2.43312190391391));
#21813=CARTESIAN_POINT('Ctrl Pts',(0.881776871053521,-2.36263772187843,
2.41885789239743));
#21814=CARTESIAN_POINT('Ctrl Pts',(0.741788212895067,-2.41025672169114,
2.410499205523));
#21815=CARTESIAN_POINT('Ctrl Pts',(0.502840146069942,-2.46873321046211,
2.39623996392119));
#21816=CARTESIAN_POINT('Ctrl Pts',(0.405965795160245,-2.48649944424717,
2.39045479294018));
#21817=CARTESIAN_POINT('Ctrl Pts',(0.287642158107969,-2.50110015553808,
2.38312350322353));
#21818=CARTESIAN_POINT('Ctrl Pts',(0.266942202756421,-2.50339405497751,
2.3818311401278));
#21819=CARTESIAN_POINT('Ctrl Pts',(0.237294140502355,-2.50630766795479,
2.37996307821561));
#21820=CARTESIAN_POINT('Ctrl Pts',(0.228366863623841,-2.50713685413932,
2.37939838393723));
#21821=CARTESIAN_POINT('Ctrl Pts',(0.212872054347985,-2.50849260457689,
2.37841414210315));
#21822=CARTESIAN_POINT('Ctrl Pts',(0.206306578213213,-2.50904110243012,
2.37799581121172));
#21823=CARTESIAN_POINT('Ctrl Pts',(0.192431466204484,-2.51014543749658,
2.37710891200246));
#21824=CARTESIAN_POINT('Ctrl Pts',(0.185121657013629,-2.51069511398835,
2.3766400354175));
#21825=CARTESIAN_POINT('Ctrl Pts',(0.16529551279393,-2.51209892969087,2.37536408230954));
#21826=CARTESIAN_POINT('Ctrl Pts',(0.152775217827282,-2.5128914334879,2.37455373897499));
#21827=CARTESIAN_POINT('Ctrl Pts',(0.0938036517867975,-2.51618184731973,
2.37071706728717));
#21828=CARTESIAN_POINT('Ctrl Pts',(0.0472978336248556,-2.51748535224016,
2.3676334598008));
#21829=CARTESIAN_POINT('Ctrl Pts',(-0.0326801620692364,-2.51751032836194,
2.36225978815277));
#21830=CARTESIAN_POINT('Ctrl Pts',(-0.0661422488160582,-2.51685345064351,
2.35999019430042));
#21831=CARTESIAN_POINT('Ctrl Pts',(-0.158656355707367,-2.51319117636813,
2.35367213343477));
#21832=CARTESIAN_POINT('Ctrl Pts',(-0.217630409161568,-2.50877228192166,
2.34959621137581));
#21833=CARTESIAN_POINT('Ctrl Pts',(-0.421969968780054,-2.48620171532827,
2.33539773304633));
#21834=CARTESIAN_POINT('Ctrl Pts',(-0.565881758997117,-2.45744660560747,
2.32528446112953));
#21835=CARTESIAN_POINT('Ctrl Pts',(-0.777886672193769,-2.39546078138107,
2.31053636865557));
#21836=CARTESIAN_POINT('Ctrl Pts',(-0.848331731333832,-2.37142892868546,
2.30565756632621));
#21837=CARTESIAN_POINT('Ctrl Pts',(-0.936788748871013,-2.33680487856067,
2.29955731608922));
#21838=CARTESIAN_POINT('Ctrl Pts',(-0.955869977998377,-2.32906479660331,
2.29824288430192));
#21839=CARTESIAN_POINT('Ctrl Pts',(-0.986608206230737,-2.31615479066974,
2.29612732356208));
#21840=CARTESIAN_POINT('Ctrl Pts',(-0.998324342961222,-2.31112900611374,
2.29532140373033));
#21841=CARTESIAN_POINT('Ctrl Pts',(-1.02073366110338,-2.30131403881312,
2.29378059853873));
#21842=CARTESIAN_POINT('Ctrl Pts',(-1.03143254653928,-2.29653879164617,
2.29304526647651));
#21843=CARTESIAN_POINT('Ctrl Pts',(-1.05583912131422,-2.28544040980704,
2.29136828208717));
#21844=CARTESIAN_POINT('Ctrl Pts',(-1.06952413915976,-2.27906828512441,
2.290428325836));
#21845=CARTESIAN_POINT('Ctrl Pts',(-1.11283251538259,-2.258426697421,2.28745409324779));
#21846=CARTESIAN_POINT('Ctrl Pts',(-1.1422347663941,-2.24369945543102,2.28543553149689));
#21847=CARTESIAN_POINT('Ctrl Pts',(-1.32860154522244,-2.14573720157006,
2.27262697284913));
#21848=CARTESIAN_POINT('Ctrl Pts',(-1.47667366616995,-2.04665918456801,
2.26243304464846));
#21849=CARTESIAN_POINT('Ctrl Pts',(-1.65754905267989,-1.89570313683784,
2.24889460737264));
#21850=CARTESIAN_POINT('Ctrl Pts',(-1.70071134221037,-1.85707832599156,
2.24556495494219));
#21851=CARTESIAN_POINT('Ctrl Pts',(-1.80856586604532,-1.75364589905302,
2.23687992568517));
#21852=CARTESIAN_POINT('Ctrl Pts',(-1.87111819856363,-1.6867417203143,2.23147851143386));
#21853=CARTESIAN_POINT('Ctrl Pts',(-1.9427993712315,-1.60116878295874,2.22460785718118));
#21854=CARTESIAN_POINT('Ctrl Pts',(-1.95553036612376,-1.58559509227524,
2.22335882250004));
#21855=CARTESIAN_POINT('Ctrl Pts',(-1.97358638854975,-1.56295911362746,
2.2215425848302));
#21856=CARTESIAN_POINT('Ctrl Pts',(-1.97906331578201,-1.55601825519887,
2.22098556684161));
#21857=CARTESIAN_POINT('Ctrl Pts',(-1.98854662789488,-1.54386907976749,
2.22001010261365));
#21858=CARTESIAN_POINT('Ctrl Pts',(-1.99256935934669,-1.53867370616994,
2.21959280891932));
#21859=CARTESIAN_POINT('Ctrl Pts',(-2.00107505419219,-1.52759927160628,
2.2187028849454));
#21860=CARTESIAN_POINT('Ctrl Pts',(-2.00555239651119,-1.52171629702125,
2.21822990897928));
#21861=CARTESIAN_POINT('Ctrl Pts',(-2.01772912772273,-1.50556967330009,
2.21693133246535));
#21862=CARTESIAN_POINT('Ctrl Pts',(-2.02537594427001,-1.49526691327455,
2.21610227185164));
#21863=CARTESIAN_POINT('Ctrl Pts',(-2.06231407211538,-1.44469596449026,
2.21203235766072));
#21864=CARTESIAN_POINT('Ctrl Pts',(-2.09048301872307,-1.40362593035789,
2.20872574789864));
#21865=CARTESIAN_POINT('Ctrl Pts',(-2.13362218567366,-1.33654799236901,
2.20335591003126));
#21866=CARTESIAN_POINT('Ctrl Pts',(-2.14937906118414,-1.31105823982704,
2.20132213576879));
#21867=CARTESIAN_POINT('Ctrl Pts',(-2.24317752538977,-1.15308401081435,
2.18878360959522));
#21868=CARTESIAN_POINT('Ctrl Pts',(-2.30940209313332,-1.01395913328513,
2.17804683246056));
#21869=CARTESIAN_POINT('Ctrl Pts',(-2.40157803687309,-0.76355264308214,
2.15986799611763));
#21870=CARTESIAN_POINT('Ctrl Pts',(-2.43344731706674,-0.654927420935664,
2.1523203673732));
#21871=CARTESIAN_POINT('Ctrl Pts',(-2.46393348524573,-0.517314352749194,
2.14320230937293));
#21872=CARTESIAN_POINT('Ctrl Pts',(-2.4695073822765,-0.490016071083766,
2.14141429813739));
#21873=CARTESIAN_POINT('Ctrl Pts',(-2.47725339657793,-0.44858231429324,
2.13873072238977));
#21874=CARTESIAN_POINT('Ctrl Pts',(-2.47975997619498,-0.434512321720601,
2.13782468434218));
#21875=CARTESIAN_POINT('Ctrl Pts',(-2.48408431912514,-0.408981626612012,
2.1361898918949));
#21876=CARTESIAN_POINT('Ctrl Pts',(-2.4859429006225,-0.39752833552041,2.13545987234389));
#21877=CARTESIAN_POINT('Ctrl Pts',(-2.48977345262704,-0.372844894953186,
2.13389363311997));
#21878=CARTESIAN_POINT('Ctrl Pts',(-2.4917193051178,-0.35961100728991,2.13305825326488));
#21879=CARTESIAN_POINT('Ctrl Pts',(-2.49670570123404,-0.323712511507988,
2.13080356723848));
#21880=CARTESIAN_POINT('Ctrl Pts',(-2.49954311498457,-0.301020627110442,
2.12939062384565));
#21881=CARTESIAN_POINT('Ctrl Pts',(-2.51292293332564,-0.180725474898618,
2.12196052162249));
#21882=CARTESIAN_POINT('Ctrl Pts',(-2.51805950468641,-0.0826007767955057,
2.11611379869366));
#21883=CARTESIAN_POINT('Ctrl Pts',(-2.51640684271091,0.184398799697227,
2.10049861623488));
#21884=CARTESIAN_POINT('Ctrl Pts',(-2.49838437356912,0.35267353641864,2.09099564336493));
#21885=CARTESIAN_POINT('Ctrl Pts',(-2.45178286763654,0.574369063215822,
2.07774655092478));
#21886=CARTESIAN_POINT('Ctrl Pts',(-2.4379681123593,0.630436107401488,2.07432776116495));
#21887=CARTESIAN_POINT('Ctrl Pts',(-2.41601911304895,0.707940006103002,
2.06944522669334));
#21888=CARTESIAN_POINT('Ctrl Pts',(-2.40950038628094,0.729818621248891,
2.06804918640699));
#21889=CARTESIAN_POINT('Ctrl Pts',(-2.39757866579965,0.767929266536848,
2.06558137170981));
#21890=CARTESIAN_POINT('Ctrl Pts',(-2.39230597874035,0.784200793257984,
2.06451611056507));
#21891=CARTESIAN_POINT('Ctrl Pts',(-2.38423478344372,0.808269351151879,
2.06292135123098));
#21892=CARTESIAN_POINT('Ctrl Pts',(-2.3815628068336,0.816108717694153,2.06239890335881));
#21893=CARTESIAN_POINT('Ctrl Pts',(-2.37692440372529,0.829500648675597,
2.06150100576316));
#21894=CARTESIAN_POINT('Ctrl Pts',(-2.37497709962775,0.835059711927412,
2.06112667664012));
#21895=CARTESIAN_POINT('Ctrl Pts',(-2.37050665545302,0.847679577014091,
2.06027318516354));
#21896=CARTESIAN_POINT('Ctrl Pts',(-2.36797152035159,0.85473583296209,2.05979333641508));
#21897=CARTESIAN_POINT('Ctrl Pts',(-2.36096669852877,0.873962584112031,
2.05847887269019));
#21898=CARTESIAN_POINT('Ctrl Pts',(-2.35643452509574,0.886109847590886,
2.05764074715221));
#21899=CARTESIAN_POINT('Ctrl Pts',(-2.33286132897366,0.947831445650328,
2.05334493348961));
#21900=CARTESIAN_POINT('Ctrl Pts',(-2.31235025908706,0.996825866338199,
2.04981228270863));
#21901=CARTESIAN_POINT('Ctrl Pts',(-2.19271862139852,1.25898746302094,2.03037003294219));
#21902=CARTESIAN_POINT('Ctrl Pts',(-2.06565605735625,1.45813438501692,2.01376501548297));
#21903=CARTESIAN_POINT('Ctrl Pts',(-1.86627400937068,1.69113728768919,1.99332074143289));
#21904=CARTESIAN_POINT('Ctrl Pts',(-1.81746338161314,1.74348860633243,1.98863398682015));
#21905=CARTESIAN_POINT('Ctrl Pts',(-1.75199737476513,1.80796152945558,1.98273508253423));
#21906=CARTESIAN_POINT('Ctrl Pts',(-1.73733744101811,1.8220533331468,1.98143732819238));
#21907=CARTESIAN_POINT('Ctrl Pts',(-1.71325185510255,1.84465048787923,1.97934192634097));
#21908=CARTESIAN_POINT('Ctrl Pts',(-1.70393000710769,1.8532646551153,1.97853965446623));
#21909=CARTESIAN_POINT('Ctrl Pts',(-1.68586570463759,1.86970606088125,1.97700143879645));
#21910=CARTESIAN_POINT('Ctrl Pts',(-1.67713291177885,1.87754337682993,1.97626508231531));
#21911=CARTESIAN_POINT('Ctrl Pts',(-1.65695066385073,1.89540292992624,1.97457966403325));
#21912=CARTESIAN_POINT('Ctrl Pts',(-1.64546443038492,1.90538305690609,1.97363235812494));
#21913=CARTESIAN_POINT('Ctrl Pts',(-1.60931320740998,1.93622330846879,1.97068704487632));
#21914=CARTESIAN_POINT('Ctrl Pts',(-1.58433616989097,1.95671376179668,1.96870398387053));
#21915=CARTESIAN_POINT('Ctrl Pts',(-1.41643741785449,2.0891298042913,1.95569370805038));
#21916=CARTESIAN_POINT('Ctrl Pts',(-1.26216234749102,2.18579810029513,1.94529339369489));
#21917=CARTESIAN_POINT('Ctrl Pts',(-0.964779236302288,2.33006474161138,
1.92629611392895));
#21918=CARTESIAN_POINT('Ctrl Pts',(-0.825251536674082,2.38305441452863,
1.91772907586008));
#21919=CARTESIAN_POINT('Ctrl Pts',(-0.664509321501718,2.42828320333141,
1.90742293460748));
#21920=CARTESIAN_POINT('Ctrl Pts',(-0.647085178356231,2.43298431616534,
1.90630005073643));
#21921=CARTESIAN_POINT('Ctrl Pts',(-0.621417936861451,2.43961423802894,
1.90463553940599));
#21922=CARTESIAN_POINT('Ctrl Pts',(-0.613212808720353,2.44168956441407,
1.90410188560876));
#21923=CARTESIAN_POINT('Ctrl Pts',(-0.598660870817896,2.44529221685999,
1.90315243871837));
#21924=CARTESIAN_POINT('Ctrl Pts',(-0.592318377344968,2.446836284385,1.90273760318398));
#21925=CARTESIAN_POINT('Ctrl Pts',(-0.578557602613034,2.45012967789807,
1.90183530145457));
#21926=CARTESIAN_POINT('Ctrl Pts',(-0.571137478273156,2.45186996297007,
1.90134735785356));
#21927=CARTESIAN_POINT('Ctrl Pts',(-0.550547143093724,2.45660059652816,
1.89998968360787));
#21928=CARTESIAN_POINT('Ctrl Pts',(-0.537360821711074,2.45951864719021,
1.89911606500862));
#21929=CARTESIAN_POINT('Ctrl Pts',(-0.464323692886314,2.47506593446538,
1.89425671650388));
#21930=CARTESIAN_POINT('Ctrl Pts',(-0.404056113338046,2.48561566169853,
1.89017140535845));
#21931=CARTESIAN_POINT('Ctrl Pts',(-0.166614283085535,2.51831632051453,
1.87392865789657));
#21932=CARTESIAN_POINT('Ctrl Pts',(0.0123314257865917,2.52379279430711,
1.86141194082279));
#21933=CARTESIAN_POINT('Ctrl Pts',(0.303536657573069,2.50171035598399,1.84156580002127));
#21934=CARTESIAN_POINT('Ctrl Pts',(0.416016816254641,2.48548295025079,1.83401891064894));
#21935=CARTESIAN_POINT('Ctrl Pts',(0.549665061238158,2.45687002296113,1.82521749442003));
#21936=CARTESIAN_POINT('Ctrl Pts',(0.572230907692743,2.45171242929946,1.82373684788367));
#21937=CARTESIAN_POINT('Ctrl Pts',(0.607651323746474,2.44310113136202,1.82142067829603));
#21938=CARTESIAN_POINT('Ctrl Pts',(0.620554678088349,2.43985556372956,1.82057858165271));
#21939=CARTESIAN_POINT('Ctrl Pts',(0.644668820239365,2.4335864818603,1.81900776961239));
#21940=CARTESIAN_POINT('Ctrl Pts',(0.655885544201494,2.43058742131456,1.81827829434706));
#21941=CARTESIAN_POINT('Ctrl Pts',(0.680956591931032,2.4236978840098,1.81665028929571));
#21942=CARTESIAN_POINT('Ctrl Pts',(0.694799186698213,2.41976598389132,1.81575311681268));
#21943=CARTESIAN_POINT('Ctrl Pts',(0.72994662999056,2.40945610145229,1.81347900279893));
#21944=CARTESIAN_POINT('Ctrl Pts',(0.751202345189274,2.4029140376617,1.81210736814316));
#21945=CARTESIAN_POINT('Ctrl Pts',(0.926328524891839,2.34646290467242,1.80083003319136));
#21946=CARTESIAN_POINT('Ctrl Pts',(1.07515375563884,2.28211010879423,1.79143139705414));
#21947=CARTESIAN_POINT('Ctrl Pts',(1.32536533555651,2.1439670883371,1.77498943707993));
#21948=CARTESIAN_POINT('Ctrl Pts',(1.42935576611394,2.076084475189,1.76792071678127));
#21949=CARTESIAN_POINT('Ctrl Pts',(1.56271786500049,1.97424334219929,1.75799770766925));
#21950=CARTESIAN_POINT('Ctrl Pts',(1.59682012413603,1.94676371574629,1.75537601467513));
#21951=CARTESIAN_POINT('Ctrl Pts',(1.65144744876503,1.90034365583597,1.7510040334261));
#21952=CARTESIAN_POINT('Ctrl Pts',(1.67240562112858,1.88192560305948,1.74928298156938));
#21953=CARTESIAN_POINT('Ctrl Pts',(1.70049587031815,1.85640006495595,1.74690900168537));
#21954=CARTESIAN_POINT('Ctrl Pts',(1.70789863090861,1.84959175620835,1.74627685303655));
#21955=CARTESIAN_POINT('Ctrl Pts',(1.72022783664916,1.83811547453024,1.74521263327353));
#21956=CARTESIAN_POINT('Ctrl Pts',(1.72517665395886,1.83347152104003,1.74478235360709));
#21957=CARTESIAN_POINT('Ctrl Pts',(1.7345468485722,1.82460703749317,1.74396157623113));
#21958=CARTESIAN_POINT('Ctrl Pts',(1.73897174212099,1.82039031236408,1.74357138101861));
#21959=CARTESIAN_POINT('Ctrl Pts',(1.7494596066996,1.81032271359423,1.74264043584657));
#21960=CARTESIAN_POINT('Ctrl Pts',(1.75550860141213,1.80445747757804,1.74209860725028));
#21961=CARTESIAN_POINT('Ctrl Pts',(1.77683732280253,1.78356793540415,1.74017106712188));
#21962=CARTESIAN_POINT('Ctrl Pts',(1.7919540507707,1.76837950116006,1.73877363762351));
#21963=CARTESIAN_POINT('Ctrl Pts',(1.89755823187141,1.6595298514891,1.72879911891637));
#21964=CARTESIAN_POINT('Ctrl Pts',(1.98084395722714,1.55917202082583,1.71982091729261));
#21965=CARTESIAN_POINT('Ctrl Pts',(2.12265427685906,1.35848848506777,1.70284528725198));
#21966=CARTESIAN_POINT('Ctrl Pts',(2.18275402492497,1.25965886273768,1.69487041119613));
#21967=CARTESIAN_POINT('Ctrl Pts',(2.28013283157017,1.07148562326009,1.68057143425173));
#21968=CARTESIAN_POINT('Ctrl Pts',(2.31946612684565,0.983446993081237,1.67420304161951));
#21969=CARTESIAN_POINT('Ctrl Pts',(2.35627749479815,0.886463218134093,1.66752945036158));
#21970=CARTESIAN_POINT('Ctrl Pts',(2.35886495348818,0.879554887728603,1.66705586916765));
#21971=CARTESIAN_POINT('Ctrl Pts',(2.36142200724207,0.872635292497862,1.66658329180866));
#21972=CARTESIAN_POINT('Origin',(0.,0.,10.));
#21973=CARTESIAN_POINT('',(2.36142199806814,0.872635317323264,0.66916271832655));
#21974=CARTESIAN_POINT('',(2.36142200728636,0.872635292378021,0.943739684385603));
#21975=CARTESIAN_POINT('',(2.36142200728636,0.87263529237802,10.));
#21976=CARTESIAN_POINT('',(2.51749944581752,0.00167042164863851,0.612583302452829));
#21977=CARTESIAN_POINT('Ctrl Pts',(2.36142199806814,0.872635317323264,0.66916271832655));
#21978=CARTESIAN_POINT('Ctrl Pts',(2.37681768646397,0.830973334898781,0.666612244616638));
#21979=CARTESIAN_POINT('Ctrl Pts',(2.39111080605859,0.788903976832428,0.664061088185206));
#21980=CARTESIAN_POINT('Ctrl Pts',(2.42299547018568,0.686207656059237,0.657849231643885));
#21981=CARTESIAN_POINT('Ctrl Pts',(2.4394324974691,0.62526498961167,0.654176172148787));
#21982=CARTESIAN_POINT('Ctrl Pts',(2.46633440053622,0.508186762100082,0.647039638474432));
#21983=CARTESIAN_POINT('Ctrl Pts',(2.47721305089561,0.452187545013459,0.643591919008456));
#21984=CARTESIAN_POINT('Ctrl Pts',(2.48825441667045,0.382844904997875,0.639227439169845));
#21985=CARTESIAN_POINT('Ctrl Pts',(2.49022626481964,0.369801833019874,0.638402376229968));
#21986=CARTESIAN_POINT('Ctrl Pts',(2.49316143652721,0.34929770678135,0.637098032199428));
#21987=CARTESIAN_POINT('Ctrl Pts',(2.49419400660206,0.341846589068485,0.636622524686075));
#21988=CARTESIAN_POINT('Ctrl Pts',(2.49597303807743,0.328571631908365,0.63577248368067));
#21989=CARTESIAN_POINT('Ctrl Pts',(2.4967325409946,0.322749655427988,0.635398687562037));
#21990=CARTESIAN_POINT('Ctrl Pts',(2.49826595554394,0.310665857198052,0.634620831734606));
#21991=CARTESIAN_POINT('Ctrl Pts',(2.49903670379824,0.304403696526905,0.634216604903073));
#21992=CARTESIAN_POINT('Ctrl Pts',(2.50074151733824,0.290109463030347,0.633291448180771));
#21993=CARTESIAN_POINT('Ctrl Pts',(2.50166043510509,0.282075699662491,0.632769718083427));
#21994=CARTESIAN_POINT('Ctrl Pts',(2.50391801978371,0.261459208743697,0.631426548146041));
#21995=CARTESIAN_POINT('Ctrl Pts',(2.5052005339591,0.248870724191182,0.630602311351134));
#21996=CARTESIAN_POINT('Ctrl Pts',(2.51374345548572,0.158247419999016,0.624641789388791));
#21997=CARTESIAN_POINT('Ctrl Pts',(2.5174505050648,0.0799288784532003,0.619348271840614));
#21998=CARTESIAN_POINT('Ctrl Pts',(2.51749950767651,0.00157443594625835,
0.613985814047302));
#21999=CARTESIAN_POINT('',(-1.91346599666507,1.63598720337494,0.));
#22000=CARTESIAN_POINT('Ctrl Pts',(2.51749944581752,0.00167042164863862,
0.61258330245283));
#22001=CARTESIAN_POINT('Ctrl Pts',(2.51755363606023,-0.0799999195505381,
0.607399299002986));
#22002=CARTESIAN_POINT('Ctrl Pts',(2.5136294010915,-0.161821619082909,0.602215295553139));
#22003=CARTESIAN_POINT('Ctrl Pts',(2.50570901083512,-0.243369272957164,
0.597031292103296));
#22004=CARTESIAN_POINT('Ctrl Pts',(2.49779912369791,-0.324808787623776,
0.591854163088201));
#22005=CARTESIAN_POINT('Ctrl Pts',(2.48590365394244,-0.405974509605015,
0.586677034073107));
#22006=CARTESIAN_POINT('Ctrl Pts',(2.47005689828212,-0.486441331764581,
0.581499905058012));
#22007=CARTESIAN_POINT('Ctrl Pts',(2.45422172607578,-0.566849335340019,
0.576326560352901));
#22008=CARTESIAN_POINT('Ctrl Pts',(2.43444108857363,-0.646558988738404,
0.571153215647791));
#22009=CARTESIAN_POINT('Ctrl Pts',(2.41080092412554,-0.725151814612256,
0.56597987094268));
#22010=CARTESIAN_POINT('Ctrl Pts',(2.38717046687464,-0.803712368457708,
0.560808650532318));
#22011=CARTESIAN_POINT('Ctrl Pts',(2.35968376436198,-0.881156551101217,
0.555637430121958));
#22012=CARTESIAN_POINT('Ctrl Pts',(2.32847715353194,-0.957079095728153,
0.550466209711596));
#22013=CARTESIAN_POINT('Ctrl Pts',(2.29727336091083,-1.03299478393624,0.545295456304193));
#22014=CARTESIAN_POINT('Ctrl Pts',(2.26235050879355,-1.10738866876217,0.540124702896787));
#22015=CARTESIAN_POINT('Ctrl Pts',(2.22389323148074,-1.17987505481477,0.534953949489385));
#22016=CARTESIAN_POINT('Ctrl Pts',(2.18540220370415,-1.25242505559305,0.529778658180765));
#22017=CARTESIAN_POINT('Ctrl Pts',(2.1433707776255,-1.32306379366159,0.524603366872146));
#22018=CARTESIAN_POINT('Ctrl Pts',(2.09802942378302,-1.39143048225224,0.519428075563527));
#22019=CARTESIAN_POINT('Ctrl Pts',(2.05266856488632,-1.45982658099178,0.514250557935464));
#22020=CARTESIAN_POINT('Ctrl Pts',(2.00399522499661,-1.52594830190349,0.509073040307402));
#22021=CARTESIAN_POINT('Ctrl Pts',(1.95228156389339,-1.58946624540504,0.50389552267934));
#22022=CARTESIAN_POINT('Ctrl Pts',(1.90048050967036,-1.65309153058629,0.498709255343585));
#22023=CARTESIAN_POINT('Ctrl Pts',(1.84562918976615,-1.71410389642268,0.493522988007832));
#22024=CARTESIAN_POINT('Ctrl Pts',(1.78803790317884,-1.77220955498943,0.488336720672077));
#22025=CARTESIAN_POINT('Ctrl Pts',(1.73906674416392,-1.8216180960024,0.483926721565561));
#22026=CARTESIAN_POINT('Ctrl Pts',(1.68811520655394,-1.86892548692704,0.479516722459043));
#22027=CARTESIAN_POINT('Ctrl Pts',(1.63539196861162,-1.91397475401339,0.475106723352527));
#22028=CARTESIAN_POINT('Ctrl Pts',(1.57247470805091,-1.96773428370012,0.469844052210049));
#22029=CARTESIAN_POINT('Ctrl Pts',(1.50679114174476,-2.01848444144763,0.464581381067567));
#22030=CARTESIAN_POINT('Ctrl Pts',(1.43866062696852,-2.0659288105863,0.459318709925087));
#22031=CARTESIAN_POINT('Ctrl Pts',(1.37062496764678,-2.11330712478304,0.454063365794076));
#22032=CARTESIAN_POINT('Ctrl Pts',(1.30014950174808,-2.15738853258599,0.448808021663067));
#22033=CARTESIAN_POINT('Ctrl Pts',(1.22758734420499,-2.19791618637921,0.443552677532056));
#22034=CARTESIAN_POINT('Ctrl Pts',(1.15463018095667,-2.23866446005214,0.438268724950235));
#22035=CARTESIAN_POINT('Ctrl Pts',(1.07956389471693,-2.27581986235599,0.432984772368411));
#22036=CARTESIAN_POINT('Ctrl Pts',(1.00277781621867,-2.30916497922944,0.42770081978659));
#22037=CARTESIAN_POINT('Ctrl Pts',(0.926540176764554,-2.3422719310034,0.422454607456127));
#22038=CARTESIAN_POINT('Ctrl Pts',(0.848607660651047,-2.37162266619502,
0.417208395125666));
#22039=CARTESIAN_POINT('Ctrl Pts',(0.769385240476353,-2.39705081334067,
0.411962182795202));
#22040=CARTESIAN_POINT('Ctrl Pts',(0.690187749994883,-2.42247095876274,
0.406717621341645));
#22041=CARTESIAN_POINT('Ctrl Pts',(0.609701599172221,-2.44397082749234,
0.401473059888088));
#22042=CARTESIAN_POINT('Ctrl Pts',(0.528348914803874,-2.46143325609807,
0.396228498434532));
#22043=CARTESIAN_POINT('Ctrl Pts',(0.446997505831167,-2.47889541093896,
0.390984019201874));
#22044=CARTESIAN_POINT('Ctrl Pts',(0.364780040117444,-2.49232015610874,
0.385739539969215));
#22045=CARTESIAN_POINT('Ctrl Pts',(0.282129543584915,-2.50164129535722,
0.380495060736557));
#22046=CARTESIAN_POINT('Ctrl Pts',(0.198397557100848,-2.51108440263805,
0.37518195697254));
#22047=CARTESIAN_POINT('Ctrl Pts',(0.114221603733744,-2.516315660127,0.369868853208523));
#22048=CARTESIAN_POINT('Ctrl Pts',(0.0300561933397463,-2.51732057458758,
0.364555749444506));
#22049=CARTESIAN_POINT('Ctrl Pts',(-0.0531422727847476,-2.51831394396955,
0.359303685901333));
#22050=CARTESIAN_POINT('Ctrl Pts',(-0.136329974024215,-2.51517766013747,
0.35405162235816));
#22051=CARTESIAN_POINT('Ctrl Pts',(-0.219070760971157,-2.50795020917233,
0.348799558814987));
#22052=CARTESIAN_POINT('Ctrl Pts',(-0.303253985504742,-2.50059676053043,
0.343455934940547));
#22053=CARTESIAN_POINT('Ctrl Pts',(-0.386974071543444,-2.48900820957633,
0.338112311066108));
#22054=CARTESIAN_POINT('Ctrl Pts',(-0.469782010250341,-2.47327942474059,
0.332768687191669));
#22055=CARTESIAN_POINT('Ctrl Pts',(-0.552589948957238,-2.45755063990485,
0.327425063317229));
#22056=CARTESIAN_POINT('Ctrl Pts',(-0.634485275099095,-2.43768180027533,
0.322081439442788));
#22057=CARTESIAN_POINT('Ctrl Pts',(-0.715036549887057,-2.41382041219425,
0.316737815568349));
#22058=CARTESIAN_POINT('Ctrl Pts',(-0.793400342988758,-2.39060701323034,
0.311539305218113));
#22059=CARTESIAN_POINT('Ctrl Pts',(-0.870795262975601,-2.36352519602271,
0.306340794867879));
#22060=CARTESIAN_POINT('Ctrl Pts',(-0.946806110785062,-2.33267323870706,
0.301142284517644));
#22061=CARTESIAN_POINT('Ctrl Pts',(-1.0227074740887,-2.30186571993403,0.295951261997806));
#22062=CARTESIAN_POINT('Ctrl Pts',(-1.09722828924589,-2.26729901643482,
0.290760239477968));
#22063=CARTESIAN_POINT('Ctrl Pts',(-1.16996737546248,-2.22912148398275,
0.28556921695813));
#22064=CARTESIAN_POINT('Ctrl Pts',(-1.24423368667912,-2.19014237860704,
0.280269204075882));
#22065=CARTESIAN_POINT('Ctrl Pts',(-1.31664211485637,-2.14739921831778,
0.274969191193632));
#22066=CARTESIAN_POINT('Ctrl Pts',(-1.38678620559988,-2.10110215600239,
0.269669178311384));
#22067=CARTESIAN_POINT('Ctrl Pts',(-1.455367490382,-2.05583658934422,0.264487249385175));
#22068=CARTESIAN_POINT('Ctrl Pts',(-1.5217838796265,-2.00717412159218,0.259305320458967));
#22069=CARTESIAN_POINT('Ctrl Pts',(-1.58568124356746,-1.95535706299344,
0.254123391532758));
#22070=CARTESIAN_POINT('Ctrl Pts',(-1.64955996115625,-1.90355512550556,
0.24894297478273));
#22071=CARTESIAN_POINT('Ctrl Pts',(-1.71092074568316,-1.84860072127404,
0.243762558032702));
#22072=CARTESIAN_POINT('Ctrl Pts',(-1.76944123177445,-1.7907774784424,0.238582141282674));
#22073=CARTESIAN_POINT('Ctrl Pts',(-1.82796321126342,-1.73295276000619,
0.233401592332405));
#22074=CARTESIAN_POINT('Ctrl Pts',(-1.88364441326875,-1.67225939038837,
0.228221043382138));
#22075=CARTESIAN_POINT('Ctrl Pts',(-1.93619925700975,-1.60901792630004,
0.223040494431869));
#22076=CARTESIAN_POINT('Ctrl Pts',(-1.99087179530924,-1.54322815086992,
0.217651195544561));
#22077=CARTESIAN_POINT('Ctrl Pts',(-2.04216031683337,-1.4746809957138,0.212261896657254));
#22078=CARTESIAN_POINT('Ctrl Pts',(-2.08979094478388,-1.403773506339,0.206872597769946));
#22079=CARTESIAN_POINT('Ctrl Pts',(-2.13565388919363,-1.33549755904706,
0.201683308316679));
#22080=CARTESIAN_POINT('Ctrl Pts',(-2.17812547157535,-1.26503383316533,
0.196494018863409));
#22081=CARTESIAN_POINT('Ctrl Pts',(-2.21700767034701,-1.19276285975986,
0.191304729410142));
#22082=CARTESIAN_POINT('Ctrl Pts',(-2.25592163863668,-1.12043283583607,
0.186111199938822));
#22083=CARTESIAN_POINT('Ctrl Pts',(-2.2912401921896,-1.04629305424291,0.180917670467504));
#22084=CARTESIAN_POINT('Ctrl Pts',(-2.32281343696738,-0.970744037861583,
0.175724140996184));
#22085=CARTESIAN_POINT('Ctrl Pts',(-2.35444103009835,-0.895064975783177,
0.170521671684311));
#22086=CARTESIAN_POINT('Ctrl Pts',(-2.38231030568149,-0.81797228520106,
0.165319202372439));
#22087=CARTESIAN_POINT('Ctrl Pts',(-2.40632137520468,-0.739880861512898,
0.160116733060566));
#22088=CARTESIAN_POINT('Ctrl Pts',(-2.40901030051494,-0.731135644834104,
0.159534124635103));
#22089=CARTESIAN_POINT('Ctrl Pts',(-2.4116508929402,-0.722377911375065,
0.158951516209639));
#22090=CARTESIAN_POINT('Ctrl Pts',(-2.41424305246311,-0.71360824941532,
0.158368907784176));
#22091=CARTESIAN_POINT('Ctrl Pts',(-2.43827539171481,-0.63230326433367,
0.152967448804556));
#22092=CARTESIAN_POINT('Ctrl Pts',(-2.45823257024162,-0.549660683368054,
0.147565989824935));
#22093=CARTESIAN_POINT('Ctrl Pts',(-2.47397350173628,-0.466113036405061,
0.142164530845315));
#22094=CARTESIAN_POINT('Ctrl Pts',(-2.48968971854399,-0.38269656680855,
0.136771552645105));
#22095=CARTESIAN_POINT('Ctrl Pts',(-2.50120277584277,-0.298378277521893,
0.131378574444896));
#22096=CARTESIAN_POINT('Ctrl Pts',(-2.50842167175663,-0.213604697190072,
0.125985596244686));
#22097=CARTESIAN_POINT('Ctrl Pts',(-2.51562919183355,-0.128964706598124,
0.120601116524215));
#22098=CARTESIAN_POINT('Ctrl Pts',(-2.51855598739321,-0.0438712799426537,
0.115216636803746));
#22099=CARTESIAN_POINT('Ctrl Pts',(-2.51716249945789,0.0412213697360415,
0.109832157083275));
#22100=CARTESIAN_POINT('Ctrl Pts',(-2.51577030759958,0.126234875114859,
0.104452685443753));
#22101=CARTESIAN_POINT('Ctrl Pts',(-2.51006582998477,0.211247176543093,
0.0990732138042305));
#22102=CARTESIAN_POINT('Ctrl Pts',(-2.50006149470586,0.295801914613631,
0.0936937421647084));
#22103=CARTESIAN_POINT('Ctrl Pts',(-2.49006408324414,0.380298133898865,
0.0883179935589642));
#22104=CARTESIAN_POINT('Ctrl Pts',(-2.4757727839072,0.464336993480074,0.0829422449532235));
#22105=CARTESIAN_POINT('Ctrl Pts',(-2.45725194307627,0.547466106939874,
0.0775664963474796));
#22106=CARTESIAN_POINT('Ctrl Pts',(-2.43873951628433,0.630557454749165,
0.0721931899504231));
#22107=CARTESIAN_POINT('Ctrl Pts',(-2.41600146512598,0.712739459447074,
0.0668198835533652));
#22108=CARTESIAN_POINT('Ctrl Pts',(-2.38915325197096,0.793569775505975,
0.0614465771563086));
#22109=CARTESIAN_POINT('Ctrl Pts',(-2.36230312891944,0.874405841576472,
0.0560728885193252));
#22110=CARTESIAN_POINT('Ctrl Pts',(-2.33134238550205,0.953889615212508,
0.050699199882339));
#22111=CARTESIAN_POINT('Ctrl Pts',(-2.29643622565225,1.03159435414898,0.0453255112453554));
#22112=CARTESIAN_POINT('Ctrl Pts',(-2.26153094627027,1.10929713307259,0.0399519581535011));
#22113=CARTESIAN_POINT('Ctrl Pts',(-2.22268063027161,1.18522057628461,0.034578405061647));
#22114=CARTESIAN_POINT('Ctrl Pts',(-2.18009787371179,1.25895969396853,0.0292048519697925));
#22115=CARTESIAN_POINT('Ctrl Pts',(-2.13748475845543,1.3327513827793,0.0238274678890403));
#22116=CARTESIAN_POINT('Ctrl Pts',(-2.09113410476751,1.40435526322514,0.018450083808286));
#22117=CARTESIAN_POINT('Ctrl Pts',(-2.04130338933839,1.47339292881282,0.0130726997275339));
#22118=CARTESIAN_POINT('Ctrl Pts',(-2.00092303771321,1.52933764459313,0.00871513315168901));
#22119=CARTESIAN_POINT('Ctrl Pts',(-1.95825834189446,1.58359765574858,0.00435756657584321));
#22120=CARTESIAN_POINT('Ctrl Pts',(-1.91346599666507,1.63598720337494,-1.77635683940025E-15));
#22121=CARTESIAN_POINT('',(1.91360977481672,1.63581902413619,1.65132641005705E-6));
#22122=CARTESIAN_POINT('Origin',(0.,0.,0.));
#22123=CARTESIAN_POINT('',(2.51749949188307,0.00159949006993195,0.887416697568047));
#22124=CARTESIAN_POINT('Ctrl Pts',(1.91360977481672,1.63581902413619,1.65132641072319E-6));
#22125=CARTESIAN_POINT('Ctrl Pts',(1.86009423852759,1.69842243676096,0.00523991872577366));
#22126=CARTESIAN_POINT('Ctrl Pts',(1.80340192327242,1.7585155596962,0.0104781861251362));
#22127=CARTESIAN_POINT('Ctrl Pts',(1.74379813375851,1.81575723011099,0.0157164535244991));
#22128=CARTESIAN_POINT('Ctrl Pts',(1.68427848419545,1.87291809507072,0.0209473263007164));
#22129=CARTESIAN_POINT('Ctrl Pts',(1.62185585512159,1.92723518240283,0.0261781990769335));
#22130=CARTESIAN_POINT('Ctrl Pts',(1.55683525052212,1.97840093326195,0.031409071853151));
#22131=CARTESIAN_POINT('Ctrl Pts',(1.49188840291163,2.02950864356998,0.0366340109191525));
#22132=CARTESIAN_POINT('Ctrl Pts',(1.4243497999245,2.07747183574107,0.0418589499851537));
#22133=CARTESIAN_POINT('Ctrl Pts',(1.35455959449404,2.12202133706618,0.0470838890511551));
#22134=CARTESIAN_POINT('Ctrl Pts',(1.28481247118473,2.16654333758367,0.0523056027153035));
#22135=CARTESIAN_POINT('Ctrl Pts',(1.2128168951504,2.20765558081316,0.0575273163794534));
#22136=CARTESIAN_POINT('Ctrl Pts',(1.13894330276347,2.24513126633839,0.0627490300436016));
#22137=CARTESIAN_POINT('Ctrl Pts',(1.06509264495393,2.28259531727295,0.0679691225899423));
#22138=CARTESIAN_POINT('Ctrl Pts',(0.989365542862862,2.31642484251573,0.0731892151362824));
#22139=CARTESIAN_POINT('Ctrl Pts',(0.912157161652249,2.34643891087037,0.0784093076826231));
#22140=CARTESIAN_POINT('Ctrl Pts',(0.834949059074677,2.3764528709089,0.0836293813904616));
#22141=CARTESIAN_POINT('Ctrl Pts',(0.756260121759999,2.40265123454484,0.0888494550983027));
#22142=CARTESIAN_POINT('Ctrl Pts',(0.676504282709394,2.42490168985793,0.0940695288061413));
#22143=CARTESIAN_POINT('Ctrl Pts',(0.596671652308013,2.44717356858702,0.0992946285599214));
#22144=CARTESIAN_POINT('Ctrl Pts',(0.515770517139345,2.46548982200541,0.104519728313704));
#22145=CARTESIAN_POINT('Ctrl Pts',(0.434228159148547,2.47976856900044,0.109744828067484));
#22146=CARTESIAN_POINT('Ctrl Pts',(0.352646405999318,2.49405421441628,0.114972452198014));
#22147=CARTESIAN_POINT('Ctrl Pts',(0.270423274645153,2.50429841098978,0.120200076328541));
#22148=CARTESIAN_POINT('Ctrl Pts',(0.187991931561763,2.51047112782993,0.12542770045907));
#22149=CARTESIAN_POINT('Ctrl Pts',(0.105419192746191,2.51665443282484,0.130664291612505));
#22150=CARTESIAN_POINT('Ctrl Pts',(0.0226379940687081,2.51875229510584,
0.135900882765937));
#22151=CARTESIAN_POINT('Ctrl Pts',(-0.059917986517188,2.51678685726299,
0.141137473919372));
#22152=CARTESIAN_POINT('Ctrl Pts',(-0.128036847781654,2.5151651287487,0.145458307173946));
#22153=CARTESIAN_POINT('Ctrl Pts',(-0.196002288236653,2.51077797126332,
0.149779140428521));
#22154=CARTESIAN_POINT('Ctrl Pts',(-0.263574933994023,2.50366421553891,
0.154099973683095));
#22155=CARTESIAN_POINT('Ctrl Pts',(-0.345901347362564,2.49499724700738,
0.159364214865687));
#22156=CARTESIAN_POINT('Ctrl Pts',(-0.427945869163083,2.48224998394257,
0.16462845604828));
#22157=CARTESIAN_POINT('Ctrl Pts',(-0.509273485255483,2.46545062153265,
0.169892697230871));
#22158=CARTESIAN_POINT('Ctrl Pts',(-0.590488851465099,2.44867444591403,
0.175149672610233));
#22159=CARTESIAN_POINT('Ctrl Pts',(-0.670988831084925,2.42785737344303,
0.180406647989593));
#22160=CARTESIAN_POINT('Ctrl Pts',(-0.750343951568759,2.40307931711464,
0.185663623368955));
#22161=CARTESIAN_POINT('Ctrl Pts',(-0.830100257938074,2.37817599342596,
0.190947175789718));
#22162=CARTESIAN_POINT('Ctrl Pts',(-0.908699628614368,2.34927157097849,
0.196230728210483));
#22163=CARTESIAN_POINT('Ctrl Pts',(-0.985716841942823,2.3164992030023,0.201514280631246));
#22164=CARTESIAN_POINT('Ctrl Pts',(-1.06221560148537,2.2839474475037,0.206762265967234));
#22165=CARTESIAN_POINT('Ctrl Pts',(-1.13715301185763,2.24757984596568,0.212010251303225));
#22166=CARTESIAN_POINT('Ctrl Pts',(-1.21012965718489,2.20757615107647,0.217258236639212));
#22167=CARTESIAN_POINT('Ctrl Pts',(-1.28308404635457,2.16758465637175,0.222504621463309));
#22168=CARTESIAN_POINT('Ctrl Pts',(-1.35407845556301,2.1239594917239,0.227751006287403));
#22169=CARTESIAN_POINT('Ctrl Pts',(-1.42273741331739,2.07692669652709,0.2329973911115));
#22170=CARTESIAN_POINT('Ctrl Pts',(-1.49139593290246,2.02989420148526,0.238243742454098));
#22171=CARTESIAN_POINT('Ctrl Pts',(-1.55771865220263,1.9794543798231,0.243490093796699));
#22172=CARTESIAN_POINT('Ctrl Pts',(-1.62135961873937,1.92587622570126,0.248736445139297));
#22173=CARTESIAN_POINT('Ctrl Pts',(-1.68578524814015,1.87163747840884,0.254047481499962));
#22174=CARTESIAN_POINT('Ctrl Pts',(-1.74746216178544,1.81418277684423,0.259358517860623));
#22175=CARTESIAN_POINT('Ctrl Pts',(-1.8060678899512,1.75383152750976,0.264669554221287));
#22176=CARTESIAN_POINT('Ctrl Pts',(-1.86404468745398,1.69412794099672,0.26992359489699));
#22177=CARTESIAN_POINT('Ctrl Pts',(-1.91901564041973,1.63159006804883,0.275177635572696));
#22178=CARTESIAN_POINT('Ctrl Pts',(-1.97070862699392,1.56656112472247,0.2804316762484));
#22179=CARTESIAN_POINT('Ctrl Pts',(-2.0232427596572,1.50047403318335,0.285771210451545));
#22180=CARTESIAN_POINT('Ctrl Pts',(-2.07239100817816,1.43181448141849,0.291110744654691));
#22181=CARTESIAN_POINT('Ctrl Pts',(-2.11791413260419,1.36097243797053,0.296450278857836));
#22182=CARTESIAN_POINT('Ctrl Pts',(-2.16343725703023,1.29013039452256,0.301789813060982));
#22183=CARTESIAN_POINT('Ctrl Pts',(-2.20533506873481,1.21710631747659,0.307129347264126));
#22184=CARTESIAN_POINT('Ctrl Pts',(-2.24341839400878,1.14231351187976,0.312468881467272));
#22185=CARTESIAN_POINT('Ctrl Pts',(-2.28085037427587,1.06879989921385,0.317717092790461));
#22186=CARTESIAN_POINT('Ctrl Pts',(-2.31473604611418,0.993305135517561,
0.32296530411365));
#22187=CARTESIAN_POINT('Ctrl Pts',(-2.34486098057096,0.916205889413401,
0.32821351543684));
#22188=CARTESIAN_POINT('Ctrl Pts',(-2.37494258213299,0.839217545907933,
0.333454177525716));
#22189=CARTESIAN_POINT('Ctrl Pts',(-2.40127402338612,0.760629731212215,
0.338694839614592));
#22190=CARTESIAN_POINT('Ctrl Pts',(-2.42368708901712,0.680842966132206,
0.343935501703468));
#22191=CARTESIAN_POINT('Ctrl Pts',(-2.44630087689435,0.600341663426275,
0.349223097017967));
#22192=CARTESIAN_POINT('Ctrl Pts',(-2.46492552564214,0.518620248947559,
0.354510692332466));
#22193=CARTESIAN_POINT('Ctrl Pts',(-2.47943830443195,0.436110014234484,
0.359798287646965));
#22194=CARTESIAN_POINT('Ctrl Pts',(-2.49379602217835,0.354481355908151,
0.365029387919509));
#22195=CARTESIAN_POINT('Ctrl Pts',(-2.50412923353572,0.272081119207604,
0.370260488192053));
#22196=CARTESIAN_POINT('Ctrl Pts',(-2.51036984617185,0.189339603440867,
0.375491588464596));
#22197=CARTESIAN_POINT('Ctrl Pts',(-2.51660833788702,0.106626208024527,
0.380720910906854));
#22198=CARTESIAN_POINT('Ctrl Pts',(-2.51875695823721,0.0235722250301544,
0.38595023334911));
#22199=CARTESIAN_POINT('Ctrl Pts',(-2.516799449759,-0.0593866962608646,
0.391179555791368));
#22200=CARTESIAN_POINT('Ctrl Pts',(-2.51484201164508,-0.142342635523984,
0.396408690261251));
#22201=CARTESIAN_POINT('Ctrl Pts',(-2.50877875002578,-0.225203057176136,
0.401637824731133));
#22202=CARTESIAN_POINT('Ctrl Pts',(-2.49864551292181,-0.307533495339446,
0.406866959201016));
#22203=CARTESIAN_POINT('Ctrl Pts',(-2.48831506543297,-0.391466226751247,
0.412197861705219));
#22204=CARTESIAN_POINT('Ctrl Pts',(-2.47375459029873,-0.474847629671242,
0.417528764209423));
#22205=CARTESIAN_POINT('Ctrl Pts',(-2.45505711055919,-0.557226016884306,
0.422859666713626));
#22206=CARTESIAN_POINT('Ctrl Pts',(-2.43669032389862,-0.638147418295674,
0.428096284181162));
#22207=CARTESIAN_POINT('Ctrl Pts',(-2.41433187505233,-0.71810056085767,
0.433332901648697));
#22208=CARTESIAN_POINT('Ctrl Pts',(-2.38812046829166,-0.796672378664167,
0.438569519116234));
#22209=CARTESIAN_POINT('Ctrl Pts',(-2.3612011589213,-0.87736621896955,0.443947564138769));
#22210=CARTESIAN_POINT('Ctrl Pts',(-2.33021796121626,-0.956602555970598,
0.449325609161306));
#22211=CARTESIAN_POINT('Ctrl Pts',(-2.29537319685894,-1.03395751225162,
0.454703654183842));
#22212=CARTESIAN_POINT('Ctrl Pts',(-2.26052843250163,-1.11131246853263,
0.460081699206377));
#22213=CARTESIAN_POINT('Ctrl Pts',(-2.22182240094526,-1.18678561188465,
0.465459744228912));
#22214=CARTESIAN_POINT('Ctrl Pts',(-2.17950621167997,-1.25998369959632,
0.470837789251448));
#22215=CARTESIAN_POINT('Ctrl Pts',(-2.13814395334591,-1.33153168787354,
0.476094597376578));
#22216=CARTESIAN_POINT('Ctrl Pts',(-2.09317876908886,-1.40117236950367,
0.481351405501709));
#22217=CARTESIAN_POINT('Ctrl Pts',(-2.04481161312267,-1.46852024733698,
0.486608213626839));
#22218=CARTESIAN_POINT('Ctrl Pts',(-1.99651294033756,-1.53577276713608,
0.491857578623765));
#22219=CARTESIAN_POINT('Ctrl Pts',(-1.94482213045194,-1.60073856010646,
0.497106943620689));
#22220=CARTESIAN_POINT('Ctrl Pts',(-1.88998522071329,-1.66305806136928,
0.502356308617614));
#22221=CARTESIAN_POINT('Ctrl Pts',(-1.83477153213647,-1.72580575359677,
0.507641741468364));
#22222=CARTESIAN_POINT('Ctrl Pts',(-1.77636857449826,-1.7858702340872,0.512927174319118));
#22223=CARTESIAN_POINT('Ctrl Pts',(-1.71507102163768,-1.84291552729329,
0.518212607169868));
#22224=CARTESIAN_POINT('Ctrl Pts',(-1.65430038653143,-1.89947045544582,
0.523452606095797));
#22225=CARTESIAN_POINT('Ctrl Pts',(-1.5906850726739,-1.95305758349209,0.528692605021722));
#22226=CARTESIAN_POINT('Ctrl Pts',(-1.52455035578429,-2.00338525068894,
0.533932603947651));
#22227=CARTESIAN_POINT('Ctrl Pts',(-1.45843739621914,-2.05369636084229,
0.539170878992959));
#22228=CARTESIAN_POINT('Ctrl Pts',(-1.38980704643993,-2.1007498608487,0.54440915403827));
#22229=CARTESIAN_POINT('Ctrl Pts',(-1.31901721811137,-2.1442947158275,0.549647429083578));
#22230=CARTESIAN_POINT('Ctrl Pts',(-1.24822936107416,-2.18783835820842,
0.554885558258122));
#22231=CARTESIAN_POINT('Ctrl Pts',(-1.1752825383405,-2.22787330911488,0.560123687432665));
#22232=CARTESIAN_POINT('Ctrl Pts',(-1.10056197765173,-2.26419292096484,
0.56536181660721));
#22233=CARTESIAN_POINT('Ctrl Pts',(-1.0246677492648,-2.30108302044024,0.570682223309577));
#22234=CARTESIAN_POINT('Ctrl Pts',(-0.946944012562917,-2.33413982481418,
0.576002630011945));
#22235=CARTESIAN_POINT('Ctrl Pts',(-0.867816815767798,-2.36319703458485,
0.581323036714313));
#22236=CARTESIAN_POINT('Ctrl Pts',(-0.789801797256569,-2.39184582855153,
0.586568662038905));
#22237=CARTESIAN_POINT('Ctrl Pts',(-0.710422986118061,-2.41660666787764,
0.591814287363496));
#22238=CARTESIAN_POINT('Ctrl Pts',(-0.630103544308487,-2.43737066804577,
0.597059912688088));
#22239=CARTESIAN_POINT('Ctrl Pts',(-0.548066557454519,-2.45857868406843,
0.602417710079344));
#22240=CARTESIAN_POINT('Ctrl Pts',(-0.465048744752886,-2.47561684540565,
0.607775507470597));
#22241=CARTESIAN_POINT('Ctrl Pts',(-0.381509456210711,-2.48842455879655,
0.613133304861853));
#22242=CARTESIAN_POINT('Ctrl Pts',(-0.297970167668535,-2.50123227218746,
0.618491102253108));
#22243=CARTESIAN_POINT('Ctrl Pts',(-0.213909912770551,-2.50980955209961,
0.623848899644367));
#22244=CARTESIAN_POINT('Ctrl Pts',(-0.129788985686316,-2.51415215712862,
0.629206697035622));
#22245=CARTESIAN_POINT('Ctrl Pts',(-0.047261723163428,-2.51841249183587,
0.634462991363071));
#22246=CARTESIAN_POINT('Ctrl Pts',(0.0356272034635327,-2.51861290613602,
0.639719285690518));
#22247=CARTESIAN_POINT('Ctrl Pts',(0.118445090380389,-2.51471211286,0.644975580017967));
#22248=CARTESIAN_POINT('Ctrl Pts',(0.20114594817007,-2.51081683175591,0.650224446728505));
#22249=CARTESIAN_POINT('Ctrl Pts',(0.28377550876694,-2.50283187606817,0.655473313439045));
#22250=CARTESIAN_POINT('Ctrl Pts',(0.365898280032954,-2.49076789337524,
0.660722180149584));
#22251=CARTESIAN_POINT('Ctrl Pts',(0.448595137540521,-2.47861957638166,
0.666007739510843));
#22252=CARTESIAN_POINT('Ctrl Pts',(0.530777618532214,-2.46233494642037,
0.6712932988721));
#22253=CARTESIAN_POINT('Ctrl Pts',(0.61200339223134,-2.44197831642653,0.676578858233359));
#22254=CARTESIAN_POINT('Ctrl Pts',(0.69252200492473,-2.42179891361421,0.681818400901843));
#22255=CARTESIAN_POINT('Ctrl Pts',(0.772100048659439,-2.39761825181994,
0.687057943570328));
#22256=CARTESIAN_POINT('Ctrl Pts',(0.850315861233121,-2.36955041856791,
0.692297486238811));
#22257=CARTESIAN_POINT('Ctrl Pts',(0.928506192134854,-2.34149172944283,
0.697535321933946));
#22258=CARTESIAN_POINT('Ctrl Pts',(1.00533473952937,-2.30954853967114,0.70277315762908));
#22259=CARTESIAN_POINT('Ctrl Pts',(1.08039615906332,-2.27388442746794,0.708010993324216));
#22260=CARTESIAN_POINT('Ctrl Pts',(1.15545574030167,-2.23822118869854,0.713248700741863));
#22261=CARTESIAN_POINT('Ctrl Pts',(1.22874786360369,-2.19883740756184,0.71848640815951));
#22262=CARTESIAN_POINT('Ctrl Pts',(1.29988955463394,-2.15594373668553,0.723724115577157));
#22263=CARTESIAN_POINT('Ctrl Pts',(1.37216199747502,-2.11236829826457,0.729045073014044));
#22264=CARTESIAN_POINT('Ctrl Pts',(1.44221462172498,-2.06517065811216,0.734366030450932));
#22265=CARTESIAN_POINT('Ctrl Pts',(1.50967588999156,-2.01461781913548,0.739686987887819));
#22266=CARTESIAN_POINT('Ctrl Pts',(1.5761773301844,-1.96478423782033,0.74493223959817));
#22267=CARTESIAN_POINT('Ctrl Pts',(1.64016035927463,-1.91169066531786,0.750177491308521));
#22268=CARTESIAN_POINT('Ctrl Pts',(1.70130337941679,-1.85563279265727,0.755422743018872));
#22269=CARTESIAN_POINT('Ctrl Pts',(1.76377013300914,-1.79836127891361,0.760781553319027));
#22270=CARTESIAN_POINT('Ctrl Pts',(1.82327210965394,-1.73799597357039,0.766140363619182));
#22271=CARTESIAN_POINT('Ctrl Pts',(1.87950830977704,-1.67488947798924,0.771499173919336));
#22272=CARTESIAN_POINT('Ctrl Pts',(1.93574450990013,-1.61178298240809,0.776857984219491));
#22273=CARTESIAN_POINT('Ctrl Pts',(1.98871466811899,-1.54593573263283,0.782216794519645));
#22274=CARTESIAN_POINT('Ctrl Pts',(2.03816460106524,-1.47773181225977,0.7875756048198));
#22275=CARTESIAN_POINT('Ctrl Pts',(2.08698103976692,-1.4104016401092,0.79286576435987));
#22276=CARTESIAN_POINT('Ctrl Pts',(2.13254746814638,-1.34052609907627,0.79815592389994));
#22277=CARTESIAN_POINT('Ctrl Pts',(2.17459027483789,-1.26844920536081,0.80344608344001));
#22278=CARTESIAN_POINT('Ctrl Pts',(2.21657188440823,-1.19647722610625,0.808728542672704));
#22279=CARTESIAN_POINT('Ctrl Pts',(2.25503983332636,-1.12231064633767,0.814011001905399));
#22280=CARTESIAN_POINT('Ctrl Pts',(2.28976238804666,-1.04632425962838,0.819293461138093));
#22281=CARTESIAN_POINT('Ctrl Pts',(2.32444439986729,-0.970426596472905,
0.824569752442869));
#22282=CARTESIAN_POINT('Ctrl Pts',(2.35538951924606,-0.892713757994868,
0.829846043747642));
#22283=CARTESIAN_POINT('Ctrl Pts',(2.38241141190576,-0.813585960068888,
0.835122335052418));
#22284=CARTESIAN_POINT('Ctrl Pts',(2.4094079578325,-0.734532384596086,0.84039367715736));
#22285=CARTESIAN_POINT('Ctrl Pts',(2.43248844884065,-0.654066916378462,
0.845665019262304));
#22286=CARTESIAN_POINT('Ctrl Pts',(2.45151479060097,-0.57260936201279,0.850936361367246));
#22287=CARTESIAN_POINT('Ctrl Pts',(2.47053084747212,-0.491195840384925,
0.856204853992769));
#22288=CARTESIAN_POINT('Ctrl Pts',(2.4854970089497,-0.408791739321907,0.861473346618289));
#22289=CARTESIAN_POINT('Ctrl Pts',(2.49632544298429,-0.325830527589564,
0.866741839243812));
#22290=CARTESIAN_POINT('Ctrl Pts',(2.50715226328724,-0.242881679337623,
0.872009546720419));
#22291=CARTESIAN_POINT('Ctrl Pts',(2.51384252043204,-0.159376334278797,
0.877277254197028));
#22292=CARTESIAN_POINT('Ctrl Pts',(2.51635994169055,-0.0757554872939529,
0.882544961673636));
#22293=CARTESIAN_POINT('Ctrl Pts',(2.51713600423197,-0.0499771211156531,
0.884168873618426));
#22294=CARTESIAN_POINT('Ctrl Pts',(2.51751587579956,-0.0241878072630997,
0.885792785563215));
#22295=CARTESIAN_POINT('Ctrl Pts',(2.51749949188368,0.0015994891165021,
0.887416697508005));
#22296=CARTESIAN_POINT('Ctrl Pts',(2.51749949188307,0.00159949006993176,
0.88741669756805));
#22297=CARTESIAN_POINT('Ctrl Pts',(2.51743985264828,0.0954679961080183,
0.893327910048533));
#22298=CARTESIAN_POINT('Ctrl Pts',(2.51212612121857,0.18913758394578,0.899239122529015));
#22299=CARTESIAN_POINT('Ctrl Pts',(2.50164908824153,0.282060435545834,0.905150335009498));
#22300=CARTESIAN_POINT('Ctrl Pts',(2.49112317160026,0.375416845910796,0.911089127982165));
#22301=CARTESIAN_POINT('Ctrl Pts',(2.47538578820664,0.468019323633379,0.917027920954832));
#22302=CARTESIAN_POINT('Ctrl Pts',(2.45457854884019,0.559330311688543,0.922966713927499));
#22303=CARTESIAN_POINT('Ctrl Pts',(2.43365820860934,0.651137634288419,0.928937788098399));
#22304=CARTESIAN_POINT('Ctrl Pts',(2.407612866569,0.741639183707493,0.934908862269296));
#22305=CARTESIAN_POINT('Ctrl Pts',(2.37663455189708,0.83030985585442,0.940879936440195));
#22306=CARTESIAN_POINT('Ctrl Pts',(2.37168903348617,0.844465643419186,0.941833185755331));
#22307=CARTESIAN_POINT('Ctrl Pts',(2.36661788834054,0.858574816053316,0.942786435070469));
#22308=CARTESIAN_POINT('Ctrl Pts',(2.36142200728636,0.872635292378022,0.943739684385605));
#22309=CARTESIAN_POINT('Origin',(0.,0.,116.208423447177));
#22310=CARTESIAN_POINT('',(1.87238193903529,2.43733217358128,95.4372285454945));
#22311=CARTESIAN_POINT('',(1.87274665176455,2.43781213467006,95.3543119584347));
#22312=CARTESIAN_POINT('',(1.8723819390353,2.43733217358128,116.208423447177));
#22313=CARTESIAN_POINT('',(0.793799282532884,-2.96922295374569,95.));
#22314=CARTESIAN_POINT('Ctrl Pts',(1.87274665176427,2.43781213467027,95.3543119584347));
#22315=CARTESIAN_POINT('Ctrl Pts',(2.06600193866627,2.29241896294923,95.341787244146));
#22316=CARTESIAN_POINT('Ctrl Pts',(2.9817068419035,1.41812695324678,95.2764728939291));
#22317=CARTESIAN_POINT('Ctrl Pts',(3.44893401864242,-1.12662596907763,95.1583689077841));
#22318=CARTESIAN_POINT('Ctrl Pts',(1.77865212890006,-2.70592999965464,95.0527896359281));
#22319=CARTESIAN_POINT('Ctrl Pts',(0.7937992825328,-2.96922295374571,95.));
#22320=CARTESIAN_POINT('',(-0.793800297434324,-2.96922268241929,95.0000201645727));
#22321=CARTESIAN_POINT('Origin',(0.,0.,95.));
#22322=CARTESIAN_POINT('Ctrl Pts',(1.87238193903529,2.43733217358128,95.4372285454945));
#22323=CARTESIAN_POINT('Ctrl Pts',(1.95199907732151,2.3761695247718,95.43203022616));
#22324=CARTESIAN_POINT('Ctrl Pts',(2.02870034980563,2.31103702475557,95.4268319068256));
#22325=CARTESIAN_POINT('Ctrl Pts',(2.1020729328552,2.2422514655938,95.4216335874911));
#22326=CARTESIAN_POINT('Ctrl Pts',(2.17232729272017,2.17638918807797,95.416656188822));
#22327=CARTESIAN_POINT('Ctrl Pts',(2.2395297596846,2.10717834640106,95.411678790153));
#22328=CARTESIAN_POINT('Ctrl Pts',(2.30335166303348,2.03493817262366,95.4067013914839));
#22329=CARTESIAN_POINT('Ctrl Pts',(2.36715550913664,1.96271843788834,95.4017254010792));
#22330=CARTESIAN_POINT('Ctrl Pts',(2.42758040087319,1.88747140367397,95.3967494106744));
#22331=CARTESIAN_POINT('Ctrl Pts',(2.48433585976231,1.80955176380757,95.3917734202697));
#22332=CARTESIAN_POINT('Ctrl Pts',(2.5410908516842,1.73163276504104,95.386797470806));
#22333=CARTESIAN_POINT('Ctrl Pts',(2.59417621222107,1.65104156053901,95.3818215213422));
#22334=CARTESIAN_POINT('Ctrl Pts',(2.64334361325069,1.5681635094233,95.3768455718785));
#22335=CARTESIAN_POINT('Ctrl Pts',(2.69252411613971,1.48526337341901,95.371868296451));
#22336=CARTESIAN_POINT('Ctrl Pts',(2.7377843613136,1.400075558836,95.3668910210236));
#22337=CARTESIAN_POINT('Ctrl Pts',(2.77892151202516,1.31301084534888,95.3619137455961));
#22338=CARTESIAN_POINT('Ctrl Pts',(2.82010539412938,1.22584722721616,95.3569308160334));
#22339=CARTESIAN_POINT('Ctrl Pts',(2.85715664663417,1.13680285365857,95.3519478864708));
#22340=CARTESIAN_POINT('Ctrl Pts',(2.88992033600746,1.04630908508459,95.3469649569081));
#22341=CARTESIAN_POINT('Ctrl Pts',(2.92270594910692,0.955754762872091,95.3419786930328));
#22342=CARTESIAN_POINT('Ctrl Pts',(2.95119815856141,0.863749534894087,95.3369924291575));
#22343=CARTESIAN_POINT('Ctrl Pts',(2.9752923225259,0.770738506575633,95.3320061652822));
#22344=CARTESIAN_POINT('Ctrl Pts',(2.99942397267683,0.677582769822665,95.3270121436769));
#22345=CARTESIAN_POINT('Ctrl Pts',(3.01914383312545,0.58341853954865,95.3220181220717));
#22346=CARTESIAN_POINT('Ctrl Pts',(3.03439864879444,0.488699386325051,95.3170241004664));
#22347=CARTESIAN_POINT('Ctrl Pts',(3.03903679627405,0.45990051970302,95.3155056941333));
#22348=CARTESIAN_POINT('Ctrl Pts',(3.0432625449371,0.431050373549066,95.3139872878003));
#22349=CARTESIAN_POINT('Ctrl Pts',(3.04707535237419,0.40216171741438,95.3124688814672));
#22350=CARTESIAN_POINT('Ctrl Pts',(3.05965199261959,0.306871766014207,95.3074603803792));
#22351=CARTESIAN_POINT('Ctrl Pts',(3.06777615614939,0.21082657494261,95.3024518792911));
#22352=CARTESIAN_POINT('Ctrl Pts',(3.07136732883625,0.114476990514523,95.297443378203));
#22353=CARTESIAN_POINT('Ctrl Pts',(3.07495362336384,0.0182582849553239,
95.2924416805377));
#22354=CARTESIAN_POINT('Ctrl Pts',(3.0740191495951,-0.0782635588336074,
95.2874399828725));
#22355=CARTESIAN_POINT('Ctrl Pts',(3.06853490026756,-0.17463051233945,95.2824382852072));
#22356=CARTESIAN_POINT('Ctrl Pts',(3.06305646302346,-0.270895338326955,
95.277441888228));
#22357=CARTESIAN_POINT('Ctrl Pts',(3.05303786108569,-0.367005166113458,
95.2724454912488));
#22358=CARTESIAN_POINT('Ctrl Pts',(3.03850212533996,-0.46250090195001,95.2674490942696));
#22359=CARTESIAN_POINT('Ctrl Pts',(3.02397702351035,-0.557926775919026,
95.2624563525072));
#22360=CARTESIAN_POINT('Ctrl Pts',(3.00494142390259,-0.65273902012935,95.2574636107449));
#22361=CARTESIAN_POINT('Ctrl Pts',(2.9814701956168,-0.746483571586628,95.2524708689826));
#22362=CARTESIAN_POINT('Ctrl Pts',(2.95800776792021,-0.840192973316017,
95.2474799992599));
#22363=CARTESIAN_POINT('Ctrl Pts',(2.93011312251414,-0.932835054094185,
95.2424891295371));
#22364=CARTESIAN_POINT('Ctrl Pts',(2.89791205806607,-1.02396677373598,95.2374982598144));
#22365=CARTESIAN_POINT('Ctrl Pts',(2.86571436112259,-1.11508896305668,95.232507912024));
#22366=CARTESIAN_POINT('Ctrl Pts',(2.82921128645578,-1.20470069310555,95.2275175642337));
#22367=CARTESIAN_POINT('Ctrl Pts',(2.78857791297204,-1.29237590246975,95.2225272164433));
#22368=CARTESIAN_POINT('Ctrl Pts',(2.74793780284242,-1.38006564759083,95.2175360412984));
#22369=CARTESIAN_POINT('Ctrl Pts',(2.70316621786208,-1.46581783771117,95.2125448661535));
#22370=CARTESIAN_POINT('Ctrl Pts',(2.65448515558461,-1.54922910145044,95.2075536910085));
#22371=CARTESIAN_POINT('Ctrl Pts',(2.60575338765648,-1.63272724543024,95.2025573171113));
#22372=CARTESIAN_POINT('Ctrl Pts',(2.55310423340784,-1.71387921678865,95.1975609432141));
#22373=CARTESIAN_POINT('Ctrl Pts',(2.49680406636686,-1.79230904259671,95.1925645693169));
#22374=CARTESIAN_POINT('Ctrl Pts',(2.44047165355774,-1.87078378887499,95.1875653337601));
#22375=CARTESIAN_POINT('Ctrl Pts',(2.38048433483173,-1.94653294191964,95.1825660982033));
#22376=CARTESIAN_POINT('Ctrl Pts',(2.31714866444604,-2.01921378681306,95.1775668626465));
#22377=CARTESIAN_POINT('Ctrl Pts',(2.25371354258339,-2.09200875724311,95.1725597771474));
#22378=CARTESIAN_POINT('Ctrl Pts',(2.18691987252752,-2.16172548314829,95.1675526916483));
#22379=CARTESIAN_POINT('Ctrl Pts',(2.11711085813903,-2.22805831708908,95.1625456061491));
#22380=CARTESIAN_POINT('Ctrl Pts',(2.07786106046433,-2.26535364827477,95.1597303953271));
#22381=CARTESIAN_POINT('Ctrl Pts',(2.037658659917,-2.30157998686302,95.1569151845051));
#22382=CARTESIAN_POINT('Ctrl Pts',(1.99656891278477,-2.33668885958345,95.1540999736831));
#22383=CARTESIAN_POINT('Ctrl Pts',(1.92387856350215,-2.39879866553469,95.149119688521));
#22384=CARTESIAN_POINT('Ctrl Pts',(1.84815642390381,-2.45762505194757,95.1441394033589));
#22385=CARTESIAN_POINT('Ctrl Pts',(1.76973267449693,-2.51285664350714,95.1391591181968));
#22386=CARTESIAN_POINT('Ctrl Pts',(1.69141397285223,-2.56801425294854,95.1341855040727));
#22387=CARTESIAN_POINT('Ctrl Pts',(1.61040121108685,-2.61958638311514,95.1292118899486));
#22388=CARTESIAN_POINT('Ctrl Pts',(1.5270587811377,-2.66730083210542,95.1242382758245));
#22389=CARTESIAN_POINT('Ctrl Pts',(1.44032909978763,-2.71695451941985,95.119062521189));
#22390=CARTESIAN_POINT('Ctrl Pts',(1.35107671067972,-2.76242995177963,95.1138867665535));
#22391=CARTESIAN_POINT('Ctrl Pts',(1.25974732844742,-2.80346908641233,95.108711011918));
#22392=CARTESIAN_POINT('Ctrl Pts',(1.17213645803605,-2.84283729649127,95.103745990174));
#22393=CARTESIAN_POINT('Ctrl Pts',(1.08261487000877,-2.87812320383586,95.09878096843));
#22394=CARTESIAN_POINT('Ctrl Pts',(0.991601232680961,-2.9091457930715,95.093815946686));
#22395=CARTESIAN_POINT('Ctrl Pts',(0.900616750682097,-2.94015844452396,
95.0888525154381));
#22396=CARTESIAN_POINT('Ctrl Pts',(0.808141587604577,-2.9669103483976,95.0838890841903));
#22397=CARTESIAN_POINT('Ctrl Pts',(0.714612621221596,-2.98926931734008,
95.0789256529424));
#22398=CARTESIAN_POINT('Ctrl Pts',(0.621087571927549,-3.01162734986602,
95.0739624295682));
#22399=CARTESIAN_POINT('Ctrl Pts',(0.526509237787314,-3.02959271093489,
95.0689992061939));
#22400=CARTESIAN_POINT('Ctrl Pts',(0.431326729031135,-3.04308388034627,
95.0640359828197));
#22401=CARTESIAN_POINT('Ctrl Pts',(0.336121702034778,-3.05657824149315,
95.059071585248));
#22402=CARTESIAN_POINT('Ctrl Pts',(0.24031265481731,-3.06559624710674,95.0541071876763));
#22403=CARTESIAN_POINT('Ctrl Pts',(0.144354772265256,-3.07010813322988,
95.0491427901047));
#22404=CARTESIAN_POINT('Ctrl Pts',(0.048291499036758,-3.07462497476385,
95.0441729401282));
#22405=CARTESIAN_POINT('Ctrl Pts',(-0.0479204930664325,-3.07462580026007,
95.0392030901517));
#22406=CARTESIAN_POINT('Ctrl Pts',(-0.143825393015308,-3.07013297860597,
95.0342332401753));
#22407=CARTESIAN_POINT('Ctrl Pts',(-0.239792625173286,-3.06563723689775,
95.029260160106));
#22408=CARTESIAN_POINT('Ctrl Pts',(-0.335451927996392,-3.05664207694859,
95.0242870800367));
#22409=CARTESIAN_POINT('Ctrl Pts',(-0.430354103305085,-3.04322158177292,
95.0193139999675));
#22410=CARTESIAN_POINT('Ctrl Pts',(-0.525401275530676,-3.02978058200484,
95.0143333217449));
#22411=CARTESIAN_POINT('Ctrl Pts',(-0.619688578614677,-3.01190083860415,
95.0093526435223));
#22412=CARTESIAN_POINT('Ctrl Pts',(-0.712778776397496,-2.98970712042456,
95.0043719652997));
#22413=CARTESIAN_POINT('Ctrl Pts',(-0.739890879895944,-2.98324329932811,
95.0029213650574));
#22414=CARTESIAN_POINT('Ctrl Pts',(-0.766901553461834,-2.97641386787412,
95.001470764815));
#22415=CARTESIAN_POINT('Ctrl Pts',(-0.793800297434324,-2.96922268241929,
95.0000201645727));
#22416=CARTESIAN_POINT('Origin',(0.,0.,116.208423447177));
#22417=CARTESIAN_POINT('',(1.87462644597698,2.44029756596839,96.4374142054168));
#22418=CARTESIAN_POINT('',(1.87238193903531,2.43733217358126,96.3541439943328));
#22419=CARTESIAN_POINT('',(1.8723819390353,2.43733217358128,116.208423447177));
#22420=CARTESIAN_POINT('',(-3.073000247725,0.000543316047154233,95.7084234157772));
#22421=CARTESIAN_POINT('Ctrl Pts',(1.87238193903531,2.43733217358126,96.3541439943328));
#22422=CARTESIAN_POINT('Ctrl Pts',(1.94890039524938,2.37854996204234,96.3491622040271));
#22423=CARTESIAN_POINT('Ctrl Pts',(2.02266131396365,2.3161507538951,96.3441804137215));
#22424=CARTESIAN_POINT('Ctrl Pts',(2.09331377339724,2.25043100229831,96.3391986234159));
#22425=CARTESIAN_POINT('Ctrl Pts',(2.16397435585413,2.18470369479934,96.334216260346));
#22426=CARTESIAN_POINT('Ctrl Pts',(2.23152544809283,2.1156553848872,96.3292338972762));
#22427=CARTESIAN_POINT('Ctrl Pts',(2.29565207766036,2.04362026519941,96.3242515342064));
#22428=CARTESIAN_POINT('Ctrl Pts',(2.3598454088084,1.97151021788219,96.3192639887109));
#22429=CARTESIAN_POINT('Ctrl Pts',(2.42060687118491,1.89640748479273,96.3142764432154));
#22430=CARTESIAN_POINT('Ctrl Pts',(2.47766112968026,1.8186801743219,96.3092888977199));
#22431=CARTESIAN_POINT('Ctrl Pts',(2.53474566539261,1.74091161598093,96.3042987054632));
#22432=CARTESIAN_POINT('Ctrl Pts',(2.58811883594471,1.6605160719845,96.2993085132065));
#22433=CARTESIAN_POINT('Ctrl Pts',(2.63754929462482,1.57788971998175,96.2943183209498));
#22434=CARTESIAN_POINT('Ctrl Pts',(2.68706324692705,1.49512380274748,96.2893196996953));
#22435=CARTESIAN_POINT('Ctrl Pts',(2.73262097536261,1.41011993708907,96.2843210784408));
#22436=CARTESIAN_POINT('Ctrl Pts',(2.77403759886778,1.32329802012542,96.2793224571864));
#22437=CARTESIAN_POINT('Ctrl Pts',(2.80820522869565,1.25167221220823,96.2751987255487));
#22438=CARTESIAN_POINT('Ctrl Pts',(2.83955533933329,1.17880957773639,96.2710749939111));
#22439=CARTESIAN_POINT('Ctrl Pts',(2.86800958600607,1.10495396491316,96.2669512622734));
#22440=CARTESIAN_POINT('Ctrl Pts',(2.90250143644083,1.01542719653439,96.2619525309236));
#22441=CARTESIAN_POINT('Ctrl Pts',(2.93285800694782,0.924126318119108,96.2569537995738));
#22442=CARTESIAN_POINT('Ctrl Pts',(2.95889528436648,0.831469149249558,96.251955068224));
#22443=CARTESIAN_POINT('Ctrl Pts',(2.98489722985203,0.738937713836757,96.2469631200274));
#22444=CARTESIAN_POINT('Ctrl Pts',(3.00659141307212,0.645054064831401,96.2419711718308));
#22445=CARTESIAN_POINT('Ctrl Pts',(3.02384217706374,0.550255157368292,96.2369792236341));
#22446=CARTESIAN_POINT('Ctrl Pts',(3.04107473805111,0.455556281701891,96.2319925429407));
#22447=CARTESIAN_POINT('Ctrl Pts',(3.05387312238288,0.359944497192783,96.2270058622473));
#22448=CARTESIAN_POINT('Ctrl Pts',(3.06215199580362,0.263870052480181,96.2220191815539));
#22449=CARTESIAN_POINT('Ctrl Pts',(3.07042494913393,0.167864309071667,96.2170360667563));
#22450=CARTESIAN_POINT('Ctrl Pts',(3.07418477861356,0.0713969993844289,
96.2120529519588));
#22451=CARTESIAN_POINT('Ctrl Pts',(3.07339771727761,-0.0250743181916119,
96.2070698371612));
#22452=CARTESIAN_POINT('Ctrl Pts',(3.07261094230205,-0.121510536134186,
96.2020885353948));
#22453=CARTESIAN_POINT('Ctrl Pts',(3.06728056700538,-0.217950320417463,
96.1971072336284));
#22454=CARTESIAN_POINT('Ctrl Pts',(3.05742492024352,-0.31393487712244,96.192125931862));
#22455=CARTESIAN_POINT('Ctrl Pts',(3.04757016647388,-0.40991073693885,96.1871450814372));
#22456=CARTESIAN_POINT('Ctrl Pts',(3.03319100146494,-0.505431014383348,
96.1821642310125));
#22457=CARTESIAN_POINT('Ctrl Pts',(3.01435764138757,-0.600041881711913,
96.1771833805877));
#22458=CARTESIAN_POINT('Ctrl Pts',(2.99552084201603,-0.694670026605536,
96.1722016205743));
#22459=CARTESIAN_POINT('Ctrl Pts',(2.97222831790626,-0.788388000908782,
96.1672198605609));
#22460=CARTESIAN_POINT('Ctrl Pts',(2.94460120804333,-0.88075307299479,96.1622381005475));
#22461=CARTESIAN_POINT('Ctrl Pts',(2.91694425733271,-0.973217911290937,
96.1572509595897));
#22462=CARTESIAN_POINT('Ctrl Pts',(2.88494349992794,-1.0643265086119,96.152263818632));
#22463=CARTESIAN_POINT('Ctrl Pts',(2.84876962586883,-1.15365240377123,96.1472766776742));
#22464=CARTESIAN_POINT('Ctrl Pts',(2.81257434529212,-1.24303115907887,96.1422865854892));
#22465=CARTESIAN_POINT('Ctrl Pts',(2.77220121464559,-1.33062471308574,96.1372964933043));
#22466=CARTESIAN_POINT('Ctrl Pts',(2.7278677424662,-1.41602960054243,96.1323064011193));
#22467=CARTESIAN_POINT('Ctrl Pts',(2.68346248210394,-1.50157278219034,96.1273082285916));
#22468=CARTESIAN_POINT('Ctrl Pts',(2.63508429541024,-1.58491984109699,96.1223100560639));
#22469=CARTESIAN_POINT('Ctrl Pts',(2.58299496575557,-1.66569482705608,96.1173118835362));
#22470=CARTESIAN_POINT('Ctrl Pts',(2.55266952755875,-1.71272052043303,96.1144020405205));
#22471=CARTESIAN_POINT('Ctrl Pts',(2.52108704166495,-1.75887502791644,96.1114921975049));
#22472=CARTESIAN_POINT('Ctrl Pts',(2.4883053372942,-1.80408946518548,96.1085823544892));
#22473=CARTESIAN_POINT('Ctrl Pts',(2.43197076052523,-1.88178939678727,96.1035818586975));
#22474=CARTESIAN_POINT('Ctrl Pts',(2.3718945114762,-1.95698440230462,96.0985813629058));
#22475=CARTESIAN_POINT('Ctrl Pts',(2.30832713238641,-2.0292925121551,96.093580867114));
#22476=CARTESIAN_POINT('Ctrl Pts',(2.24484601165398,-2.10150250283078,96.0885871567925));
#22477=CARTESIAN_POINT('Ctrl Pts',(2.17788346331487,-2.17083305675957,96.0835934464709));
#22478=CARTESIAN_POINT('Ctrl Pts',(2.10773239764918,-2.2369323614942,96.0785997361493));
#22479=CARTESIAN_POINT('Ctrl Pts',(2.03765539409394,-2.3029618817721,96.0736112979462));
#22480=CARTESIAN_POINT('Ctrl Pts',(1.96439688289154,-2.36576663526249,96.068622859743));
#22481=CARTESIAN_POINT('Ctrl Pts',(1.88828831398959,-2.42502979223975,96.0636344215399));
#22482=CARTESIAN_POINT('Ctrl Pts',(1.81223436368252,-2.48425041957272,96.0586495632422));
#22483=CARTESIAN_POINT('Ctrl Pts',(1.73333476695209,-2.53993423425027,96.0536647049446));
#22484=CARTESIAN_POINT('Ctrl Pts',(1.65195517251102,-2.59180368817048,96.0486798466469));
#22485=CARTESIAN_POINT('Ctrl Pts',(1.57060532800669,-2.64365418017543,96.0436968106638));
#22486=CARTESIAN_POINT('Ctrl Pts',(1.48677765678592,-2.69169284641807,96.0387137746808));
#22487=CARTESIAN_POINT('Ctrl Pts',(1.4008672035044,-2.73568516612306,96.0337307386977));
#22488=CARTESIAN_POINT('Ctrl Pts',(1.31496472709016,-2.77967340109933,96.0287481653942));
#22489=CARTESIAN_POINT('Ctrl Pts',(1.22698024374369,-2.81961583669491,96.0237655920907));
#22490=CARTESIAN_POINT('Ctrl Pts',(1.13733288238007,-2.85532417855785,96.0187830187873));
#22491=CARTESIAN_POINT('Ctrl Pts',(1.04766939667527,-2.89103894306924,96.0137995492978));
#22492=CARTESIAN_POINT('Ctrl Pts',(0.956342846597565,-2.92251793905592,
96.0088160798083));
#22493=CARTESIAN_POINT('Ctrl Pts',(0.86379078274741,-2.94962162550396,96.0038326103188));
#22494=CARTESIAN_POINT('Ctrl Pts',(0.77113935568867,-2.97675441026853,95.9988437906135));
#22495=CARTESIAN_POINT('Ctrl Pts',(0.677260209959345,-2.99950238421146,
95.9938549709082));
#22496=CARTESIAN_POINT('Ctrl Pts',(0.582604231448032,-3.01777642636078,
95.9888661512028));
#22497=CARTESIAN_POINT('Ctrl Pts',(0.487892539284682,-3.03606122444588,
95.9838743951234));
#22498=CARTESIAN_POINT('Ctrl Pts',(0.392403537956677,-3.04986678451124,
95.978882639044));
#22499=CARTESIAN_POINT('Ctrl Pts',(0.296594328969761,-3.05915577472331,
95.9738908829645));
#22500=CARTESIAN_POINT('Ctrl Pts',(0.200630793355014,-3.06845972736488,
95.9688910863127));
#22501=CARTESIAN_POINT('Ctrl Pts',(0.104346458129836,-3.07323256149298,
95.9638912896608));
#22502=CARTESIAN_POINT('Ctrl Pts',(0.00819946362641492,-3.07348906274225,
95.9588914930089));
#22503=CARTESIAN_POINT('Ctrl Pts',(-0.0474273367138514,-3.07363746409223,
95.9559988109076));
#22504=CARTESIAN_POINT('Ctrl Pts',(-0.103008221685502,-3.07227507766361,
95.9531061288063));
#22505=CARTESIAN_POINT('Ctrl Pts',(-0.15845552235523,-3.06941266326884,
95.950213446705));
#22506=CARTESIAN_POINT('Ctrl Pts',(-0.254304418075243,-3.06446455478534,
95.9452130159946));
#22507=CARTESIAN_POINT('Ctrl Pts',(-0.350089038366274,-3.05501385990303,
95.9402125852842));
#22508=CARTESIAN_POINT('Ctrl Pts',(-0.445352560841227,-3.04106286461694,
95.9352121545737));
#22509=CARTESIAN_POINT('Ctrl Pts',(-0.540487134578819,-3.02713075340295,
95.930218492448));
#22510=CARTESIAN_POINT('Ctrl Pts',(-0.635101581926603,-3.00871051163352,
95.9252248303224));
#22511=CARTESIAN_POINT('Ctrl Pts',(-0.728741322152277,-2.98585638224409,
95.9202311681967));
#22512=CARTESIAN_POINT('Ctrl Pts',(-0.822282514218609,-2.96302630495454,
95.9152427614915));
#22513=CARTESIAN_POINT('Ctrl Pts',(-0.914850614413196,-2.93577171996645,
95.9102543547863));
#22514=CARTESIAN_POINT('Ctrl Pts',(-1.00599941533267,-2.90419824157207,
95.9052659480812));
#22515=CARTESIAN_POINT('Ctrl Pts',(-1.09708325569609,-2.87264726518203,
95.9002810965481));
#22516=CARTESIAN_POINT('Ctrl Pts',(-1.18674939422637,-2.83678365758152,
95.895296245015));
#22517=CARTESIAN_POINT('Ctrl Pts',(-1.27456596348003,-2.79676310307795,
95.8903113934819));
#22518=CARTESIAN_POINT('Ctrl Pts',(-1.3623506983059,-2.75675705644531,95.8853283490098));
#22519=CARTESIAN_POINT('Ctrl Pts',(-1.44828679720389,-2.71259723883619,
95.8803453045378));
#22520=CARTESIAN_POINT('Ctrl Pts',(-1.5319624912743,-2.66448741324268,95.8753622600657));
#22521=CARTESIAN_POINT('Ctrl Pts',(-1.61563067019821,-2.61638190852623,
95.8703796631346));
#22522=CARTESIAN_POINT('Ctrl Pts',(-1.69703846764458,-2.56432732002754,
95.8653970662036));
#22523=CARTESIAN_POINT('Ctrl Pts',(-1.77579978769978,-2.50857277430921,
95.8604144692726));
#22524=CARTESIAN_POINT('Ctrl Pts',(-1.85457551170371,-2.45280803214398,
95.8554309611193));
#22525=CARTESIAN_POINT('Ctrl Pts',(-1.93070343900024,-2.39334224243777,
95.8504474529659));
#22526=CARTESIAN_POINT('Ctrl Pts',(-2.00382834816003,-2.33046652005779,
95.8454639448126));
#22527=CARTESIAN_POINT('Ctrl Pts',(-2.07703209272744,-2.26752301184038,
95.8404750639771));
#22528=CARTESIAN_POINT('Ctrl Pts',(-2.14722602247896,-2.20116251823993,
95.8354861831416));
#22529=CARTESIAN_POINT('Ctrl Pts',(-2.2140899552858,-2.13171478390111,95.8304973023061));
#22530=CARTESIAN_POINT('Ctrl Pts',(-2.28099341415391,-2.06222599610808,
95.8255054723349));
#22531=CARTESIAN_POINT('Ctrl Pts',(-2.3445626674711,-1.98964666357807,95.8205136423637));
#22532=CARTESIAN_POINT('Ctrl Pts',(-2.40451759767676,-1.91433993127208,
95.8155218123926));
#22533=CARTESIAN_POINT('Ctrl Pts',(-2.46456933067151,-1.8389116092703,95.8105219226494));
#22534=CARTESIAN_POINT('Ctrl Pts',(-2.52099483136462,-1.76074744989398,
95.8055220329063));
#22535=CARTESIAN_POINT('Ctrl Pts',(-2.5735571384206,-1.68023983564382,95.8005221431632));
#22536=CARTESIAN_POINT('Ctrl Pts',(-2.60396546887915,-1.63366459426521,
95.7976296084158));
#22537=CARTESIAN_POINT('Ctrl Pts',(-2.63308169225606,-1.58630551453297,
95.7947370736683));
#22538=CARTESIAN_POINT('Ctrl Pts',(-2.66086712515347,-1.53824198105418,
95.7918445389209));
#22539=CARTESIAN_POINT('Ctrl Pts',(-2.71074598685348,-1.45196100252656,
95.7866520216345));
#22540=CARTESIAN_POINT('Ctrl Pts',(-2.75649795601848,-1.36312477777713,
95.7814595043481));
#22541=CARTESIAN_POINT('Ctrl Pts',(-2.79786374839681,-1.27214806347649,
95.7762669870617));
#22542=CARTESIAN_POINT('Ctrl Pts',(-2.83915701351187,-1.18133086001146,
95.7710835738936));
#22543=CARTESIAN_POINT('Ctrl Pts',(-2.87607924651253,-1.08838099000229,
95.7659001607256));
#22544=CARTESIAN_POINT('Ctrl Pts',(-2.9084162021105,-0.993739123362437,
95.7607167475575));
#22545=CARTESIAN_POINT('Ctrl Pts',(-2.94068575767816,-0.899294519098164,
95.7555441381957));
#22546=CARTESIAN_POINT('Ctrl Pts',(-2.96838895106745,-0.803165312865599,
95.7503715288339));
#22547=CARTESIAN_POINT('Ctrl Pts',(-2.99135941124075,-0.705812384973069,
95.7451989194722));
#22548=CARTESIAN_POINT('Ctrl Pts',(-3.01430118770704,-0.608581023772685,
95.7400327692588));
#22549=CARTESIAN_POINT('Ctrl Pts',(-3.03252190065904,-0.51012936038651,
95.7348666190454));
#22550=CARTESIAN_POINT('Ctrl Pts',(-3.04590469133192,-0.410934132583531,
95.7297004688321));
#22551=CARTESIAN_POINT('Ctrl Pts',(-3.05926884892359,-0.311877015939915,
95.7245415115353));
#22552=CARTESIAN_POINT('Ctrl Pts',(-3.06780845018851,-0.212078783790839,
95.7193825542385));
#22553=CARTESIAN_POINT('Ctrl Pts',(-3.07145769837096,-0.112026144795582,
95.7142235969417));
#22554=CARTESIAN_POINT('Ctrl Pts',(-3.07282529940395,-0.0745301769681272,
95.7122902136869));
#22555=CARTESIAN_POINT('Ctrl Pts',(-3.0735065820639,-0.0369985695992274,
95.7103568304322));
#22556=CARTESIAN_POINT('Ctrl Pts',(-3.07349995206979,0.000542795567035782,
95.7084234471775));
#22557=CARTESIAN_POINT('Ctrl Pts',(-3.06853913704955,0.000547962633554823,
95.7084231354506));
#22558=CARTESIAN_POINT('Ctrl Pts',(-3.06913019292027,0.484861479280904,
95.6834406340126));
#22559=CARTESIAN_POINT('Ctrl Pts',(-2.733190250717,1.9916708787895,95.6056684966466));
#22560=CARTESIAN_POINT('Ctrl Pts',(-0.606155923754067,3.45373062715694,
95.4876314376412));
#22561=CARTESIAN_POINT('Ctrl Pts',(1.25146230115526,2.90522756078225,95.394576880074));
#22562=CARTESIAN_POINT('Ctrl Pts',(1.87274665176427,2.43781213467027,95.3543119584347));
#22563=CARTESIAN_POINT('',(-3.07399806097456,0.000489289934194882,95.7915766089109));
#22564=CARTESIAN_POINT('Ctrl Pts',(-3.07349996089424,0.000490288814122033,
95.7915765528225));
#22565=CARTESIAN_POINT('Ctrl Pts',(-3.07349587727009,0.0260895240076914,
95.7902429034883));
#22566=CARTESIAN_POINT('Ctrl Pts',(-3.0731719752456,0.0516859350238667,
95.7889092541541));
#22567=CARTESIAN_POINT('Ctrl Pts',(-3.07252842825033,0.0772742362857353,
95.7875756048199));
#22568=CARTESIAN_POINT('Ctrl Pts',(-3.07011545939872,0.173217150113296,
95.7825751086228));
#22569=CARTESIAN_POINT('Ctrl Pts',(-3.06320007643443,0.269215187868969,
95.7775746124258));
#22570=CARTESIAN_POINT('Ctrl Pts',(-3.05177238829369,0.364811650099374,
95.7725741162287));
#22571=CARTESIAN_POINT('Ctrl Pts',(-3.04036020706927,0.46027839174918,95.7675804055052));
#22572=CARTESIAN_POINT('Ctrl Pts',(-3.02444794151189,0.555344208923741,
95.7625866947818));
#22573=CARTESIAN_POINT('Ctrl Pts',(-3.00407769839575,0.649553255708325,
95.7575929840583));
#22574=CARTESIAN_POINT('Ctrl Pts',(-2.98372896121357,0.743662841061493,
95.7526045454572));
#22575=CARTESIAN_POINT('Ctrl Pts',(-2.9589316950746,0.836917027616928,95.747616106856));
#22576=CARTESIAN_POINT('Ctrl Pts',(-2.92977958303345,0.92886696832234,95.7426276682549));
#22577=CARTESIAN_POINT('Ctrl Pts',(-2.90064839177123,1.02075092189175,95.7376428095666));
#22578=CARTESIAN_POINT('Ctrl Pts',(-2.8671686997368,1.11133207327179,95.7326579508783));
#22579=CARTESIAN_POINT('Ctrl Pts',(-2.82948462399554,1.20017457587338,95.72767309219));
#22580=CARTESIAN_POINT('Ctrl Pts',(-2.79181432445534,1.28898460024232,95.7226900558209));
#22581=CARTESIAN_POINT('Ctrl Pts',(-2.74994286626322,1.37605683518936,95.7177070194519));
#22582=CARTESIAN_POINT('Ctrl Pts',(-2.7040629642024,1.46097424194573,95.7127239830828));
#22583=CARTESIAN_POINT('Ctrl Pts',(-2.65818732218065,1.54588376395401,95.7077414093985));
#22584=CARTESIAN_POINT('Ctrl Pts',(-2.6083041850157,1.62863846962425,95.7027588357141));
#22585=CARTESIAN_POINT('Ctrl Pts',(-2.55465229994161,1.7088457731472,95.6977762620298));
#22586=CARTESIAN_POINT('Ctrl Pts',(-2.50099076488044,1.78906750299351,95.692792792165));
#22587=CARTESIAN_POINT('Ctrl Pts',(-2.4435593796705,1.86674055605838,95.6878093223002));
#22588=CARTESIAN_POINT('Ctrl Pts',(-2.38263968880861,1.94150208944364,95.6828258524354));
#22589=CARTESIAN_POINT('Ctrl Pts',(-2.32165459515316,2.01634388609131,95.6778370323653));
#22590=CARTESIAN_POINT('Ctrl Pts',(-2.25717399687822,2.0882675819913,95.6728482122952));
#22591=CARTESIAN_POINT('Ctrl Pts',(-2.18951898812381,2.15694433183736,95.6678593922252));
#22592=CARTESIAN_POINT('Ctrl Pts',(-2.12182415832039,2.22566150411882,95.6628676357864));
#22593=CARTESIAN_POINT('Ctrl Pts',(-2.05095151978951,2.29112762732478,95.6578758793477));
#22594=CARTESIAN_POINT('Ctrl Pts',(-1.97725662449484,2.35305301489177,95.6528841229089));
#22595=CARTESIAN_POINT('Ctrl Pts',(-1.90344302383817,2.41507814987707,95.6478843259098));
#22596=CARTESIAN_POINT('Ctrl Pts',(-1.82679843763728,2.4735508949663,95.6428845289107));
#22597=CARTESIAN_POINT('Ctrl Pts',(-1.74770879545561,2.52822392526594,95.6378847319115));
#22598=CARTESIAN_POINT('Ctrl Pts',(-1.70195075945917,2.55985550709481,95.6349920536195));
#22599=CARTESIAN_POINT('Ctrl Pts',(-1.65537479165772,2.59021604073263,95.6320993753275));
#22600=CARTESIAN_POINT('Ctrl Pts',(-1.60805923467315,2.6192647341921,95.6292066970355));
#22601=CARTESIAN_POINT('Ctrl Pts',(-1.52626713370109,2.66947979705859,95.6242062648306));
#22602=CARTESIAN_POINT('Ctrl Pts',(-1.44197754952503,2.71594785869701,95.6192058326257));
#22603=CARTESIAN_POINT('Ctrl Pts',(-1.35556824555185,2.75841203986125,95.6142054004208));
#22604=CARTESIAN_POINT('Ctrl Pts',(-1.26927590504828,2.80081874159058,95.6092117367914));
#22605=CARTESIAN_POINT('Ctrl Pts',(-1.18086993769247,2.8392321422873,95.604218073162));
#22606=CARTESIAN_POINT('Ctrl Pts',(-1.09075569008632,2.87343945030069,95.5992244095326));
#22607=CARTESIAN_POINT('Ctrl Pts',(-1.00073628019014,2.90761075798291,95.5942360013166));
#22608=CARTESIAN_POINT('Ctrl Pts',(-0.909012572083997,2.93758461792952,
95.5892475931007));
#22609=CARTESIAN_POINT('Ctrl Pts',(-0.816012110743412,2.96319531673497,
95.5842591848847));
#22610=CARTESIAN_POINT('Ctrl Pts',(-0.723077929512727,2.98878776315859,
95.5792743318364));
#22611=CARTESIAN_POINT('Ctrl Pts',(-0.62886922575727,3.01002311398092,95.5742894787882));
#22612=CARTESIAN_POINT('Ctrl Pts',(-0.533830088582683,3.0267850413473,95.56930462574));
#22613=CARTESIAN_POINT('Ctrl Pts',(-0.438825404042331,3.043540892348,95.5643215797507));
#22614=CARTESIAN_POINT('Ctrl Pts',(-0.342991315883686,3.05582646586484,
95.5593385337614));
#22615=CARTESIAN_POINT('Ctrl Pts',(-0.246782583713422,3.06357644043293,
95.5543554877721));
#22616=CARTESIAN_POINT('Ctrl Pts',(-0.150582492309382,3.07132571895487,
95.5493728893236));
#22617=CARTESIAN_POINT('Ctrl Pts',(-0.054008261156951,3.07454017339115,
95.5443902908752));
#22618=CARTESIAN_POINT('Ctrl Pts',(0.0424808114944798,3.07320640872929,
95.5394076924267));
#22619=CARTESIAN_POINT('Ctrl Pts',(0.138987530126228,3.07187240014773,95.5344241827576));
#22620=CARTESIAN_POINT('Ctrl Pts',(0.235408620609279,3.06598852661926,95.5294406730884));
#22621=CARTESIAN_POINT('Ctrl Pts',(0.331286444502977,3.05559348436414,95.5244571634193));
#22622=CARTESIAN_POINT('Ctrl Pts',(0.42726763329119,3.04518723532102,95.5194682810798));
#22623=CARTESIAN_POINT('Ctrl Pts',(0.522703949282092,3.03026015549755,95.5144793987402));
#22624=CARTESIAN_POINT('Ctrl Pts',(0.617144748484151,3.01090262370247,95.5094905164006));
#22625=CARTESIAN_POINT('Ctrl Pts',(0.711641375483698,2.99153364888305,95.5044986849298));
#22626=CARTESIAN_POINT('Ctrl Pts',(0.805140888896846,2.96772911533756,95.499506853459));
#22627=CARTESIAN_POINT('Ctrl Pts',(0.897206742691589,2.93962962137558,95.4945150219882));
#22628=CARTESIAN_POINT('Ctrl Pts',(0.989421244889705,2.91148475831376,95.4895151307672));
#22629=CARTESIAN_POINT('Ctrl Pts',(1.08019705249857,2.87903123556852,95.4845152395462));
#22630=CARTESIAN_POINT('Ctrl Pts',(1.16911662325572,2.84245819164102,95.4795153483253));
#22631=CARTESIAN_POINT('Ctrl Pts',(1.22055806427665,2.82130008138327,95.476622828634));
#22632=CARTESIAN_POINT('Ctrl Pts',(1.2713786822235,2.79876411974557,95.4737303089427));
#22633=CARTESIAN_POINT('Ctrl Pts',(1.32150163250936,2.77489381513511,95.4708377892515));
#22634=CARTESIAN_POINT('Ctrl Pts',(1.40804369735621,2.73367945249822,95.4658435775128));
#22635=CARTESIAN_POINT('Ctrl Pts',(1.49281002673697,2.68833922668901,95.4608493657742));
#22636=CARTESIAN_POINT('Ctrl Pts',(1.5753800256132,2.63904907587922,95.4558551540356));
#22637=CARTESIAN_POINT('Ctrl Pts',(1.65782752464194,2.58983205133852,95.4508683516488));
#22638=CARTESIAN_POINT('Ctrl Pts',(1.73808479715806,2.53667697695274,95.4458815492621));
#22639=CARTESIAN_POINT('Ctrl Pts',(1.81575327570771,2.47980690614344,95.4408947468753));
#22640=CARTESIAN_POINT('Ctrl Pts',(1.8347867338384,2.46587031137745,95.4396726797484));
#22641=CARTESIAN_POINT('Ctrl Pts',(1.85366483429822,2.45171083285497,95.4384506126214));
#22642=CARTESIAN_POINT('Ctrl Pts',(1.87238193903529,2.43733217358128,95.4372285454945));
#22643=CARTESIAN_POINT('Ctrl Pts',(1.87462644597698,2.44029756596839,96.4374142054168));
#22644=CARTESIAN_POINT('Ctrl Pts',(1.95834925157173,2.37696725901686,96.4319598822634));
#22645=CARTESIAN_POINT('Ctrl Pts',(2.81520938972617,1.65344307781877,96.3737159231819));
#22646=CARTESIAN_POINT('Ctrl Pts',(3.57003808721136,-0.655357920372746,
96.2626823281723));
#22647=CARTESIAN_POINT('Ctrl Pts',(1.39401266499885,-3.35130737712119,96.1043134203881));
#22648=CARTESIAN_POINT('Ctrl Pts',(-2.02307198855743,-2.99696810683408,
95.9472783470963));
#22649=CARTESIAN_POINT('Ctrl Pts',(-3.07630577576351,-0.988793015625566,
95.8430329097325));
#22650=CARTESIAN_POINT('Ctrl Pts',(-3.0784329222612,0.000480396352174041,
95.7915771082968));
#22651=CARTESIAN_POINT('Origin',(0.,0.,116.208423447177));
#22652=CARTESIAN_POINT('',(1.87238193903531,2.43733217358127,97.4373604997054));
#22653=CARTESIAN_POINT('',(1.87238193903531,2.43733217358127,97.3540855889292));
#22654=CARTESIAN_POINT('',(1.8723819390353,2.43733217358128,116.208423447177));
#22655=CARTESIAN_POINT('',(-3.07349878913888,-0.00272821586942156,96.7084234471429));
#22656=CARTESIAN_POINT('Ctrl Pts',(1.87238193903531,2.43733217358127,97.3540855889292));
#22657=CARTESIAN_POINT('Ctrl Pts',(1.94866488721299,2.37873088157338,97.3490953090774));
#22658=CARTESIAN_POINT('Ctrl Pts',(2.02229111276488,2.31647038074485,97.3441050292257));
#22659=CARTESIAN_POINT('Ctrl Pts',(2.09289233906605,2.25082293996632,97.339114749374));
#22660=CARTESIAN_POINT('Ctrl Pts',(2.16478061199566,2.18397875910626,97.3340334976909));
#22661=CARTESIAN_POINT('Ctrl Pts',(2.23353210894762,2.11362317016449,97.3289522460077));
#22662=CARTESIAN_POINT('Ctrl Pts',(2.29879203377926,2.04008760484274,97.3238709943246));
#22663=CARTESIAN_POINT('Ctrl Pts',(2.36278895497312,1.9679752052195,97.3188880823097));
#22664=CARTESIAN_POINT('Ctrl Pts',(2.42342794060438,1.89280516011432,97.3139051702948));
#22665=CARTESIAN_POINT('Ctrl Pts',(2.48041155381986,1.81492720891967,97.30892225828));
#22666=CARTESIAN_POINT('Ctrl Pts',(2.53738140951798,1.73706805974906,97.3039405492864));
#22667=CARTESIAN_POINT('Ctrl Pts',(2.5906973874908,1.65650265779948,97.2989588402928));
#22668=CARTESIAN_POINT('Ctrl Pts',(2.64010346854948,1.57361238090992,97.2939771312992));
#22669=CARTESIAN_POINT('Ctrl Pts',(2.68951110915327,1.49071948751804,97.2889952650537));
#22670=CARTESIAN_POINT('Ctrl Pts',(2.73500838355779,1.40550195090539,97.2840133988082));
#22671=CARTESIAN_POINT('Ctrl Pts',(2.77638415978595,1.31836764496465,97.2790315325627));
#22672=CARTESIAN_POINT('Ctrl Pts',(2.81920258234809,1.22819523319272,97.2738759639307));
#22673=CARTESIAN_POINT('Ctrl Pts',(2.85760659608389,1.13597038545078,97.2687203952986));
#22674=CARTESIAN_POINT('Ctrl Pts',(2.8914161828386,1.04216827221858,97.2635648266666));
#22675=CARTESIAN_POINT('Ctrl Pts',(2.92413458878274,0.951393556709182,97.2585756504132));
#22676=CARTESIAN_POINT('Ctrl Pts',(2.95255051386505,0.859142272147958,97.2535864741597));
#22677=CARTESIAN_POINT('Ctrl Pts',(2.97655192666899,0.765859567964746,97.2485972979063));
#22678=CARTESIAN_POINT('Ctrl Pts',(3.00175403432598,0.667910302537554,97.2433585330849));
#22679=CARTESIAN_POINT('Ctrl Pts',(3.0220883572468,0.56882428666938,97.2381197682636));
#22680=CARTESIAN_POINT('Ctrl Pts',(3.03748631368271,0.469125936386219,97.2328810034423));
#22681=CARTESIAN_POINT('Ctrl Pts',(3.05288427011861,0.369427586103058,97.227642238621));
#22682=CARTESIAN_POINT('Ctrl Pts',(3.06334587623904,0.269117458435972,97.2224034737997));
#22683=CARTESIAN_POINT('Ctrl Pts',(3.06886550244303,0.168721006146533,97.2171647089784));
#22684=CARTESIAN_POINT('Ctrl Pts',(3.07413303278099,0.0729099242519637,
97.212165212344));
#22685=CARTESIAN_POINT('Ctrl Pts',(3.07491863032797,-0.0233163652926922,
97.2071657157097));
#22686=CARTESIAN_POINT('Ctrl Pts',(3.07117585748342,-0.119503566520019,
97.2021662190754));
#22687=CARTESIAN_POINT('Ctrl Pts',(3.06743816170377,-0.215560289974863,
97.1971735042496));
#22688=CARTESIAN_POINT('Ctrl Pts',(3.05918432071533,-0.311577595611862,
97.1921807894238));
#22689=CARTESIAN_POINT('Ctrl Pts',(3.04641979592841,-0.407097871494691,
97.187188074598));
#22690=CARTESIAN_POINT('Ctrl Pts',(3.03366873739887,-0.502517375853227,
97.1822006269626));
#22691=CARTESIAN_POINT('Ctrl Pts',(3.01641651283108,-0.597440460058204,
97.1772131793273));
#22692=CARTESIAN_POINT('Ctrl Pts',(2.99472055478194,-0.691412357979333,
97.1722257316919));
#22693=CARTESIAN_POINT('Ctrl Pts',(2.97304012043542,-0.785317017947915,
97.1672418526316));
#22694=CARTESIAN_POINT('Ctrl Pts',(2.94692237185042,-0.878271418115299,
97.1622579735713));
#22695=CARTESIAN_POINT('Ctrl Pts',(2.91647605472128,-0.96982971301018,97.1572740945109));
#22696=CARTESIAN_POINT('Ctrl Pts',(2.88604082512443,-1.06135466543058,97.152292030413));
#22697=CARTESIAN_POINT('Ctrl Pts',(2.8512802973318,-1.15148410663098,97.147309966315));
#22698=CARTESIAN_POINT('Ctrl Pts',(2.81235316369519,-1.23978705133327,97.1423279022171));
#22699=CARTESIAN_POINT('Ctrl Pts',(2.77342957883461,-1.32808194593417,97.1373462923069));
#22700=CARTESIAN_POINT('Ctrl Pts',(2.73034032057302,-1.41455027350001,97.1323646823968));
#22701=CARTESIAN_POINT('Ctrl Pts',(2.68329192137924,-1.49878174350401,97.1273830724866));
#22702=CARTESIAN_POINT('Ctrl Pts',(2.63623496719825,-1.58302852963269,97.1224005567516));
#22703=CARTESIAN_POINT('Ctrl Pts',(2.5852176564402,-1.66503726720775,97.1174180410167));
#22704=CARTESIAN_POINT('Ctrl Pts',(2.53049155840198,-1.74442389425744,97.1124355252817));
#22705=CARTESIAN_POINT('Ctrl Pts',(2.47570647140233,-1.82389609171776,97.1074476389202));
#22706=CARTESIAN_POINT('Ctrl Pts',(2.417204865677,-1.90074017407882,97.1024597525588));
#22707=CARTESIAN_POINT('Ctrl Pts',(2.35528045009995,-1.97460280851035,97.0974718661974));
#22708=CARTESIAN_POINT('Ctrl Pts',(2.29331945369033,-2.04850907608139,97.0924810333239));
#22709=CARTESIAN_POINT('Ctrl Pts',(2.22793191877006,-2.11943006622527,97.0874902004505));
#22710=CARTESIAN_POINT('Ctrl Pts',(2.15944902676273,-2.18704873078162,97.082499367577));
#22711=CARTESIAN_POINT('Ctrl Pts',(2.09085546075036,-2.25477667268014,97.0775004691058));
#22712=CARTESIAN_POINT('Ctrl Pts',(2.01915687537714,-2.3191913393532,97.0725015706345));
#22713=CARTESIAN_POINT('Ctrl Pts',(1.9447181137197,-2.3800154848594,97.0675026721632));
#22714=CARTESIAN_POINT('Ctrl Pts',(1.90150001300119,-2.41532913043965,97.0646003818403));
#22715=CARTESIAN_POINT('Ctrl Pts',(1.85735882408159,-2.44943327562251,97.0616980915173));
#22716=CARTESIAN_POINT('Ctrl Pts',(1.81237015424912,-2.48228053893733,97.0587958011943));
#22717=CARTESIAN_POINT('Ctrl Pts',(1.73487214875217,-2.53886361646355,97.0537962821545));
#22718=CARTESIAN_POINT('Ctrl Pts',(1.65458565811884,-2.59191331061371,97.0487967631147));
#22719=CARTESIAN_POINT('Ctrl Pts',(1.57186646274079,-2.64114332691559,97.0437972440749));
#22720=CARTESIAN_POINT('Ctrl Pts',(1.48925947665256,-2.69030656228299,97.0388045069251));
#22721=CARTESIAN_POINT('Ctrl Pts',(1.40422671830548,-2.73566019496757,97.0338117697752));
#22722=CARTESIAN_POINT('Ctrl Pts',(1.31715500584991,-2.77695965771282,97.0288190326253));
#22723=CARTESIAN_POINT('Ctrl Pts',(1.23017515339638,-2.81821554983537,97.0238315627757));
#22724=CARTESIAN_POINT('Ctrl Pts',(1.14116101755377,-2.85542558755582,97.018844092926));
#22725=CARTESIAN_POINT('Ctrl Pts',(1.05052532509124,-2.88839034608239,97.0138566230763));
#22726=CARTESIAN_POINT('Ctrl Pts',(0.959954487793827,-2.92133151638671,
97.0088727220544));
#22727=CARTESIAN_POINT('Ctrl Pts',(0.867764811876671,-2.95003329678853,
97.0038888210325));
#22728=CARTESIAN_POINT('Ctrl Pts',(0.774389478947485,-2.97434416046554,
96.9989049200107));
#22729=CARTESIAN_POINT('Ctrl Pts',(0.681048153119648,-2.99864617017674,
96.9939228341151));
#22730=CARTESIAN_POINT('Ctrl Pts',(0.586522452611931,-3.01856033004005,
96.9889407482196));
#22731=CARTESIAN_POINT('Ctrl Pts',(0.491260287932881,-3.03398509876039,
96.9839586623241));
#22732=CARTESIAN_POINT('Ctrl Pts',(0.396006811374262,-3.04940846070766,
96.9789770308058));
#22733=CARTESIAN_POINT('Ctrl Pts',(0.300017437531326,-3.06034317557799,
96.9739953992876));
#22734=CARTESIAN_POINT('Ctrl Pts',(0.203748764977606,-3.06673909727745,
96.9690137677693));
#22735=CARTESIAN_POINT('Ctrl Pts',(0.107462591762245,-3.07313618169016,
96.9640312306413));
#22736=CARTESIAN_POINT('Ctrl Pts',(0.010897456992419,-3.07499280520594,
96.9590486935133));
#22737=CARTESIAN_POINT('Ctrl Pts',(-0.085487520602769,-3.07231087844658,
96.9540661563853));
#22738=CARTESIAN_POINT('Ctrl Pts',(-0.181976381768099,-3.06962606111098,
96.949078249087));
#22739=CARTESIAN_POINT('Ctrl Pts',(-0.278284258591738,-3.06239294001798,
96.9440903417887));
#22740=CARTESIAN_POINT('Ctrl Pts',(-0.373954864658887,-3.05066550267281,
96.9391024344904));
#22741=CARTESIAN_POINT('Ctrl Pts',(-0.469681981989062,-3.0389311380976,
96.9341115809064));
#22742=CARTESIAN_POINT('Ctrl Pts',(-0.564770646537324,-3.0226972451083,
96.9291207273223));
#22743=CARTESIAN_POINT('Ctrl Pts',(-0.658774604986502,-3.00206899817857,
96.9241298737383));
#22744=CARTESIAN_POINT('Ctrl Pts',(-0.75293047041527,-2.98140741675168,
96.9191309551163));
#22745=CARTESIAN_POINT('Ctrl Pts',(-0.845997706132988,-2.95633741612214,
96.9141320364943));
#22746=CARTESIAN_POINT('Ctrl Pts',(-0.937545117289906,-2.92701407633203,
96.9091331178723));
#22747=CARTESIAN_POINT('Ctrl Pts',(-0.990692099049544,-2.9099906893759,
96.9062310430516));
#22748=CARTESIAN_POINT('Ctrl Pts',(-1.04332721268546,-2.89153472117561,
96.9033289682308));
#22749=CARTESIAN_POINT('Ctrl Pts',(-1.0953695685853,-2.87168378450993,96.9004268934101));
#22750=CARTESIAN_POINT('Ctrl Pts',(-1.18502535444122,-2.83748565308476,
96.8954273542047));
#22751=CARTESIAN_POINT('Ctrl Pts',(-1.27323553386468,-2.79902477074773,
96.8904278149992));
#22752=CARTESIAN_POINT('Ctrl Pts',(-1.35956625780384,-2.75644369444421,
96.8854282757938));
#22753=CARTESIAN_POINT('Ctrl Pts',(-1.44577987898086,-2.71392037697119,
96.8804355181815));
#22754=CARTESIAN_POINT('Ctrl Pts',(-1.53011872108289,-2.66728816543942,
96.8754427605693));
#22755=CARTESIAN_POINT('Ctrl Pts',(-1.6121670374189,-2.6167383693178,96.870450002957));
#22756=CARTESIAN_POINT('Ctrl Pts',(-1.69412879811219,-2.56624189994666,
96.8654625123797));
#22757=CARTESIAN_POINT('Ctrl Pts',(-1.77380446487575,-2.51183629076463,
96.8604750218023));
#22758=CARTESIAN_POINT('Ctrl Pts',(-1.85080205055773,-2.45375916088994,
96.8554875312249));
#22759=CARTESIAN_POINT('Ctrl Pts',(-1.92774454489346,-2.39572358488013,
96.8505036091695));
#22760=CARTESIAN_POINT('Ctrl Pts',(-2.00201241792848,-2.33402197401046,
96.845519687114));
#22761=CARTESIAN_POINT('Ctrl Pts',(-2.073242722576,-2.26893518269819,96.8405357650585));
#22762=CARTESIAN_POINT('Ctrl Pts',(-2.14444708798958,-2.20387209339751,
96.8355536579486));
#22763=CARTESIAN_POINT('Ctrl Pts',(-2.21261575912116,-2.13542656878813,
96.8305715508386));
#22764=CARTESIAN_POINT('Ctrl Pts',(-2.27741969742316,-2.0639190322755,96.8255894437286));
#22765=CARTESIAN_POINT('Ctrl Pts',(-2.34221772748717,-1.9924180151744,96.8206077908421));
#22766=CARTESIAN_POINT('Ctrl Pts',(-2.40365133999704,-1.91785586658859,
96.8156261379557));
#22767=CARTESIAN_POINT('Ctrl Pts',(-2.46142987624377,-1.84058827941899,
96.8106444850693));
#22768=CARTESIAN_POINT('Ctrl Pts',(-2.51921891746298,-1.76330664388595,
96.8056619264464));
#22769=CARTESIAN_POINT('Ctrl Pts',(-2.57335129978882,-1.6833189444371,96.8006793678235));
#22770=CARTESIAN_POINT('Ctrl Pts',(-2.62357865729354,-1.60101133006417,
96.7956968092006));
#22771=CARTESIAN_POINT('Ctrl Pts',(-2.67386015012781,-1.51861500407966,
96.7907088803479));
#22772=CARTESIAN_POINT('Ctrl Pts',(-2.72022798650951,-1.4338941466383,96.7857209514952));
#22773=CARTESIAN_POINT('Ctrl Pts',(-2.76247902432589,-1.3472608842238,96.7807330226425));
#22774=CARTESIAN_POINT('Ctrl Pts',(-2.80475501967376,-1.26057644786218,
96.7757421474387));
#22775=CARTESIAN_POINT('Ctrl Pts',(-2.84290920085046,-1.17197776018121,
96.7707512722349));
#22776=CARTESIAN_POINT('Ctrl Pts',(-2.87678682353888,-1.08189640073026,
96.7657603970311));
#22777=CARTESIAN_POINT('Ctrl Pts',(-2.91071919022953,-0.991669475748106,
96.7607614569024));
#22778=CARTESIAN_POINT('Ctrl Pts',(-2.94036106451332,-0.89995551231489,
96.7557625167737));
#22779=CARTESIAN_POINT('Ctrl Pts',(-2.9656077610954,-0.807200630160035,
96.7507635766449));
#22780=CARTESIAN_POINT('Ctrl Pts',(-2.98026336204054,-0.753356812052726,
96.7478617129719));
#22781=CARTESIAN_POINT('Ctrl Pts',(-2.99343885263844,-0.699162428364548,
96.7449598492989));
#22782=CARTESIAN_POINT('Ctrl Pts',(-3.00512174427709,-0.644705787218516,
96.7420579856259));
#22783=CARTESIAN_POINT('Ctrl Pts',(-3.03303922606691,-0.51457599276761,
96.7351236812812));
#22784=CARTESIAN_POINT('Ctrl Pts',(-3.05251243821152,-0.382575811799598,
96.7281893769366));
#22785=CARTESIAN_POINT('Ctrl Pts',(-3.0633464197383,-0.2496216390391,96.7212550725919));
#22786=CARTESIAN_POINT('Ctrl Pts',(-3.07002902195233,-0.167613021333926,
96.7169778641204));
#22787=CARTESIAN_POINT('Ctrl Pts',(-3.07342554527863,-0.0852417967828543,
96.7127006556489));
#22788=CARTESIAN_POINT('Ctrl Pts',(-3.07349878913829,-0.00272821653494097,
96.7084234471774));
#22789=CARTESIAN_POINT('Ctrl Pts',(-3.07349878913888,-0.00272821586942156,
96.7084234471429));
#22790=CARTESIAN_POINT('Ctrl Pts',(-3.07358304670424,0.0921929844691349,
96.7035030720848));
#22791=CARTESIAN_POINT('Ctrl Pts',(-3.06926580554714,0.18724875112797,96.6985826970266));
#22792=CARTESIAN_POINT('Ctrl Pts',(-3.06053637932574,0.28199170346609,96.6936623219685));
#22793=CARTESIAN_POINT('Ctrl Pts',(-3.0518144921111,0.37665283281373,96.6887461963009));
#22794=CARTESIAN_POINT('Ctrl Pts',(-3.03868803264072,0.471001235998057,
96.6838300706332));
#22795=CARTESIAN_POINT('Ctrl Pts',(-3.0211983720668,0.564590689456483,96.6789139449656));
#22796=CARTESIAN_POINT('Ctrl Pts',(-3.0037165249272,0.658138332209337,96.674000015557));
#22797=CARTESIAN_POINT('Ctrl Pts',(-2.98187542952173,0.750927254409376,
96.6690860861484));
#22798=CARTESIAN_POINT('Ctrl Pts',(-2.95576803510189,0.842518588916523,
96.6641721567398));
#22799=CARTESIAN_POINT('Ctrl Pts',(-2.9296647045998,0.934095666173676,96.6592589922411));
#22800=CARTESIAN_POINT('Ctrl Pts',(-2.89929651865308,1.02447509116612,96.6543458277424));
#22801=CARTESIAN_POINT('Ctrl Pts',(-2.86480673424856,1.11323161354864,96.6494326632437));
#22802=CARTESIAN_POINT('Ctrl Pts',(-2.8303122788876,1.20200015623968,96.6445188333544));
#22803=CARTESIAN_POINT('Ctrl Pts',(-2.7916952822282,1.28914493889506,96.6396050034651));
#22804=CARTESIAN_POINT('Ctrl Pts',(-2.74914726062367,1.37426037904225,96.6346911735759));
#22805=CARTESIAN_POINT('Ctrl Pts',(-2.70655560981867,1.45946309748023,96.6297723049924));
#22806=CARTESIAN_POINT('Ctrl Pts',(-2.66002509260195,1.54263191558396,96.624853436409));
#22807=CARTESIAN_POINT('Ctrl Pts',(-2.60979313043381,1.62338598809417,96.6199345678255));
#22808=CARTESIAN_POINT('Ctrl Pts',(-2.55953193290358,1.70418706005351,96.6150128364253));
#22809=CARTESIAN_POINT('Ctrl Pts',(-2.5055652614669,1.78257021878091,96.610091105025));
#22810=CARTESIAN_POINT('Ctrl Pts',(-2.44817249361536,1.85818559124356,96.6051693736248));
#22811=CARTESIAN_POINT('Ctrl Pts',(-2.39069007411127,1.93391908038454,96.6002399541243));
#22812=CARTESIAN_POINT('Ctrl Pts',(-2.32977116879369,2.00687581022152,96.5953105346238));
#22813=CARTESIAN_POINT('Ctrl Pts',(-2.26573359723045,2.07674108072748,96.5903811151233));
#22814=CARTESIAN_POINT('Ctrl Pts',(-2.23675507915326,2.10835677062488,96.5881504360295));
#22815=CARTESIAN_POINT('Ctrl Pts',(-2.20713840149301,2.13933992704164,96.5859197569356));
#22816=CARTESIAN_POINT('Ctrl Pts',(-2.17691522278127,2.16966411290392,96.5836890778418));
#22817=CARTESIAN_POINT('Ctrl Pts',(-2.10917614296048,2.23762957961467,96.5786894664299));
#22818=CARTESIAN_POINT('Ctrl Pts',(-2.03813212500065,2.30253904379334,96.573689855018));
#22819=CARTESIAN_POINT('Ctrl Pts',(-1.96409002225505,2.36405427908882,96.5686902436061));
#22820=CARTESIAN_POINT('Ctrl Pts',(-1.89014836370427,2.42548606391423,96.5636974145778));
#22821=CARTESIAN_POINT('Ctrl Pts',(-1.81321703829942,2.48353249300041,96.5587045855495));
#22822=CARTESIAN_POINT('Ctrl Pts',(-1.73364005777044,2.53789172347713,96.5537117565212));
#22823=CARTESIAN_POINT('Ctrl Pts',(-1.6541470385018,2.59219359981109,96.5487241954009));
#22824=CARTESIAN_POINT('Ctrl Pts',(-1.57201427380566,2.64281576503736,96.5437366342807));
#22825=CARTESIAN_POINT('Ctrl Pts',(-1.4876183993823,2.68949693210817,96.5387490731605));
#22826=CARTESIAN_POINT('Ctrl Pts',(-1.40328293555489,2.73614468478352,96.5337650821382));
#22827=CARTESIAN_POINT('Ctrl Pts',(-1.316687965361,2.77885683541977,96.5287810911159));
#22828=CARTESIAN_POINT('Ctrl Pts',(-1.22823779052362,2.81741622411912,96.5237971000936));
#22829=CARTESIAN_POINT('Ctrl Pts',(-1.13981984296242,2.85596156350686,96.5188149250141));
#22830=CARTESIAN_POINT('Ctrl Pts',(-1.04954843576476,2.89035697205567,96.5138327499346));
#22831=CARTESIAN_POINT('Ctrl Pts',(-0.957850206143674,2.92043237082979,
96.5088505748551));
#22832=CARTESIAN_POINT('Ctrl Pts',(-0.86616035638254,2.95050502115795,96.5038688550726));
#22833=CARTESIAN_POINT('Ctrl Pts',(-0.773044360578548,2.97625830999605,
96.4988871352901));
#22834=CARTESIAN_POINT('Ctrl Pts',(-0.678945444151034,2.99757157276796,
96.4939054155076));
#22835=CARTESIAN_POINT('Ctrl Pts',(-0.584829441143728,3.01888870562444,
96.4889227911392));
#22836=CARTESIAN_POINT('Ctrl Pts',(-0.489730591155304,3.03576411432382,
96.4839401667708));
#22837=CARTESIAN_POINT('Ctrl Pts',(-0.394102718476329,3.04812816287137,
96.4789575424024));
#22838=CARTESIAN_POINT('Ctrl Pts',(-0.298371819986878,3.06050553197166,
96.4739695499452));
#22839=CARTESIAN_POINT('Ctrl Pts',(-0.202111196998124,3.06836178126515,
96.468981557488));
#22840=CARTESIAN_POINT('Ctrl Pts',(-0.105779988667777,3.07167915707312,
96.4639935650308));
#22841=CARTESIAN_POINT('Ctrl Pts',(-0.00939190008039556,3.07499849167713,
96.459002627336));
#22842=CARTESIAN_POINT('Ctrl Pts',(0.0870664181326297,3.07377362194052,
96.4540116896412));
#22843=CARTESIAN_POINT('Ctrl Pts',(0.18313776291556,3.06803891921114,96.4490207519465));
#22844=CARTESIAN_POINT('Ctrl Pts',(0.27936430523661,3.06229495241091,96.444021751689));
#22845=CARTESIAN_POINT('Ctrl Pts',(0.375202189722728,3.05202665207337,96.4390227514315));
#22846=CARTESIAN_POINT('Ctrl Pts',(0.470201313175157,3.03732003172013,96.434023751174));
#22847=CARTESIAN_POINT('Ctrl Pts',(0.525334508772668,3.02878497426857,96.4311225574685));
#22848=CARTESIAN_POINT('Ctrl Pts',(0.580185407945726,3.01875599274042,96.428221363763));
#22849=CARTESIAN_POINT('Ctrl Pts',(0.634668328288215,3.00725761501536,96.4253201700575));
#22850=CARTESIAN_POINT('Ctrl Pts',(0.728566358212649,2.98744085392906,96.4203201375397));
#22851=CARTESIAN_POINT('Ctrl Pts',(0.821700203521094,2.96318730838223,96.4153201050219));
#22852=CARTESIAN_POINT('Ctrl Pts',(0.91361899032501,2.93457025653119,96.4103200725041));
#22853=CARTESIAN_POINT('Ctrl Pts',(1.00539028441085,2.90599912354947,96.4053280630295));
#22854=CARTESIAN_POINT('Ctrl Pts',(1.09594998283726,2.87307854152665,96.4003360535548));
#22855=CARTESIAN_POINT('Ctrl Pts',(1.18485783210905,2.8359326803875,96.3953440440801));
#22856=CARTESIAN_POINT('Ctrl Pts',(1.27368277071042,2.79882145947726,96.3903566898845));
#22857=CARTESIAN_POINT('Ctrl Pts',(1.36085851744708,2.75749295450866,96.3853693356889));
#22858=CARTESIAN_POINT('Ctrl Pts',(1.44596091047329,2.7121208113547,96.3803819814933));
#22859=CARTESIAN_POINT('Ctrl Pts',(1.53100536935423,2.66677955565571,96.3753980224795));
#22860=CARTESIAN_POINT('Ctrl Pts',(1.61397889340451,2.61740033821018,96.3704140634658));
#22861=CARTESIAN_POINT('Ctrl Pts',(1.69447922616217,2.56420404845341,96.3654301044521));
#22862=CARTESIAN_POINT('Ctrl Pts',(1.75524321035264,2.5240499472337,96.3616680677457));
#22863=CARTESIAN_POINT('Ctrl Pts',(1.81459844688948,2.48172200613711,96.3579060310392));
#22864=CARTESIAN_POINT('Ctrl Pts',(1.87238193903531,2.43733217358126,96.3541439943328));
#22865=CARTESIAN_POINT('',(-3.07349915159075,0.00228367488303187,96.7915765528226));
#22866=CARTESIAN_POINT('Ctrl Pts',(-3.07056037769426,0.00230326753188174,
96.7915754276343));
#22867=CARTESIAN_POINT('Ctrl Pts',(-3.07296424660638,0.349288135212611,
96.7736466355977));
#22868=CARTESIAN_POINT('Ctrl Pts',(-2.85878184482725,1.71505316958018,96.7029282076332));
#22869=CARTESIAN_POINT('Ctrl Pts',(-0.943444564451998,3.44751893046241,
96.5848744668941));
#22870=CARTESIAN_POINT('Ctrl Pts',(1.14803854905623,2.98990927824168,96.4847495181914));
#22871=CARTESIAN_POINT('Ctrl Pts',(1.87462644597698,2.44029756596839,96.4374142054168));
#22872=CARTESIAN_POINT('Ctrl Pts',(1.8723819390353,2.43733217358127,97.4373604997054));
#22873=CARTESIAN_POINT('Ctrl Pts',(1.94890431270062,2.37854695261874,97.4323776874656));
#22874=CARTESIAN_POINT('Ctrl Pts',(2.02263347195522,2.3161715702656,97.4273948752259));
#22875=CARTESIAN_POINT('Ctrl Pts',(2.09322696924329,2.25051174296704,97.4224120629862));
#22876=CARTESIAN_POINT('Ctrl Pts',(2.16389828936707,2.18477953175001,97.4174237576544));
#22877=CARTESIAN_POINT('Ctrl Pts',(2.23142672611253,2.11575594801334,97.4124354523226));
#22878=CARTESIAN_POINT('Ctrl Pts',(2.29550652016526,2.04378376201563,97.4074471469909));
#22879=CARTESIAN_POINT('Ctrl Pts',(2.3596267818964,1.97176612413531,97.402455691444));
#22880=CARTESIAN_POINT('Ctrl Pts',(2.42029378929588,1.89679651771012,97.3974642358971));
#22881=CARTESIAN_POINT('Ctrl Pts',(2.47724324675447,1.81924933596508,97.3924727803502));
#22882=CARTESIAN_POINT('Ctrl Pts',(2.53428199789625,1.74158056441412,97.3874734984698));
#22883=CARTESIAN_POINT('Ctrl Pts',(2.5875913217096,1.66132651533092,97.3824742165893));
#22884=CARTESIAN_POINT('Ctrl Pts',(2.63695134636908,1.57888880130372,97.3774749347089));
#22885=CARTESIAN_POINT('Ctrl Pts',(2.65739016148488,1.54475329980844,97.3754048506931));
#22886=CARTESIAN_POINT('Ctrl Pts',(2.67715239088241,1.51024365654688,97.3733347666773));
#22887=CARTESIAN_POINT('Ctrl Pts',(2.69622482896227,1.47538941357438,97.3712646826615));
#22888=CARTESIAN_POINT('Ctrl Pts',(2.7422871163402,1.39121212331832,97.3662651747626));
#22889=CARTESIAN_POINT('Ctrl Pts',(2.78448445429822,1.30472778727541,97.3612656668637));
#22890=CARTESIAN_POINT('Ctrl Pts',(2.82257907131634,1.21632628688481,97.3562661589648));
#22891=CARTESIAN_POINT('Ctrl Pts',(2.86062201321497,1.12804470259924,97.3512734328684));
#22892=CARTESIAN_POINT('Ctrl Pts',(2.89457312263953,1.03785152220718,97.346280706772));
#22893=CARTESIAN_POINT('Ctrl Pts',(2.92424002577248,0.946161995469138,97.3412879806756));
#22894=CARTESIAN_POINT('Ctrl Pts',(2.95387563107546,0.854569198855065,97.3363005217785));
#22895=CARTESIAN_POINT('Ctrl Pts',(2.9792358806208,0.761483609495415,97.3313130628814));
#22896=CARTESIAN_POINT('Ctrl Pts',(3.00017652003359,0.667340316959154,97.3263256039843));
#22897=CARTESIAN_POINT('Ctrl Pts',(3.02110217596745,0.573264385978197,97.3213417137216));
#22898=CARTESIAN_POINT('Ctrl Pts',(3.03761441328648,0.478132683583798,97.3163578234589));
#22899=CARTESIAN_POINT('Ctrl Pts',(3.04961912253582,0.382394374257599,97.3113739331962));
#22900=CARTESIAN_POINT('Ctrl Pts',(3.06161945998259,0.286690930331169,97.3063918579365));
#22901=CARTESIAN_POINT('Ctrl Pts',(3.06911547633185,0.190381753504808,97.3014097826769));
#22902=CARTESIAN_POINT('Ctrl Pts',(3.07206453494666,0.0939241349331538,
97.2964277074172));
#22903=CARTESIAN_POINT('Ctrl Pts',(3.07501332468038,-0.00252468909283135,
97.2914460863994));
#22904=CARTESIAN_POINT('Ctrl Pts',(3.07341596769022,-0.0991214891924568,
97.2864644653817));
#22905=CARTESIAN_POINT('Ctrl Pts',(3.06728191506374,-0.195407020147495,
97.2814828443639));
#22906=CARTESIAN_POINT('Ctrl Pts',(3.06114674714497,-0.291710057719588,
97.2765003175887));
#22907=CARTESIAN_POINT('Ctrl Pts',(3.05047327335789,-0.387701275681762,
97.2715177908135));
#22908=CARTESIAN_POINT('Ctrl Pts',(3.03532288909604,-0.482925676403381,
97.2665352640384));
#22909=CARTESIAN_POINT('Ctrl Pts',(3.02015617486979,-0.57825271551669,97.2615473668064));
#22910=CARTESIAN_POINT('Ctrl Pts',(3.00050298564189,-0.672810853089337,
97.2565594695743));
#22911=CARTESIAN_POINT('Ctrl Pts',(2.97647598743741,-0.766154649015789,
97.2515715723423));
#22912=CARTESIAN_POINT('Ctrl Pts',(2.95243479609223,-0.859553584648742,
97.2465807286778));
#22913=CARTESIAN_POINT('Ctrl Pts',(2.92401478050595,-0.951736331027809,
97.2415898850134));
#22914=CARTESIAN_POINT('Ctrl Pts',(2.89137806169206,-1.04227403036142,97.2365990413489));
#22915=CARTESIAN_POINT('Ctrl Pts',(2.85868860087712,-1.13295804156727,97.2316001323184));
#22916=CARTESIAN_POINT('Ctrl Pts',(2.82176899815312,-1.22199129218172,97.226601223288));
#22917=CARTESIAN_POINT('Ctrl Pts',(2.78082890764678,-1.30896632362946,97.2216023142575));
#22918=CARTESIAN_POINT('Ctrl Pts',(2.75706062086986,-1.35946077697127,97.2187001344641));
#22919=CARTESIAN_POINT('Ctrl Pts',(2.73193807334052,-1.40926197064841,97.2157979546707));
#22920=CARTESIAN_POINT('Ctrl Pts',(2.70550904928966,-1.45829456359536,97.2128957748773));
#22921=CARTESIAN_POINT('Ctrl Pts',(2.65998045166647,-1.54276174597812,97.2078962646499));
#22922=CARTESIAN_POINT('Ctrl Pts',(2.61041244107992,-1.62524311105927,97.2028967544224));
#22923=CARTESIAN_POINT('Ctrl Pts',(2.55700259225754,-1.70532694612741,97.1978972441949));
#22924=CARTESIAN_POINT('Ctrl Pts',(2.50366519367961,-1.78530214779636,97.1929045157829));
#22925=CARTESIAN_POINT('Ctrl Pts',(2.44649655572826,-1.86288592099231,97.1879117873709));
#22926=CARTESIAN_POINT('Ctrl Pts',(2.38574024872595,-1.93769082043783,97.1829190589589));
#22927=CARTESIAN_POINT('Ctrl Pts',(2.32504803824859,-2.01241680241223,97.1779315977621));
#22928=CARTESIAN_POINT('Ctrl Pts',(2.26077595816414,-2.08436939965339,97.1729441365652));
#22929=CARTESIAN_POINT('Ctrl Pts',(2.19321041897331,-2.15319072729448,97.1679566753684));
#22930=CARTESIAN_POINT('Ctrl Pts',(2.12569322480403,-2.22196281136246,97.1629727828387));
#22931=CARTESIAN_POINT('Ctrl Pts',(2.05488756290188,-2.28760776751967,97.157988890309));
#22932=CARTESIAN_POINT('Ctrl Pts',(1.98111895117006,-2.34980210896894,97.1530049977793));
#22933=CARTESIAN_POINT('Ctrl Pts',(1.90737720434542,-2.41197380060588,97.1480229202737));
#22934=CARTESIAN_POINT('Ctrl Pts',(1.83067498688838,-2.47069709168082,97.1430408427681));
#22935=CARTESIAN_POINT('Ctrl Pts',(1.75137265774965,-2.52568724581785,97.1380587652625));
#22936=CARTESIAN_POINT('Ctrl Pts',(1.67207755939211,-2.5806723859562,97.1330771420224));
#22937=CARTESIAN_POINT('Ctrl Pts',(1.59018318153496,-2.63192481592623,97.1280955187823));
#22938=CARTESIAN_POINT('Ctrl Pts',(1.50607988143107,-2.67920242623595,97.1231138955423));
#22939=CARTESIAN_POINT('Ctrl Pts',(1.42196129013103,-2.72648863229888,97.118131366571));
#22940=CARTESIAN_POINT('Ctrl Pts',(1.33563336163968,-2.76979836839094,97.1131488375998));
#22941=CARTESIAN_POINT('Ctrl Pts',(1.24751117153615,-2.8089354081026,97.1081663086286));
#22942=CARTESIAN_POINT('Ctrl Pts',(1.15929399919801,-2.84811463155348,97.1031784092537));
#22943=CARTESIAN_POINT('Ctrl Pts',(1.06927910615813,-2.88311200125748,97.0981905098788));
#22944=CARTESIAN_POINT('Ctrl Pts',(0.97790146560417,-2.91377949981964,97.0932026105038));
#22945=CARTESIAN_POINT('Ctrl Pts',(0.88646984729801,-2.94446511400208,97.0882117647233));
#22946=CARTESIAN_POINT('Ctrl Pts',(0.793674300682157,-2.97081564438874,
97.0832209189427));
#22947=CARTESIAN_POINT('Ctrl Pts',(0.699962815698049,-2.99273358430717,
97.0782300731621));
#22948=CARTESIAN_POINT('Ctrl Pts',(0.606099891146746,-3.01468694403926,
97.0732311620785));
#22949=CARTESIAN_POINT('Ctrl Pts',(0.511318504016708,-3.03219333039695,
97.0682322509949));
#22950=CARTESIAN_POINT('Ctrl Pts',(0.41607457425234,-3.04520675794941,97.0632333399113));
#22951=CARTESIAN_POINT('Ctrl Pts',(0.360779952969739,-3.0527618068631,97.0603311823052));
#22952=CARTESIAN_POINT('Ctrl Pts',(0.305329505627397,-3.05880348903059,
97.0574290246992));
#22953=CARTESIAN_POINT('Ctrl Pts',(0.249812441843652,-3.06333086588767,
97.0545268670932));
#22954=CARTESIAN_POINT('Ctrl Pts',(0.154173822864202,-3.07113012688421,
97.0495273529513));
#22955=CARTESIAN_POINT('Ctrl Pts',(0.0580016288474361,-3.0744599702639,
97.0445278388095));
#22956=CARTESIAN_POINT('Ctrl Pts',(-0.0382512281636187,-3.07326196305228,
97.0395283246676));
#22957=CARTESIAN_POINT('Ctrl Pts',(-0.134373519396679,-3.07206558092223,
97.0345355923032));
#22958=CARTESIAN_POINT('Ctrl Pts',(-0.230575820989438,-3.06635356038032,
97.0295428599388));
#22959=CARTESIAN_POINT('Ctrl Pts',(-0.326400533937449,-3.05611926165282,
97.0245501275743));
#22960=CARTESIAN_POINT('Ctrl Pts',(-0.42212415468589,-3.04589575980367,
97.0195626623929));
#22961=CARTESIAN_POINT('Ctrl Pts',(-0.517470544516665,-3.03115951033572,
97.0145751972114));
#22962=CARTESIAN_POINT('Ctrl Pts',(-0.611983575133122,-3.01195590169698,
97.00958773203));
#22963=CARTESIAN_POINT('Ctrl Pts',(-0.70642897969296,-2.99276603364318,
97.0046038354845));
#22964=CARTESIAN_POINT('Ctrl Pts',(-0.800041781488772,-2.96911524804222,
96.999619938939));
#22965=CARTESIAN_POINT('Ctrl Pts',(-0.892373413025865,-2.94110046440521,
96.9946360423936));
#22966=CARTESIAN_POINT('Ctrl Pts',(-0.984671419767091,-2.91309588302897,
96.9896539608546));
#22967=CARTESIAN_POINT('Ctrl Pts',(-1.0756887636492,-2.88073058861448,96.9846718793155));
#22968=CARTESIAN_POINT('Ctrl Pts',(-1.16499041151238,-2.8441518227908,96.9796897977765));
#22969=CARTESIAN_POINT('Ctrl Pts',(-1.25428391709092,-2.80757639212084,
96.9747081704903));
#22970=CARTESIAN_POINT('Ctrl Pts',(-1.34186163153142,-2.76678842040393,
96.9697265432041));
#22971=CARTESIAN_POINT('Ctrl Pts',(-1.42730794418423,-2.72198351987454,
96.9647449159178));
#22972=CARTESIAN_POINT('Ctrl Pts',(-1.51276979233033,-2.67717047310444,
96.9597623828929));
#22973=CARTESIAN_POINT('Ctrl Pts',(-1.59609908033135,-2.62833925094222,
96.9547798498679));
#22974=CARTESIAN_POINT('Ctrl Pts',(-1.67690522600176,-2.57573118026862,
96.9497973168429));
#22975=CARTESIAN_POINT('Ctrl Pts',(-1.75779846804352,-2.5230664063329,96.9448094134276));
#22976=CARTESIAN_POINT('Ctrl Pts',(-1.83616276994022,-2.46661689670211,
96.9398215100122));
#22977=CARTESIAN_POINT('Ctrl Pts',(-1.91163715358443,-2.40666691568144,
96.9348336065969));
#22978=CARTESIAN_POINT('Ctrl Pts',(-1.98715612069678,-2.34668152161148,
96.9298427567775));
#22979=CARTESIAN_POINT('Ctrl Pts',(-2.05978144010712,-2.28319182767184,
96.924851906958));
#22980=CARTESIAN_POINT('Ctrl Pts',(-2.12918741472047,-2.21652051716107,
96.9198610571386));
#22981=CARTESIAN_POINT('Ctrl Pts',(-2.19870555004368,-2.14974146518342,
96.9148621420588));
#22982=CARTESIAN_POINT('Ctrl Pts',(-2.26499365065353,-2.07977084860068,
96.9098632269789));
#22983=CARTESIAN_POINT('Ctrl Pts',(-2.32776491757109,-2.00696605315716,
96.9048643118991));
#22984=CARTESIAN_POINT('Ctrl Pts',(-2.36420674368624,-1.96469926731411,
96.9019621943691));
#22985=CARTESIAN_POINT('Ctrl Pts',(-2.39946404159902,-1.92147784769679,
96.899060076839));
#22986=CARTESIAN_POINT('Ctrl Pts',(-2.43348745577258,-1.87737610845496,
96.896157959309));
#22987=CARTESIAN_POINT('Ctrl Pts',(-2.49213133510029,-1.80136089548879,
96.8911557737741));
#22988=CARTESIAN_POINT('Ctrl Pts',(-2.54731629060798,-1.72245755890727,
96.8861535882393));
#22989=CARTESIAN_POINT('Ctrl Pts',(-2.59874527060311,-1.64101348821939,
96.8811514027044));
#22990=CARTESIAN_POINT('Ctrl Pts',(-2.65010560182581,-1.55967813124652,
96.87615589422));
#22991=CARTESIAN_POINT('Ctrl Pts',(-2.69771968649096,-1.47580914427467,
96.8711603857356));
#22992=CARTESIAN_POINT('Ctrl Pts',(-2.74133111800883,-1.38978629703868,
96.8661648772513));
#22993=CARTESIAN_POINT('Ctrl Pts',(-2.78489616873654,-1.30385493516529,
96.8611746814939));
#22994=CARTESIAN_POINT('Ctrl Pts',(-2.82446682901955,-1.21577465312144,
96.8561844857365));
#22995=CARTESIAN_POINT('Ctrl Pts',(-2.8598309453293,-1.12595258076746,96.8511942899792));
#22996=CARTESIAN_POINT('Ctrl Pts',(-2.89516771522501,-1.03619996615305,
96.8462079530475));
#22997=CARTESIAN_POINT('Ctrl Pts',(-2.92630424711921,-0.944708644435166,
96.8412216161158));
#22998=CARTESIAN_POINT('Ctrl Pts',(-2.95307560184055,-0.851907706159584,
96.8362352791841));
#22999=CARTESIAN_POINT('Ctrl Pts',(-2.97983400188649,-0.759151674316428,
96.831251355144));
#23000=CARTESIAN_POINT('Ctrl Pts',(-3.00223130379482,-0.665087706013686,
96.8262674311039));
#23001=CARTESIAN_POINT('Ctrl Pts',(-3.0201520710862,-0.570161132938504,
96.8212835070637));
#23002=CARTESIAN_POINT('Ctrl Pts',(-3.03807483177263,-0.475224000819851,
96.8162990286428));
#23003=CARTESIAN_POINT('Ctrl Pts',(-3.05151996977012,-0.379424500303791,
96.8113145502219));
#23004=CARTESIAN_POINT('Ctrl Pts',(-3.06042308111738,-0.283218669165731,
96.806330071801));
#23005=CARTESIAN_POINT('Ctrl Pts',(-3.06920716450155,-0.188299038286348,
96.8014122321415));
#23006=CARTESIAN_POINT('Ctrl Pts',(-3.07356993770723,-0.0929842945523692,
96.7964943924821));
#23007=CARTESIAN_POINT('Ctrl Pts',(-3.07349915159074,0.00228367488303187,
96.7915765528226));
#23008=CARTESIAN_POINT('Origin',(0.,0.,116.208423447177));
#23009=CARTESIAN_POINT('',(1.8723819390353,2.43733217358127,98.4372333997809));
#23010=CARTESIAN_POINT('',(1.87238193903531,2.43733217358127,98.354260042891));
#23011=CARTESIAN_POINT('',(1.8723819390353,2.43733217358128,116.208423447177));
#23012=CARTESIAN_POINT('',(-3.07349950430575,0.00174557505997315,97.7084234472127));
#23013=CARTESIAN_POINT('Ctrl Pts',(1.87238193903531,2.43733217358127,98.354260042891));
#23014=CARTESIAN_POINT('Ctrl Pts',(1.94887360315701,2.37857054398451,98.3492617290814));
#23015=CARTESIAN_POINT('Ctrl Pts',(2.02251066494388,2.31627054257947,98.3442634152718));
#23016=CARTESIAN_POINT('Ctrl Pts',(2.09296620165726,2.25075425773681,98.3392651014622));
#23017=CARTESIAN_POINT('Ctrl Pts',(2.15648232986216,2.19169089747168,98.3347590887974));
#23018=CARTESIAN_POINT('Ctrl Pts',(2.21741311751157,2.13001428347652,98.3302530761326));
#23019=CARTESIAN_POINT('Ctrl Pts',(2.27554719676962,2.06598335067684,98.3257470634677));
#23020=CARTESIAN_POINT('Ctrl Pts',(2.3400480999962,1.99493977257722,98.3207475538764));
#23021=CARTESIAN_POINT('Ctrl Pts',(2.40133208819396,1.92074789682503,98.3157480442851));
#23022=CARTESIAN_POINT('Ctrl Pts',(2.4590766680417,1.84373105161598,98.3107485346938));
#23023=CARTESIAN_POINT('Ctrl Pts',(2.51674291773897,1.76681867926115,98.305755806905));
#23024=CARTESIAN_POINT('Ctrl Pts',(2.57087904005066,1.68708930160601,98.3007630791163));
#23025=CARTESIAN_POINT('Ctrl Pts',(2.62120073287719,1.60490154463259,98.2957703513275));
#23026=CARTESIAN_POINT('Ctrl Pts',(2.67146933758932,1.52280049366606,98.2907828907404));
#23027=CARTESIAN_POINT('Ctrl Pts',(2.7179312845413,1.4382465915319,98.2857954301533));
#23028=CARTESIAN_POINT('Ctrl Pts',(2.76034440402892,1.35162902497181,98.2808079695662));
#23029=CARTESIAN_POINT('Ctrl Pts',(2.80272717593779,1.26507343530597,98.2758240776237));
#23030=CARTESIAN_POINT('Ctrl Pts',(2.84106668705415,1.17645750973203,98.2708401856813));
#23031=CARTESIAN_POINT('Ctrl Pts',(2.87516621973593,1.08619586580386,98.2658562937389));
#23032=CARTESIAN_POINT('Ctrl Pts',(2.909253334212,0.995967092932087,98.2608742168065));
#23033=CARTESIAN_POINT('Ctrl Pts',(2.93910338322924,0.904094202725765,98.2558921398742));
#23034=CARTESIAN_POINT('Ctrl Pts',(2.96456778565997,0.811011771941172,98.2509100629418));
#23035=CARTESIAN_POINT('Ctrl Pts',(2.99002986632277,0.717937828133745,98.2459284402603));
#23036=CARTESIAN_POINT('Ctrl Pts',(3.01110697976169,0.623654986462369,98.2409468175788));
#23037=CARTESIAN_POINT('Ctrl Pts',(3.02770072523178,0.528611926114938,98.2359651948973));
#23038=CARTESIAN_POINT('Ctrl Pts',(3.04429748773597,0.43355158527145,98.2309826664694));
#23039=CARTESIAN_POINT('Ctrl Pts',(3.05640918791082,0.337731183667423,98.2260001380414));
#23040=CARTESIAN_POINT('Ctrl Pts',(3.06398891884574,0.241607440263167,98.2210176096135));
#23041=CARTESIAN_POINT('Ctrl Pts',(3.07157681961165,0.145380089653701,98.2160297107555));
#23042=CARTESIAN_POINT('Ctrl Pts',(3.07462296453397,0.0488491828327223,
98.2110418118975));
#23043=CARTESIAN_POINT('Ctrl Pts',(3.07313252958506,-0.0475258414563746,
98.2060539130394));
#23044=CARTESIAN_POINT('Ctrl Pts',(3.07164121421593,-0.143957795784586,
98.2010630677616));
#23045=CARTESIAN_POINT('Ctrl Pts',(3.0656080104583,-0.240233246332413,98.1960722224838));
#23046=CARTESIAN_POINT('Ctrl Pts',(3.05509005777202,-0.335897289215853,
98.191081377206));
#23047=CARTESIAN_POINT('Ctrl Pts',(3.04455510781254,-0.431715927572407,
98.1860824665981));
#23048=CARTESIAN_POINT('Ctrl Pts',(3.02952100576024,-0.526920752049771,
98.1810835559902));
#23049=CARTESIAN_POINT('Ctrl Pts',(3.01009611464282,-0.621066526720114,
98.1760846453823));
#23050=CARTESIAN_POINT('Ctrl Pts',(2.99881881660216,-0.675723716498384,
98.1731824821494));
#23051=CARTESIAN_POINT('Ctrl Pts',(2.98606255056658,-0.730024210174861,
98.1702803189164));
#23052=CARTESIAN_POINT('Ctrl Pts',(2.97185612004777,-0.783883570267034,
98.1673781556835));
#23053=CARTESIAN_POINT('Ctrl Pts',(2.94738293373129,-0.876666212090917,
98.162378646382));
#23054=CARTESIAN_POINT('Ctrl Pts',(2.91851752568576,-0.968464626203716,
98.1573791370805));
#23055=CARTESIAN_POINT('Ctrl Pts',(2.88535551907953,-1.05883227119186,98.152379627779));
#23056=CARTESIAN_POINT('Ctrl Pts',(2.85223849652507,-1.14907733304233,98.1473869002802));
#23057=CARTESIAN_POINT('Ctrl Pts',(2.81483660871829,-1.23789507447157,98.1423941727814));
#23058=CARTESIAN_POINT('Ctrl Pts',(2.77329587960945,-1.32485177062993,98.1374014452826));
#23059=CARTESIAN_POINT('Ctrl Pts',(2.73179897492065,-1.41171672967004,98.1324139849852));
#23060=CARTESIAN_POINT('Ctrl Pts',(2.68617209722699,-1.49672415249134,98.1274265246878));
#23061=CARTESIAN_POINT('Ctrl Pts',(2.63660984365751,-1.57945901571656,98.1224390643904));
#23062=CARTESIAN_POINT('Ctrl Pts',(2.587083053026,-1.66213468023488,98.1174551727361));
#23063=CARTESIAN_POINT('Ctrl Pts',(2.53362670923431,-1.74254064222001,98.1124712810818));
#23064=CARTESIAN_POINT('Ctrl Pts',(2.47648148702774,-1.8202861572865,98.1074873894275));
#23065=CARTESIAN_POINT('Ctrl Pts',(2.41935707568555,-1.89800335937587,98.1025053127822));
#23066=CARTESIAN_POINT('Ctrl Pts',(2.35854671482401,-1.97306168624915,98.097523236137));
#23067=CARTESIAN_POINT('Ctrl Pts',(2.29433402881454,-2.04509990323789,98.0925411594917));
#23068=CARTESIAN_POINT('Ctrl Pts',(2.23012719750764,-2.11713155201776,98.0875595370958));
#23069=CARTESIAN_POINT('Ctrl Pts',(2.16251895003478,-2.18614331082863,98.0825779147));
#23070=CARTESIAN_POINT('Ctrl Pts',(2.09183206056623,-2.25180835782871,98.0775962923042));
#23071=CARTESIAN_POINT('Ctrl Pts',(2.02113231895527,-2.31748534391032,98.0726137641602));
#23072=CARTESIAN_POINT('Ctrl Pts',(1.94735314530763,-2.37981411098498,98.0676312360162));
#23073=CARTESIAN_POINT('Ctrl Pts',(1.87085209339092,-2.43850665257547,98.0626487078722));
#23074=CARTESIAN_POINT('Ctrl Pts',(1.79426858456159,-2.49726245611664,98.0576608092937));
#23075=CARTESIAN_POINT('Ctrl Pts',(1.71495768928043,-2.55237394197662,98.0526729107152));
#23076=CARTESIAN_POINT('Ctrl Pts',(1.63330759925468,-2.60359530960879,98.0476850121367));
#23077=CARTESIAN_POINT('Ctrl Pts',(1.55160927737255,-2.65484693442313,98.0426941671364));
#23078=CARTESIAN_POINT('Ctrl Pts',(1.46756939161196,-2.70220365002367,98.0377033221361));
#23079=CARTESIAN_POINT('Ctrl Pts',(1.38160062147527,-2.74546571144845,98.0327124771357));
#23080=CARTESIAN_POINT('Ctrl Pts',(1.29549292355664,-2.78879768549646,98.0277135667993));
#23081=CARTESIAN_POINT('Ctrl Pts',(1.20745051774667,-2.82802161402931,98.0227146564629));
#23082=CARTESIAN_POINT('Ctrl Pts',(1.11790586289056,-2.86298598175313,98.0177157461265));
#23083=CARTESIAN_POINT('Ctrl Pts',(1.06591984151815,-2.88328488592205,98.0148135800507));
#23084=CARTESIAN_POINT('Ctrl Pts',(1.01342778663993,-2.9021490366,98.011911413975));
#23085=CARTESIAN_POINT('Ctrl Pts',(0.960516206142954,-2.91955662177269,
98.0090092478992));
#23086=CARTESIAN_POINT('Ctrl Pts',(0.869366374068857,-2.94954435697928,
98.0040097383784));
#23087=CARTESIAN_POINT('Ctrl Pts',(0.776650752559451,-2.97531206584531,
97.9990102288576));
#23088=CARTESIAN_POINT('Ctrl Pts',(0.682795959320957,-2.99669683617395,
97.9940107193368));
#23089=CARTESIAN_POINT('Ctrl Pts',(0.589068479545639,-3.01805259819012,
97.9890179916206));
#23090=CARTESIAN_POINT('Ctrl Pts',(0.4942053235143,-3.03503714113321,97.9840252639044));
#23091=CARTESIAN_POINT('Ctrl Pts',(0.39864979928181,-3.04753680659194,97.9790325361882));
#23092=CARTESIAN_POINT('Ctrl Pts',(0.303195083751813,-3.06002328521435,
97.9740450756756));
#23093=CARTESIAN_POINT('Ctrl Pts',(0.20704988501364,-3.06803423552479,97.9690576151631));
#23094=CARTESIAN_POINT('Ctrl Pts',(0.110668270214102,-3.07150692396547,
97.9640701546505));
#23095=CARTESIAN_POINT('Ctrl Pts',(0.0143556187644802,-3.07497712761453,
97.9590862627852));
#23096=CARTESIAN_POINT('Ctrl Pts',(-0.082192675041899,-3.07391550898284,
97.9541023709199));
#23097=CARTESIAN_POINT('Ctrl Pts',(-0.178517822059432,-3.06831120279661,
97.9491184790546));
#23098=CARTESIAN_POINT('Ctrl Pts',(-0.2748078898121,-3.06270893756175,97.9441364022009));
#23099=CARTESIAN_POINT('Ctrl Pts',(-0.370874534466474,-3.0525672972281,
97.9391543253472));
#23100=CARTESIAN_POINT('Ctrl Pts',(-0.466260335408199,-3.03792750894833,
97.9341722484936));
#23101=CARTESIAN_POINT('Ctrl Pts',(-0.561637439330315,-3.02328905548491,
97.9291906258922));
#23102=CARTESIAN_POINT('Ctrl Pts',(-0.656333389107419,-3.00415333626096,
97.9242090032908));
#23103=CARTESIAN_POINT('Ctrl Pts',(-0.749898314168346,-2.98061315309576,
97.9192273806894));
#23104=CARTESIAN_POINT('Ctrl Pts',(-0.843480250949397,-2.9570686899185,
97.914244852343));
#23105=CARTESIAN_POINT('Ctrl Pts',(-0.935930328930217,-2.92911827952979,
97.9092623239966));
#23106=CARTESIAN_POINT('Ctrl Pts',(-1.0268122997602,-2.8969050296931,97.9042797956501));
#23107=CARTESIAN_POINT('Ctrl Pts',(-1.11779222791188,-2.86465705873792,
97.8992918968751));
#23108=CARTESIAN_POINT('Ctrl Pts',(-1.20720026018258,-2.82813722231406,
97.8943039981001));
#23109=CARTESIAN_POINT('Ctrl Pts',(-1.2946188693551,-2.78753730613775,97.8893160993251));
#23110=CARTESIAN_POINT('Ctrl Pts',(-1.3820891178739,-2.74691340704579,97.8843252541313));
#23111=CARTESIAN_POINT('Ctrl Pts',(-1.4675672145334,-2.70220483253513,97.8793344089376));
#23112=CARTESIAN_POINT('Ctrl Pts',(-1.55066093076454,-2.65364898353201,
97.8743435637438));
#23113=CARTESIAN_POINT('Ctrl Pts',(-1.63388892849863,-2.60501466707458,
97.8693446532206));
#23114=CARTESIAN_POINT('Ctrl Pts',(-1.71472448388021,-2.55252090047919,
97.8643457426974));
#23115=CARTESIAN_POINT('Ctrl Pts',(-1.7928050541175,-2.49644793415179,97.8593468321742));
#23116=CARTESIAN_POINT('Ctrl Pts',(-1.83813545571699,-2.46389425178534,
97.8564446681545));
#23117=CARTESIAN_POINT('Ctrl Pts',(-1.88253790919386,-2.43013496034154,
97.8535425041349));
#23118=CARTESIAN_POINT('Ctrl Pts',(-1.92594701958118,-2.39523074624688,
97.8506403401152));
#23119=CARTESIAN_POINT('Ctrl Pts',(-1.99978831977924,-2.33585674553263,
97.8457035984338));
#23120=CARTESIAN_POINT('Ctrl Pts',(-2.07102703883305,-2.27294759451819,
97.8407668567525));
#23121=CARTESIAN_POINT('Ctrl Pts',(-2.1392990935973,-2.20676270544292,97.8358301150711));
#23122=CARTESIAN_POINT('Ctrl Pts',(-2.20747811774654,-2.14066800291552,
97.8309001004191));
#23123=CARTESIAN_POINT('Ctrl Pts',(-2.27269818618689,-2.07130673938253,
97.8259700857671));
#23124=CARTESIAN_POINT('Ctrl Pts',(-2.33462698575195,-1.9989795115005,97.8210400711151));
#23125=CARTESIAN_POINT('Ctrl Pts',(-2.39648614566971,-1.92673361641799,
97.8161156003212));
#23126=CARTESIAN_POINT('Ctrl Pts',(-2.45506110199223,-1.85152872758815,
97.8111911295274));
#23127=CARTESIAN_POINT('Ctrl Pts',(-2.51005617571016,-1.77370241156155,
97.8062666587335));
#23128=CARTESIAN_POINT('Ctrl Pts',(-2.56501759495709,-1.69592372168251,
97.8013452014907));
#23129=CARTESIAN_POINT('Ctrl Pts',(-2.61640322143425,-1.61552715686622,
97.7964237442478));
#23130=CARTESIAN_POINT('Ctrl Pts',(-2.66395808802082,-1.53288275979229,
97.791502287005));
#23131=CARTESIAN_POINT('Ctrl Pts',(-2.71149762595039,-1.45026500200278,
97.7865824161262));
#23132=CARTESIAN_POINT('Ctrl Pts',(-2.75520863196226,-1.36540124188588,
97.7816625452474));
#23133=CARTESIAN_POINT('Ctrl Pts',(-2.79488053362013,-1.27868880216856,
97.7767426743686));
#23134=CARTESIAN_POINT('Ctrl Pts',(-2.83455113660563,-1.19197920101063,
97.7718229645433));
#23135=CARTESIAN_POINT('Ctrl Pts',(-2.87018271202133,-1.10342145149765,
97.766903254718));
#23136=CARTESIAN_POINT('Ctrl Pts',(-2.90161208415863,-1.01343453812498,
97.7619835448928));
#23137=CARTESIAN_POINT('Ctrl Pts',(-2.93306694789383,-0.923374638559616,
97.7570598448107));
#23138=CARTESIAN_POINT('Ctrl Pts',(-2.9603126535254,-0.831883687086739,
97.7521361447287));
#23139=CARTESIAN_POINT('Ctrl Pts',(-2.98323552026053,-0.739397106199298,
97.7472124446467));
#23140=CARTESIAN_POINT('Ctrl Pts',(-3.00616832327337,-0.646870435546328,
97.7422866103093));
#23141=CARTESIAN_POINT('Ctrl Pts',(-3.024774468657,-0.55334771875868,97.7373607759719));
#23142=CARTESIAN_POINT('Ctrl Pts',(-3.03899158497072,-0.459273770726299,
97.7324349416345));
#23143=CARTESIAN_POINT('Ctrl Pts',(-3.05322924500887,-0.365063885896224,
97.7275019894695));
#23144=CARTESIAN_POINT('Ctrl Pts',(-3.06306516685465,-0.270301628072282,
97.7225690373045));
#23145=CARTESIAN_POINT('Ctrl Pts',(-3.06848896336662,-0.175435833561094,
97.7176360851395));
#23146=CARTESIAN_POINT('Ctrl Pts',(-3.0718654048822,-0.116379634404259,
97.7145652058306));
#23147=CARTESIAN_POINT('Ctrl Pts',(-3.0735330294058,-0.0572833264886464,
97.7114943265216));
#23148=CARTESIAN_POINT('Ctrl Pts',(-3.07349950430575,0.00174557505997277,
97.7084234472127));
#23149=CARTESIAN_POINT('Ctrl Pts',(-3.07349950430537,0.00174557573727362,
97.7084234471775));
#23150=CARTESIAN_POINT('Ctrl Pts',(-3.07344072655593,0.105237724430831,
97.7030394422287));
#23151=CARTESIAN_POINT('Ctrl Pts',(-3.06815507510877,0.208578390863187,
97.6976554372799));
#23152=CARTESIAN_POINT('Ctrl Pts',(-3.05768593427089,0.311382365207073,
97.692271432331));
#23153=CARTESIAN_POINT('Ctrl Pts',(-3.04796444388583,0.406844625540194,
97.6872719244293));
#23154=CARTESIAN_POINT('Ctrl Pts',(-3.03375103466145,0.502018859025492,
97.6822724165276));
#23155=CARTESIAN_POINT('Ctrl Pts',(-3.01507060365512,0.596449079951323,
97.6772729086259));
#23156=CARTESIAN_POINT('Ctrl Pts',(-2.99641551254137,0.690751206848963,
97.6722801825266));
#23157=CARTESIAN_POINT('Ctrl Pts',(-2.97330552693452,0.784310900067703,
97.6672874564274));
#23158=CARTESIAN_POINT('Ctrl Pts',(-2.94581732589708,0.87667698295587,97.6622947303281));
#23159=CARTESIAN_POINT('Ctrl Pts',(-2.91835812421426,0.968945621970214,
97.6573072714282));
#23160=CARTESIAN_POINT('Ctrl Pts',(-2.88653001374994,1.06002273543477,97.6523198125283));
#23161=CARTESIAN_POINT('Ctrl Pts',(-2.85046056698401,1.14946805352267,97.6473323536284));
#23162=CARTESIAN_POINT('Ctrl Pts',(-2.8144169286848,1.23884937155729,97.6423484633629));
#23163=CARTESIAN_POINT('Ctrl Pts',(-2.77413815075664,1.32660080937809,97.6373645730973));
#23164=CARTESIAN_POINT('Ctrl Pts',(-2.72980110282041,1.41229890215933,97.6323806828318));
#23165=CARTESIAN_POINT('Ctrl Pts',(-2.68548020128289,1.49796578592604,97.6273986075694));
#23166=CARTESIAN_POINT('Ctrl Pts',(-2.63710416769728,1.58158042092399,97.6224165323069));
#23167=CARTESIAN_POINT('Ctrl Pts',(-2.58489689381886,1.66274180146094,97.6174344570445));
#23168=CARTESIAN_POINT('Ctrl Pts',(-2.53269437995089,1.74389578208999,97.6124528360239));
#23169=CARTESIAN_POINT('Ctrl Pts',(-2.47666155792127,1.82259658388718,97.6074712150034));
#23170=CARTESIAN_POINT('Ctrl Pts',(-2.4170663519432,1.89847109546181,97.6024895939828));
#23171=CARTESIAN_POINT('Ctrl Pts',(-2.35746031037621,1.97435940252559,97.5975070672049));
#23172=CARTESIAN_POINT('Ctrl Pts',(-2.29429086967186,2.04742005362503,97.5925245404269));
#23173=CARTESIAN_POINT('Ctrl Pts',(-2.22786635543717,2.11731286122554,97.587542013649));
#23174=CARTESIAN_POINT('Ctrl Pts',(-2.16137024500247,2.18728100335412,97.5825541164142));
#23175=CARTESIAN_POINT('Ctrl Pts',(-2.09161235952636,2.25407416656305,97.5775662191795));
#23176=CARTESIAN_POINT('Ctrl Pts',(-2.0189378630642,2.31738908150655,97.5725783219447));
#23177=CARTESIAN_POINT('Ctrl Pts',(-1.94622043658912,2.38074139760518,97.5675874782776));
#23178=CARTESIAN_POINT('Ctrl Pts',(-1.87058331260046,2.44061110196734,97.5625966346104));
#23179=CARTESIAN_POINT('Ctrl Pts',(-1.79240301819493,2.49673660412261,97.5576057909433));
#23180=CARTESIAN_POINT('Ctrl Pts',(-1.71409638188708,2.55295280691754,97.5526068819102));
#23181=CARTESIAN_POINT('Ctrl Pts',(-1.63323873670845,2.60541248673435,97.5476079728771));
#23182=CARTESIAN_POINT('Ctrl Pts',(-1.55023366048267,2.65389861296668,97.542609063844));
#23183=CARTESIAN_POINT('Ctrl Pts',(-1.5020440152854,2.68204784583735,97.5397068840783));
#23184=CARTESIAN_POINT('Ctrl Pts',(-1.45313101222759,2.70885865259285,97.5368047043125));
#23185=CARTESIAN_POINT('Ctrl Pts',(-1.4035767066912,2.73429601148703,97.5339025245467));
#23186=CARTESIAN_POINT('Ctrl Pts',(-1.31821078268786,2.77811629355338,97.5289030143196));
#23187=CARTESIAN_POINT('Ctrl Pts',(-1.23064081993939,2.81801196854969,97.5239035040924));
#23188=CARTESIAN_POINT('Ctrl Pts',(-1.14126285133205,2.85375565775513,97.5189039938653));
#23189=CARTESIAN_POINT('Ctrl Pts',(-1.052006123578,2.88945086079059,97.5139112654536));
#23190=CARTESIAN_POINT('Ctrl Pts',(-0.960946668342703,2.92100510996173,
97.5089185370419));
#23191=CARTESIAN_POINT('Ctrl Pts',(-0.868504677489902,2.94823707920143,
97.5039258086301));
#23192=CARTESIAN_POINT('Ctrl Pts',(-0.776160210839561,2.97544031933158,
97.4989383474336));
#23193=CARTESIAN_POINT('Ctrl Pts',(-0.682436526901436,2.9983302209688,97.4939508862371));
#23194=CARTESIAN_POINT('Ctrl Pts',(-0.587772377970094,3.01677408529299,
97.4889634250405));
#23195=CARTESIAN_POINT('Ctrl Pts',(-0.493175963867824,3.03520475251975,
97.483979532511));
#23196=CARTESIAN_POINT('Ctrl Pts',(-0.397640852148199,3.04919562292873,
97.4789956399816));
#23197=CARTESIAN_POINT('Ctrl Pts',(-0.301618539097904,3.05866449727204,
97.4740117474521));
#23198=CARTESIAN_POINT('Ctrl Pts',(-0.205631195263303,3.06812992325947,
97.4690296699467));
#23199=CARTESIAN_POINT('Ctrl Pts',(-0.10915743902516,3.07307658218339,97.4640475924413));
#23200=CARTESIAN_POINT('Ctrl Pts',(-0.012655529398233,3.07347394450899,
97.459065514936));
#23201=CARTESIAN_POINT('Ctrl Pts',(0.0838375811911415,3.07387127060312,
97.4540838916961));
#23202=CARTESIAN_POINT('Ctrl Pts',(0.180358401106432,3.06972012318302,97.4491022684562));
#23203=CARTESIAN_POINT('Ctrl Pts',(0.276448095310002,3.06104209389539,97.4441206452164));
#23204=CARTESIAN_POINT('Ctrl Pts',(0.37255526000993,3.0523624868165,97.4391381162453));
#23205=CARTESIAN_POINT('Ctrl Pts',(0.468230706150381,3.03915440280407,97.4341555872743));
#23206=CARTESIAN_POINT('Ctrl Pts',(0.563021218355264,3.02149124732834,97.4291730583032));
#23207=CARTESIAN_POINT('Ctrl Pts',(0.657913900226234,3.00380905367405,97.4241851589285));
#23208=CARTESIAN_POINT('Ctrl Pts',(0.751919311691618,2.98166228258095,97.4191972595537));
#23209=CARTESIAN_POINT('Ctrl Pts',(0.844595147304252,2.95517533949343,97.4142093601789));
#23210=CARTESIAN_POINT('Ctrl Pts',(0.937325727527124,2.9286727502845,97.4092185143984));
#23211=CARTESIAN_POINT('Ctrl Pts',(1.02872475232966,2.89782502447123,97.404227668618));
#23212=CARTESIAN_POINT('Ctrl Pts',(1.11836780050234,2.86280556671241,97.3992368228375));
#23213=CARTESIAN_POINT('Ctrl Pts',(1.20815571357048,2.82772951683417,97.394237911754));
#23214=CARTESIAN_POINT('Ctrl Pts',(1.29618158314048,2.78846845221175,97.3892390006705));
#23215=CARTESIAN_POINT('Ctrl Pts',(1.38204363664166,2.74524272814232,97.384240089587));
#23216=CARTESIAN_POINT('Ctrl Pts',(1.43189153504418,2.72014769006757,97.3813379319789));
#23217=CARTESIAN_POINT('Ctrl Pts',(1.48101061626524,2.69371721716037,97.3784357743708));
#23218=CARTESIAN_POINT('Ctrl Pts',(1.52932683084278,2.66600106797885,97.3755336167627));
#23219=CARTESIAN_POINT('Ctrl Pts',(1.61255620384157,2.61825730869455,97.37053436837));
#23220=CARTESIAN_POINT('Ctrl Pts',(1.69369385600289,2.56652847870588,97.3655351199774));
#23221=CARTESIAN_POINT('Ctrl Pts',(1.77233350698893,2.51102293697296,97.3605358715848));
#23222=CARTESIAN_POINT('Ctrl Pts',(1.80615512289055,2.48715091962086,97.3583857773662));
#23223=CARTESIAN_POINT('Ctrl Pts',(1.83951493944344,2.46258091771763,97.3562356831477));
#23224=CARTESIAN_POINT('Ctrl Pts',(1.87238193903531,2.43733217358127,97.3540855889292));
#23225=CARTESIAN_POINT('',(-3.07349919776137,-0.00222066661297698,97.7915765528574));
#23226=CARTESIAN_POINT('Ctrl Pts',(-3.07349919776186,-0.00222066593792731,
97.7915765528225));
#23227=CARTESIAN_POINT('Ctrl Pts',(-3.07356904943382,0.0944571161890471,
97.7865867807264));
#23228=CARTESIAN_POINT('Ctrl Pts',(-3.06907304335083,0.191177787731082,
97.7815970086303));
#23229=CARTESIAN_POINT('Ctrl Pts',(-3.06002570027429,0.287480370914012,
97.7766072365341));
#23230=CARTESIAN_POINT('Ctrl Pts',(-3.05097913287416,0.383774697568821,
97.7716178922375));
#23231=CARTESIAN_POINT('Ctrl Pts',(-3.03738204494624,0.479650572509984,
97.7666285479408));
#23232=CARTESIAN_POINT('Ctrl Pts',(-3.01930089212336,0.574651522945046,
97.7616392036442));
#23233=CARTESIAN_POINT('Ctrl Pts',(-3.00121642371484,0.669669893938976,
97.7566489444391));
#23234=CARTESIAN_POINT('Ctrl Pts',(-2.97864633831454,0.76381259281622,97.7516586852341));
#23235=CARTESIAN_POINT('Ctrl Pts',(-2.95170812541139,0.856633756269486,
97.746668426029));
#23236=CARTESIAN_POINT('Ctrl Pts',(-2.9247387155029,0.949562415433147,97.7416723876305));
#23237=CARTESIAN_POINT('Ctrl Pts',(-2.89339119687211,1.04116606243066,97.7366763492321));
#23238=CARTESIAN_POINT('Ctrl Pts',(-2.85783282778683,1.13101449081077,97.7316803108336));
#23239=CARTESIAN_POINT('Ctrl Pts',(-2.82225376596991,1.22091520531829,97.7266813650554));
#23240=CARTESIAN_POINT('Ctrl Pts',(-2.78245915294648,1.3090582689151,97.7216824192772));
#23241=CARTESIAN_POINT('Ctrl Pts',(-2.73866333821666,1.39503597441355,97.7166834734989));
#23242=CARTESIAN_POINT('Ctrl Pts',(-2.69478773475782,1.48117031706761,97.7116754204685));
#23243=CARTESIAN_POINT('Ctrl Pts',(-2.64689658149737,1.56513103983351,97.7066673674381));
#23244=CARTESIAN_POINT('Ctrl Pts',(-2.5952490191003,1.64653720846476,97.7016593144077));
#23245=CARTESIAN_POINT('Ctrl Pts',(-2.54830188139988,1.72053463314501,97.6971070423484));
#23246=CARTESIAN_POINT('Ctrl Pts',(-2.49825164975594,1.79242150070637,97.6925547702891));
#23247=CARTESIAN_POINT('Ctrl Pts',(-2.44532132719365,1.86193605066658,97.6880024982298));
#23248=CARTESIAN_POINT('Ctrl Pts',(-2.38719087098629,1.93828004984554,97.6830029887091));
#23249=CARTESIAN_POINT('Ctrl Pts',(-2.32537964657829,2.01203324522605,97.6780034791883));
#23250=CARTESIAN_POINT('Ctrl Pts',(-2.2601469502219,2.08281972657325,97.6730039696676));
#23251=CARTESIAN_POINT('Ctrl Pts',(-2.19500274162626,2.15351018648371,97.6680112419515));
#23252=CARTESIAN_POINT('Ctrl Pts',(-2.12644658009942,2.2212416104132,97.6630185142354));
#23253=CARTESIAN_POINT('Ctrl Pts',(-2.05477941583094,2.28566922416115,97.6580257865192));
#23254=CARTESIAN_POINT('Ctrl Pts',(-1.98318785863915,2.35002886837825,97.6530383260068));
#23255=CARTESIAN_POINT('Ctrl Pts',(-1.90849214789139,2.41109133934675,97.6480508654943));
#23256=CARTESIAN_POINT('Ctrl Pts',(-1.83103094631659,2.46854773574079,97.6430634049818));
#23257=CARTESIAN_POINT('Ctrl Pts',(-1.75362517008367,2.52596302070938,97.6380795131166));
#23258=CARTESIAN_POINT('Ctrl Pts',(-1.67345818828568,2.57977709972297,97.6330956212513));
#23259=CARTESIAN_POINT('Ctrl Pts',(-1.59090193540887,2.62972114147343,97.6281117293861));
#23260=CARTESIAN_POINT('Ctrl Pts',(-1.50837574750221,2.6796469948242,97.6231296525325));
#23261=CARTESIAN_POINT('Ctrl Pts',(-1.42346239253632,2.72570538419995,97.6181475756789));
#23262=CARTESIAN_POINT('Ctrl Pts',(-1.3365621845007,2.76767118295558,97.6131654988253));
#23263=CARTESIAN_POINT('Ctrl Pts',(-1.24966989979133,2.80963315538302,97.608183876224));
#23264=CARTESIAN_POINT('Ctrl Pts',(-1.16079151754669,2.84750308835942,97.6032022536227));
#23265=CARTESIAN_POINT('Ctrl Pts',(-1.07035034378284,2.88110263468068,97.5982206310214));
#23266=CARTESIAN_POINT('Ctrl Pts',(-0.979892726250969,2.91470828997999,
97.5932381026751));
#23267=CARTESIAN_POINT('Ctrl Pts',(-0.887872164384384,2.94404186379848,
97.5882555743288));
#23268=CARTESIAN_POINT('Ctrl Pts',(-0.794729233475481,2.96897418234977,
97.5832730459824));
#23269=CARTESIAN_POINT('Ctrl Pts',(-0.701485908264306,2.99393337425259,
97.5782851472075));
#23270=CARTESIAN_POINT('Ctrl Pts',(-0.607118223597923,3.01448172643295,
97.5732972484326));
#23271=CARTESIAN_POINT('Ctrl Pts',(-0.512078899859159,3.03054078512714,
97.5683093496577));
#23272=CARTESIAN_POINT('Ctrl Pts',(-0.416983435115779,3.04660933012293,
97.563318504464));
#23273=CARTESIAN_POINT('Ctrl Pts',(-0.321215976901245,3.05818324865149,
97.5583276592703));
#23274=CARTESIAN_POINT('Ctrl Pts',(-0.225234235281423,3.06523600873688,
97.5533368140766));
#23275=CARTESIAN_POINT('Ctrl Pts',(-0.129097384790456,3.07230016625721,
97.5483379035535));
#23276=CARTESIAN_POINT('Ctrl Pts',(-0.0327459979506133,3.07482856475272,
97.5433389930304));
#23277=CARTESIAN_POINT('Ctrl Pts',(0.063362407555235,3.07284679984356,97.5383400825073));
#23278=CARTESIAN_POINT('Ctrl Pts',(0.119159036688698,3.07169626778464,97.5354379184868));
#23279=CARTESIAN_POINT('Ctrl Pts',(0.174873848989266,3.06902656260381,97.5325357544663));
#23280=CARTESIAN_POINT('Ctrl Pts',(0.230418577026407,3.06485065367974,97.5296335904458));
#23281=CARTESIAN_POINT('Ctrl Pts',(0.326094831378455,3.0576576159516,97.5246345888697));
#23282=CARTESIAN_POINT('Ctrl Pts',(0.421601973471025,3.04596752585046,97.5196355872936));
#23283=CARTESIAN_POINT('Ctrl Pts',(0.516483657699913,3.02979320768413,97.5146365857176));
#23284=CARTESIAN_POINT('Ctrl Pts',(0.611243167896439,3.0136397163158,97.5096440210865));
#23285=CARTESIAN_POINT('Ctrl Pts',(0.70537839149724,2.99301354198044,97.5046514564554));
#23286=CARTESIAN_POINT('Ctrl Pts',(0.798436325656736,2.96797939411172,97.4996588918244));
#23287=CARTESIAN_POINT('Ctrl Pts',(0.895202885872508,2.94194756352071,97.4944673591478));
#23288=CARTESIAN_POINT('Ctrl Pts',(0.990804017801527,2.911149102255,97.4892758264712));
#23289=CARTESIAN_POINT('Ctrl Pts',(1.08473981285586,2.87571587407474,97.4840842937946));
#23290=CARTESIAN_POINT('Ctrl Pts',(1.17491270328855,2.84170203940684,97.4791007248904));
#23291=CARTESIAN_POINT('Ctrl Pts',(1.2635506597892,2.80341779712293,97.4741171559862));
#23292=CARTESIAN_POINT('Ctrl Pts',(1.35022649850534,2.76103072288847,97.469133587082));
#23293=CARTESIAN_POINT('Ctrl Pts',(1.43686593133514,2.71866145221991,97.4641521113937));
#23294=CARTESIAN_POINT('Ctrl Pts',(1.52154449194907,2.67219297011668,97.4591706357054));
#23295=CARTESIAN_POINT('Ctrl Pts',(1.60385651248083,2.62184029593201,97.4541891600171));
#23296=CARTESIAN_POINT('Ctrl Pts',(1.68616392127089,2.57149044288482,97.4492079634288));
#23297=CARTESIAN_POINT('Ctrl Pts',(1.76610467867593,2.51725705834576,97.4442267668404));
#23298=CARTESIAN_POINT('Ctrl Pts',(1.84330001440335,2.45939978590318,97.439245570252));
#23299=CARTESIAN_POINT('Ctrl Pts',(1.85303787899999,2.4521013360724,97.4386172134031));
#23300=CARTESIAN_POINT('Ctrl Pts',(1.86273209567925,2.44474527574693,97.4379888565543));
#23301=CARTESIAN_POINT('Ctrl Pts',(1.8723819390353,2.43733217358127,97.4373604997054));
#23302=CARTESIAN_POINT('Ctrl Pts',(1.8723819390353,2.43733217358127,98.4372333997809));
#23303=CARTESIAN_POINT('Ctrl Pts',(1.94879667949973,2.3786296374754,98.4322491033839));
#23304=CARTESIAN_POINT('Ctrl Pts',(2.02250938947208,2.31628298897807,98.427264806987));
#23305=CARTESIAN_POINT('Ctrl Pts',(2.09315882163261,2.25057512592262,98.42228051059));
#23306=CARTESIAN_POINT('Ctrl Pts',(2.16377952620586,2.18489398110555,98.4172982409158));
#23307=CARTESIAN_POINT('Ctrl Pts',(2.23133910669081,2.11585463573883,98.4123159712416));
#23308=CARTESIAN_POINT('Ctrl Pts',(2.29551041638283,2.04377938591178,98.4073337015674));
#23309=CARTESIAN_POINT('Ctrl Pts',(2.35967315132447,1.97171376698176,98.402352097638));
#23310=CARTESIAN_POINT('Ctrl Pts',(2.42044822365573,1.89661337785966,98.3973704937086));
#23311=CARTESIAN_POINT('Ctrl Pts',(2.47754703950436,1.8188355937366,98.3923888897792));
#23312=CARTESIAN_POINT('Ctrl Pts',(2.53465381334927,1.74104696954082,98.387406591552));
#23313=CARTESIAN_POINT('Ctrl Pts',(2.58808305355812,1.66058056326875,98.3824242933247));
#23314=CARTESIAN_POINT('Ctrl Pts',(2.63758861081898,1.57782399844787,98.3774419950975));
#23315=CARTESIAN_POINT('Ctrl Pts',(2.68714635867861,1.49498018857999,98.3724544443463));
#23316=CARTESIAN_POINT('Ctrl Pts',(2.73277193785748,1.40984177645768,98.3674668935951));
#23317=CARTESIAN_POINT('Ctrl Pts',(2.77426454507443,1.32282216640899,98.3624793428438));
#23318=CARTESIAN_POINT('Ctrl Pts',(2.81578008312558,1.23575446508853,98.3574890357293));
#23319=CARTESIAN_POINT('Ctrl Pts',(2.8531579303546,1.14680390010304,98.3524987286148));
#23320=CARTESIAN_POINT('Ctrl Pts',(2.88624578645053,1.05640310023995,98.3475084215002));
#23321=CARTESIAN_POINT('Ctrl Pts',(2.91938864408817,0.965852028224121,98.3425098190587));
#23322=CARTESIAN_POINT('Ctrl Pts',(2.94822713534302,0.873846325235199,98.3375112166172));
#23323=CARTESIAN_POINT('Ctrl Pts',(2.97265908194401,0.780833037553993,98.3325126141758));
#23324=CARTESIAN_POINT('Ctrl Pts',(2.99063703656771,0.712390326351174,98.3288344525727));
#23325=CARTESIAN_POINT('Ctrl Pts',(3.00623009381549,0.643402335271145,98.3251562909697));
#23326=CARTESIAN_POINT('Ctrl Pts',(3.01941544185753,0.574049335399231,98.3214781293667));
#23327=CARTESIAN_POINT('Ctrl Pts',(3.03733751258853,0.479781867817168,98.316478619896));
#23328=CARTESIAN_POINT('Ctrl Pts',(3.05087222367182,0.38450871946811,98.3114791104254));
#23329=CARTESIAN_POINT('Ctrl Pts',(3.05991332529291,0.28867402324231,98.3064796009548));
#23330=CARTESIAN_POINT('Ctrl Pts',(3.06894216271708,0.192969326173176,98.301486873287));
#23331=CARTESIAN_POINT('Ctrl Pts',(3.07348946431034,0.0967050284110289,
98.2964941456192));
#23332=CARTESIAN_POINT('Ctrl Pts',(3.07349998169631,0.000335429283253844,
98.2915014179515));
#23333=CARTESIAN_POINT('Ctrl Pts',(3.07351048798669,-0.095932502347352,
98.2865139574855));
#23334=CARTESIAN_POINT('Ctrl Pts',(3.06899372468457,-0.192305077874619,
98.2815264970195));
#23335=CARTESIAN_POINT('Ctrl Pts',(3.05994633315224,-0.288323929336723,
98.2765390365535));
#23336=CARTESIAN_POINT('Ctrl Pts',(3.05090541523968,-0.384274077069903,
98.2715551447319));
#23337=CARTESIAN_POINT('Ctrl Pts',(3.03734035464377,-0.479870568110944,
98.2665712529103));
#23338=CARTESIAN_POINT('Ctrl Pts',(3.01929983554887,-0.574657074310022,
98.2615873610886));
#23339=CARTESIAN_POINT('Ctrl Pts',(3.00126588636379,-0.669409061613417,
98.2566052842769));
#23340=CARTESIAN_POINT('Ctrl Pts',(2.97875979900632,-0.763351219380252,
98.2516232074651));
#23341=CARTESIAN_POINT('Ctrl Pts',(2.95188173341891,-0.856035327488177,
98.2466411306533));
#23342=CARTESIAN_POINT('Ctrl Pts',(2.92500611849093,-0.948710984943907,
98.241659508092));
#23343=CARTESIAN_POINT('Ctrl Pts',(2.89375944030682,-1.04012839925424,98.2366778855306));
#23344=CARTESIAN_POINT('Ctrl Pts',(2.85829202006636,-1.12985352060564,98.2316962629693));
#23345=CARTESIAN_POINT('Ctrl Pts',(2.82281815122272,-1.21959495556821,98.226713734661));
#23346=CARTESIAN_POINT('Ctrl Pts',(2.78312217765326,-1.30764307829281,98.2217312063528));
#23347=CARTESIAN_POINT('Ctrl Pts',(2.73940253685439,-1.39358386582068,98.2167486780445));
#23348=CARTESIAN_POINT('Ctrl Pts',(2.69563577272231,-1.47961728485911,98.2117607793047));
#23349=CARTESIAN_POINT('Ctrl Pts',(2.64783688246335,-1.56353844217188,98.2067728805648));
#23350=CARTESIAN_POINT('Ctrl Pts',(2.59625014480326,-1.64495818658379,98.2017849818249));
#23351=CARTESIAN_POINT('Ctrl Pts',(2.54463293414702,-1.72642602675967,98.1967941366645));
#23352=CARTESIAN_POINT('Ctrl Pts',(2.48922367281748,-1.80538915269852,98.1918032915042));
#23353=CARTESIAN_POINT('Ctrl Pts',(2.43030859142751,-1.88148941013061,98.1868124463438));
#23354=CARTESIAN_POINT('Ctrl Pts',(2.37129830177163,-1.95771264750899,98.1818135358511));
#23355=CARTESIAN_POINT('Ctrl Pts',(2.30877116388989,-2.0310634445112,98.1768146253584));
#23356=CARTESIAN_POINT('Ctrl Pts',(2.24305204931632,-2.10121863547273,98.1718157148657));
#23357=CARTESIAN_POINT('Ctrl Pts',(2.20489820022924,-2.14194789036287,98.1689135504379));
#23358=CARTESIAN_POINT('Ctrl Pts',(2.16566916856287,-2.18160077883473,98.1660113860102));
#23359=CARTESIAN_POINT('Ctrl Pts',(2.12543360399782,-2.22012032218906,98.1631092215824));
#23360=CARTESIAN_POINT('Ctrl Pts',(2.05612047864035,-2.28647728688168,98.1581097120947));
#23361=CARTESIAN_POINT('Ctrl Pts',(1.98357509118963,-2.34970171259639,98.1531102026069));
#23362=CARTESIAN_POINT('Ctrl Pts',(1.90811212901156,-2.40946266896148,98.1481106931191));
#23363=CARTESIAN_POINT('Ctrl Pts',(1.83275153186626,-2.46914255996576,98.1431179654345));
#23364=CARTESIAN_POINT('Ctrl Pts',(1.75448156678403,-2.52536804874238,98.1381252377498));
#23365=CARTESIAN_POINT('Ctrl Pts',(1.67365321647241,-2.57784544939986,98.1331325100651));
#23366=CARTESIAN_POINT('Ctrl Pts',(1.59291013803702,-2.63026748771978,98.1281450495826));
#23367=CARTESIAN_POINT('Ctrl Pts',(1.50961440609933,-2.67894906074651,98.1231575891001));
#23368=CARTESIAN_POINT('Ctrl Pts',(1.42414866755533,-2.72363779212662,98.1181701286175));
#23369=CARTESIAN_POINT('Ctrl Pts',(1.33874408175006,-2.7682945476722,98.1131862367798));
#23370=CARTESIAN_POINT('Ctrl Pts',(1.25117296389306,-2.80896393827999,98.1082023449421));
#23371=CARTESIAN_POINT('Ctrl Pts',(1.16184458469751,-2.84543835129301,98.1032184531044));
#23372=CARTESIAN_POINT('Ctrl Pts',(1.0725487366886,-2.88189948122681,98.0982363762769));
#23373=CARTESIAN_POINT('Ctrl Pts',(0.981497304829406,-2.91416850318698,
98.0932542994494));
#23374=CARTESIAN_POINT('Ctrl Pts',(0.889120784939191,-2.94208539641342,
98.0882722226218));
#23375=CARTESIAN_POINT('Ctrl Pts',(0.796752687662835,-2.96999974426132,
98.0832906000451));
#23376=CARTESIAN_POINT('Ctrl Pts',(0.703060162809543,-2.99356262550506,
98.0783089774684));
#23377=CARTESIAN_POINT('Ctrl Pts',(0.608489130627945,-3.01266380930691,
98.0733273548917));
#23378=CARTESIAN_POINT('Ctrl Pts',(0.513900903769525,-3.03176846603991,
98.0683448265683));
#23379=CARTESIAN_POINT('Ctrl Pts',(0.418434282638778,-3.04640972738691,
98.063362298245));
#23380=CARTESIAN_POINT('Ctrl Pts',(0.322544586106083,-3.05652862574092,
98.0583797699217));
#23381=CARTESIAN_POINT('Ctrl Pts',(0.226551534616821,-3.06665843077559,
98.0533918711674));
#23382=CARTESIAN_POINT('Ctrl Pts',(0.13013493460024,-3.07225609530408,98.0484039724131));
#23383=CARTESIAN_POINT('Ctrl Pts',(0.0337542009956394,-3.07331464447023,
98.0434160736588));
#23384=CARTESIAN_POINT('Ctrl Pts',(-0.0626834660288813,-3.07437381893586,
98.0384252284843));
#23385=CARTESIAN_POINT('Ctrl Pts',(-0.159084785984224,-3.07088855494982,
98.0334343833099));
#23386=CARTESIAN_POINT('Ctrl Pts',(-0.254993503125497,-3.06290394288881,
98.0284435381354));
#23387=CARTESIAN_POINT('Ctrl Pts',(-0.351057211173044,-3.05490642749328,
98.0234446276293));
#23388=CARTESIAN_POINT('Ctrl Pts',(-0.446626291898313,-3.0423951022646,
98.0184457171231));
#23389=CARTESIAN_POINT('Ctrl Pts',(-0.54125279961846,-3.02546651888683,
98.013446806617));
#23390=CARTESIAN_POINT('Ctrl Pts',(-0.596189104167083,-3.01563847139332,
98.0105446423441));
#23391=CARTESIAN_POINT('Ctrl Pts',(-0.650807945735842,-3.00432253982776,
98.0076424780711));
#23392=CARTESIAN_POINT('Ctrl Pts',(-0.705024154619203,-2.99154528486591,
98.0047403137982));
#23393=CARTESIAN_POINT('Ctrl Pts',(-0.798421505988598,-2.96953412259938,
97.9997408042067));
#23394=CARTESIAN_POINT('Ctrl Pts',(-0.89095111788327,-2.94310624791073,
97.9947412946151));
#23395=CARTESIAN_POINT('Ctrl Pts',(-0.982164076418903,-2.912345442593,97.9897417850236));
#23396=CARTESIAN_POINT('Ctrl Pts',(-1.07325330516414,-2.88162636410943,
97.9847490572345));
#23397=CARTESIAN_POINT('Ctrl Pts',(-1.16302901778237,-2.84658617539717,
97.9797563294455));
#23398=CARTESIAN_POINT('Ctrl Pts',(-1.2510537797181,-2.80735938031686,97.9747636016565));
#23399=CARTESIAN_POINT('Ctrl Pts',(-1.33898567775394,-2.76817396851429,
97.9697761410692));
#23400=CARTESIAN_POINT('Ctrl Pts',(-1.42516989842704,-2.72481090833102,
97.9647886804818));
#23401=CARTESIAN_POINT('Ctrl Pts',(-1.50918641768823,-2.67745375434673,
97.9598012198945));
#23402=CARTESIAN_POINT('Ctrl Pts',(-1.59314282116564,-2.63013048551328,
97.9548173279518));
#23403=CARTESIAN_POINT('Ctrl Pts',(-1.67493422532557,-2.57881901911081,
97.9498334360091));
#23404=CARTESIAN_POINT('Ctrl Pts',(-1.75416365818427,-2.52374961323535,
97.9448495440664));
#23405=CARTESIAN_POINT('Ctrl Pts',(-1.83336423764461,-2.46870026227444,
97.9398674671338));
#23406=CARTESIAN_POINT('Ctrl Pts',(-1.9100043395087,-2.40989594127437,97.9348853902012));
#23407=CARTESIAN_POINT('Ctrl Pts',(-1.98371535546732,-2.34761062326851,
97.9299033132686));
#23408=CARTESIAN_POINT('Ctrl Pts',(-2.05741965067641,-2.28533098425129,
97.9249216905869));
#23409=CARTESIAN_POINT('Ctrl Pts',(-2.12819505578402,-2.21957126270958,
97.9199400679051));
#23410=CARTESIAN_POINT('Ctrl Pts',(-2.19570632802947,-2.15064547776972,
97.9149584452233));
#23411=CARTESIAN_POINT('Ctrl Pts',(-2.26322987500894,-2.0817071609126,97.9099759167951));
#23412=CARTESIAN_POINT('Ctrl Pts',(-2.32748780335053,-2.00960195103968,
97.904993388367));
#23413=CARTESIAN_POINT('Ctrl Pts',(-2.38818275240191,-1.93467966111448,
97.9000108599388));
#23414=CARTESIAN_POINT('Ctrl Pts',(-2.44894312164816,-1.85967661602127,
97.8950229610805));
#23415=CARTESIAN_POINT('Ctrl Pts',(-2.50613256789654,-1.78185077064053,
97.8900350622222));
#23416=CARTESIAN_POINT('Ctrl Pts',(-2.55949511150196,-1.70158368122098,
97.885047163364));
#23417=CARTESIAN_POINT('Ctrl Pts',(-2.6128891770883,-1.62126917693907,97.8800563180859));
#23418=CARTESIAN_POINT('Ctrl Pts',(-2.66245161337136,-1.53851093362595,
97.8750654728079));
#23419=CARTESIAN_POINT('Ctrl Pts',(-2.70797183264986,-1.45371620462007,
97.8700746275299));
#23420=CARTESIAN_POINT('Ctrl Pts',(-2.75356561373528,-1.36878444522237,
97.8650757169217));
#23421=CARTESIAN_POINT('Ctrl Pts',(-2.79510394516053,-1.28181002454817,
97.8600768063135));
#23422=CARTESIAN_POINT('Ctrl Pts',(-2.83242392899805,-1.19322124370934,
97.8550778957054));
#23423=CARTESIAN_POINT('Ctrl Pts',(-2.85409038662106,-1.14179021752574,
97.8521757324749));
#23424=CARTESIAN_POINT('Ctrl Pts',(-2.87433597636449,-1.08981539643607,
97.8492735692445));
#23425=CARTESIAN_POINT('Ctrl Pts',(-2.89313660636368,-1.03738268103842,
97.8463714060141));
#23426=CARTESIAN_POINT('Ctrl Pts',(-2.93067890649147,-0.932681682292151,
97.8405761809062));
#23427=CARTESIAN_POINT('Ctrl Pts',(-2.96256548532845,-0.825852277625856,
97.8347809557982));
#23428=CARTESIAN_POINT('Ctrl Pts',(-2.98858506992045,-0.717468835454609,
97.8289857306903));
#23429=CARTESIAN_POINT('Ctrl Pts',(-3.01448640612548,-0.609577951770032,
97.823216842514));
#23430=CARTESIAN_POINT('Ctrl Pts',(-3.03457384715709,-0.500147256877293,
97.8174479543377));
#23431=CARTESIAN_POINT('Ctrl Pts',(-3.04868590390206,-0.389764684584056,
97.8116790661614));
#23432=CARTESIAN_POINT('Ctrl Pts',(-3.062686713896,-0.280252269119051,97.8059556547061));
#23433=CARTESIAN_POINT('Ctrl Pts',(-3.07080588040819,-0.169803074558109,
97.8002322432507));
#23434=CARTESIAN_POINT('Ctrl Pts',(-3.07293345960593,-0.0590101926311166,
97.7945088317954));
#23435=CARTESIAN_POINT('Ctrl Pts',(-3.07329680092891,-0.0400893306770456,
97.7935314054827));
#23436=CARTESIAN_POINT('Ctrl Pts',(-3.07348551479518,-0.0211584870746742,
97.79255397917));
#23437=CARTESIAN_POINT('Ctrl Pts',(-3.07349919776137,-0.00222066661295415,
97.7915765528574));
#23438=CARTESIAN_POINT('Origin',(0.,0.,116.208423447177));
#23439=CARTESIAN_POINT('',(1.87238193903529,2.43733217358128,99.4373602300224));
#23440=CARTESIAN_POINT('',(1.87238193903531,2.43733217358127,99.3541713863777));
#23441=CARTESIAN_POINT('',(1.8723819390353,2.43733217358128,116.208423447177));
#23442=CARTESIAN_POINT('',(-3.07349970959527,0.00133608300057976,98.7084234471481));
#23443=CARTESIAN_POINT('Ctrl Pts',(1.87238193903531,2.43733217358127,99.3541713863777));
#23444=CARTESIAN_POINT('Ctrl Pts',(1.94890764724692,2.37854439098831,99.3491895972089));
#23445=CARTESIAN_POINT('Ctrl Pts',(2.02266023466669,2.31615050135599,99.3442078080402));
#23446=CARTESIAN_POINT('Ctrl Pts',(2.09329231361966,2.25045096363837,99.3392260188715));
#23447=CARTESIAN_POINT('Ctrl Pts',(2.16394410004746,2.18473309470346,99.3342428397042));
#23448=CARTESIAN_POINT('Ctrl Pts',(2.23147332718422,2.11570804446625,99.329259660537));
#23449=CARTESIAN_POINT('Ctrl Pts',(2.2955691098263,2.04371346132752,99.3242764813697));
#23450=CARTESIAN_POINT('Ctrl Pts',(2.35973727932181,1.97163757079034,99.3192876744272));
#23451=CARTESIAN_POINT('Ctrl Pts',(2.42046397465964,1.89658578347112,99.3142988674847));
#23452=CARTESIAN_POINT('Ctrl Pts',(2.47747849109117,1.81892896402818,99.3093100605422));
#23453=CARTESIAN_POINT('Ctrl Pts',(2.53453165653656,1.74121950256213,99.304317871786));
#23454=CARTESIAN_POINT('Ctrl Pts',(2.58786739174473,1.66090185891364,99.2993256830299));
#23455=CARTESIAN_POINT('Ctrl Pts',(2.63725936478344,1.57837425627196,99.2943334942738));
#23456=CARTESIAN_POINT('Ctrl Pts',(2.68672617834146,1.49572160479625,99.2893337411711));
#23457=CARTESIAN_POINT('Ctrl Pts',(2.73223709994962,1.41085269856006,99.2843339880684));
#23458=CARTESIAN_POINT('Ctrl Pts',(2.77361272540734,1.32418831721869,99.2793342349658));
#23459=CARTESIAN_POINT('Ctrl Pts',(2.78291918318436,1.3046952365268,99.2782096600348));
#23460=CARTESIAN_POINT('Ctrl Pts',(2.79201662624458,1.2851113883725,99.2770850851037));
#23461=CARTESIAN_POINT('Ctrl Pts',(2.80090335865005,1.26544167210617,99.2759605101727));
#23462=CARTESIAN_POINT('Ctrl Pts',(2.84041099999358,1.17799624670995,99.2709610006779));
#23463=CARTESIAN_POINT('Ctrl Pts',(2.87588898208135,1.08854528768625,99.2659614911831));
#23464=CARTESIAN_POINT('Ctrl Pts',(2.90712996357781,0.997495676616248,99.2609619816883));
#23465=CARTESIAN_POINT('Ctrl Pts',(2.93832856688126,0.906569573765421,99.2559692539964));
#23466=CARTESIAN_POINT('Ctrl Pts',(2.96530145105313,0.814049540389896,99.2509765263044));
#23467=CARTESIAN_POINT('Ctrl Pts',(2.9878884751466,0.720364289846532,99.2459837986125));
#23468=CARTESIAN_POINT('Ctrl Pts',(3.01045167049912,0.626777874880536,99.2409963381224));
#23469=CARTESIAN_POINT('Ctrl Pts',(3.02863810157716,0.532029110936636,99.2360088776323));
#23470=CARTESIAN_POINT('Ctrl Pts',(3.04233711995342,0.436562823146337,99.2310214171422));
#23471=CARTESIAN_POINT('Ctrl Pts',(3.05602633636178,0.341164843716829,99.2260375252967));
#23472=CARTESIAN_POINT('Ctrl Pts',(3.06523446091201,0.245050794331692,99.2210536334512));
#23473=CARTESIAN_POINT('Ctrl Pts',(3.06990191756383,0.148675709306916,99.2160697416057));
#23474=CARTESIAN_POINT('Ctrl Pts',(3.07456767444353,0.0523357217012599,
99.2110876647702));
#23475=CARTESIAN_POINT('Ctrl Pts',(3.07469602773365,-0.0442646746643785,
99.2061055879347));
#23476=CARTESIAN_POINT('Ctrl Pts',(3.07027934411709,-0.140666268479421,
99.2011235110992));
#23477=CARTESIAN_POINT('Ctrl Pts',(3.06586306320034,-0.237059072689754,
99.1961418885143));
#23478=CARTESIAN_POINT('Ctrl Pts',(3.05690258955944,-0.333252671893883,
99.1911602659294));
#23479=CARTESIAN_POINT('Ctrl Pts',(3.04344237491033,-0.428789879311707,
99.1861786433445));
#23480=CARTESIAN_POINT('Ctrl Pts',(3.02997971295706,-0.524344457077083,
99.1811961150129));
#23481=CARTESIAN_POINT('Ctrl Pts',(3.01201574645876,-0.619241971379589,
99.1762135866812));
#23482=CARTESIAN_POINT('Ctrl Pts',(2.98964639614413,-0.713033432611991,
99.1712310583496));
#23483=CARTESIAN_POINT('Ctrl Pts',(2.96725293496671,-0.806925987216338,
99.1662431595867));
#23484=CARTESIAN_POINT('Ctrl Pts',(2.94044471232729,-0.899709681014647,
99.1612552608239));
#23485=CARTESIAN_POINT('Ctrl Pts',(2.90936804124939,-0.990948964657948,
99.1562673620611));
#23486=CARTESIAN_POINT('Ctrl Pts',(2.87827301275542,-1.08224214459819,99.151276516878));
#23487=CARTESIAN_POINT('Ctrl Pts',(2.84290467611058,-1.17198868963417,99.1462856716949));
#23488=CARTESIAN_POINT('Ctrl Pts',(2.80345739047923,-1.25977335650798,99.1412948265118));
#23489=CARTESIAN_POINT('Ctrl Pts',(2.76394635703844,-1.34769988561961,99.1362959159969));
#23490=CARTESIAN_POINT('Ctrl Pts',(2.72034341092015,-1.43365781467906,99.131297005482));
#23491=CARTESIAN_POINT('Ctrl Pts',(2.6728886737526,-1.51725686280375,99.1262980949671));
#23492=CARTESIAN_POINT('Ctrl Pts',(2.64533838282884,-1.56579107106736,99.1233959307743));
#23493=CARTESIAN_POINT('Ctrl Pts',(2.61649066732709,-1.61353075371004,99.1204937665814));
#23494=CARTESIAN_POINT('Ctrl Pts',(2.58639891787788,-1.66040443494954,99.1175916023886));
#23495=CARTESIAN_POINT('Ctrl Pts',(2.53456036672751,-1.74115293801154,99.1125920928982));
#23496=CARTESIAN_POINT('Ctrl Pts',(2.47884563517596,-1.81961330989724,99.1075925834077));
#23497=CARTESIAN_POINT('Ctrl Pts',(2.41948312504004,-1.89539010698233,99.1025930739172));
#23498=CARTESIAN_POINT('Ctrl Pts',(2.36020113977226,-1.97106411332323,99.0976003462296));
#23499=CARTESIAN_POINT('Ctrl Pts',(2.29728147850438,-2.04406143702507,99.092607618542));
#23500=CARTESIAN_POINT('Ctrl Pts',(2.2309965537036,-2.11401433944112,99.0876148908544));
#23501=CARTESIAN_POINT('Ctrl Pts',(2.16478155782714,-2.18389344330894,99.0826274303687));
#23502=CARTESIAN_POINT('Ctrl Pts',(2.09520865645798,-2.2507341937906,99.0776399698829));
#23503=CARTESIAN_POINT('Ctrl Pts',(2.02259072277512,-2.31420159410195,99.0726525093971));
#23504=CARTESIAN_POINT('Ctrl Pts',(1.95002474892108,-2.37762358200499,99.0676686175559));
#23505=CARTESIAN_POINT('Ctrl Pts',(1.87441840365887,-2.43767673003947,99.0626847257147));
#23506=CARTESIAN_POINT('Ctrl Pts',(1.7961209299935,-2.49406332213905,99.0577008338735));
#23507=CARTESIAN_POINT('Ctrl Pts',(1.71785197032867,-2.55042937963845,99.0527187570422));
#23508=CARTESIAN_POINT('Ctrl Pts',(1.63689418534052,-2.60313127797436,99.047736680211));
#23509=CARTESIAN_POINT('Ctrl Pts',(1.55362860196168,-2.65191259606469,99.0427546033797));
#23510=CARTESIAN_POINT('Ctrl Pts',(1.47037061048527,-2.70068946642294,99.037772980799));
#23511=CARTESIAN_POINT('Ctrl Pts',(1.38480561781128,-2.74554624551174,99.0327913582184));
#23512=CARTESIAN_POINT('Ctrl Pts',(1.29734131048932,-2.78627130303168,99.0278097356377));
#23513=CARTESIAN_POINT('Ctrl Pts',(1.20986110061474,-2.82700376508485,99.0228272073103));
#23514=CARTESIAN_POINT('Ctrl Pts',(1.12048128821925,-2.86360282839112,99.0178446789829));
#23515=CARTESIAN_POINT('Ctrl Pts',(1.02963070651139,-2.89590449742543,99.0128621506554));
#23516=CARTESIAN_POINT('Ctrl Pts',(0.938682201265032,-2.9282409828987,99.0078742518967));
#23517=CARTESIAN_POINT('Ctrl Pts',(0.846260176139689,-2.95627067952686,
99.002886353138));
#23518=CARTESIAN_POINT('Ctrl Pts',(0.752809626922593,-2.9798791780226,98.9978984543793));
#23519=CARTESIAN_POINT('Ctrl Pts',(0.659303875182713,-3.00350162238262,
98.9929076092003));
#23520=CARTESIAN_POINT('Ctrl Pts',(0.564768819575584,-3.02269758105268,
98.9879167640213));
#23521=CARTESIAN_POINT('Ctrl Pts',(0.46965858209221,-3.03740400116072,98.9829259188423));
#23522=CARTESIAN_POINT('Ctrl Pts',(0.374394644062165,-3.05213418721519,
98.9779270083313));
#23523=CARTESIAN_POINT('Ctrl Pts',(0.278554104323566,-3.06236030112,98.9729280978205));
#23524=CARTESIAN_POINT('Ctrl Pts',(0.182595062064441,-3.06807126600894,
98.9679291873096));
#23525=CARTESIAN_POINT('Ctrl Pts',(0.126885142899932,-3.07138682007059,
98.9650270230745));
#23526=CARTESIAN_POINT('Ctrl Pts',(0.0711352808583605,-3.07318152364689,
98.9621248588395));
#23527=CARTESIAN_POINT('Ctrl Pts',(0.0154344978905465,-3.07346124528598,
98.9592226946044));
#23528=CARTESIAN_POINT('Ctrl Pts',(-0.0805203036166465,-3.0739431170466,
98.9542231851132));
#23529=CARTESIAN_POINT('Ctrl Pts',(-0.176666230816496,-3.06992790199966,
98.949223675622));
#23530=CARTESIAN_POINT('Ctrl Pts',(-0.272547234921952,-3.06139188192828,
98.9442241661308));
#23531=CARTESIAN_POINT('Ctrl Pts',(-0.368298177053213,-3.05286744091402,
98.9392314384426));
#23532=CARTESIAN_POINT('Ctrl Pts',(-0.463784476814253,-3.03983442129326,
98.9342387107543));
#23533=CARTESIAN_POINT('Ctrl Pts',(-0.558549362472165,-3.02232110466144,
98.929245983066));
#23534=CARTESIAN_POINT('Ctrl Pts',(-0.653214273563878,-3.00482626413731,
98.9242585225797));
#23535=CARTESIAN_POINT('Ctrl Pts',(-0.747158854163399,-2.98286060214701,
98.9192710620933));
#23536=CARTESIAN_POINT('Ctrl Pts',(-0.839931767261859,-2.95650416477711,
98.9142836016069));
#23537=CARTESIAN_POINT('Ctrl Pts',(-0.932638299171926,-2.93016658605436,
98.9092997097651));
#23538=CARTESIAN_POINT('Ctrl Pts',(-1.02417440914999,-2.89944459712448,
98.9043158179233));
#23539=CARTESIAN_POINT('Ctrl Pts',(-1.11410022935702,-2.86446904834851,
98.8993319260815));
#23540=CARTESIAN_POINT('Ctrl Pts',(-1.2039933008072,-2.82950623680129,98.8943498492497));
#23541=CARTESIAN_POINT('Ctrl Pts',(-1.29227683896434,-2.79029310213957,
98.8893677724179));
#23542=CARTESIAN_POINT('Ctrl Pts',(-1.37852830909465,-2.74700963795627,
98.8843856955861));
#23543=CARTESIAN_POINT('Ctrl Pts',(-1.46477191507737,-2.70373012022803,
98.879404073005));
#23544=CARTESIAN_POINT('Ctrl Pts',(-1.54898342914967,-2.65638120788158,
98.8744224504239));
#23545=CARTESIAN_POINT('Ctrl Pts',(-1.6307633718706,-2.60518964280247,98.8694408278427));
#23546=CARTESIAN_POINT('Ctrl Pts',(-1.71255818362577,-2.55398877019501,
98.8644582995149));
#23547=CARTESIAN_POINT('Ctrl Pts',(-1.7919201739585,-2.49894409024715,98.859475771187));
#23548=CARTESIAN_POINT('Ctrl Pts',(-1.86847830577755,-2.4403260173261,98.8544932428591));
#23549=CARTESIAN_POINT('Ctrl Pts',(-1.94511895597981,-2.38164476276138,
98.8495053441));
#23550=CARTESIAN_POINT('Ctrl Pts',(-2.01894936512326,-2.31938269317944,
98.8445174453409));
#23551=CARTESIAN_POINT('Ctrl Pts',(-2.08963128892913,-2.25385077729835,
98.8395295465818));
#23552=CARTESIAN_POINT('Ctrl Pts',(-2.16035496551738,-2.18828015081523,
98.8345387014024));
#23553=CARTESIAN_POINT('Ctrl Pts',(-2.22792614615563,-2.1194361451444,98.8295478562231));
#23554=CARTESIAN_POINT('Ctrl Pts',(-2.29204469515411,-2.04766534507372,
98.8245570110437));
#23555=CARTESIAN_POINT('Ctrl Pts',(-2.35626686134706,-1.97577856157759,
98.8195581005325));
#23556=CARTESIAN_POINT('Ctrl Pts',(-2.41702497826903,-1.90095587990278,
98.8145591900213));
#23557=CARTESIAN_POINT('Ctrl Pts',(-2.47406034191185,-1.82357551929692,
98.8095602795101));
#23558=CARTESIAN_POINT('Ctrl Pts',(-2.507172755474,-1.77865162755117,98.8066581152801));
#23559=CARTESIAN_POINT('Ctrl Pts',(-2.53903123834827,-1.73286620261018,
98.8037559510502));
#23560=CARTESIAN_POINT('Ctrl Pts',(-2.56959224488766,-1.68629711053931,
98.8008537868202));
#23561=CARTESIAN_POINT('Ctrl Pts',(-2.62325694576495,-1.60452243492808,
98.7957576269441));
#23562=CARTESIAN_POINT('Ctrl Pts',(-2.67310143600297,-1.52005111545229,
98.7906614670681));
#23563=CARTESIAN_POINT('Ctrl Pts',(-2.71885041936436,-1.43326712343592,
98.785565307192));
#23564=CARTESIAN_POINT('Ctrl Pts',(-2.76453038786018,-1.34661404985973,
98.7804768351543));
#23565=CARTESIAN_POINT('Ctrl Pts',(-2.80612694355087,-1.25765560699959,
98.7753883631166));
#23566=CARTESIAN_POINT('Ctrl Pts',(-2.84340806514103,-1.16680453594033,
98.7702998910789));
#23567=CARTESIAN_POINT('Ctrl Pts',(-2.88118664928777,-1.07474118895833,
98.7651435207538));
#23568=CARTESIAN_POINT('Ctrl Pts',(-2.91453352864961,-0.980734682921244,
98.7599871504287));
#23569=CARTESIAN_POINT('Ctrl Pts',(-2.94325508540529,-0.885241070124925,
98.7548307801035));
#23570=CARTESIAN_POINT('Ctrl Pts',(-2.9715268151876,-0.791243044882755,
98.7497551670464));
#23571=CARTESIAN_POINT('Ctrl Pts',(-2.99531692166486,-0.695804569698325,
98.7446795539893));
#23572=CARTESIAN_POINT('Ctrl Pts',(-3.014489253313,-0.59938033973466,98.7396039409322));
#23573=CARTESIAN_POINT('Ctrl Pts',(-3.03411915681741,-0.500654824006531,
98.7344071919731));
#23574=CARTESIAN_POINT('Ctrl Pts',(-3.04890789387831,-0.400896316070449,
98.729210443014));
#23575=CARTESIAN_POINT('Ctrl Pts',(-3.05876400967397,-0.300607689727384,
98.7240136940548));
#23576=CARTESIAN_POINT('Ctrl Pts',(-3.06862012546962,-0.20031906338432,
98.7188169450957));
#23577=CARTESIAN_POINT('Ctrl Pts',(-3.07354354443464,-0.0995007836641929,
98.7136201961365));
#23578=CARTESIAN_POINT('Ctrl Pts',(-3.07349970959552,0.00133608243214189,
98.7084234471774));
#23579=CARTESIAN_POINT('Ctrl Pts',(-3.07349970959527,0.00133608300055935,
98.7084234471481));
#23580=CARTESIAN_POINT('Ctrl Pts',(-3.07345335998039,0.107957848126409,
98.7029285664721));
#23581=CARTESIAN_POINT('Ctrl Pts',(-3.06785451553832,0.214401037669215,
98.6974336857961));
#23582=CARTESIAN_POINT('Ctrl Pts',(-3.05678458077965,0.320109788522285,
98.6919388051201));
#23583=CARTESIAN_POINT('Ctrl Pts',(-3.04577427243555,0.425249156272434,
98.6864735217308));
#23584=CARTESIAN_POINT('Ctrl Pts',(-3.02935184224795,0.529661712284398,
98.6810082383416));
#23585=CARTESIAN_POINT('Ctrl Pts',(-3.00764794743082,0.632815987720909,
98.6755429549523));
#23586=CARTESIAN_POINT('Ctrl Pts',(-2.98576774618479,0.736808212386391,
98.6700332756329));
#23587=CARTESIAN_POINT('Ctrl Pts',(-2.95852002197215,0.839521339036963,
98.6645235963136));
#23588=CARTESIAN_POINT('Ctrl Pts',(-2.92608819126525,0.940430830491022,
98.6590139169942));
#23589=CARTESIAN_POINT('Ctrl Pts',(-2.89365636055835,1.04134032194509,98.6535042376748));
#23590=CARTESIAN_POINT('Ctrl Pts',(-2.85604060187747,1.14044592852212,98.6479945583555));
#23591=CARTESIAN_POINT('Ctrl Pts',(-2.8134715159663,1.23724705651146,98.6424848790361));
#23592=CARTESIAN_POINT('Ctrl Pts',(-2.77484412300311,1.32508486486674,98.6374853695654));
#23593=CARTESIAN_POINT('Ctrl Pts',(-2.73203143908153,1.41126627409199,98.6324858600948));
#23594=CARTESIAN_POINT('Ctrl Pts',(-2.68519747882601,1.49536508910247,98.6274863506241));
#23595=CARTESIAN_POINT('Ctrl Pts',(-2.63842704854006,1.57934982460463,98.6224936229563));
#23596=CARTESIAN_POINT('Ctrl Pts',(-2.5876463947889,1.66125720022001,98.6175008952884));
#23597=CARTESIAN_POINT('Ctrl Pts',(-2.53306732127339,1.74068153201465,98.6125081676206));
#23598=CARTESIAN_POINT('Ctrl Pts',(-2.4785458273042,1.82002207314196,98.6075207071546));
#23599=CARTESIAN_POINT('Ctrl Pts',(-2.42023412700094,1.8968844180998,98.6025332466886));
#23600=CARTESIAN_POINT('Ctrl Pts',(-2.35838909114258,1.97088892248641,98.5975457862225));
#23601=CARTESIAN_POINT('Ctrl Pts',(-2.2965883068507,2.04484047492304,98.5925618944008));
#23602=CARTESIAN_POINT('Ctrl Pts',(-2.23125949359266,2.11593791599362,98.5875780025792));
#23603=CARTESIAN_POINT('Ctrl Pts',(-2.16270125530425,2.18383276152397,98.5825941107575));
#23604=CARTESIAN_POINT('Ctrl Pts',(-2.09416798422655,2.25170288143481,98.5776120339457));
#23605=CARTESIAN_POINT('Ctrl Pts',(-2.02240793643468,2.3163724145637,98.5726299571338));
#23606=CARTESIAN_POINT('Ctrl Pts',(-1.94775754441361,2.37752871658364,98.567647880322));
#23607=CARTESIAN_POINT('Ctrl Pts',(-1.87311395878615,2.43867944255968,98.5626662577606));
#23608=CARTESIAN_POINT('Ctrl Pts',(-1.79558089255998,2.49631729625335,98.5576846351993));
#23609=CARTESIAN_POINT('Ctrl Pts',(-1.71552808955889,2.5501697245349,98.5527030126379));
#23610=CARTESIAN_POINT('Ctrl Pts',(-1.63546073154467,2.60403194413882,98.5477204843296));
#23611=CARTESIAN_POINT('Ctrl Pts',(-1.5528730911389,2.65410712646822,98.5427379560213));
#23612=CARTESIAN_POINT('Ctrl Pts',(-1.46816322085729,2.70016647763095,98.537755427713));
#23613=CARTESIAN_POINT('Ctrl Pts',(-1.38336204581268,2.74627547399003,98.532767528973));
#23614=CARTESIAN_POINT('Ctrl Pts',(-1.29643446048882,2.78835978774973,98.5277796302331));
#23615=CARTESIAN_POINT('Ctrl Pts',(-1.20780220683728,2.82623708827816,98.5227917314932));
#23616=CARTESIAN_POINT('Ctrl Pts',(-1.11911759689321,2.8641367634495,98.5178008863328));
#23617=CARTESIAN_POINT('Ctrl Pts',(-1.02872672471051,2.89782432384418,98.5128100411724));
#23618=CARTESIAN_POINT('Ctrl Pts',(-0.937068346938756,2.92716674673061,
98.507819196012));
#23619=CARTESIAN_POINT('Ctrl Pts',(-0.845261846903743,2.95655658771665,
98.5028202855192));
#23620=CARTESIAN_POINT('Ctrl Pts',(-0.752184174851212,2.98158715618758,
98.4978213750265));
#23621=CARTESIAN_POINT('Ctrl Pts',(-0.658286112490856,3.00217615141112,
98.4928224645337));
#23622=CARTESIAN_POINT('Ctrl Pts',(-0.603772710666914,3.01412928592272,
98.4899203001064));
#23623=CARTESIAN_POINT('Ctrl Pts',(-0.548982947401211,3.02458635673339,
98.4870181356791));
#23624=CARTESIAN_POINT('Ctrl Pts',(-0.494005672129448,3.03353929361463,
98.4841159712518));
#23625=CARTESIAN_POINT('Ctrl Pts',(-0.399285209413585,3.04896432731927,
98.4791158260815));
#23626=CARTESIAN_POINT('Ctrl Pts',(-0.303675206864667,3.0599758189329,98.4741156809111));
#23627=CARTESIAN_POINT('Ctrl Pts',(-0.207622622940845,3.06647926724496,
98.4691155357407));
#23628=CARTESIAN_POINT('Ctrl Pts',(-0.111730386717616,3.07297185886851,
98.4641237376834));
#23629=CARTESIAN_POINT('Ctrl Pts',(-0.0153974733967171,3.07497135061767,
98.4591319396262));
#23630=CARTESIAN_POINT('Ctrl Pts',(0.0809207697427157,3.07243455243952,
98.4541401415689));
#23631=CARTESIAN_POINT('Ctrl Pts',(0.177147010391447,3.06990017739268,98.4491531116411));
#23632=CARTESIAN_POINT('Ctrl Pts',(0.273358172546258,3.06283813231317,98.4441660817132));
#23633=CARTESIAN_POINT('Ctrl Pts',(0.369096078452734,3.05125717285037,98.4391790517854));
#23634=CARTESIAN_POINT('Ctrl Pts',(0.46476867590044,3.03968411344143,98.4341954238042));
#23635=CARTESIAN_POINT('Ctrl Pts',(0.559968224302033,3.02359831840271,98.4292117958229));
#23636=CARTESIAN_POINT('Ctrl Pts',(0.654239913682788,3.00306050311084,98.4242281678417));
#23637=CARTESIAN_POINT('Ctrl Pts',(0.748473032011306,2.98253109082046,98.4192465789007));
#23638=CARTESIAN_POINT('Ctrl Pts',(0.841778617905281,2.95755337362891,98.4142649899598));
#23639=CARTESIAN_POINT('Ctrl Pts',(0.933711384315625,2.92823928339188,98.4092834010188));
#23640=CARTESIAN_POINT('Ctrl Pts',(1.02566263452351,2.89891929932907,98.4043008104907));
#23641=CARTESIAN_POINT('Ctrl Pts',(1.11624009255976,2.86526132485732,98.3993182199626));
#23642=CARTESIAN_POINT('Ctrl Pts',(1.2050135810746,2.82742719082663,98.3943356294344));
#23643=CARTESIAN_POINT('Ctrl Pts',(1.29379444950277,2.78958991157055,98.3893526246938));
#23644=CARTESIAN_POINT('Ctrl Pts',(1.38077064941425,2.7475759621702,98.3843696199532));
#23645=CARTESIAN_POINT('Ctrl Pts',(1.46553343141306,2.70159471635008,98.3793866152126));
#23646=CARTESIAN_POINT('Ctrl Pts',(1.55037166299099,2.65557254141505,98.3743991749686));
#23647=CARTESIAN_POINT('Ctrl Pts',(1.63299216003407,2.60557623509644,98.3694117347245));
#23648=CARTESIAN_POINT('Ctrl Pts',(1.71301247083479,2.55186020870354,98.3644242944805));
#23649=CARTESIAN_POINT('Ctrl Pts',(1.76737212438089,2.51536966579796,98.3610362106173));
#23650=CARTESIAN_POINT('Ctrl Pts',(1.82053241882744,2.47716347201369,98.3576481267542));
#23651=CARTESIAN_POINT('Ctrl Pts',(1.87238193903531,2.43733217358127,98.354260042891));
#23652=CARTESIAN_POINT('',(-3.07349994395351,-0.00058695637196295,98.7915765527878));
#23653=CARTESIAN_POINT('Ctrl Pts',(-3.07349994395351,-0.000586956371967045,
98.7915765527878));
#23654=CARTESIAN_POINT('Ctrl Pts',(-3.07351817682241,0.094886445460421,
98.7866030213858));
#23655=CARTESIAN_POINT('Ctrl Pts',(-3.0690835429351,0.190535387119877,98.7816294899839));
#23656=CARTESIAN_POINT('Ctrl Pts',(-3.06017303934281,0.285907711122693,
98.7766559585819));
#23657=CARTESIAN_POINT('Ctrl Pts',(-3.05127451808939,0.381151783843896,
98.7716891153024));
#23658=CARTESIAN_POINT('Ctrl Pts',(-3.03791212734771,0.47611953978147,98.7667222720228));
#23659=CARTESIAN_POINT('Ctrl Pts',(-3.02011486886673,0.570358158397045,
98.7617554287432));
#23660=CARTESIAN_POINT('Ctrl Pts',(-3.00167035590524,0.668024067131597,
98.7566079502512));
#23661=CARTESIAN_POINT('Ctrl Pts',(-2.97846221221157,0.764906306697993,
98.7514604717592));
#23662=CARTESIAN_POINT('Ctrl Pts',(-2.95058168534517,0.860505646759896,
98.7463129932672));
#23663=CARTESIAN_POINT('Ctrl Pts',(-2.92372606122301,0.952590705099405,
98.7413547387758));
#23664=CARTESIAN_POINT('Ctrl Pts',(-2.89253567597502,1.04348506014707,98.7363964842844));
#23665=CARTESIAN_POINT('Ctrl Pts',(-2.85714392584538,1.13275365239088,98.7314382297929));
#23666=CARTESIAN_POINT('Ctrl Pts',(-2.82176350666418,1.22199366458953,98.7264815627259));
#23667=CARTESIAN_POINT('Ctrl Pts',(-2.78218455822006,1.30960853552735,98.7215248956588));
#23668=CARTESIAN_POINT('Ctrl Pts',(-2.73858945230785,1.39518101395775,98.7165682285918));
#23669=CARTESIAN_POINT('Ctrl Pts',(-2.69499608012731,1.48075008926038,98.7116117586461));
#23670=CARTESIAN_POINT('Ctrl Pts',(-2.64738707020622,1.56427653816429,98.7066552887005));
#23671=CARTESIAN_POINT('Ctrl Pts',(-2.59599128452805,1.64536667665733,98.7016988187549));
#23672=CARTESIAN_POINT('Ctrl Pts',(-2.54458313179807,1.72647632737169,98.6967411561644));
#23673=CARTESIAN_POINT('Ctrl Pts',(-2.4893866319005,1.80514812878637,98.6917834935739));
#23674=CARTESIAN_POINT('Ctrl Pts',(-2.43067395941607,1.88101737180085,98.6868258309835));
#23675=CARTESIAN_POINT('Ctrl Pts',(-2.37189661767665,1.95697018122809,98.6818627077601));
#23676=CARTESIAN_POINT('Ctrl Pts',(-2.30959564770612,2.03011392141336,98.6768995845368));
#23677=CARTESIAN_POINT('Ctrl Pts',(-2.24408326980453,2.10011726534101,98.6719364613135));
#23678=CARTESIAN_POINT('Ctrl Pts',(-2.17852785422086,2.17016659724463,98.6669700776175));
#23679=CARTESIAN_POINT('Ctrl Pts',(-2.10975715023411,2.23707111855631,98.6620036939215));
#23680=CARTESIAN_POINT('Ctrl Pts',(-2.03811839317448,2.30053812517938,98.6570373102255));
#23681=CARTESIAN_POINT('Ctrl Pts',(-1.96637053317777,2.36410178949327,98.6520633629275));
#23682=CARTESIAN_POINT('Ctrl Pts',(-1.89174625052971,2.4242172172049,98.6470894156295));
#23683=CARTESIAN_POINT('Ctrl Pts',(-1.81462350537452,2.4806337463927,98.6421154683315));
#23684=CARTESIAN_POINT('Ctrl Pts',(-1.79446902637195,2.49537707212139,98.6408156271993));
#23685=CARTESIAN_POINT('Ctrl Pts',(-1.77414405639444,2.50986802799386,98.6395157860671));
#23686=CARTESIAN_POINT('Ctrl Pts',(-1.75365561779317,2.52410265721948,98.638215944935));
#23687=CARTESIAN_POINT('Ctrl Pts',(-1.67485203117638,2.57885255099956,98.6332164354438));
#23688=CARTESIAN_POINT('Ctrl Pts',(-1.59334360087784,2.63000464830929,98.6282169259526));
#23689=CARTESIAN_POINT('Ctrl Pts',(-1.50949272260857,2.67728107795797,98.6232174164614));
#23690=CARTESIAN_POINT('Ctrl Pts',(-1.42575558752384,2.72449337742968,98.6182246887732));
#23691=CARTESIAN_POINT('Ctrl Pts',(-1.33968269867362,2.76784024406897,98.6132319610849));
#23692=CARTESIAN_POINT('Ctrl Pts',(-1.25166650240203,2.80708625032518,98.6082392333967));
#23693=CARTESIAN_POINT('Ctrl Pts',(-1.16374316099921,2.84629085303392,98.6032517729103));
#23694=CARTESIAN_POINT('Ctrl Pts',(-1.07388098651105,2.88140301797678,98.5982643124239));
#23695=CARTESIAN_POINT('Ctrl Pts',(-0.982497268071358,2.91223305527431,
98.5932768519375));
#23696=CARTESIAN_POINT('Ctrl Pts',(-0.89117893681916,2.94304103295921,98.5882929600957));
#23697=CARTESIAN_POINT('Ctrl Pts',(-0.79834164063746,2.96957283409185,98.583309068254));
#23698=CARTESIAN_POINT('Ctrl Pts',(-0.704421994544591,2.9916871333082,98.5783251764122));
#23699=CARTESIAN_POINT('Ctrl Pts',(-0.610536551661147,3.01379337904437,
98.5733430995804));
#23700=CARTESIAN_POINT('Ctrl Pts',(-0.515569968870673,3.03148521876159,
98.5683610227486));
#23701=CARTESIAN_POINT('Ctrl Pts',(-0.41997241371209,3.04467164431911,98.5633789459169));
#23702=CARTESIAN_POINT('Ctrl Pts',(-0.324383574848405,3.05785686757838,
98.5583973233357));
#23703=CARTESIAN_POINT('Ctrl Pts',(-0.228164312867165,3.06653743360497,
98.5534157007546));
#23704=CARTESIAN_POINT('Ctrl Pts',(-0.13177227556886,3.07067391909193,98.5484340781734));
#23705=CARTESIAN_POINT('Ctrl Pts',(-0.0353627124998721,3.07481115666483,
98.5434515498455));
#23706=CARTESIAN_POINT('Ctrl Pts',(0.0612192497179335,3.07440265409146,
98.5384690215176));
#23707=CARTESIAN_POINT('Ctrl Pts',(0.157514664773568,3.06946108956951,98.5334864931898));
#23708=CARTESIAN_POINT('Ctrl Pts',(0.25391387209432,3.06451419876931,98.5284985944307));
#23709=CARTESIAN_POINT('Ctrl Pts',(0.350025476538818,3.05502451416117,98.5235106956716));
#23710=CARTESIAN_POINT('Ctrl Pts',(0.445394584749105,3.04105671007237,98.5185227969125));
#23711=CARTESIAN_POINT('Ctrl Pts',(0.540820028800482,3.02708065501,98.5135319517332));
#23712=CARTESIAN_POINT('Ctrl Pts',(0.63550167263886,3.00862129722929,98.5085411065538));
#23713=CARTESIAN_POINT('Ctrl Pts',(0.728995853848436,2.98579424861657,98.5035502613745));
#23714=CARTESIAN_POINT('Ctrl Pts',(0.822641124016088,2.96293031091679,98.4985513508633));
#23715=CARTESIAN_POINT('Ctrl Pts',(0.915094679021009,2.93568471252292,98.4935524403521));
#23716=CARTESIAN_POINT('Ctrl Pts',(1.00592908130586,2.90422260396533,98.4885535298409));
#23717=CARTESIAN_POINT('Ctrl Pts',(1.05866384272606,2.88595698271581,98.4856513656108));
#23718=CARTESIAN_POINT('Ctrl Pts',(1.11085324558548,2.86627109189438,98.4827492013808));
#23719=CARTESIAN_POINT('Ctrl Pts',(1.16241729726026,2.8452044350152,98.4798470371507));
#23720=CARTESIAN_POINT('Ctrl Pts',(1.25124149116091,2.80891502883593,98.4748477713846));
#23721=CARTESIAN_POINT('Ctrl Pts',(1.33852068826598,2.76839840732892,98.4698485056184));
#23722=CARTESIAN_POINT('Ctrl Pts',(1.42382456802978,2.72380723427243,98.4648492398523));
#23723=CARTESIAN_POINT('Ctrl Pts',(1.50900204416191,2.67928213659528,98.4598573820183));
#23724=CARTESIAN_POINT('Ctrl Pts',(1.5922096376006,2.63069469437216,98.4548655241842));
#23725=CARTESIAN_POINT('Ctrl Pts',(1.67303641751327,2.57824579814927,98.4498736663502));
#23726=CARTESIAN_POINT('Ctrl Pts',(1.74125898300543,2.53397583884341,98.4456602441604));
#23727=CARTESIAN_POINT('Ctrl Pts',(1.80778554719658,2.48695574098692,98.4414468219706));
#23728=CARTESIAN_POINT('Ctrl Pts',(1.8723819390353,2.43733217358127,98.4372333997809));
#23729=CARTESIAN_POINT('Ctrl Pts',(1.87238193903529,2.43733217358128,99.4373602300224));
#23730=CARTESIAN_POINT('Ctrl Pts',(1.90947719062037,2.4088352457334,99.4349269813002));
#23731=CARTESIAN_POINT('Ctrl Pts',(1.94589304168592,2.37951330214532,99.432493732578));
#23732=CARTESIAN_POINT('Ctrl Pts',(1.9815920072363,2.3494031937616,99.4300604838558));
#23733=CARTESIAN_POINT('Ctrl Pts',(2.05494140039069,2.28753702638926,99.4250609743626));
#23734=CARTESIAN_POINT('Ctrl Pts',(2.12551961643353,2.22212390310521,99.4200614648694));
#23735=CARTESIAN_POINT('Ctrl Pts',(2.19296414688146,2.15344154796281,99.4150619553762));
#23736=CARTESIAN_POINT('Ctrl Pts',(2.26031718925207,2.08485235999908,99.4100692276858));
#23737=CARTESIAN_POINT('Ctrl Pts',(2.32454468933311,2.01300306435795,99.4050764999955));
#23738=CARTESIAN_POINT('Ctrl Pts',(2.38531731363497,1.9382114340993,99.4000837723052));
#23739=CARTESIAN_POINT('Ctrl Pts',(2.44602582435009,1.86349870712528,99.3950963118167));
#23740=CARTESIAN_POINT('Ctrl Pts',(2.5032864295953,1.7858501551383,99.3901088513282));
#23741=CARTESIAN_POINT('Ctrl Pts',(2.55680750521989,1.70561942743721,99.3851213908398));
#23742=CARTESIAN_POINT('Ctrl Pts',(2.61029028526379,1.62544610669723,99.3801374989959));
#23743=CARTESIAN_POINT('Ctrl Pts',(2.66003861199281,1.54269464731914,99.3751536071519));
#23744=CARTESIAN_POINT('Ctrl Pts',(2.70580254100521,1.45774993023144,99.370169715308));
#23745=CARTESIAN_POINT('Ctrl Pts',(2.7515498039281,1.37283614790586,99.3651876384741));
#23746=CARTESIAN_POINT('Ctrl Pts',(2.79331534416602,1.28573108091295,99.3602055616402));
#23747=CARTESIAN_POINT('Ctrl Pts',(2.83089428315928,1.19684577434861,99.3552234848062));
#23748=CARTESIAN_POINT('Ctrl Pts',(2.86846979581905,1.10796857207647,99.3502418622229));
#23749=CARTESIAN_POINT('Ctrl Pts',(2.90185929540075,1.0173118573331,99.3452602396396));
#23750=CARTESIAN_POINT('Ctrl Pts',(2.93090577140742,0.925307305240087,99.3402786170563));
#23751=CARTESIAN_POINT('Ctrl Pts',(2.9599575285752,0.833286025098481,99.3352960887262));
#23752=CARTESIAN_POINT('Ctrl Pts',(2.98466456182656,0.739916839519692,99.3303135603962));
#23753=CARTESIAN_POINT('Ctrl Pts',(3.00491983427052,0.645646218611726,99.3253310320661));
#23754=CARTESIAN_POINT('Ctrl Pts',(3.02519693891298,0.551273987867915,99.3203431333048));
#23755=CARTESIAN_POINT('Ctrl Pts',(3.04101261093616,0.455998811935668,99.3153552345435));
#23756=CARTESIAN_POINT('Ctrl Pts',(3.05231107613794,0.360276760956968,99.3103673357823));
#23757=CARTESIAN_POINT('Ctrl Pts',(3.06361621549819,0.26449816564895,99.3053764906007));
#23758=CARTESIAN_POINT('Ctrl Pts',(3.07039880401429,0.168272607348081,99.3003856454192));
#23759=CARTESIAN_POINT('Ctrl Pts',(3.0726551735271,0.0720585497850684,99.2953948002376));
#23760=CARTESIAN_POINT('Ctrl Pts',(3.07491518939003,-0.0243109921245982,
99.2903958897243));
#23761=CARTESIAN_POINT('Ctrl Pts',(3.07263439122162,-0.12066855764159,99.2853969792109));
#23762=CARTESIAN_POINT('Ctrl Pts',(3.06586116397397,-0.216558475327454,
99.2803980686975));
#23763=CARTESIAN_POINT('Ctrl Pts',(3.06192890360598,-0.272228263040121,
99.2774959044889));
#23764=CARTESIAN_POINT('Ctrl Pts',(3.05648344205991,-0.327740558712226,
99.2745937402803));
#23765=CARTESIAN_POINT('Ctrl Pts',(3.04954213539397,-0.383007851690783,
99.2716915760716));
#23766=CARTESIAN_POINT('Ctrl Pts',(3.03758446309371,-0.4782158881838,99.2666920665789));
#23767=CARTESIAN_POINT('Ctrl Pts',(3.02114285983535,-0.573030628378096,
99.2616925570862));
#23768=CARTESIAN_POINT('Ctrl Pts',(3.00025291010258,-0.666996795660201,
99.2566930475935));
#23769=CARTESIAN_POINT('Ctrl Pts',(2.97939129745398,-0.760835498433068,
99.2517003199037));
#23770=CARTESIAN_POINT('Ctrl Pts',(2.95409342525884,-0.85382749116087,99.2467075922139));
#23771=CARTESIAN_POINT('Ctrl Pts',(2.92444653297567,-0.945523519414831,
99.241714864524));
#23772=CARTESIAN_POINT('Ctrl Pts',(2.89483091741653,-1.03712281067037,99.2367274040361));
#23773=CARTESIAN_POINT('Ctrl Pts',(2.8608755369712,-1.12742843992935,99.2317399435481));
#23774=CARTESIAN_POINT('Ctrl Pts',(2.8227182547191,-1.21600325019121,99.2267524830602));
#23775=CARTESIAN_POINT('Ctrl Pts',(2.78458827489435,-1.30451468310593,99.2217685912167));
#23776=CARTESIAN_POINT('Ctrl Pts',(2.7422625433336,-1.39129735699729,99.2167846993733));
#23777=CARTESIAN_POINT('Ctrl Pts',(2.69592781257063,-1.47593207140712,99.2118008075299));
#23778=CARTESIAN_POINT('Ctrl Pts',(2.64960995576901,-1.56053596395017,99.2068187306965));
#23779=CARTESIAN_POINT('Ctrl Pts',(2.59928621116296,-1.64299306658165,99.2018366538631));
#23780=CARTESIAN_POINT('Ctrl Pts',(2.54518981375611,-1.72290773460222,99.1968545770296));
#23781=CARTESIAN_POINT('Ctrl Pts',(2.49109834869436,-1.80281511624624,99.1918729544468));
#23782=CARTESIAN_POINT('Ctrl Pts',(2.43323516094607,-1.88018016075809,99.186891331864));
#23783=CARTESIAN_POINT('Ctrl Pts',(2.3718768516627,-1.95463614275052,99.1819097092812));
#23784=CARTESIAN_POINT('Ctrl Pts',(2.3105073863576,-2.02910566215235,99.1769271809516));
#23785=CARTESIAN_POINT('Ctrl Pts',(2.2456418166526,-2.10066472987187,99.171944652622));
#23786=CARTESIAN_POINT('Ctrl Pts',(2.17759636182742,-2.16898048284349,99.1669621242925));
#23787=CARTESIAN_POINT('Ctrl Pts',(2.10947756403026,-2.23736987012866,99.1619742255317));
#23788=CARTESIAN_POINT('Ctrl Pts',(2.03817234882155,-2.30250865206996,99.1569863267708));
#23789=CARTESIAN_POINT('Ctrl Pts',(1.96403289796642,-2.36410173759625,99.15199842801));
#23790=CARTESIAN_POINT('Ctrl Pts',(1.88984965192002,-2.42573120700361,99.147007582829));
#23791=CARTESIAN_POINT('Ctrl Pts',(1.81282918689692,-2.48381054535344,99.1420167376479));
#23792=CARTESIAN_POINT('Ctrl Pts',(1.73335406160244,-2.53808706452839,99.1370258924669));
#23793=CARTESIAN_POINT('Ctrl Pts',(1.65375050249836,-2.59245129592906,99.1320269819539));
#23794=CARTESIAN_POINT('Ctrl Pts',(1.57168473581269,-2.64300020698688,99.127028071441));
#23795=CARTESIAN_POINT('Ctrl Pts',(1.48756531849523,-2.68952629160047,99.1220291609281));
#23796=CARTESIAN_POINT('Ctrl Pts',(1.43872900466873,-2.71653744481296,99.1191269967146));
#23797=CARTESIAN_POINT('Ctrl Pts',(1.38920092920491,-2.74219358975948,99.1162248325011));
#23798=CARTESIAN_POINT('Ctrl Pts',(1.33906394489779,-2.76646163925596,99.1133226682876));
#23799=CARTESIAN_POINT('Ctrl Pts',(1.25269380505265,-2.80826780007209,99.108323158795));
#23800=CARTESIAN_POINT('Ctrl Pts',(1.16421227589896,-2.84609874340984,99.1033236493024));
#23801=CARTESIAN_POINT('Ctrl Pts',(1.07402061397536,-2.87973644119666,99.0983241398098));
#23802=CARTESIAN_POINT('Ctrl Pts',(0.98395129646859,-2.91332850965997,99.0933314121201));
#23803=CARTESIAN_POINT('Ctrl Pts',(0.892176864380095,-2.94273848523513,
99.0883386844303));
#23804=CARTESIAN_POINT('Ctrl Pts',(0.799121646518137,-2.9677949464318,99.0833459567406));
#23805=CARTESIAN_POINT('Ctrl Pts',(0.706164599565391,-2.99282497369351,
99.0783584962527));
#23806=CARTESIAN_POINT('Ctrl Pts',(0.611929874548104,-3.01351050335598,
99.0733710357649));
#23807=CARTESIAN_POINT('Ctrl Pts',(0.51685921515451,-3.02972916309525,99.0683835752771));
#23808=CARTESIAN_POINT('Ctrl Pts',(0.421856581040128,-3.04593621800435,
99.0633996834338));
#23809=CARTESIAN_POINT('Ctrl Pts',(0.326019633074976,-3.0576826831781,99.0584157915905));
#23810=CARTESIAN_POINT('Ctrl Pts',(0.229801671077851,-3.06489697085723,
99.0534318997472));
#23811=CARTESIAN_POINT('Ctrl Pts',(0.133618749279474,-3.07210863127146,
99.0484498229139));
#23812=CARTESIAN_POINT('Ctrl Pts',(0.037055526428251,-3.07479136078171,
99.0434677460806));
#23813=CARTESIAN_POINT('Ctrl Pts',(-0.0594291485925616,-3.07292538573548,
99.0384856692473));
#23814=CARTESIAN_POINT('Ctrl Pts',(-0.155905026433875,-3.07105958082318,
99.0335040466646));
#23815=CARTESIAN_POINT('Ctrl Pts',(-0.252301931807038,-3.06464590459951,
99.0285224240819));
#23816=CARTESIAN_POINT('Ctrl Pts',(-0.348161662357746,-3.05371670376679,
99.0235408014992));
#23817=CARTESIAN_POINT('Ctrl Pts',(-0.444038821896402,-3.0427855158128,
99.0185582731698));
#23818=CARTESIAN_POINT('Ctrl Pts',(-0.539378176515784,-3.02733722249843,
99.0135757448403));
#23819=CARTESIAN_POINT('Ctrl Pts',(-0.63372835716399,-3.00745583830025,
99.0085932165109));
#23820=CARTESIAN_POINT('Ctrl Pts',(-0.728180233401813,-2.98755302489997,
99.0036053177502));
#23821=CARTESIAN_POINT('Ctrl Pts',(-0.821640376889052,-2.96320767200392,
98.9986174189896));
#23822=CARTESIAN_POINT('Ctrl Pts',(-0.913669521600026,-2.93455452416533,
98.9936295202289));
#23823=CARTESIAN_POINT('Ctrl Pts',(-1.00575302918991,-2.90588445051903,
98.988638675048));
#23824=CARTESIAN_POINT('Ctrl Pts',(-1.09640344253843,-2.87290166508771,
98.9836478298671));
#23825=CARTESIAN_POINT('Ctrl Pts',(-1.18520052411789,-2.83578947872205,
98.9786569846862));
#23826=CARTESIAN_POINT('Ctrl Pts',(-1.27414110402368,-2.79861731812599,
98.9736580741734));
#23827=CARTESIAN_POINT('Ctrl Pts',(-1.361221975422,-2.75730261968959,98.9686591636606));
#23828=CARTESIAN_POINT('Ctrl Pts',(-1.4460466443268,-2.71207510080956,98.9636602531478));
#23829=CARTESIAN_POINT('Ctrl Pts',(-1.49529239857694,-2.68581784205611,
98.960758088933));
#23830=CARTESIAN_POINT('Ctrl Pts',(-1.54377821304985,-2.65824260261122,
98.9578559247182));
#23831=CARTESIAN_POINT('Ctrl Pts',(-1.59143122513768,-2.62940086439036,
98.9549537605033));
#23832=CARTESIAN_POINT('Ctrl Pts',(-1.67352226780585,-2.57971568691305,
98.9499542510085));
#23833=CARTESIAN_POINT('Ctrl Pts',(-1.75342847792337,-2.52609517900815,
98.9449547415137));
#23834=CARTESIAN_POINT('Ctrl Pts',(-1.83074851047602,-2.46875720584059,
98.9399552320189));
#23835=CARTESIAN_POINT('Ctrl Pts',(-1.90796365889549,-2.41149701126953,
98.934962504327));
#23836=CARTESIAN_POINT('Ctrl Pts',(-1.9825992523572,-2.35052963273801,98.929969776635));
#23837=CARTESIAN_POINT('Ctrl Pts',(-2.05428047735531,-2.28611766327913,
98.9249770489431));
#23838=CARTESIAN_POINT('Ctrl Pts',(-2.12588608046794,-2.22177364682438,
98.919989588453));
#23839=CARTESIAN_POINT('Ctrl Pts',(-2.19454318632489,-2.15399255536408,
98.9150021279629));
#23840=CARTESIAN_POINT('Ctrl Pts',(-2.25990864192412,-2.08307829429349,
98.9100146674729));
#23841=CARTESIAN_POINT('Ctrl Pts',(-2.32522732701191,-2.01221477403436,
98.9050307756274));
#23842=CARTESIAN_POINT('Ctrl Pts',(-2.38725874731746,-1.93822286270734,
98.9000468837819));
#23843=CARTESIAN_POINT('Ctrl Pts',(-2.44569605578645,-1.86144380863635,
98.8950629919364));
#23844=CARTESIAN_POINT('Ctrl Pts',(-2.50411208283503,-1.78469271559525,
98.8900809151008));
#23845=CARTESIAN_POINT('Ctrl Pts',(-2.55893633307966,-1.70515684546293,
98.8850988382653));
#23846=CARTESIAN_POINT('Ctrl Pts',(-2.60990239954228,-1.62321031134707,
98.8801167614298));
#23847=CARTESIAN_POINT('Ctrl Pts',(-2.66086381907369,-1.5412712488674,98.8751351388449));
#23848=CARTESIAN_POINT('Ctrl Pts',(-2.707967522548,-1.45692233224867,98.87015351626));
#23849=CARTESIAN_POINT('Ctrl Pts',(-2.75099117314239,-1.37056550930361,
98.8651718936751));
#23850=CARTESIAN_POINT('Ctrl Pts',(-2.79402264619452,-1.28419298516657,
98.8601893653434));
#23851=CARTESIAN_POINT('Ctrl Pts',(-2.8329723973875,-1.19581222258103,98.8552068370118));
#23852=CARTESIAN_POINT('Ctrl Pts',(-2.8676651488311,-1.10584756823872,98.8502243086801));
#23853=CARTESIAN_POINT('Ctrl Pts',(-2.90239529394758,-1.01578594525843,
98.8452364099173));
#23854=CARTESIAN_POINT('Ctrl Pts',(-2.93285912076048,-0.924137432494293,
98.8402485111544));
#23855=CARTESIAN_POINT('Ctrl Pts',(-2.95893049288799,-0.831343844782441,
98.8352606123916));
#23856=CARTESIAN_POINT('Ctrl Pts',(-2.98501726573278,-0.738495442624959,
98.8302697672085));
#23857=CARTESIAN_POINT('Ctrl Pts',(-3.00670631880345,-0.644501046197165,
98.8252789220254));
#23858=CARTESIAN_POINT('Ctrl Pts',(-3.02392261284924,-0.549812951374382,
98.8202880768423));
#23859=CARTESIAN_POINT('Ctrl Pts',(-3.04116672886086,-0.45497183819986,
98.8152891663274));
#23860=CARTESIAN_POINT('Ctrl Pts',(-3.05392359488709,-0.359435222980361,
98.8102902558125));
#23861=CARTESIAN_POINT('Ctrl Pts',(-3.0621700243383,-0.263660751808075,
98.8052913452975));
#23862=CARTESIAN_POINT('Ctrl Pts',(-3.0669575659837,-0.208057987967436,
98.8023891811047));
#23863=CARTESIAN_POINT('Ctrl Pts',(-3.07022584521813,-0.152375079105688,
98.7994870169119));
#23864=CARTESIAN_POINT('Ctrl Pts',(-3.07197837451438,-0.0967011712233662,
98.7965848527191));
#23865=CARTESIAN_POINT('Ctrl Pts',(-3.07298649485838,-0.064675458851045,
98.7949154194203));
#23866=CARTESIAN_POINT('Ctrl Pts',(-3.07349382383657,-0.0326338998043769,
98.7932459861214));
#23867=CARTESIAN_POINT('Ctrl Pts',(-3.07349994395338,-0.000586957040365301,
98.7915765528226));
#23868=CARTESIAN_POINT('Origin',(0.,0.,116.208423447177));
#23869=CARTESIAN_POINT('',(1.8723819390353,2.43733217358127,100.43738386173));
#23870=CARTESIAN_POINT('',(1.87238193903531,2.43733217358127,100.354075679943));
#23871=CARTESIAN_POINT('',(1.8723819390353,2.43733217358128,116.208423447177));
#23872=CARTESIAN_POINT('',(-3.0734987850259,-0.00273284546552975,99.7084234472081));
#23873=CARTESIAN_POINT('Ctrl Pts',(1.87238193903531,2.43733217358127,100.354075679943));
#23874=CARTESIAN_POINT('Ctrl Pts',(1.94872699621459,2.378683168843,100.349088366481));
#23875=CARTESIAN_POINT('Ctrl Pts',(2.02239556219247,2.31638085683682,100.34410105302));
#23876=CARTESIAN_POINT('Ctrl Pts',(2.09302229050685,2.25070209966611,100.339113739558));
#23877=CARTESIAN_POINT('Ctrl Pts',(2.1635994165791,2.18506946970099,100.334129928764));
#23878=CARTESIAN_POINT('Ctrl Pts',(2.23113863126896,2.11606540665456,100.32914611797));
#23879=CARTESIAN_POINT('Ctrl Pts',(2.29530794381499,2.04400677422062,100.324162307176));
#23880=CARTESIAN_POINT('Ctrl Pts',(2.35945446148497,1.97197373918721,100.319180266782));
#23881=CARTESIAN_POINT('Ctrl Pts',(2.4202331638817,1.89688861821699,100.314198226387));
#23882=CARTESIAN_POINT('Ctrl Pts',(2.47734988312798,1.81910412196932,100.309216185993));
#23883=CARTESIAN_POINT('Ctrl Pts',(2.534461905551,1.74132602209799,100.304234555282));
#23884=CARTESIAN_POINT('Ctrl Pts',(2.58791228391867,1.66084934224848,100.299252924571));
#23885=CARTESIAN_POINT('Ctrl Pts',(2.63744867501404,1.57805790028968,100.29427129386));
#23886=CARTESIAN_POINT('Ctrl Pts',(2.68699451579225,1.4952506648334,100.289288712841));
#23887=CARTESIAN_POINT('Ctrl Pts',(2.73262466108324,1.41012816697903,100.284306131822));
#23888=CARTESIAN_POINT('Ctrl Pts',(2.77413198545853,1.32310013878615,100.279323550803));
#23889=CARTESIAN_POINT('Ctrl Pts',(2.81568425155709,1.23597788169224,100.274335574935));
#23890=CARTESIAN_POINT('Ctrl Pts',(2.85310459601087,1.1469463723038,100.269347599066));
#23891=CARTESIAN_POINT('Ctrl Pts',(2.88623356395202,1.05643649327199,100.264359623197));
#23892=CARTESIAN_POINT('Ctrl Pts',(2.91938236737993,0.965872422769139,100.25936866085));
#23893=CARTESIAN_POINT('Ctrl Pts',(2.94823454715684,0.873828638819195,100.254377698504));
#23894=CARTESIAN_POINT('Ctrl Pts',(2.97268079764369,0.780750360435693,100.249386736157));
#23895=CARTESIAN_POINT('Ctrl Pts',(2.99716631982083,0.687522556409266,100.244387756077));
#23896=CARTESIAN_POINT('Ctrl Pts',(3.0172316893431,0.593257368747633,100.239388775997));
#23897=CARTESIAN_POINT('Ctrl Pts',(3.03281889489707,0.498409270334469,100.234389795916));
#23898=CARTESIAN_POINT('Ctrl Pts',(3.04135810155053,0.44644822380602,100.231651182904));
#23899=CARTESIAN_POINT('Ctrl Pts',(3.0485542237069,0.394312318422457,100.228912569891));
#23900=CARTESIAN_POINT('Ctrl Pts',(3.05440435245981,0.342076455890416,100.226173956878));
#23901=CARTESIAN_POINT('Ctrl Pts',(3.06508412871854,0.246716618853292,100.221174447385));
#23902=CARTESIAN_POINT('Ctrl Pts',(3.071312619333,0.150688668851936,100.216174937892));
#23903=CARTESIAN_POINT('Ctrl Pts',(3.07301775946222,0.0544435490191098,
100.211175428399));
#23904=CARTESIAN_POINT('Ctrl Pts',(3.07472058657968,-0.0416710149198213,
100.206182700709));
#23905=CARTESIAN_POINT('Ctrl Pts',(3.07191225019029,-0.138001728073925,
100.201189973019));
#23906=CARTESIAN_POINT('Ctrl Pts',(3.06457231374881,-0.234091400534577,
100.196197245329));
#23907=CARTESIAN_POINT('Ctrl Pts',(3.05724012075527,-0.330079700812884,
100.19120978484));
#23908=CARTESIAN_POINT('Ctrl Pts',(3.04538586475535,-0.425827030554686,
100.186222324352));
#23909=CARTESIAN_POINT('Ctrl Pts',(3.02904115811324,-0.520876100868515,
100.181234863864));
#23910=CARTESIAN_POINT('Ctrl Pts',(3.0127081464908,-0.61585716135073,100.17625097202));
#23911=CARTESIAN_POINT('Ctrl Pts',(2.99189114574195,-0.710140524255589,
100.171267080177));
#23912=CARTESIAN_POINT('Ctrl Pts',(2.9666735038666,-0.803274904037155,100.166283188333));
#23913=CARTESIAN_POINT('Ctrl Pts',(2.94146504563184,-0.896375366584292,
100.161301111499));
#23914=CARTESIAN_POINT('Ctrl Pts',(2.91185924507951,-0.988327254113311,
100.156319034665));
#23915=CARTESIAN_POINT('Ctrl Pts',(2.87799015759056,-1.07869129171041,100.151336957832));
#23916=CARTESIAN_POINT('Ctrl Pts',(2.84412415818208,-1.16904709018915,100.146355335249));
#23917=CARTESIAN_POINT('Ctrl Pts',(2.80599579890358,-1.25781491560126,100.141373712665));
#23918=CARTESIAN_POINT('Ctrl Pts',(2.76378806945563,-1.34457344802533,100.136392090082));
#23919=CARTESIAN_POINT('Ctrl Pts',(2.7215726658988,-1.43134775467922,100.131409561753));
#23920=CARTESIAN_POINT('Ctrl Pts',(2.67527661121658,-1.51611164810015,100.126427033423));
#23921=CARTESIAN_POINT('Ctrl Pts',(2.62512934372775,-1.59846744686887,100.121444505093));
#23922=CARTESIAN_POINT('Ctrl Pts',(2.57492802487519,-1.68091201305121,100.116456606332));
#23923=CARTESIAN_POINT('Ctrl Pts',(2.52086743472272,-1.76094292721634,100.111468707571));
#23924=CARTESIAN_POINT('Ctrl Pts',(2.46322082222888,-1.83819080373559,100.10648080881));
#23925=CARTESIAN_POINT('Ctrl Pts',(2.40554015708981,-1.91548431163577,100.101489963628));
#23926=CARTESIAN_POINT('Ctrl Pts',(2.34426953038545,-1.98999116957381,100.096499118447));
#23927=CARTESIAN_POINT('Ctrl Pts',(2.27972165651885,-2.06137609833794,100.091508273266));
#23928=CARTESIAN_POINT('Ctrl Pts',(2.21506947165803,-2.13287638694966,100.086509362752));
#23929=CARTESIAN_POINT('Ctrl Pts',(2.1471297736734,-2.20124436124788,100.081510452239));
#23930=CARTESIAN_POINT('Ctrl Pts',(2.07625113663158,-2.26618257597134,100.076511541726));
#23931=CARTESIAN_POINT('Ctrl Pts',(2.03510188157209,-2.30388306334367,100.073609377515));
#23932=CARTESIAN_POINT('Ctrl Pts',(1.99296267411118,-2.34042831230001,100.070707213305));
#23933=CARTESIAN_POINT('Ctrl Pts',(1.94990630988358,-2.37576674626871,100.067805049094));
#23934=CARTESIAN_POINT('Ctrl Pts',(1.87573383511689,-2.43664367233664,100.062805539601));
#23935=CARTESIAN_POINT('Ctrl Pts',(1.79857744293256,-2.49415064949343,100.057806030108));
#23936=CARTESIAN_POINT('Ctrl Pts',(1.71877614513625,-2.54798171361385,100.052806520615));
#23937=CARTESIAN_POINT('Ctrl Pts',(1.63908309729366,-2.60173975623762,100.047813792925));
#23938=CARTESIAN_POINT('Ctrl Pts',(1.55675263514356,-2.65183155249234,100.042821065235));
#23939=CARTESIAN_POINT('Ctrl Pts',(1.47215711934522,-2.6979910426021,100.037828337545));
#23940=CARTESIAN_POINT('Ctrl Pts',(1.38765084968367,-2.74410183561333,100.032840877057));
#23941=CARTESIAN_POINT('Ctrl Pts',(1.30088465998618,-2.78628836027702,100.027853416568));
#23942=CARTESIAN_POINT('Ctrl Pts',(1.21225933204805,-2.82432816114955,100.02286595608));
#23943=CARTESIAN_POINT('Ctrl Pts',(1.12369741760369,-2.86234074365537,100.017882064237));
#23944=CARTESIAN_POINT('Ctrl Pts',(1.03327941162508,-2.89621232814008,100.012898172393));
#23945=CARTESIAN_POINT('Ctrl Pts',(0.941429227895216,-2.92576712314303,
100.007914280549));
#23946=CARTESIAN_POINT('Ctrl Pts',(0.849612493727385,-2.95531115502162,
100.002932203716));
#23947=CARTESIAN_POINT('Ctrl Pts',(0.756365035534493,-2.98054138662742,
99.9979501268819));
#23948=CARTESIAN_POINT('Ctrl Pts',(0.662128300386727,-3.00133109866722,
99.9929680500482));
#23949=CARTESIAN_POINT('Ctrl Pts',(0.567900157458148,-3.02211891516424,
99.9879864274651));
#23950=CARTESIAN_POINT('Ctrl Pts',(0.472683345601994,-3.03846692267068,
99.9830048048821));
#23951=CARTESIAN_POINT('Ctrl Pts',(0.376930893746072,-3.05029922324676,
99.978023182299));
#23952=CARTESIAN_POINT('Ctrl Pts',(0.28116103240736,-3.06213367514355,99.9730406539692));
#23953=CARTESIAN_POINT('Ctrl Pts',(0.184855773303206,-3.06945073573493,
99.9680581256394));
#23954=CARTESIAN_POINT('Ctrl Pts',(0.0884736065908541,-3.0722263378431,
99.9630755973096));
#23955=CARTESIAN_POINT('Ctrl Pts',(-0.00801244589267319,-3.07500493164128,
99.9580876985486));
#23956=CARTESIAN_POINT('Ctrl Pts',(-0.104575131968766,-3.07323228183818,
99.9530997997875));
#23957=CARTESIAN_POINT('Ctrl Pts',(-0.200755842999826,-3.06693647497,99.9481119010265));
#23958=CARTESIAN_POINT('Ctrl Pts',(-0.296993369297024,-3.0606369490823,
99.9431210558452));
#23959=CARTESIAN_POINT('Ctrl Pts',(-0.392848035282793,-3.04980899520767,
99.9381302106639));
#23960=CARTESIAN_POINT('Ctrl Pts',(-0.487868353496007,-3.03453237248461,
99.9331393654826));
#23961=CARTESIAN_POINT('Ctrl Pts',(-0.583042226943077,-3.01923106235344,
99.9281404549695));
#23962=CARTESIAN_POINT('Ctrl Pts',(-0.677378630961432,-2.99946681815902,
99.9231415444563));
#23963=CARTESIAN_POINT('Ctrl Pts',(-0.770438289065952,-2.97537007660243,
99.9181426339432));
#23964=CARTESIAN_POINT('Ctrl Pts',(-0.824464943183301,-2.96138048811747,
99.915240469732));
#23965=CARTESIAN_POINT('Ctrl Pts',(-0.878061573359936,-2.94593156383606,
99.9123383055208));
#23966=CARTESIAN_POINT('Ctrl Pts',(-0.931145283868457,-2.92905628323007,
99.9094361413096));
#23967=CARTESIAN_POINT('Ctrl Pts',(-1.02259169947179,-2.89998552105208,
99.9044366318167));
#23968=CARTESIAN_POINT('Ctrl Pts',(-1.11283602642308,-2.86657709801935,
99.8994371223238));
#23969=CARTESIAN_POINT('Ctrl Pts',(-1.20143704886778,-2.82894879197342,
99.8944376128309));
#23970=CARTESIAN_POINT('Ctrl Pts',(-1.28991788458815,-2.79137152848571,
99.8894448851408));
#23971=CARTESIAN_POINT('Ctrl Pts',(-1.37675944547547,-2.74958592866531,
99.8844521574508));
#23972=CARTESIAN_POINT('Ctrl Pts',(-1.46153583030011,-2.70375946910019,
99.8794594297608));
#23973=CARTESIAN_POINT('Ctrl Pts',(-1.54622277817571,-2.65798135529477,
99.8744719692726));
#23974=CARTESIAN_POINT('Ctrl Pts',(-1.62884849702787,-2.6081710639704,99.8694845087845));
#23975=CARTESIAN_POINT('Ctrl Pts',(-1.70900818667259,-2.55454365159143,
99.8644970482963));
#23976=CARTESIAN_POINT('Ctrl Pts',(-1.78911052018557,-2.5009546108796,99.8595131564527));
#23977=CARTESIAN_POINT('Ctrl Pts',(-1.86674996843881,-2.44355412207145,
99.8545292646091));
#23978=CARTESIAN_POINT('Ctrl Pts',(-1.94154827839042,-2.38260205084256,
99.8495453727655));
#23979=CARTESIAN_POINT('Ctrl Pts',(-2.01631934865012,-2.32167217684838,
99.8445632959318));
#23980=CARTESIAN_POINT('Ctrl Pts',(-2.08825099645011,-2.25719356728725,
99.8395812190982));
#23981=CARTESIAN_POINT('Ctrl Pts',(-2.15699658407839,-2.18946751203897,
99.8345991422646));
#23982=CARTESIAN_POINT('Ctrl Pts',(-2.22573590369289,-2.12174763184662,
99.8296175196816));
#23983=CARTESIAN_POINT('Ctrl Pts',(-2.29128942811944,-2.0507812028496,99.8246358970986));
#23984=CARTESIAN_POINT('Ctrl Pts',(-2.35334684244476,-1.97690689946575,
99.8196542745156));
#23985=CARTESIAN_POINT('Ctrl Pts',(-2.41541553990144,-1.90301916443189,
99.8146717461858));
#23986=CARTESIAN_POINT('Ctrl Pts',(-2.47398658253122,-1.82622284113484,
99.8096892178561));
#23987=CARTESIAN_POINT('Ctrl Pts',(-2.52879015728921,-1.7468894041688,99.8047066895263));
#23988=CARTESIAN_POINT('Ctrl Pts',(-2.58365280222392,-1.66747045744974,
99.7997187907653));
#23989=CARTESIAN_POINT('Ctrl Pts',(-2.63473962241708,-1.5855092993811,99.7947308920043));
#23990=CARTESIAN_POINT('Ctrl Pts',(-2.68182448644991,-1.50140589910847,
99.7897429932433));
#23991=CARTESIAN_POINT('Ctrl Pts',(-2.72893716415821,-1.41725281780289,
99.7847521480621));
#23992=CARTESIAN_POINT('Ctrl Pts',(-2.77204298251292,-1.33095536708632,
99.7797613028808));
#23993=CARTESIAN_POINT('Ctrl Pts',(-2.8109630298111,-1.24293567614547,99.7747704576996));
#23994=CARTESIAN_POINT('Ctrl Pts',(-2.84994597288857,-1.15477374316127,
99.7697715471865));
#23995=CARTESIAN_POINT('Ctrl Pts',(-2.8847294797668,-1.06488442165541,99.7647726366734));
#23996=CARTESIAN_POINT('Ctrl Pts',(-2.91518379497631,-0.973707189820183,
99.7597737261603));
#23997=CARTESIAN_POINT('Ctrl Pts',(-2.93286433225755,-0.920773395854607,
99.7568715619486));
#23998=CARTESIAN_POINT('Ctrl Pts',(-2.94908666272494,-0.867405765000334,
99.7539693977369));
#23999=CARTESIAN_POINT('Ctrl Pts',(-2.96383331659686,-0.813691785278971,
99.7510672335252));
#24000=CARTESIAN_POINT('Ctrl Pts',(-2.99602294044364,-0.696442623702255,
99.7447322659369));
#24001=CARTESIAN_POINT('Ctrl Pts',(-3.02127028321447,-0.57721156375486,
99.7383972983485));
#24002=CARTESIAN_POINT('Ctrl Pts',(-3.03937583012655,-0.45672400116763,
99.7320623307601));
#24003=CARTESIAN_POINT('Ctrl Pts',(-3.05716351922146,-0.338351697170771,
99.7258385787555));
#24004=CARTESIAN_POINT('Ctrl Pts',(-3.06805797241941,-0.218766467410884,
99.7196148267509));
#24005=CARTESIAN_POINT('Ctrl Pts',(-3.0719155261535,-0.0986775059325435,
99.7133910747463));
#24006=CARTESIAN_POINT('Ctrl Pts',(-3.0729418572233,-0.0667269380851964,
99.7117351989002));
#24007=CARTESIAN_POINT('Ctrl Pts',(-3.07347032466039,-0.0347408385625631,
99.7100793230542));
#24008=CARTESIAN_POINT('Ctrl Pts',(-3.0734987850259,-0.0027328454655318,
99.7084234472081));
#24009=CARTESIAN_POINT('Ctrl Pts',(-3.07349878502643,-0.00273284487125647,
99.7084234471774));
#24010=CARTESIAN_POINT('Ctrl Pts',(-3.07358364945221,0.0927100806662572,
99.7034858794082));
#24011=CARTESIAN_POINT('Ctrl Pts',(-3.06921850417963,0.18825319576249,99.6985483116391));
#24012=CARTESIAN_POINT('Ctrl Pts',(-3.06040211108497,0.283445177180123,
99.6936107438699));
#24013=CARTESIAN_POINT('Ctrl Pts',(-3.05159013460821,0.378589471680395,
99.6886756496009));
#24014=CARTESIAN_POINT('Ctrl Pts',(-3.03833137923279,0.473382536297822,
99.683740555332));
#24015=CARTESIAN_POINT('Ctrl Pts',(-3.02067664917373,0.567375388201277,
99.678805461063));
#24016=CARTESIAN_POINT('Ctrl Pts',(-3.00302571337087,0.661348039684788,
99.673871427417));
#24017=CARTESIAN_POINT('Ctrl Pts',(-2.98098076247416,0.754520379674263,
99.668937393771));
#24018=CARTESIAN_POINT('Ctrl Pts',(-2.95464399798693,0.846452063119824,
99.664003360125));
#24019=CARTESIAN_POINT('Ctrl Pts',(-2.92830536019262,0.938390285571876,
99.6590689755262));
#24020=CARTESIAN_POINT('Ctrl Pts',(-2.89767442726149,1.02908724559419,99.6541345909275));
#24021=CARTESIAN_POINT('Ctrl Pts',(-2.86290337241046,1.11811740449775,99.6492002063287));
#24022=CARTESIAN_POINT('Ctrl Pts',(-2.82809727594385,1.2072372863222,99.6442608489499));
#24023=CARTESIAN_POINT('Ctrl Pts',(-2.78914288936945,1.29468659433648,99.639321491571));
#24024=CARTESIAN_POINT('Ctrl Pts',(-2.74624057952636,1.38005975572174,99.6343821341922));
#24025=CARTESIAN_POINT('Ctrl Pts',(-2.70331618395766,1.46547686644732,99.6294402340764));
#24026=CARTESIAN_POINT('Ctrl Pts',(-2.65644003945883,1.5488153123457,99.6244983339605));
#24027=CARTESIAN_POINT('Ctrl Pts',(-2.60585741201884,1.62969610609661,99.6195564338447));
#24028=CARTESIAN_POINT('Ctrl Pts',(-2.55518929445766,1.71071359715271,99.6146061813821));
#24029=CARTESIAN_POINT('Ctrl Pts',(-2.50080243814957,1.7892647716427,99.6096559289196));
#24030=CARTESIAN_POINT('Ctrl Pts',(-2.44298415873699,1.86500151478763,99.6047056764571));
#24031=CARTESIAN_POINT('Ctrl Pts',(-2.39623608114133,1.9262372897251,99.6007032262184));
#24032=CARTESIAN_POINT('Ctrl Pts',(-2.34724563429205,1.98563375214153,99.5967007759797));
#24033=CARTESIAN_POINT('Ctrl Pts',(-2.29618206789302,2.04302475782515,99.592698325741));
#24034=CARTESIAN_POINT('Ctrl Pts',(-2.23239794323971,2.11471256419374,99.5876988162483));
#24035=CARTESIAN_POINT('Ctrl Pts',(-2.16514138169983,2.18353636970958,99.5826993067556));
#24036=CARTESIAN_POINT('Ctrl Pts',(-2.0946995960865,2.24914113655747,99.5776997972629));
#24037=CARTESIAN_POINT('Ctrl Pts',(-2.02435336430823,2.31465691095556,99.5727070695731));
#24038=CARTESIAN_POINT('Ctrl Pts',(-1.95083081411207,2.37696202841577,99.5677143418832));
#24039=CARTESIAN_POINT('Ctrl Pts',(-1.8744583160611,2.43573567353877,99.5627216141934));
#24040=CARTESIAN_POINT('Ctrl Pts',(-1.79816638907032,2.49444731394778,99.5577341537054));
#24041=CARTESIAN_POINT('Ctrl Pts',(-1.71903083723589,2.54963462202604,99.5527466932175));
#24042=CARTESIAN_POINT('Ctrl Pts',(-1.63741289766001,2.60101542720851,99.5477592327295));
#24043=CARTESIAN_POINT('Ctrl Pts',(-1.55585335762769,2.65235946822385,99.5427753408861));
#24044=CARTESIAN_POINT('Ctrl Pts',(-1.47181533128459,2.69990218762713,99.5377914490427));
#24045=CARTESIAN_POINT('Ctrl Pts',(-1.38569017429653,2.74340390589101,99.5328075571993));
#24046=CARTESIAN_POINT('Ctrl Pts',(-1.29959638195762,2.78688978190649,99.5278254803658));
#24047=CARTESIAN_POINT('Ctrl Pts',(-1.21141736058979,2.8263373830523,99.5228434035324));
#24048=CARTESIAN_POINT('Ctrl Pts',(-1.12156942919324,2.86155277174808,99.517861326699));
#24049=CARTESIAN_POINT('Ctrl Pts',(-1.03172968985804,2.89676494961175,99.5128797041162));
#24050=CARTESIAN_POINT('Ctrl Pts',(-0.940221751787076,2.92774552221313,
99.5078980815334));
#24051=CARTESIAN_POINT('Ctrl Pts',(-0.847481291008796,2.95434894881936,
99.5029164589506));
#24052=CARTESIAN_POINT('Ctrl Pts',(-0.754723968380491,2.98095721239736,
99.497933930621));
#24053=CARTESIAN_POINT('Ctrl Pts',(-0.660734099943554,3.00318662843291,
99.4929514022914));
#24054=CARTESIAN_POINT('Ctrl Pts',(-0.565960830078548,3.02094200355068,
99.4879688739618));
#24055=CARTESIAN_POINT('Ctrl Pts',(-0.471085408596105,3.03871651634608,
99.482980975201));
#24056=CARTESIAN_POINT('Ctrl Pts',(-0.375425332107708,3.05200727986838,
99.4779930764402));
#24057=CARTESIAN_POINT('Ctrl Pts',(-0.279437986122745,3.06077059936083,
99.4730051776794));
#24058=CARTESIAN_POINT('Ctrl Pts',(-0.183393939094897,3.0695390954664,99.4680143324983));
#24059=CARTESIAN_POINT('Ctrl Pts',(-0.0870226759677632,3.07377480306248,
99.4630234873172));
#24060=CARTESIAN_POINT('Ctrl Pts',(0.00921740284671422,3.07348617850882,
99.4580326421362));
#24061=CARTESIAN_POINT('Ctrl Pts',(0.105613008058961,3.0731970875306,99.4530337316233));
#24062=CARTESIAN_POINT('Ctrl Pts',(0.201876567531194,3.06836908705604,99.4480348211103));
#24063=CARTESIAN_POINT('Ctrl Pts',(0.297553848616778,3.05906259451704,99.4430359105974));
#24064=CARTESIAN_POINT('Ctrl Pts',(0.353100188262375,3.05365962330366,99.4401337463839));
#24065=CARTESIAN_POINT('Ctrl Pts',(0.408449077096889,3.04674814463559,99.4372315821705));
#24066=CARTESIAN_POINT('Ctrl Pts',(0.463513494017044,3.03834782256148,99.434329417957));
#24067=CARTESIAN_POINT('Ctrl Pts',(0.558371274461476,3.02387684563053,99.4293299487685));
#24068=CARTESIAN_POINT('Ctrl Pts',(0.652717335024171,3.00493397786565,99.42433047958));
#24069=CARTESIAN_POINT('Ctrl Pts',(0.746097510232636,2.98156682890467,99.4193310103915));
#24070=CARTESIAN_POINT('Ctrl Pts',(0.839355661825531,2.95823021473328,99.4143380742096));
#24071=CARTESIAN_POINT('Ctrl Pts',(0.931650013755398,2.93048091252956,99.4093451380278));
#24072=CARTESIAN_POINT('Ctrl Pts',(1.02253371972923,2.89841802402909,99.404352201846));
#24073=CARTESIAN_POINT('Ctrl Pts',(1.11330987119278,2.86639307971492,99.3993651744549));
#24074=CARTESIAN_POINT('Ctrl Pts',(1.20267828575442,2.8300648489633,99.3943781470639));
#24075=CARTESIAN_POINT('Ctrl Pts',(1.29020571752677,2.78958266707786,99.3893911196728));
#24076=CARTESIAN_POINT('Ctrl Pts',(1.37767342091869,2.74912811007655,99.38440749541));
#24077=CARTESIAN_POINT('Ctrl Pts',(1.46330224105315,2.70452541902491,99.3794238711471));
#24078=CARTESIAN_POINT('Ctrl Pts',(1.54667812735834,2.65597233049429,99.3744402468842));
#24079=CARTESIAN_POINT('Ctrl Pts',(1.63002246332206,2.60743761498003,99.3694585084789));
#24080=CARTESIAN_POINT('Ctrl Pts',(1.71111518098379,2.55495569354762,99.3644767700737));
#24081=CARTESIAN_POINT('Ctrl Pts',(1.78956701695306,2.49877012584866,99.3594950316684));
#24082=CARTESIAN_POINT('Ctrl Pts',(1.81751239887433,2.47875622651269,99.3577204832382));
#24083=CARTESIAN_POINT('Ctrl Pts',(1.84512294216106,2.4582727962739,99.3559459348079));
#24084=CARTESIAN_POINT('Ctrl Pts',(1.87238193903531,2.43733217358127,99.3541713863777));
#24085=CARTESIAN_POINT('',(-3.07349882820719,0.0026838422157513,99.7915765527815));
#24086=CARTESIAN_POINT('Ctrl Pts',(-3.07349882820719,0.00268384221573294,
99.7915765527815));
#24087=CARTESIAN_POINT('Ctrl Pts',(-3.07339561550422,0.120881596078696,
99.7854645576999));
#24088=CARTESIAN_POINT('Ctrl Pts',(-3.06647036213536,0.238780932134677,
99.7793525626182));
#24089=CARTESIAN_POINT('Ctrl Pts',(-3.05284834088149,0.355695456222244,
99.7732405675365));
#24090=CARTESIAN_POINT('Ctrl Pts',(-3.03901199464307,0.474449479977432,
99.7670324080731));
#24091=CARTESIAN_POINT('Ctrl Pts',(-3.01826654307125,0.592187533253163,
99.7608242486097));
#24092=CARTESIAN_POINT('Ctrl Pts',(-2.99079197937576,0.708212952509057,
99.7546160891463));
#24093=CARTESIAN_POINT('Ctrl Pts',(-2.97925928798004,0.756915649635332,
99.7520101592389));
#24094=CARTESIAN_POINT('Ctrl Pts',(-2.96654152276501,0.80531684908909,99.7494042293315));
#24095=CARTESIAN_POINT('Ctrl Pts',(-2.95265448210355,0.853366134384175,
99.7467982994241));
#24096=CARTESIAN_POINT('Ctrl Pts',(-2.92601201892033,0.945549296057218,
99.7417987899312));
#24097=CARTESIAN_POINT('Ctrl Pts',(-2.89500162464424,1.03664549094737,99.7367992804382));
#24098=CARTESIAN_POINT('Ctrl Pts',(-2.85972936878449,1.1262105430653,99.7317997709453));
#24099=CARTESIAN_POINT('Ctrl Pts',(-2.82450495951587,1.2156541007587,99.7268070432552));
#24100=CARTESIAN_POINT('Ctrl Pts',(-2.78503033786379,1.30357023861343,99.7218143155651));
#24101=CARTESIAN_POINT('Ctrl Pts',(-2.7414616596724,1.38952877571724,99.7168215878751));
#24102=CARTESIAN_POINT('Ctrl Pts',(-2.69793894533826,1.47539662873118,99.7118341273869));
#24103=CARTESIAN_POINT('Ctrl Pts',(-2.65033095802679,1.55931059706762,99.7068466668987));
#24104=CARTESIAN_POINT('Ctrl Pts',(-2.59884197479933,1.64086033531837,99.7018592064105));
#24105=CARTESIAN_POINT('Ctrl Pts',(-2.54738983314294,1.72235172282517,99.6968753145668));
#24106=CARTESIAN_POINT('Ctrl Pts',(-2.49206244968104,1.80148187308355,99.6918914227232));
#24107=CARTESIAN_POINT('Ctrl Pts',(-2.43310959700793,1.87786579364658,99.6869075308795));
#24108=CARTESIAN_POINT('Ctrl Pts',(-2.37417821350366,1.95422189707758,99.6819254540459));
#24109=CARTESIAN_POINT('Ctrl Pts',(-2.31162425201878,2.02783341077531,99.6769433772122));
#24110=CARTESIAN_POINT('Ctrl Pts',(-2.24573973087618,2.09834585117997,99.6719613003785));
#24111=CARTESIAN_POINT('Ctrl Pts',(-2.17986121688395,2.16885186247465,99.6669796777955));
#24112=CARTESIAN_POINT('Ctrl Pts',(-2.11065304680986,2.23625904165095,99.6619980552124));
#24113=CARTESIAN_POINT('Ctrl Pts',(-2.03844557093221,2.30024822668052,99.6570164326294));
#24114=CARTESIAN_POINT('Ctrl Pts',(-1.96622496646332,2.36424904607125,99.6520339042996));
#24115=CARTESIAN_POINT('Ctrl Pts',(-1.89100430171671,2.42483034600694,99.6470513759698));
#24116=CARTESIAN_POINT('Ctrl Pts',(-1.81314778667537,2.48171258482408,99.64206884764));
#24117=CARTESIAN_POINT('Ctrl Pts',(-1.73520735378508,2.53865613431153,99.637080948879));
#24118=CARTESIAN_POINT('Ctrl Pts',(-1.65462575371984,2.59189240353175,99.632093050118));
#24119=CARTESIAN_POINT('Ctrl Pts',(-1.57179683613089,2.64118476368635,99.6271051513569));
#24120=CARTESIAN_POINT('Ctrl Pts',(-1.48891899036346,2.69050624151464,99.6221143061757));
#24121=CARTESIAN_POINT('Ctrl Pts',(-1.40379157095317,2.73587896504871,99.6171234609943));
#24122=CARTESIAN_POINT('Ctrl Pts',(-1.3168318284825,2.77711292271226,99.6121326158131));
#24123=CARTESIAN_POINT('Ctrl Pts',(-1.22973155687197,2.8184135154927,99.6071337052999));
#24124=CARTESIAN_POINT('Ctrl Pts',(-1.1407934543542,2.85556181817568,99.6021347947868));
#24125=CARTESIAN_POINT('Ctrl Pts',(-1.05045341429752,2.88841649946657,99.5971358842737));
#24126=CARTESIAN_POINT('Ctrl Pts',(-0.998005659851746,2.9074905917036,99.5942337200625));
#24127=CARTESIAN_POINT('Ctrl Pts',(-0.945085660605878,2.92511845906008,
99.5913315558513));
#24128=CARTESIAN_POINT('Ctrl Pts',(-0.891780412032025,2.94128032440228,
99.5884293916401));
#24129=CARTESIAN_POINT('Ctrl Pts',(-0.799949516312664,2.96912295923802,
99.5834297275138));
#24130=CARTESIAN_POINT('Ctrl Pts',(-0.706652142229662,2.99270974290835,
99.5784300633876));
#24131=CARTESIAN_POINT('Ctrl Pts',(-0.612318651122561,3.01188779994997,
99.5734303992613));
#24132=CARTESIAN_POINT('Ctrl Pts',(-0.518113881799054,3.03103968777342,
99.5684375573746));
#24133=CARTESIAN_POINT('Ctrl Pts',(-0.422876231971961,3.04579471883114,
99.563444715488));
#24134=CARTESIAN_POINT('Ctrl Pts',(-0.327051584553492,3.05604965781662,
99.5584518736014));
#24135=CARTESIAN_POINT('Ctrl Pts',(-0.230216586280553,3.06641272228594,
99.5534063884522));
#24136=CARTESIAN_POINT('Ctrl Pts',(-0.132782570099405,3.0721800947961,99.5483609033031));
#24137=CARTESIAN_POINT('Ctrl Pts',(-0.0352210732845736,3.07329818371024,
99.543315418154));
#24138=CARTESIAN_POINT('Ctrl Pts',(0.0611469184591723,3.07440259463837,
99.5383316562493));
#24139=CARTESIAN_POINT('Ctrl Pts',(0.1576388379333,3.07097083768206,99.5333478943445));
#24140=CARTESIAN_POINT('Ctrl Pts',(0.253795789654246,3.0630034193833,99.5283641324398));
#24141=CARTESIAN_POINT('Ctrl Pts',(0.349916924314426,3.05503896883154,99.5233822269137));
#24142=CARTESIAN_POINT('Ctrl Pts',(0.445702902217803,3.04254225069144,99.5184003213875));
#24143=CARTESIAN_POINT('Ctrl Pts',(0.540697505617908,3.02556580781489,99.5134184158613));
#24144=CARTESIAN_POINT('Ctrl Pts',(0.63568265805823,3.00859105391512,99.5084370059821));
#24145=CARTESIAN_POINT('Ctrl Pts',(0.729876160657855,2.98713753949268,99.5034555961029));
#24146=CARTESIAN_POINT('Ctrl Pts',(0.822830638672055,2.96130916826706,99.4984741862237));
#24147=CARTESIAN_POINT('Ctrl Pts',(0.917864240869227,2.93490309070206,99.4933813565403));
#24148=CARTESIAN_POINT('Ctrl Pts',(1.01160225962071,2.90392420678091,99.4882885268569));
#24149=CARTESIAN_POINT('Ctrl Pts',(1.10358298894315,2.86853740371558,99.4831956971734));
#24150=CARTESIAN_POINT('Ctrl Pts',(1.19365258115027,2.83388585284088,99.4782086841746));
#24151=CARTESIAN_POINT('Ctrl Pts',(1.28203681523046,2.7950080159714,99.4732216711759));
#24152=CARTESIAN_POINT('Ctrl Pts',(1.36832381372345,2.75210686398572,99.4682346581771));
#24153=CARTESIAN_POINT('Ctrl Pts',(1.45735712672751,2.70784026809427,99.4630889201513));
#24154=CARTESIAN_POINT('Ctrl Pts',(1.54415701328919,2.65929019006871,99.4579431821255));
#24155=CARTESIAN_POINT('Ctrl Pts',(1.62830142014859,2.60672912577085,99.4527974440998));
#24156=CARTESIAN_POINT('Ctrl Pts',(1.712445827008,2.554168061473,99.447651706074));
#24157=CARTESIAN_POINT('Ctrl Pts',(1.79393437018822,2.49759634793658,99.4425059680482));
#24158=CARTESIAN_POINT('Ctrl Pts',(1.87238193903529,2.43733217358128,99.4373602300224));
#24159=CARTESIAN_POINT('Ctrl Pts',(1.8723819390353,2.43733217358127,100.43738386173));
#24160=CARTESIAN_POINT('Ctrl Pts',(1.94893925283926,2.37852011126932,100.43239647173));
#24161=CARTESIAN_POINT('Ctrl Pts',(2.02268566713518,2.31612623548597,100.427409081731));
#24162=CARTESIAN_POINT('Ctrl Pts',(2.09328189820265,2.25046065165715,100.422421691731));
#24163=CARTESIAN_POINT('Ctrl Pts',(2.16391581914448,2.18476001032501,100.417431639067));
#24164=CARTESIAN_POINT('Ctrl Pts',(2.23139590007027,2.11578449591865,100.412441586403));
#24165=CARTESIAN_POINT('Ctrl Pts',(2.29542082359019,2.04388000935195,100.407451533738));
#24166=CARTESIAN_POINT('Ctrl Pts',(2.3595536676993,1.97185432038267,100.402453069827));
#24167=CARTESIAN_POINT('Ctrl Pts',(2.42021944330251,1.89689013799153,100.397454605916));
#24168=CARTESIAN_POINT('Ctrl Pts',(2.47715805099304,1.81936534000193,100.392456142005));
#24169=CARTESIAN_POINT('Ctrl Pts',(2.52341480577271,1.756384425726,100.388395404857));
#24170=CARTESIAN_POINT('Ctrl Pts',(2.56721243459908,1.69171419247052,100.384334667709));
#24171=CARTESIAN_POINT('Ctrl Pts',(2.60843375910548,1.62556930776848,100.380273930561));
#24172=CARTESIAN_POINT('Ctrl Pts',(2.65918474240463,1.54413286730871,100.375274421068));
#24173=CARTESIAN_POINT('Ctrl Pts',(2.70620748898614,1.46017440983936,100.370274911575));
#24174=CARTESIAN_POINT('Ctrl Pts',(2.7492425500123,1.37406974029772,100.365275402082));
#24175=CARTESIAN_POINT('Ctrl Pts',(2.79221923425145,1.28808187119356,100.360282674392));
#24176=CARTESIAN_POINT('Ctrl Pts',(2.8312187889334,1.19995396537158,100.355289946702));
#24177=CARTESIAN_POINT('Ctrl Pts',(2.8660256549653,1.11008972388754,100.350297219012));
#24178=CARTESIAN_POINT('Ctrl Pts',(2.90079580063089,1.02032028691314,100.345309758524));
#24179=CARTESIAN_POINT('Ctrl Pts',(2.93138189296096,0.92881856291917,100.340322298035));
#24180=CARTESIAN_POINT('Ctrl Pts',(2.95761529276879,0.836010783411429,100.335334837547));
#24181=CARTESIAN_POINT('Ctrl Pts',(2.98382992196587,0.743269410039213,100.330350945703));
#24182=CARTESIAN_POINT('Ctrl Pts',(3.00569793096851,0.649224260121703,100.32536705386));
#24183=CARTESIAN_POINT('Ctrl Pts',(3.02309994888467,0.554318454548931,100.320383162016));
#24184=CARTESIAN_POINT('Ctrl Pts',(3.0404956294169,0.459447211320003,100.315401085182));
#24185=CARTESIAN_POINT('Ctrl Pts',(3.05342847126171,0.363716366508996,100.310419008349));
#24186=CARTESIAN_POINT('Ctrl Pts',(3.061830034121,0.267580066810998,100.305436931515));
#24187=CARTESIAN_POINT('Ctrl Pts',(3.07023083095134,0.171452532528594,100.300455308932));
#24188=CARTESIAN_POINT('Ctrl Pts',(3.07410113217776,0.0749200541701876,
100.295473686349));
#24189=CARTESIAN_POINT('Ctrl Pts',(3.07342439124172,-0.0215583236932937,
100.290492063766));
#24190=CARTESIAN_POINT('Ctrl Pts',(3.07274752726225,-0.118054243026111,
100.285509535436));
#24191=CARTESIAN_POINT('Ctrl Pts',(3.06752198234294,-0.214495603382103,
100.280527007106));
#24192=CARTESIAN_POINT('Ctrl Pts',(3.057783311344,-0.310424662142246,100.275544478776));
#24193=CARTESIAN_POINT('Ctrl Pts',(3.04803414349302,-0.406457118289549,
100.270556580015));
#24194=CARTESIAN_POINT('Ctrl Pts',(3.03376218247675,-0.501975733011638,
100.265568681254));
#24195=CARTESIAN_POINT('Ctrl Pts',(3.01505471239693,-0.596529405187283,
100.260580782493));
#24196=CARTESIAN_POINT('Ctrl Pts',(2.99633619155775,-0.691138931514897,
100.255589937312));
#24197=CARTESIAN_POINT('Ctrl Pts',(2.97317704991245,-0.784781954398285,
100.25059909213));
#24198=CARTESIAN_POINT('Ctrl Pts',(2.94571488551018,-0.877021130465937,
100.245608246949));
#24199=CARTESIAN_POINT('Ctrl Pts',(2.91820834155675,-0.969409367371377,
100.240609336436));
#24200=CARTESIAN_POINT('Ctrl Pts',(2.88638503449228,-1.06038881339784,100.235610425923));
#24201=CARTESIAN_POINT('Ctrl Pts',(2.85043123004095,-1.14954080084493,100.23061151541));
#24202=CARTESIAN_POINT('Ctrl Pts',(2.82955791289528,-1.20129882024089,100.227709351199));
#24203=CARTESIAN_POINT('Ctrl Pts',(2.8072932968787,-1.2524413162764,100.224807186988));
#24204=CARTESIAN_POINT('Ctrl Pts',(2.78368082639769,-1.302890366357,100.221905022777));
#24205=CARTESIAN_POINT('Ctrl Pts',(2.74300402048885,-1.38979809674736,100.216905513284));
#24206=CARTESIAN_POINT('Ctrl Pts',(2.69818192186844,-1.47495172703947,100.211906003791));
#24207=CARTESIAN_POINT('Ctrl Pts',(2.64938849549389,-1.55792902596511,100.206906494298));
#24208=CARTESIAN_POINT('Ctrl Pts',(2.60066125709239,-1.64079376671167,100.201913766608));
#24209=CARTESIAN_POINT('Ctrl Pts',(2.5479736180061,-1.72148766820019,100.196921038918));
#24210=CARTESIAN_POINT('Ctrl Pts',(2.49154683808155,-1.79961012545658,100.191928311228));
#24211=CARTESIAN_POINT('Ctrl Pts',(2.43517958698741,-1.87765016548986,100.18694085074));
#24212=CARTESIAN_POINT('Ctrl Pts',(2.37508129253556,-1.9531238002365,100.181953390251));
#24213=CARTESIAN_POINT('Ctrl Pts',(2.31151765855626,-2.02565751403898,100.176965929763));
#24214=CARTESIAN_POINT('Ctrl Pts',(2.24799950584286,-2.09813932827378,100.17198203792));
#24215=CARTESIAN_POINT('Ctrl Pts',(2.18102123127155,-2.1676850741982,100.166998146076));
#24216=CARTESIAN_POINT('Ctrl Pts',(2.1108895295578,-2.23395336656861,100.162014254232));
#24217=CARTESIAN_POINT('Ctrl Pts',(2.04078336807288,-2.3001975256682,100.157032177399));
#24218=CARTESIAN_POINT('Ctrl Pts',(1.96752637992255,-2.36316630152999,100.152050100565));
#24219=CARTESIAN_POINT('Ctrl Pts',(1.89146223742386,-2.4225550260829,100.147068023731));
#24220=CARTESIAN_POINT('Ctrl Pts',(1.81540503022257,-2.48193833575235,100.142086401148));
#24221=CARTESIAN_POINT('Ctrl Pts',(1.73654152365057,-2.53774197309553,100.137104778565));
#24222=CARTESIAN_POINT('Ctrl Pts',(1.65524775195289,-2.58970213145352,100.132123155982));
#24223=CARTESIAN_POINT('Ctrl Pts',(1.57393919961505,-2.64167173708388,100.127140627652));
#24224=CARTESIAN_POINT('Ctrl Pts',(1.49019987448773,-2.68979623951408,100.122158099322));
#24225=CARTESIAN_POINT('Ctrl Pts',(1.40443308544748,-2.73385624320308,100.117175570992));
#24226=CARTESIAN_POINT('Ctrl Pts',(1.31857385244889,-2.77796373708253,100.112187672231));
#24227=CARTESIAN_POINT('Ctrl Pts',(1.23068318387448,-2.81799778518139,100.10719977347));
#24228=CARTESIAN_POINT('Ctrl Pts',(1.14118698183003,-2.85378599802117,100.102211874709));
#24229=CARTESIAN_POINT('Ctrl Pts',(1.05163791315072,-2.88959535144945,100.097221029528));
#24230=CARTESIAN_POINT('Ctrl Pts',(0.960481837174163,-2.92115373209521,
100.092230184347));
#24231=CARTESIAN_POINT('Ctrl Pts',(0.86816050961901,-2.9483384438592,100.087239339165));
#24232=CARTESIAN_POINT('Ctrl Pts',(0.775689988467065,-2.97556708680391,
100.082240428652));
#24233=CARTESIAN_POINT('Ctrl Pts',(0.682050881821392,-2.9984078437609,100.077241518139));
#24234=CARTESIAN_POINT('Ctrl Pts',(0.587695777583457,-3.01678900869958,
100.072242607626));
#24235=CARTESIAN_POINT('Ctrl Pts',(0.532917040111328,-3.0274603657686,100.069340443415));
#24236=CARTESIAN_POINT('Ctrl Pts',(0.477897104043139,-3.03662958942373,
100.066438279204));
#24237=CARTESIAN_POINT('Ctrl Pts',(0.422724983624898,-3.04429069541976,
100.063536114993));
#24238=CARTESIAN_POINT('Ctrl Pts',(0.327680899375573,-3.05748835391485,
100.0585366055));
#24239=CARTESIAN_POINT('Ctrl Pts',(0.231851229668309,-3.06625395032696,
100.053537096007));
#24240=CARTESIAN_POINT('Ctrl Pts',(0.135684854326108,-3.07050352064714,
100.048537586514));
#24241=CARTESIAN_POINT('Ctrl Pts',(0.0396489280611693,-3.07474732645219,
100.043544858824));
#24242=CARTESIAN_POINT('Ctrl Pts',(-0.0567223613169125,-3.07448726189378,
100.038552131134));
#24243=CARTESIAN_POINT('Ctrl Pts',(-0.152972524177658,-3.06969080802069,
100.033559403444));
#24244=CARTESIAN_POINT('Ctrl Pts',(-0.249121145542297,-3.06489941428556,
100.028571942955));
#24245=CARTESIAN_POINT('Ctrl Pts',(-0.345148458332253,-3.05558116680173,
100.023584482467));
#24246=CARTESIAN_POINT('Ctrl Pts',(-0.440596497630456,-3.04175557470941,
100.018597021979));
#24247=CARTESIAN_POINT('Ctrl Pts',(-0.535976241625584,-3.02793987515138,
100.013613130135));
#24248=CARTESIAN_POINT('Ctrl Pts',(-0.630777102920117,-3.00962330509827,
100.008629238292));
#24249=CARTESIAN_POINT('Ctrl Pts',(-0.724545749788833,-2.98687724998249,
100.003645346448));
#24250=CARTESIAN_POINT('Ctrl Pts',(-0.818280248438755,-2.96413947841662,
99.9986632696142));
#24251=CARTESIAN_POINT('Ctrl Pts',(-0.91098285339435,-2.93697553023507,
99.9936811927805));
#24252=CARTESIAN_POINT('Ctrl Pts',(-1.00221089849853,-2.90550779811908,
99.9886991159468));
#24253=CARTESIAN_POINT('Ctrl Pts',(-1.09343062570669,-2.87404293513531,
99.9837174933637));
#24254=CARTESIAN_POINT('Ctrl Pts',(-1.1831756454572,-2.83827521170346,99.9787358707807));
#24255=CARTESIAN_POINT('Ctrl Pts',(-1.27101994632812,-2.79837641249995,
99.9737542481976));
#24256=CARTESIAN_POINT('Ctrl Pts',(-1.35888021884078,-2.75847035899171,
99.9687717198678));
#24257=CARTESIAN_POINT('Ctrl Pts',(-1.4448386864932,-2.71443191958095,99.9637891915379));
#24258=CARTESIAN_POINT('Ctrl Pts',(-1.52849173985072,-2.66647993639707,
99.9588066632081));
#24259=CARTESIAN_POINT('Ctrl Pts',(-1.61223495887111,-2.6184762680424,99.953818764447));
#24260=CARTESIAN_POINT('Ctrl Pts',(-1.69366742126704,-2.56655085328486,
99.948830865686));
#24261=CARTESIAN_POINT('Ctrl Pts',(-1.77241264500758,-2.51096707780433,
99.9438429669249));
#24262=CARTESIAN_POINT('Ctrl Pts',(-1.85120438463253,-2.45535046822476,
99.9388521217436));
#24263=CARTESIAN_POINT('Ctrl Pts',(-1.92730537871458,-2.39607146455465,
99.9338612765623));
#24264=CARTESIAN_POINT('Ctrl Pts',(-2.00037219612163,-2.33343380599998,
99.928870431381));
#24265=CARTESIAN_POINT('Ctrl Pts',(-2.07355709135082,-2.27069492340725,
99.9238715208678));
#24266=CARTESIAN_POINT('Ctrl Pts',(-2.14369769986152,-2.20458684894214,
99.9188726103547));
#24267=CARTESIAN_POINT('Ctrl Pts',(-2.21048746299902,-2.13545016938447,
99.9138736998415));
#24268=CARTESIAN_POINT('Ctrl Pts',(-2.24926288410972,-2.09531222401513,
99.9109715356305));
#24269=CARTESIAN_POINT('Ctrl Pts',(-2.28690964825366,-2.05415412424212,
99.9080693714194));
#24270=CARTESIAN_POINT('Ctrl Pts',(-2.32337427194694,-2.01204727639662,
99.9051672072084));
#24271=CARTESIAN_POINT('Ctrl Pts',(-2.38566669364708,-1.94011625786977,
99.900209447644));
#24272=CARTESIAN_POINT('Ctrl Pts',(-2.44473485011727,-1.8651516831922,99.8952516880796));
#24273=CARTESIAN_POINT('Ctrl Pts',(-2.50026567549644,-1.78747693745524,
99.8902939285151));
#24274=CARTESIAN_POINT('Ctrl Pts',(-2.55572621153801,-1.70990051019973,
99.8853424443416));
#24275=CARTESIAN_POINT('Ctrl Pts',(-2.607658049446,-1.62962108272174,99.8803909601681));
#24276=CARTESIAN_POINT('Ctrl Pts',(-2.65578668753765,-1.54699687145701,
99.8754394759946));
#24277=CARTESIAN_POINT('Ctrl Pts',(-2.70386808833047,-1.46445375420853,
99.8704928516041));
#24278=CARTESIAN_POINT('Ctrl Pts',(-2.74815347955921,-1.379570807569,99.8655462272136));
#24279=CARTESIAN_POINT('Ctrl Pts',(-2.78841090588688,-1.29273619502632,
99.8605996028231));
#24280=CARTESIAN_POINT('Ctrl Pts',(-2.82864026125435,-1.20596213108732,
99.855656427647));
#24281=CARTESIAN_POINT('Ctrl Pts',(-2.86484704507828,-1.11723950925545,
99.850713252471));
#24282=CARTESIAN_POINT('Ctrl Pts',(-2.89684519413524,-1.02698109584137,
99.8457700772949));
#24283=CARTESIAN_POINT('Ctrl Pts',(-2.92883661597063,-0.936741658160721,
99.8408279413613));
#24284=CARTESIAN_POINT('Ctrl Pts',(-2.9566210024437,-0.844967487724284,
99.8358858054277));
#24285=CARTESIAN_POINT('Ctrl Pts',(-2.98006075985854,-0.75209049824561,
99.8309436694941));
#24286=CARTESIAN_POINT('Ctrl Pts',(-3.00349711253167,-0.659226999613062,
99.8260022514304));
#24287=CARTESIAN_POINT('Ctrl Pts',(-3.02258998671406,-0.565261435023065,
99.8210608333667));
#24288=CARTESIAN_POINT('Ctrl Pts',(-3.03725230660657,-0.470638583217584,
99.8161194153029));
#24289=CARTESIAN_POINT('Ctrl Pts',(-3.05192271450474,-0.375963535704594,
99.811175271462));
#24290=CARTESIAN_POINT('Ctrl Pts',(-3.06215762251637,-0.280630919460878,
99.8062311276211));
#24291=CARTESIAN_POINT('Ctrl Pts',(-3.0679215976678,-0.185092735036906,
99.8012869837802));
#24292=CARTESIAN_POINT('Ctrl Pts',(-3.07169513153947,-0.122546217140886,
99.798050173461));
#24293=CARTESIAN_POINT('Ctrl Pts',(-3.07355348791211,-0.0599117111426067,
99.7948133631418));
#24294=CARTESIAN_POINT('Ctrl Pts',(-3.07349882820788,0.00268384142361682,
99.7915765528225));
#24295=CARTESIAN_POINT('Origin',(0.,0.,116.208423447177));
#24296=CARTESIAN_POINT('',(1.87238193903531,2.43733217358127,101.437247300765));
#24297=CARTESIAN_POINT('',(1.8723819390353,2.43733217358127,101.354247327612));
#24298=CARTESIAN_POINT('',(1.8723819390353,2.43733217358128,116.208423447177));
#24299=CARTESIAN_POINT('',(-3.0734998880982,0.000829373466577904,100.708423447224));
#24300=CARTESIAN_POINT('Ctrl Pts',(1.8723819390353,2.43733217358127,101.354247327612));
#24301=CARTESIAN_POINT('Ctrl Pts',(1.94878097456855,2.37864170215407,101.349247767036));
#24302=CARTESIAN_POINT('Ctrl Pts',(2.02231682918563,2.31643333910141,101.34424820646));
#24303=CARTESIAN_POINT('Ctrl Pts',(2.09266737696025,2.25103209648514,101.339248645885));
#24304=CARTESIAN_POINT('Ctrl Pts',(2.11373844172856,2.23144342429015,101.337751201045));
#24305=CARTESIAN_POINT('Ctrl Pts',(2.13452402208501,2.21156855431721,101.336253756206));
#24306=CARTESIAN_POINT('Ctrl Pts',(2.15501616577209,2.19141679633541,101.334756311367));
#24307=CARTESIAN_POINT('Ctrl Pts',(2.22343315463915,2.12413625104229,101.329756801874));
#24308=CARTESIAN_POINT('Ctrl Pts',(2.28881650109087,2.05353044898987,101.324757292381));
#24309=CARTESIAN_POINT('Ctrl Pts',(2.35082593556615,1.97990395491033,101.319757782888));
#24310=CARTESIAN_POINT('Ctrl Pts',(2.41275125463732,1.90637733470247,101.314765055198));
#24311=CARTESIAN_POINT('Ctrl Pts',(2.47131147724654,1.82983849895284,101.309772327508));
#24312=CARTESIAN_POINT('Ctrl Pts',(2.52620246685421,1.75062941437065,101.304779599818));
#24313=CARTESIAN_POINT('Ctrl Pts',(2.58103554785143,1.67150389337614,101.29979213933));
#24314=CARTESIAN_POINT('Ctrl Pts',(2.63220684236026,1.58971408254266,101.294804678841));
#24315=CARTESIAN_POINT('Ctrl Pts',(2.67945254972848,1.50563484409519,101.289817218353));
#24316=CARTESIAN_POINT('Ctrl Pts',(2.72666445168872,1.42161576630816,101.28483332651));
#24317=CARTESIAN_POINT('Ctrl Pts',(2.76995613594748,1.33531089903656,101.279849434666));
#24318=CARTESIAN_POINT('Ctrl Pts',(2.80910774232447,1.24712306610563,101.274865542822));
#24319=CARTESIAN_POINT('Ctrl Pts',(2.84824509065609,1.1589673489993,101.269883465989));
#24320=CARTESIAN_POINT('Ctrl Pts',(2.88324517883544,1.06893042949496,101.264901389155));
#24321=CARTESIAN_POINT('Ctrl Pts',(2.91393507687157,0.977437782049311,101.259919312321));
#24322=CARTESIAN_POINT('Ctrl Pts',(2.94462217669606,0.885953476625236,101.254937689738));
#24323=CARTESIAN_POINT('Ctrl Pts',(2.97099972828884,0.793014123380588,101.249956067155));
#24324=CARTESIAN_POINT('Ctrl Pts',(2.99294410379898,0.699062115648467,101.244974444572));
#24325=CARTESIAN_POINT('Ctrl Pts',(3.01489246918324,0.605093025785963,101.239991916242));
#24326=CARTESIAN_POINT('Ctrl Pts',(3.03240595790338,0.510111343237367,101.235009387912));
#24327=CARTESIAN_POINT('Ctrl Pts',(3.0454118986007,0.414570401574087,101.230026859582));
#24328=CARTESIAN_POINT('Ctrl Pts',(3.05843185778529,0.318926480856358,101.225038960821));
#24329=CARTESIAN_POINT('Ctrl Pts',(3.06693451014776,0.222722533263559,101.22005106206));
#24330=CARTESIAN_POINT('Ctrl Pts',(3.07089902991346,0.126417554463543,101.215063163299));
#24331=CARTESIAN_POINT('Ctrl Pts',(3.07486589157541,0.0300556869906981,
101.210072318118));
#24332=CARTESIAN_POINT('Ctrl Pts',(3.07428928547725,-0.0664068917735554,
101.205081472937));
#24333=CARTESIAN_POINT('Ctrl Pts',(3.06920052266676,-0.162512773842821,
101.200090627755));
#24334=CARTESIAN_POINT('Ctrl Pts',(3.06410353628706,-0.258773965444505,
101.195091717242));
#24335=CARTESIAN_POINT('Ctrl Pts',(3.05447987696273,-0.354676872871681,
101.190092806729));
#24336=CARTESIAN_POINT('Ctrl Pts',(3.04041254424233,-0.44977084255639,101.185093896216));
#24337=CARTESIAN_POINT('Ctrl Pts',(3.0322456227786,-0.504978535267258,101.182191732005));
#24338=CARTESIAN_POINT('Ctrl Pts',(3.02258192059223,-0.559913777938571,
101.179289567794));
#24339=CARTESIAN_POINT('Ctrl Pts',(3.01144541790487,-0.614490638642901,
101.176387403583));
#24340=CARTESIAN_POINT('Ctrl Pts',(2.99226075196033,-0.708509278992459,
101.17138789409));
#24341=CARTESIAN_POINT('Ctrl Pts',(2.96863521495117,-0.801793764721477,
101.166388384597));
#24342=CARTESIAN_POINT('Ctrl Pts',(2.94063901313135,-0.893892859603363,
101.161388875104));
#24343=CARTESIAN_POINT('Ctrl Pts',(2.91268078798154,-0.985867022647843,
101.156396147414));
#24344=CARTESIAN_POINT('Ctrl Pts',(2.88036380765222,-1.07665857419504,101.151403419724));
#24345=CARTESIAN_POINT('Ctrl Pts',(2.84380932356711,-1.16582622255324,101.146410692034));
#24346=CARTESIAN_POINT('Ctrl Pts',(2.8072934035413,-1.25489980129004,101.141423231546));
#24347=CARTESIAN_POINT('Ctrl Pts',(2.76654903238328,-1.34235247853228,101.136435771057));
#24348=CARTESIAN_POINT('Ctrl Pts',(2.72174701495846,-1.42775888600447,101.131448310569));
#24349=CARTESIAN_POINT('Ctrl Pts',(2.67697705442436,-1.51310418319572,101.126464418726));
#24350=CARTESIAN_POINT('Ctrl Pts',(2.62815542265787,-1.5964057336758,101.121480526882));
#24351=CARTESIAN_POINT('Ctrl Pts',(2.57550030195752,-1.6772598023612,101.116496635038));
#24352=CARTESIAN_POINT('Ctrl Pts',(2.522864356948,-1.75808442599732,101.111514558204));
#24353=CARTESIAN_POINT('Ctrl Pts',(2.46639793613185,-1.83646297131814,101.106532481371));
#24354=CARTESIAN_POINT('Ctrl Pts',(2.40636377219734,-1.91201873574925,101.101550404537));
#24355=CARTESIAN_POINT('Ctrl Pts',(2.34633508199547,-1.98756761123537,101.096568781954));
#24356=CARTESIAN_POINT('Ctrl Pts',(2.282739568645,-2.0602938739694,101.091587159371));
#24357=CARTESIAN_POINT('Ctrl Pts',(2.21588099888434,-2.12985296412296,101.086605536788));
#24358=CARTESIAN_POINT('Ctrl Pts',(2.14901027305768,-2.19942470134469,101.081623008458));
#24359=CARTESIAN_POINT('Ctrl Pts',(2.0788756167751,-2.26582780590346,101.076640480128));
#24360=CARTESIAN_POINT('Ctrl Pts',(2.00581771670423,-2.32875450345361,101.071657951798));
#24361=CARTESIAN_POINT('Ctrl Pts',(1.93268107098425,-2.39174902670966,101.066670053037));
#24362=CARTESIAN_POINT('Ctrl Pts',(1.85661522429097,-2.45125937535987,101.061682154276));
#24363=CARTESIAN_POINT('Ctrl Pts',(1.777993840024,-2.50701817999725,101.056694255515));
#24364=CARTESIAN_POINT('Ctrl Pts',(1.69932601302621,-2.56280992212586,101.051703410334));
#24365=CARTESIAN_POINT('Ctrl Pts',(1.61810001205964,-2.61484547096914,101.046712565153));
#24366=CARTESIAN_POINT('Ctrl Pts',(1.5347165547633,-2.66290205350018,101.041721719971));
#24367=CARTESIAN_POINT('Ctrl Pts',(1.45119834769425,-2.71103629668218,101.036722809458));
#24368=CARTESIAN_POINT('Ctrl Pts',(1.36551611247566,-2.75517853314257,101.031723898945));
#24369=CARTESIAN_POINT('Ctrl Pts',(1.27809304307741,-2.7951530232238,101.026724988432));
#24370=CARTESIAN_POINT('Ctrl Pts',(1.22733876320914,-2.81836058698402,101.023822824221));
#24371=CARTESIAN_POINT('Ctrl Pts',(1.17599808773117,-2.84016432677214,101.02092066001));
#24372=CARTESIAN_POINT('Ctrl Pts',(1.1241561517504,-2.86053757124106,101.018018495799));
#24373=CARTESIAN_POINT('Ctrl Pts',(1.0348489202403,-2.89563421695802,101.013018986306));
#24374=CARTESIAN_POINT('Ctrl Pts',(0.943739652778536,-2.92660618265729,
101.008019476813));
#24375=CARTESIAN_POINT('Ctrl Pts',(0.851245066735334,-2.95326668053509,
101.00301996732));
#24376=CARTESIAN_POINT('Ctrl Pts',(0.758875949010772,-2.97989101361682,
100.99802723963));
#24377=CARTESIAN_POINT('Ctrl Pts',(0.665125665624834,-3.00221538180517,
100.99303451194));
#24378=CARTESIAN_POINT('Ctrl Pts',(0.570430384170966,-3.02010122790852,
100.98804178425));
#24379=CARTESIAN_POINT('Ctrl Pts',(0.475835003852092,-3.03796820489507,
100.983054323761));
#24380=CARTESIAN_POINT('Ctrl Pts',(0.380297036382195,-3.05140588734464,
100.978066863273));
#24381=CARTESIAN_POINT('Ctrl Pts',(0.284266272364707,-3.06032595263901,
100.973079402785));
#24382=CARTESIAN_POINT('Ctrl Pts',(0.188304220603611,-3.06923963541815,
100.968095510941));
#24383=CARTESIAN_POINT('Ctrl Pts',(0.0918505090894153,-3.07364208653821,
100.963111619098));
#24384=CARTESIAN_POINT('Ctrl Pts',(-0.00463742261154345,-3.07349650143148,
100.958127727254));
#24385=CARTESIAN_POINT('Ctrl Pts',(-0.101090215797521,-3.07335096934323,
100.95314565042));
#24386=CARTESIAN_POINT('Ctrl Pts',(-0.197576765896115,-3.06866069254261,
100.948163573586));
#24387=CARTESIAN_POINT('Ctrl Pts',(-0.293638052471836,-3.05944095287694,
100.943181496753));
#24388=CARTESIAN_POINT('Ctrl Pts',(-0.389690580471286,-3.05022205383911,
100.93819987417));
#24389=CARTESIAN_POINT('Ctrl Pts',(-0.485317485101434,-3.03647455514257,
100.933218251587));
#24390=CARTESIAN_POINT('Ctrl Pts',(-0.580064365961525,-3.01826565784751,
100.928236629004));
#24391=CARTESIAN_POINT('Ctrl Pts',(-0.674828473473925,-3.0000534498541,
100.923254100674));
#24392=CARTESIAN_POINT('Ctrl Pts',(-0.768711808385901,-2.97737831517518,
100.918271572344));
#24393=CARTESIAN_POINT('Ctrl Pts',(-0.861270724562729,-2.95035845093629,
100.913289044014));
#24394=CARTESIAN_POINT('Ctrl Pts',(-0.953929405610073,-2.92330946326588,
100.908301145253));
#24395=CARTESIAN_POINT('Ctrl Pts',(-1.04526039592031,-2.89190652011422,
100.903313246492));
#24396=CARTESIAN_POINT('Ctrl Pts',(-1.13483598647635,-2.85631747776718,
100.898325347731));
#24397=CARTESIAN_POINT('Ctrl Pts',(-1.22446449056317,-2.82070741248435,
100.89333450255));
#24398=CARTESIAN_POINT('Ctrl Pts',(-1.31233513051131,-2.78090650531461,
100.888343657368));
#24399=CARTESIAN_POINT('Ctrl Pts',(-1.39804287468036,-2.73712958599981,
100.883352812187));
#24400=CARTESIAN_POINT('Ctrl Pts',(-1.48388912472846,-2.69328192207785,
100.878353901674));
#24401=CARTESIAN_POINT('Ctrl Pts',(-1.56756511884022,-2.64544563374788,
100.873354991161));
#24402=CARTESIAN_POINT('Ctrl Pts',(-1.64869303932916,-2.59388001111608,
100.868356080647));
#24403=CARTESIAN_POINT('Ctrl Pts',(-1.69579261167301,-2.56394310703961,
100.865453916436));
#24404=CARTESIAN_POINT('Ctrl Pts',(-1.74203393130438,-2.53275002469661,
100.862551752225));
#24405=CARTESIAN_POINT('Ctrl Pts',(-1.78734827456124,-2.50035765350139,
100.859649588015));
#24406=CARTESIAN_POINT('Ctrl Pts',(-1.86486694926472,-2.44494443320328,
100.854684892352));
#24407=CARTESIAN_POINT('Ctrl Pts',(-1.93995177014106,-2.38581864905339,
100.84972019669));
#24408=CARTESIAN_POINT('Ctrl Pts',(-2.012222153803,-2.32322281620692,100.844755501028));
#24409=CARTESIAN_POINT('Ctrl Pts',(-2.0843942196799,-2.26071213973193,100.839797559417));
#24410=CARTESIAN_POINT('Ctrl Pts',(-2.1537591213382,-2.19474108272794,100.834839617806));
#24411=CARTESIAN_POINT('Ctrl Pts',(-2.21996586383073,-2.12559493164297,
100.829881676195));
#24412=CARTESIAN_POINT('Ctrl Pts',(-2.28754560356957,-2.05501482577546,
100.824820916654));
#24413=CARTESIAN_POINT('Ctrl Pts',(-2.35183433745526,-1.98112672110582,
100.819760157114));
#24414=CARTESIAN_POINT('Ctrl Pts',(-2.41249487126628,-1.90427696150374,
100.814699397573));
#24415=CARTESIAN_POINT('Ctrl Pts',(-2.47181879393756,-1.82912053096285,
100.809750148222));
#24416=CARTESIAN_POINT('Ctrl Pts',(-2.52767247112215,-1.75113198889134,
100.80480089887));
#24417=CARTESIAN_POINT('Ctrl Pts',(-2.57977928200124,-1.67067085512293,
100.799851649518));
#24418=CARTESIAN_POINT('Ctrl Pts',(-2.63186879451738,-1.59023643275504,
100.794904043213));
#24419=CARTESIAN_POINT('Ctrl Pts',(-2.68021366949828,-1.50733142313592,
100.789956436908));
#24420=CARTESIAN_POINT('Ctrl Pts',(-2.72458015982701,-1.42234496613058,
100.785008830603));
#24421=CARTESIAN_POINT('Ctrl Pts',(-2.76894446929391,-1.33736268668626,
100.7800614675));
#24422=CARTESIAN_POINT('Ctrl Pts',(-2.80933057728387,-1.25029955885745,
100.775114104398));
#24423=CARTESIAN_POINT('Ctrl Pts',(-2.84555087825066,-1.1615689601943,100.770166741295));
#24424=CARTESIAN_POINT('Ctrl Pts',(-2.88322011483119,-1.06928883485691,
100.765021466789));
#24425=CARTESIAN_POINT('Ctrl Pts',(-2.91638305279106,-0.975205509234439,
100.759876192283));
#24426=CARTESIAN_POINT('Ctrl Pts',(-2.94488468889632,-0.879804761923921,
100.754730917777));
#24427=CARTESIAN_POINT('Ctrl Pts',(-2.97232631723532,-0.787952075246951,
100.749777001793));
#24428=CARTESIAN_POINT('Ctrl Pts',(-2.99544715264274,-0.69487867798545,
100.744823085808));
#24429=CARTESIAN_POINT('Ctrl Pts',(-3.01416077415875,-0.601030013828543,
100.739869169823));
#24430=CARTESIAN_POINT('Ctrl Pts',(-3.03288686416883,-0.507118820272323,
100.734911953148));
#24431=CARTESIAN_POINT('Ctrl Pts',(-3.04719983161355,-0.412431771858417,
100.729954736472));
#24432=CARTESIAN_POINT('Ctrl Pts',(-3.05706504618843,-0.317420152751691,
100.724997519797));
#24433=CARTESIAN_POINT('Ctrl Pts',(-3.06694455849489,-0.222270832572669,
100.72003311859));
#24434=CARTESIAN_POINT('Ctrl Pts',(-3.07236343782549,-0.126796446613842,
100.715068717382));
#24435=CARTESIAN_POINT('Ctrl Pts',(-3.0733391029767,-0.0314484993980698,
100.710104316174));
#24436=CARTESIAN_POINT('Ctrl Pts',(-3.07344921798623,-0.0206873892944004,
100.709544026524));
#24437=CARTESIAN_POINT('Ctrl Pts',(-3.07350279090739,-0.00992788374707534,
100.708983736874));
#24438=CARTESIAN_POINT('Ctrl Pts',(-3.0734998880982,0.000829373466577527,
100.708423447224));
#24439=CARTESIAN_POINT('Ctrl Pts',(-3.07349988809796,0.000829374362847938,
100.708423447177));
#24440=CARTESIAN_POINT('Ctrl Pts',(-3.07348755274493,0.0465417906926426,
100.706042524862));
#24441=CARTESIAN_POINT('Ctrl Pts',(-3.07245544142314,0.0922390841767112,
100.703661602546));
#24442=CARTESIAN_POINT('Ctrl Pts',(-3.07040526815993,0.137890316033153,
100.701280680231));
#24443=CARTESIAN_POINT('Ctrl Pts',(-3.06610027230853,0.233749708641906,
100.696281170738));
#24444=CARTESIAN_POINT('Ctrl Pts',(-3.0572942542034,0.329575672356581,100.691281661245));
#24445=CARTESIAN_POINT('Ctrl Pts',(-3.04398627306699,0.424911543006023,
100.686282151752));
#24446=CARTESIAN_POINT('Ctrl Pts',(-3.0306963441225,0.520118091152141,100.681289424061));
#24447=CARTESIAN_POINT('Ctrl Pts',(-3.01291664934247,0.614835436466869,
100.676296696371));
#24448=CARTESIAN_POINT('Ctrl Pts',(-2.99069821909291,0.708608786506702,
100.671303968681));
#24449=CARTESIAN_POINT('Ctrl Pts',(-2.96850322872718,0.802283208026099,
100.666316508193));
#24450=CARTESIAN_POINT('Ctrl Pts',(-2.94187891259058,0.895015189177,100.661329047705));
#24451=CARTESIAN_POINT('Ctrl Pts',(-2.91092773001718,0.986357947510458,
100.656341587216));
#24452=CARTESIAN_POINT('Ctrl Pts',(-2.87999869373841,1.07763534796513,100.651357695373));
#24453=CARTESIAN_POINT('Ctrl Pts',(-2.84474908614237,1.16752508711852,100.646373803529));
#24454=CARTESIAN_POINT('Ctrl Pts',(-2.80533153550899,1.25559437155427,100.641389911685));
#24455=CARTESIAN_POINT('Ctrl Pts',(-2.76592833977128,1.34363158333789,100.636407834852));
#24456=CARTESIAN_POINT('Ctrl Pts',(-2.72236039596523,1.42984925738979,100.631425758018));
#24457=CARTESIAN_POINT('Ctrl Pts',(-2.67482854984605,1.51383436310861,100.626443681184));
#24458=CARTESIAN_POINT('Ctrl Pts',(-2.62730103753619,1.59781181132066,100.621462058601));
#24459=CARTESIAN_POINT('Ctrl Pts',(-2.57581055784407,1.67955671397915,100.616480436018));
#24460=CARTESIAN_POINT('Ctrl Pts',(-2.52060349661687,1.75868139890169,100.611498813435));
#24461=CARTESIAN_POINT('Ctrl Pts',(-2.46538639777322,1.83782047008608,100.606516285105));
#24462=CARTESIAN_POINT('Ctrl Pts',(-2.40645162657808,1.91433801742719,100.601533756775));
#24463=CARTESIAN_POINT('Ctrl Pts',(-2.34408776827968,1.98787695408986,100.596551228446));
#24464=CARTESIAN_POINT('Ctrl Pts',(-2.28165669093311,2.06149515488822,100.591563329684));
#24465=CARTESIAN_POINT('Ctrl Pts',(-2.21578943204242,2.13212800019319,100.586575430923));
#24466=CARTESIAN_POINT('Ctrl Pts',(-2.14681344500452,2.19945317803035,100.581587532162));
#24467=CARTESIAN_POINT('Ctrl Pts',(-2.07779671290436,2.26681812577413,100.576596686981));
#24468=CARTESIAN_POINT('Ctrl Pts',(-2.00566792421729,2.33087122420806,100.5716058418));
#24469=CARTESIAN_POINT('Ctrl Pts',(-1.93078820320179,2.39132999905425,100.566614996618));
#24470=CARTESIAN_POINT('Ctrl Pts',(-1.85578747466614,2.4518864768074,100.561616086105));
#24471=CARTESIAN_POINT('Ctrl Pts',(-1.77802729087215,2.50883677345381,100.556617175592));
#24472=CARTESIAN_POINT('Ctrl Pts',(-1.69789830452878,2.56194137276369,100.551618265079));
#24473=CARTESIAN_POINT('Ctrl Pts',(-1.65137867273835,2.59277174413127,100.548716100868));
#24474=CARTESIAN_POINT('Ctrl Pts',(-1.60406112681858,2.62230677207033,100.545813936657));
#24475=CARTESIAN_POINT('Ctrl Pts',(-1.55602560798124,2.65050684913407,100.542911772446));
#24476=CARTESIAN_POINT('Ctrl Pts',(-1.47327562728728,2.69908664777214,100.537912262953));
#24477=CARTESIAN_POINT('Ctrl Pts',(-1.38810309789947,2.7438728232548,100.53291275346));
#24478=CARTESIAN_POINT('Ctrl Pts',(-1.30089055399368,2.78461595494424,100.527913243967));
#24479=CARTESIAN_POINT('Ctrl Pts',(-1.21379631335,2.82530381883421,100.522920516277));
#24480=CARTESIAN_POINT('Ctrl Pts',(-1.12466795224931,2.86195935453384,100.517927788587));
#24481=CARTESIAN_POINT('Ctrl Pts',(-1.03391473064704,2.89437775346465,100.512935060897));
#24482=CARTESIAN_POINT('Ctrl Pts',(-0.94325725140587,2.92676195180178,100.507947600409));
#24483=CARTESIAN_POINT('Ctrl Pts',(-0.850978730544745,2.95491775272394,
100.50296013992));
#24484=CARTESIAN_POINT('Ctrl Pts',(-0.757509709879373,2.97868784692832,
100.497972679432));
#24485=CARTESIAN_POINT('Ctrl Pts',(-0.664107568483129,3.00244093307467,
100.492988787589));
#24486=CARTESIAN_POINT('Ctrl Pts',(-0.569517044882587,3.02181444297084,
100.488004895745));
#24487=CARTESIAN_POINT('Ctrl Pts',(-0.47418426156171,3.03670076498939,100.483021003901));
#24488=CARTESIAN_POINT('Ctrl Pts',(-0.378886196079398,3.05158166577816,
100.478038927068));
#24489=CARTESIAN_POINT('Ctrl Pts',(-0.282846841221909,3.0619785578591,100.473056850234));
#24490=CARTESIAN_POINT('Ctrl Pts',(-0.186521994656168,3.06783503394649,
100.4680747734));
#24491=CARTESIAN_POINT('Ctrl Pts',(-0.0902059306972084,3.0736909760582,
100.463093150817));
#24492=CARTESIAN_POINT('Ctrl Pts',(0.00639513505272708,3.07500729879151,
100.458111528234));
#24493=CARTESIAN_POINT('Ctrl Pts',(0.102821880998748,3.07177959996935,100.453129905651));
#24494=CARTESIAN_POINT('Ctrl Pts',(0.199266159026103,3.06855131429468,100.448147377321));
#24495=CARTESIAN_POINT('Ctrl Pts',(0.29553561559349,3.06077738098397,100.443164848991));
#24496=CARTESIAN_POINT('Ctrl Pts',(0.391173608329545,3.04850544663224,100.438182320662));
#24497=CARTESIAN_POINT('Ctrl Pts',(0.486914684726831,3.0362202849439,100.4331944219));
#24498=CARTESIAN_POINT('Ctrl Pts',(0.582022502373442,3.01942749922723,100.428206523139));
#24499=CARTESIAN_POINT('Ctrl Pts',(0.676048425958704,2.99822627160773,100.423218624378));
#24500=CARTESIAN_POINT('Ctrl Pts',(0.770129891947641,2.97701252013206,100.418227779197));
#24501=CARTESIAN_POINT('Ctrl Pts',(0.863127768352573,2.95138525807356,100.413236934016));
#24502=CARTESIAN_POINT('Ctrl Pts',(0.954608503262189,2.92149360011271,100.408246088834));
#24503=CARTESIAN_POINT('Ctrl Pts',(1.04623707334957,2.89155363647774,100.403247178321));
#24504=CARTESIAN_POINT('Ctrl Pts',(1.13634319626868,2.85733567212782,100.398248267808));
#24505=CARTESIAN_POINT('Ctrl Pts',(1.22451327617656,2.81903697855622,100.393249357295));
#24506=CARTESIAN_POINT('Ctrl Pts',(1.27570123997732,2.79680231411894,100.390347193084));
#24507=CARTESIAN_POINT('Ctrl Pts',(1.32623710529685,2.77319311371393,100.387445028873));
#24508=CARTESIAN_POINT('Ctrl Pts',(1.37604412559679,2.74825486707666,100.384542864662));
#24509=CARTESIAN_POINT('Ctrl Pts',(1.46319056629028,2.70462086892769,100.379465000542));
#24510=CARTESIAN_POINT('Ctrl Pts',(1.54841499802168,2.65675983856468,100.374387136422));
#24511=CARTESIAN_POINT('Ctrl Pts',(1.63128015375264,2.60486608292495,100.369309272302));
#24512=CARTESIAN_POINT('Ctrl Pts',(1.71414530948361,2.55297232728521,100.364231408183));
#24513=CARTESIAN_POINT('Ctrl Pts',(1.7946507457641,2.4970460213523,100.359153544063));
#24514=CARTESIAN_POINT('Ctrl Pts',(1.87238193903531,2.43733217358127,100.354075679943));
#24515=CARTESIAN_POINT('',(-3.0734996196979,-0.00152895940825499,100.791576552855));
#24516=CARTESIAN_POINT('Ctrl Pts',(-3.07349961969821,-0.00152895878437358,
100.791576552823));
#24517=CARTESIAN_POINT('Ctrl Pts',(-3.07354837615827,0.0964808522008683,
100.786524377151));
#24518=CARTESIAN_POINT('Ctrl Pts',(-3.06890468339488,0.19448503801226,100.781472201478));
#24519=CARTESIAN_POINT('Ctrl Pts',(-3.05959658800328,0.292011932425183,
100.776420025806));
#24520=CARTESIAN_POINT('Ctrl Pts',(-3.05028541410575,0.389571082322173,
100.771366179206));
#24521=CARTESIAN_POINT('Ctrl Pts',(-3.03630680849132,0.486652207185376,
100.766312332606));
#24522=CARTESIAN_POINT('Ctrl Pts',(-3.01774058051128,0.582789875285645,
100.761258486006));
#24523=CARTESIAN_POINT('Ctrl Pts',(-2.99916372480891,0.678982574727879,
100.756201746471));
#24524=CARTESIAN_POINT('Ctrl Pts',(-2.97599410203961,0.774230329524674,
100.751145006937));
#24525=CARTESIAN_POINT('Ctrl Pts',(-2.94836220263535,0.868079818951714,
100.746088267403));
#24526=CARTESIAN_POINT('Ctrl Pts',(-2.92068929198974,0.962068599710314,
100.74102402266));
#24527=CARTESIAN_POINT('Ctrl Pts',(-2.88854100335846,1.0546545678525,100.735959777917));
#24528=CARTESIAN_POINT('Ctrl Pts',(-2.85209712144358,1.14540135317419,100.730895533175));
#24529=CARTESIAN_POINT('Ctrl Pts',(-2.81562133876217,1.23622757273446,100.725826855499));
#24530=CARTESIAN_POINT('Ctrl Pts',(-2.77484264850276,1.32521102066264,100.720758177823));
#24531=CARTESIAN_POINT('Ctrl Pts',(-2.72998732910008,1.41193889136642,100.715689500148));
#24532=CARTESIAN_POINT('Ctrl Pts',(-2.68505404545288,1.49881750612927,100.710612012466));
#24533=CARTESIAN_POINT('Ctrl Pts',(-2.63603019868476,1.58343235411485,100.705534524784));
#24534=CARTESIAN_POINT('Ctrl Pts',(-2.58318596836571,1.66539860178833,100.700457037103));
#24535=CARTESIAN_POINT('Ctrl Pts',(-2.57123361704824,1.68393779485544,100.699308606778));
#24536=CARTESIAN_POINT('Ctrl Pts',(-2.5590859869867,1.70234162478948,100.698160176454));
#24537=CARTESIAN_POINT('Ctrl Pts',(-2.54674648514763,1.72060587886598,100.697011746129));
#24538=CARTESIAN_POINT('Ctrl Pts',(-2.49302841861834,1.80011641570814,100.692012236636));
#24539=CARTESIAN_POINT('Ctrl Pts',(-2.43548890078887,1.87724854367466,100.687012727143));
#24540=CARTESIAN_POINT('Ctrl Pts',(-2.37436554489057,1.9516122845577,100.68201321765));
#24541=CARTESIAN_POINT('Ctrl Pts',(-2.31332510243647,2.02587515149837,100.67702048996));
#24542=CARTESIAN_POINT('Ctrl Pts',(-2.24871076007897,2.09737675855472,100.67202776227));
#24543=CARTESIAN_POINT('Ctrl Pts',(-2.18080347983684,2.16575585704657,100.66703503458));
#24544=CARTESIAN_POINT('Ctrl Pts',(-2.11296784006364,2.23406281731314,100.662047574092));
#24545=CARTESIAN_POINT('Ctrl Pts',(-2.04184647611333,2.29925350781209,100.657060113603));
#24546=CARTESIAN_POINT('Ctrl Pts',(-1.96776003170119,2.36100036163473,100.652072653115));
#24547=CARTESIAN_POINT('Ctrl Pts',(-1.89372659787175,2.42270303414017,100.647088761271));
#24548=CARTESIAN_POINT('Ctrl Pts',(-1.81673263742507,2.48096648834149,100.642104869428));
#24549=CARTESIAN_POINT('Ctrl Pts',(-1.73713427956381,2.53550128076566,100.637120977584));
#24550=CARTESIAN_POINT('Ctrl Pts',(-1.65756490945309,2.59001621296908,100.63213890075));
#24551=CARTESIAN_POINT('Ctrl Pts',(-1.57539338816331,2.64080493352111,100.627156823917));
#24552=CARTESIAN_POINT('Ctrl Pts',(-1.49100665160184,2.68762002799486,100.622174747083));
#24553=CARTESIAN_POINT('Ctrl Pts',(-1.40662760916653,2.73443085401058,100.6171931245));
#24554=CARTESIAN_POINT('Ctrl Pts',(-1.32003413696557,2.77726856148609,100.612211501917));
#24555=CARTESIAN_POINT('Ctrl Pts',(-1.23163877272392,2.8159311396984,100.607229879334));
#24556=CARTESIAN_POINT('Ctrl Pts',(-1.14322733664759,2.85460074744863,100.602247351004));
#24557=CARTESIAN_POINT('Ctrl Pts',(-1.05301376007122,2.8890935424676,100.597264822674));
#24558=CARTESIAN_POINT('Ctrl Pts',(-0.961430604396251,2.91925563165172,
100.592282294344));
#24559=CARTESIAN_POINT('Ctrl Pts',(-0.869748735576916,2.9494502311227,100.587294395583));
#24560=CARTESIAN_POINT('Ctrl Pts',(-0.776694758177426,2.97530466826145,
100.582306496822));
#24561=CARTESIAN_POINT('Ctrl Pts',(-0.682716228799109,2.99671500161999,
100.577318598061));
#24562=CARTESIAN_POINT('Ctrl Pts',(-0.588682185013639,3.01813798235631,
100.57232775288));
#24563=CARTESIAN_POINT('Ctrl Pts',(-0.493722933696055,3.03511155492146,
100.567336907699));
#24564=CARTESIAN_POINT('Ctrl Pts',(-0.398293950692616,3.04758333419148,
100.562346062517));
#24565=CARTESIAN_POINT('Ctrl Pts',(-0.302710752042614,3.06007526817177,
100.557347152004));
#24566=CARTESIAN_POINT('Ctrl Pts',(-0.206656743117444,3.0680508459679,100.552348241491));
#24567=CARTESIAN_POINT('Ctrl Pts',(-0.110590156886658,3.0715097374418,100.547349330978));
#24568=CARTESIAN_POINT('Ctrl Pts',(-0.0548178025511639,3.07351782920876,
100.544447166767));
#24569=CARTESIAN_POINT('Ctrl Pts',(0.000958815562382781,3.07400455206058,
100.541545002556));
#24570=CARTESIAN_POINT('Ctrl Pts',(0.0566508376247306,3.07297786073971,
100.538642838345));
#24571=CARTESIAN_POINT('Ctrl Pts',(0.152574884939159,3.07120948560817,100.533644145053));
#24572=CARTESIAN_POINT('Ctrl Pts',(0.248584508306219,3.06494224889118,100.528645451761));
#24573=CARTESIAN_POINT('Ctrl Pts',(0.344223451978229,3.05416313662322,100.52364675847));
#24574=CARTESIAN_POINT('Ctrl Pts',(0.439740601233117,3.04339775135438,100.518654430921));
#24575=CARTESIAN_POINT('Ctrl Pts',(0.534887576440721,3.02813195419978,100.513662103372));
#24576=CARTESIAN_POINT('Ctrl Pts',(0.629208503991605,3.00840471155472,100.508669775823));
#24577=CARTESIAN_POINT('Ctrl Pts',(0.723435077350063,2.98869720310966,100.503682442363));
#24578=CARTESIAN_POINT('Ctrl Pts',(0.816836817974346,2.96453720784374,100.498695108902));
#24579=CARTESIAN_POINT('Ctrl Pts',(0.908964422445171,2.93601531479809,100.493707775442));
#24580=CARTESIAN_POINT('Ctrl Pts',(1.00102824561016,2.90751316788166,100.488723894786));
#24581=CARTESIAN_POINT('Ctrl Pts',(1.09181926773591,2.87465525458155,100.48374001413));
#24582=CARTESIAN_POINT('Ctrl Pts',(1.18090080967825,2.83758269090105,100.478756133474));
#24583=CARTESIAN_POINT('Ctrl Pts',(1.2699445459253,2.80052586060388,100.473774367949));
#24584=CARTESIAN_POINT('Ctrl Pts',(1.35727984015054,2.75925810589058,100.468792602424));
#24585=CARTESIAN_POINT('Ctrl Pts',(1.4424885671648,2.71396923040753,100.463810836898));
#24586=CARTESIAN_POINT('Ctrl Pts',(1.52770834936352,2.66867447903724,100.458828425027));
#24587=CARTESIAN_POINT('Ctrl Pts',(1.61080062163714,2.61935776367916,100.453846013155));
#24588=CARTESIAN_POINT('Ctrl Pts',(1.6913711379829,2.56625523352577,100.448863601284));
#24589=CARTESIAN_POINT('Ctrl Pts',(1.75325071004712,2.52547155743119,100.445037021432));
#24590=CARTESIAN_POINT('Ctrl Pts',(1.81364326519963,2.48245578586724,100.441210441581));
#24591=CARTESIAN_POINT('Ctrl Pts',(1.8723819390353,2.43733217358127,100.43738386173));
#24592=CARTESIAN_POINT('Ctrl Pts',(1.8723819390353,2.43733217358127,101.437247300765));
#24593=CARTESIAN_POINT('Ctrl Pts',(1.94884000716434,2.37859635274812,101.432264386686));
#24594=CARTESIAN_POINT('Ctrl Pts',(2.02257777502802,2.31622396885693,101.427281472606));
#24595=CARTESIAN_POINT('Ctrl Pts',(2.09323711758791,2.2505023038318,101.422298558526));
#24596=CARTESIAN_POINT('Ctrl Pts',(2.16387933174016,2.18479657028054,101.417316852346));
#24597=CARTESIAN_POINT('Ctrl Pts',(2.23144428227298,2.11574346786595,101.412335146166));
#24598=CARTESIAN_POINT('Ctrl Pts',(2.29560854168267,2.04366916925259,101.407353439986));
#24599=CARTESIAN_POINT('Ctrl Pts',(2.35977476377393,1.97159266600227,101.402371581424));
#24600=CARTESIAN_POINT('Ctrl Pts',(2.42053979676236,1.8964951113874,101.397389722861));
#24601=CARTESIAN_POINT('Ctrl Pts',(2.47761928898509,1.8187371742088,101.392407864299));
#24602=CARTESIAN_POINT('Ctrl Pts',(2.53674029629675,1.73819813306707,101.387247823712));
#24603=CARTESIAN_POINT('Ctrl Pts',(2.59190685923281,1.65480522729768,101.382087783126));
#24604=CARTESIAN_POINT('Ctrl Pts',(2.64285179868346,1.5689922307633,101.37692774254));
#24605=CARTESIAN_POINT('Ctrl Pts',(2.69210967599394,1.48602096608979,101.371938578772));
#24606=CARTESIAN_POINT('Ctrl Pts',(2.73742097378704,1.4007877967329,101.366949415003));
#24607=CARTESIAN_POINT('Ctrl Pts',(2.7785916612906,1.3137087309622,101.361960251234));
#24608=CARTESIAN_POINT('Ctrl Pts',(2.82187746759233,1.22215603164039,101.35671477224));
#24609=CARTESIAN_POINT('Ctrl Pts',(2.86058565957799,1.12856323312179,101.351469293245));
#24610=CARTESIAN_POINT('Ctrl Pts',(2.89454931285437,1.03343433533742,101.34622381425));
#24611=CARTESIAN_POINT('Ctrl Pts',(2.92851296613076,0.938305437553028,101.340978335255));
#24612=CARTESIAN_POINT('Ctrl Pts',(2.95773199094319,0.841640994127167,101.335732856261));
#24613=CARTESIAN_POINT('Ctrl Pts',(2.98210140691277,0.743957961775299,101.330487377266));
#24614=CARTESIAN_POINT('Ctrl Pts',(3.00532809919398,0.65085545425668,101.325487867773));
#24615=CARTESIAN_POINT('Ctrl Pts',(3.02423135712574,0.556500655140469,101.32048835828));
#24616=CARTESIAN_POINT('Ctrl Pts',(3.03867997357276,0.461330974689379,101.315488848787));
#24617=CARTESIAN_POINT('Ctrl Pts',(3.05310899056328,0.366290391305736,101.310496121097));
#24618=CARTESIAN_POINT('Ctrl Pts',(3.06309531019677,0.270437553736443,101.305503393407));
#24619=CARTESIAN_POINT('Ctrl Pts',(3.06855806990335,0.174222907882483,101.300510665717));
#24620=CARTESIAN_POINT('Ctrl Pts',(3.07401506653613,0.0781097660547342,
101.295523205229));
#24621=CARTESIAN_POINT('Ctrl Pts',(3.07495796541972,-0.0183639893377553,
101.29053574474));
#24622=CARTESIAN_POINT('Ctrl Pts',(3.07135748041999,-0.114740914534327,
101.285548284252));
#24623=CARTESIAN_POINT('Ctrl Pts',(3.06775957165143,-0.211048879788368,
101.280564392409));
#24624=CARTESIAN_POINT('Ctrl Pts',(3.05962475797039,-0.307259715181775,
101.275580500565));
#24625=CARTESIAN_POINT('Ctrl Pts',(3.04697582811149,-0.402915069095557,
101.270596608721));
#24626=CARTESIAN_POINT('Ctrl Pts',(3.03433150467958,-0.498535587698538,
101.265614531888));
#24627=CARTESIAN_POINT('Ctrl Pts',(3.01717638886501,-0.593600592025961,
101.260632455054));
#24628=CARTESIAN_POINT('Ctrl Pts',(2.99558512143411,-0.687656913178777,
101.25565037822));
#24629=CARTESIAN_POINT('Ctrl Pts',(2.97399582262933,-0.781704658562207,
101.250668755637));
#24630=CARTESIAN_POINT('Ctrl Pts',(2.94797127476999,-0.874743475828466,
101.245687133054));
#24631=CARTESIAN_POINT('Ctrl Pts',(2.91763700124182,-0.966331505739423,
101.240705510471));
#24632=CARTESIAN_POINT('Ctrl Pts',(2.88729721240838,-1.05793618796758,101.235722982141));
#24633=CARTESIAN_POINT('Ctrl Pts',(2.85264627975232,-1.14808914228928,101.230740453811));
#24634=CARTESIAN_POINT('Ctrl Pts',(2.81385889893677,-1.23636578198943,101.225757925482));
#24635=CARTESIAN_POINT('Ctrl Pts',(2.77502971104104,-1.3247375708973,101.220770026721));
#24636=CARTESIAN_POINT('Ctrl Pts',(2.7320553509119,-1.41122860512118,101.215782127959));
#24637=CARTESIAN_POINT('Ctrl Pts',(2.68515768917594,-1.49543653635295,101.210794229198));
#24638=CARTESIAN_POINT('Ctrl Pts',(2.6382323243475,-1.57969421036549,101.205803384017));
#24639=CARTESIAN_POINT('Ctrl Pts',(2.58737927459469,-1.66166572314443,101.200812538836));
#24640=CARTESIAN_POINT('Ctrl Pts',(2.53286404893341,-1.74097730014513,101.195821693655));
#24641=CARTESIAN_POINT('Ctrl Pts',(2.4782607252907,-1.82041704665726,101.190822783141));
#24642=CARTESIAN_POINT('Ctrl Pts',(2.41998367369567,-1.89718792478939,101.185823872628));
#24643=CARTESIAN_POINT('Ctrl Pts',(2.35833896172744,-1.9709489063896,101.180824962115));
#24644=CARTESIAN_POINT('Ctrl Pts',(2.32255054815166,-2.01377153352141,101.177922797904));
#24645=CARTESIAN_POINT('Ctrl Pts',(2.28562777722862,-2.05558034855792,101.175020633693));
#24646=CARTESIAN_POINT('Ctrl Pts',(2.24763596500687,-2.09631458011617,101.172118469482));
#24647=CARTESIAN_POINT('Ctrl Pts',(2.18218810883934,-2.16648675596708,101.167118959989));
#24648=CARTESIAN_POINT('Ctrl Pts',(2.11333593956034,-2.23371428055537,101.162119450496));
#24649=CARTESIAN_POINT('Ctrl Pts',(2.04137491759407,-2.29764894964783,101.157119941003));
#24650=CARTESIAN_POINT('Ctrl Pts',(1.96951151029715,-2.36149689176766,101.152127213313));
#24651=CARTESIAN_POINT('Ctrl Pts',(1.89454795694443,-2.42206056667833,101.147134485623));
#24652=CARTESIAN_POINT('Ctrl Pts',(1.81681806233013,-2.47902690150611,101.142141757933));
#24653=CARTESIAN_POINT('Ctrl Pts',(1.73917017079561,-2.53593313828639,101.137154297445));
#24654=CARTESIAN_POINT('Ctrl Pts',(1.65876209181881,-2.58924932131834,101.132166836956));
#24655=CARTESIAN_POINT('Ctrl Pts',(1.57596158081565,-2.63870182964901,101.127179376468));
#24656=CARTESIAN_POINT('Ctrl Pts',(1.49322031551337,-2.68811895355414,101.122195484625));
#24657=CARTESIAN_POINT('Ctrl Pts',(1.40809039702697,-2.73367767411584,101.117211592781));
#24658=CARTESIAN_POINT('Ctrl Pts',(1.3209686945205,-2.77514755609441,101.112227700937));
#24659=CARTESIAN_POINT('Ctrl Pts',(1.23387871958018,-2.81660233576914,101.107245624104));
#24660=CARTESIAN_POINT('Ctrl Pts',(1.14479879777426,-2.8539710469787,101.10226354727));
#24661=CARTESIAN_POINT('Ctrl Pts',(1.05414968196086,-2.88706956930757,101.097281470436));
#24662=CARTESIAN_POINT('Ctrl Pts',(0.963508831258191,-2.92016507381383,
101.092299847853));
#24663=CARTESIAN_POINT('Ctrl Pts',(0.87129948340515,-2.94899101314185,101.08731822527));
#24664=CARTESIAN_POINT('Ctrl Pts',(0.777960607925135,-2.97341210438727,
101.082336602687));
#24665=CARTESIAN_POINT('Ctrl Pts',(0.684604761793506,-2.99783763581723,
101.077354074357));
#24666=CARTESIAN_POINT('Ctrl Pts',(0.59011940484592,-3.01785661754358,101.072371546027));
#24667=CARTESIAN_POINT('Ctrl Pts',(0.494955790469876,-3.03338441604099,
101.067389017697));
#24668=CARTESIAN_POINT('Ctrl Pts',(0.399689603742445,-3.04892895121674,
101.062401118936));
#24669=CARTESIAN_POINT('Ctrl Pts',(0.303744134041005,-3.05997256807873,
101.057413220175));
#24670=CARTESIAN_POINT('Ctrl Pts',(0.207577665831377,-3.0664823108324,101.052425321414));
#24671=CARTESIAN_POINT('Ctrl Pts',(0.111354390769157,-3.07299589898045,
101.047434476233));
#24672=CARTESIAN_POINT('Ctrl Pts',(0.0149102959240317,-3.07497027126291,
101.042443631052));
#24673=CARTESIAN_POINT('Ctrl Pts',(-0.0812965427013993,-3.07242463245965,
101.03745278587));
#24674=CARTESIAN_POINT('Ctrl Pts',(-0.177658854007724,-3.06987487983979,
101.032453875357));
#24675=CARTESIAN_POINT('Ctrl Pts',(-0.273782706025204,-3.06279056299999,
101.027454964844));
#24676=CARTESIAN_POINT('Ctrl Pts',(-0.369215407999756,-3.05124273575466,
101.022456054331));
#24677=CARTESIAN_POINT('Ctrl Pts',(-0.42461975490707,-3.0445385367381,101.01955389012));
#24678=CARTESIAN_POINT('Ctrl Pts',(-0.479791326678711,-3.03633087595215,
101.016651725909));
#24679=CARTESIAN_POINT('Ctrl Pts',(-0.534643587322911,-3.02664145292013,
101.013749561698));
#24680=CARTESIAN_POINT('Ctrl Pts',(-0.629136654518057,-3.00994964676859,
101.008750052205));
#24681=CARTESIAN_POINT('Ctrl Pts',(-0.723013254539368,-2.98879910906617,
101.003750542712));
#24682=CARTESIAN_POINT('Ctrl Pts',(-0.815820452473183,-2.96324808939894,
100.998751033219));
#24683=CARTESIAN_POINT('Ctrl Pts',(-0.908501758032551,-2.93773172952757,
100.993758305529));
#24684=CARTESIAN_POINT('Ctrl Pts',(-1.00011612495393,-2.90782686665276,
100.988765577839));
#24685=CARTESIAN_POINT('Ctrl Pts',(-1.09021920958482,-2.87364304064584,
100.983772850148));
#24686=CARTESIAN_POINT('Ctrl Pts',(-1.18022723773209,-2.83949527771389,
100.97878538966));
#24687=CARTESIAN_POINT('Ctrl Pts',(-1.26872674485357,-2.80107768048225,
100.973797929172));
#24688=CARTESIAN_POINT('Ctrl Pts',(-1.3552879947946,-2.75854974600162,100.968810468684));
#24689=CARTESIAN_POINT('Ctrl Pts',(-1.44178730813832,-2.71605224125202,
100.96382657684));
#24690=CARTESIAN_POINT('Ctrl Pts',(-1.52635072847931,-2.66945043891615,
100.958842684996));
#24691=CARTESIAN_POINT('Ctrl Pts',(-1.60856889248042,-2.61895176896107,
100.953858793153));
#24692=CARTESIAN_POINT('Ctrl Pts',(-1.69075711466253,-2.56847148937086,
100.948876716319));
#24693=CARTESIAN_POINT('Ctrl Pts',(-1.77060140381673,-2.5140973913475,100.943894639485));
#24694=CARTESIAN_POINT('Ctrl Pts',(-1.84771824160846,-2.4560821544947,100.938912562652));
#24695=CARTESIAN_POINT('Ctrl Pts',(-1.92482804812148,-2.39807220729474,
100.933930940069));
#24696=CARTESIAN_POINT('Ctrl Pts',(-1.99921054702392,-2.33642204535948,
100.928949317485));
#24697=CARTESIAN_POINT('Ctrl Pts',(-2.07051326641702,-2.27142621795011,
100.923967694902));
#24698=CARTESIAN_POINT('Ctrl Pts',(-2.14182894990078,-2.20641857315415,
100.918985166573));
#24699=CARTESIAN_POINT('Ctrl Pts',(-2.21006341741581,-2.13806435053479,
100.914002638243));
#24700=CARTESIAN_POINT('Ctrl Pts',(-2.27489999340274,-2.06669597909712,
100.909020109913));
#24701=CARTESIAN_POINT('Ctrl Pts',(-2.33980645366294,-1.99525068307335,
100.904032211152));
#24702=CARTESIAN_POINT('Ctrl Pts',(-2.40130741504089,-1.92078507772949,
100.899044312391));
#24703=CARTESIAN_POINT('Ctrl Pts',(-2.45912572077757,-1.84366562570609,
100.89405641363));
#24704=CARTESIAN_POINT('Ctrl Pts',(-2.51697818058096,-1.76650061816396,
100.889065568448));
#24705=CARTESIAN_POINT('Ctrl Pts',(-2.571143406811,-1.68667900552759,100.884074723267));
#24706=CARTESIAN_POINT('Ctrl Pts',(-2.62138810809422,-1.60459547448638,
100.879083878086));
#24707=CARTESIAN_POINT('Ctrl Pts',(-2.67171400608364,-1.52237929438601,
100.874084967573));
#24708=CARTESIAN_POINT('Ctrl Pts',(-2.71810651705663,-1.43789428152925,
100.86908605706));
#24709=CARTESIAN_POINT('Ctrl Pts',(-2.76037877221685,-1.35155883478841,
100.864087146546));
#24710=CARTESIAN_POINT('Ctrl Pts',(-2.78492032496541,-1.30143598441692,
100.861184982335));
#24711=CARTESIAN_POINT('Ctrl Pts',(-2.80807405079476,-1.25068982192612,
100.858282818124));
#24712=CARTESIAN_POINT('Ctrl Pts',(-2.82981103644184,-1.19940474737762,
100.855380653913));
#24713=CARTESIAN_POINT('Ctrl Pts',(-2.87129753361498,-1.10152373780138,
100.849841678579));
#24714=CARTESIAN_POINT('Ctrl Pts',(-2.90774489594132,-1.00138651678959,
100.844302703245));
#24715=CARTESIAN_POINT('Ctrl Pts',(-2.93892843199391,-0.899500929192315,
100.838763727911));
#24716=CARTESIAN_POINT('Ctrl Pts',(-2.97002309322088,-0.797905721230475,
100.833240538968));
#24717=CARTESIAN_POINT('Ctrl Pts',(-2.9958837450267,-0.694572335139929,
100.827717350024));
#24718=CARTESIAN_POINT('Ctrl Pts',(-3.01633389163178,-0.590027206316343,
100.82219416108));
#24719=CARTESIAN_POINT('Ctrl Pts',(-3.03668036550995,-0.486012072646383,
100.816698972134));
#24720=CARTESIAN_POINT('Ctrl Pts',(-3.05167093851318,-0.38079770440686,
100.811203783188));
#24721=CARTESIAN_POINT('Ctrl Pts',(-3.0611795685935,-0.27492162305963,100.805708594242));
#24722=CARTESIAN_POINT('Ctrl Pts',(-3.06933072015189,-0.184160706063101,
100.80099791378));
#24723=CARTESIAN_POINT('Ctrl Pts',(-3.07345415884847,-0.0929139253420787,
100.796287233317));
#24724=CARTESIAN_POINT('Ctrl Pts',(-3.0734996196979,-0.00152895940824786,
100.791576552855));
#24725=CARTESIAN_POINT('Origin',(0.,0.,116.208423447177));
#24726=CARTESIAN_POINT('',(1.87238193903529,2.43733217358128,102.437311095123));
#24727=CARTESIAN_POINT('',(1.8723819390353,2.43733217358127,102.354198413529));
#24728=CARTESIAN_POINT('',(1.8723819390353,2.43733217358128,116.208423447177));
#24729=CARTESIAN_POINT('',(-3.0734992979985,0.00207730659809526,101.708423447141));
#24730=CARTESIAN_POINT('Ctrl Pts',(1.8723819390353,2.43733217358127,102.354198413529));
#24731=CARTESIAN_POINT('Ctrl Pts',(1.94890699904715,2.37854488894159,102.349215952023));
#24732=CARTESIAN_POINT('Ctrl Pts',(2.02264391055518,2.31616314582571,102.344233490517));
#24733=CARTESIAN_POINT('Ctrl Pts',(2.09324892654711,2.25049132002534,102.339251029012));
#24734=CARTESIAN_POINT('Ctrl Pts',(2.16392958878789,2.18474913339851,102.334263229294));
#24735=CARTESIAN_POINT('Ctrl Pts',(2.23147133415777,2.11571012581288,102.329275429577));
#24736=CARTESIAN_POINT('Ctrl Pts',(2.29556689235758,2.04371595206177,102.324287629859));
#24737=CARTESIAN_POINT('Ctrl Pts',(2.35969963902613,1.97168000703734,102.319296936203));
#24738=CARTESIAN_POINT('Ctrl Pts',(2.42038194099289,1.89668582278075,102.314306242547));
#24739=CARTESIAN_POINT('Ctrl Pts',(2.47734783506712,1.81910691112102,102.30931554889));
#24740=CARTESIAN_POINT('Ctrl Pts',(2.5344065073427,1.7414016496163,102.30431672708));
#24741=CARTESIAN_POINT('Ctrl Pts',(2.58773644184387,1.66110361976615,102.299317905269));
#24742=CARTESIAN_POINT('Ctrl Pts',(2.6371159008827,1.57861394118753,102.294319083458));
#24743=CARTESIAN_POINT('Ctrl Pts',(2.66790079696583,1.52718696664379,102.291202641663));
#24744=CARTESIAN_POINT('Ctrl Pts',(2.69715117320429,1.47490865119322,102.288086199867));
#24745=CARTESIAN_POINT('Ctrl Pts',(2.72482273064766,1.42188021174284,102.284969758072));
#24746=CARTESIAN_POINT('Ctrl Pts',(2.76921445146489,1.33681005679139,102.279970248579));
#24747=CARTESIAN_POINT('Ctrl Pts',(2.80969643364758,1.24950959633869,102.274970739086));
#24748=CARTESIAN_POINT('Ctrl Pts',(2.84603864801093,1.16037332959187,102.269971229593));
#24749=CARTESIAN_POINT('Ctrl Pts',(2.88233156439122,1.071357975625,102.264978501903));
#24750=CARTESIAN_POINT('Ctrl Pts',(2.91449570921459,0.980512167589046,102.259985774213));
#24751=CARTESIAN_POINT('Ctrl Pts',(2.94234694291599,0.888254871933135,102.254993046523));
#24752=CARTESIAN_POINT('Ctrl Pts',(2.97016879426802,0.796094905398126,102.250005586035));
#24753=CARTESIAN_POINT('Ctrl Pts',(2.99368665346061,0.702526829448201,102.245018125546));
#24754=CARTESIAN_POINT('Ctrl Pts',(3.01276488262564,0.607988496616256,102.240030665058));
#24755=CARTESIAN_POINT('Ctrl Pts',(3.03182946087167,0.513517808171705,102.235046773214));
#24756=CARTESIAN_POINT('Ctrl Pts',(3.04646063755337,0.418078672018671,102.230062881371));
#24757=CARTESIAN_POINT('Ctrl Pts',(3.05657318778474,0.32212202302148,102.225078989527));
#24758=CARTESIAN_POINT('Ctrl Pts',(3.06668205527578,0.226200319059179,102.220096912693));
#24759=CARTESIAN_POINT('Ctrl Pts',(3.07227551993007,0.1297619128116,102.21511483586));
#24760=CARTESIAN_POINT('Ctrl Pts',(3.07331998006636,0.0332648481871961,
102.210132759026));
#24761=CARTESIAN_POINT('Ctrl Pts',(3.07436434497195,-0.0632234181279897,
102.205151136443));
#24762=CARTESIAN_POINT('Ctrl Pts',(3.07086052542035,-0.159769893248088,
102.20016951386));
#24763=CARTESIAN_POINT('Ctrl Pts',(3.06282703587785,-0.255915607761009,
102.195187891277));
#24764=CARTESIAN_POINT('Ctrl Pts',(3.05479208570543,-0.352078803258626,
102.190205362947));
#24765=CARTESIAN_POINT('Ctrl Pts',(3.04222586650856,-0.447840656007861,
102.185222834617));
#24766=CARTESIAN_POINT('Ctrl Pts',(3.02519874309424,-0.542747468700733,
102.180240306287));
#24767=CARTESIAN_POINT('Ctrl Pts',(3.00815326695027,-0.637756576950667,
102.175252407526));
#24768=CARTESIAN_POINT('Ctrl Pts',(2.98663736511165,-0.731908372460368,
102.170264508765));
#24769=CARTESIAN_POINT('Ctrl Pts',(2.96077247436852,-0.824759725630283,
102.165276610004));
#24770=CARTESIAN_POINT('Ctrl Pts',(2.93489230487937,-0.91766592736909,102.160285764823));
#24771=CARTESIAN_POINT('Ctrl Pts',(2.90465816868865,-1.00926974052806,102.155294919642));
#24772=CARTESIAN_POINT('Ctrl Pts',(2.87024062061863,-1.09914559078896,102.15030407446));
#24773=CARTESIAN_POINT('Ctrl Pts',(2.8357674529218,-1.18916668269344,102.145305163947));
#24774=CARTESIAN_POINT('Ctrl Pts',(2.79709755011772,-1.27745383401738,102.140306253434));
#24775=CARTESIAN_POINT('Ctrl Pts',(2.75444856847819,-1.36360380375255,102.135307342921));
#24776=CARTESIAN_POINT('Ctrl Pts',(2.72968830365192,-1.41361897371482,102.13240517871));
#24777=CARTESIAN_POINT('Ctrl Pts',(2.7035877408453,-1.46291429447095,102.129503014499));
#24778=CARTESIAN_POINT('Ctrl Pts',(2.67619614131916,-1.51141538406504,102.126600850288));
#24779=CARTESIAN_POINT('Ctrl Pts',(2.6290090933427,-1.59496739567365,102.121601340795));
#24780=CARTESIAN_POINT('Ctrl Pts',(2.57782261901536,-1.67645424199027,102.116601831302));
#24781=CARTESIAN_POINT('Ctrl Pts',(2.52284238147984,-1.75546819060019,102.111602321809));
#24782=CARTESIAN_POINT('Ctrl Pts',(2.4679367242875,-1.83437495729044,102.106609594119));
#24783=CARTESIAN_POINT('Ctrl Pts',(2.40924778022428,-1.9108151358268,102.101616866429));
#24784=CARTESIAN_POINT('Ctrl Pts',(2.34702672004184,-1.98440616442543,102.096624138739));
#24785=CARTESIAN_POINT('Ctrl Pts',(2.28487130150936,-2.05791955634404,102.091636678251));
#24786=CARTESIAN_POINT('Ctrl Pts',(2.21919145641307,-2.1285894402129,102.086649217762));
#24787=CARTESIAN_POINT('Ctrl Pts',(2.15028060383059,-2.19606365453963,102.081661757274));
#24788=CARTESIAN_POINT('Ctrl Pts',(2.08141905857399,-2.26348958948873,102.076677865431));
#24789=CARTESIAN_POINT('Ctrl Pts',(2.0093314144485,-2.32772409427521,102.071693973587));
#24790=CARTESIAN_POINT('Ctrl Pts',(1.93434951131722,-2.3884501707314,102.066710081743));
#24791=CARTESIAN_POINT('Ctrl Pts',(1.85939491473803,-2.4491541322545,102.061728004909));
#24792=CARTESIAN_POINT('Ctrl Pts',(1.78154849414504,-2.50635192807946,102.056745928076));
#24793=CARTESIAN_POINT('Ctrl Pts',(1.70117615874711,-2.55976599065431,102.051763851242));
#24794=CARTESIAN_POINT('Ctrl Pts',(1.62081115145448,-2.61317518309725,102.046782228659));
#24795=CARTESIAN_POINT('Ctrl Pts',(1.53792105293775,-2.66280108538063,102.041800606076));
#24796=CARTESIAN_POINT('Ctrl Pts',(1.452900923429,-2.70840934068304,102.036818983493));
#24797=CARTESIAN_POINT('Ctrl Pts',(1.36786533576248,-2.75402588836998,102.031836455163));
#24798=CARTESIAN_POINT('Ctrl Pts',(1.28069933480315,-2.79562313087121,102.026853926833));
#24799=CARTESIAN_POINT('Ctrl Pts',(1.19182178858177,-2.83301307343644,102.021871398503));
#24800=CARTESIAN_POINT('Ctrl Pts',(1.10284844546438,-2.8704433168492,102.016883499742));
#24801=CARTESIAN_POINT('Ctrl Pts',(1.01216027941154,-2.90365703641808,102.011895600981));
#24802=CARTESIAN_POINT('Ctrl Pts',(0.920195100562621,-2.93251482978357,
102.00690770222));
#24803=CARTESIAN_POINT('Ctrl Pts',(0.828175596620137,-2.96138966984374,
102.001916857039));
#24804=CARTESIAN_POINT('Ctrl Pts',(0.734878002203351,-2.98590334872931,
101.996926011858));
#24805=CARTESIAN_POINT('Ctrl Pts',(0.640752144606385,-3.0059672219075,101.991935166676));
#24806=CARTESIAN_POINT('Ctrl Pts',(0.546474177246778,-3.02606351881139,
101.986936256163));
#24807=CARTESIAN_POINT('Ctrl Pts',(0.451365706888683,-3.04169558002853,
101.98193734565));
#24808=CARTESIAN_POINT('Ctrl Pts',(0.355883472275826,-3.05282642876415,
101.976938435137));
#24809=CARTESIAN_POINT('Ctrl Pts',(0.300450368732722,-3.0592885470104,101.974036270926));
#24810=CARTESIAN_POINT('Ctrl Pts',(0.244891341822553,-3.06423451062689,
101.971134106715));
#24811=CARTESIAN_POINT('Ctrl Pts',(0.189295602926459,-3.06766514220713,
101.968231942504));
#24812=CARTESIAN_POINT('Ctrl Pts',(0.0935217582459618,-3.07357503355216,
101.963232433011));
#24813=CARTESIAN_POINT('Ctrl Pts',(-0.00269733563999103,-3.07500585446188,
101.958232923518));
#24814=CARTESIAN_POINT('Ctrl Pts',(-0.0989077023084138,-3.07190812304406,
101.953233414025));
#24815=CARTESIAN_POINT('Ctrl Pts',(-0.194987560225561,-3.06881459367923,
101.948240686335));
#24816=CARTESIAN_POINT('Ctrl Pts',(-0.291058279471199,-3.06120473470361,
101.943247958645));
#24817=CARTESIAN_POINT('Ctrl Pts',(-0.386662219864625,-3.04908093984554,
101.938255230955));
#24818=CARTESIAN_POINT('Ctrl Pts',(-0.482165300510678,-3.03696993528546,
101.933267770466));
#24819=CARTESIAN_POINT('Ctrl Pts',(-0.577202148086172,-3.02035451651745,
101.928280309978));
#24820=CARTESIAN_POINT('Ctrl Pts',(-0.671317619773322,-2.99928906632587,
101.92329284949));
#24821=CARTESIAN_POINT('Ctrl Pts',(-0.765365749640313,-2.97823868895634,
101.918308957646));
#24822=CARTESIAN_POINT('Ctrl Pts',(-0.858493387073436,-2.95274470561038,
101.913325065802));
#24823=CARTESIAN_POINT('Ctrl Pts',(-0.950253965723744,-2.92291287085782,
101.908341173959));
#24824=CARTESIAN_POINT('Ctrl Pts',(-1.04198112744394,-2.89309190012063,
101.903359097125));
#24825=CARTESIAN_POINT('Ctrl Pts',(-1.13234180252452,-2.85893635232294,
101.898377020291));
#24826=CARTESIAN_POINT('Ctrl Pts',(-1.22090394960432,-2.82060202719926,
101.893394943458));
#24827=CARTESIAN_POINT('Ctrl Pts',(-1.30945802185682,-2.78227119728279,
101.888413320875));
#24828=CARTESIAN_POINT('Ctrl Pts',(-1.39621348936957,-2.73976252209492,
101.883431698292));
#24829=CARTESIAN_POINT('Ctrl Pts',(-1.48075868428877,-2.69327977917323,
101.878450075708));
#24830=CARTESIAN_POINT('Ctrl Pts',(-1.56531925101342,-2.64678858487022,
101.873467547379));
#24831=CARTESIAN_POINT('Ctrl Pts',(-1.64766836239948,-2.59632209935035,
101.868485019049));
#24832=CARTESIAN_POINT('Ctrl Pts',(-1.72742027654751,-2.54212931185109,
101.863502490719));
#24833=CARTESIAN_POINT('Ctrl Pts',(-1.80725815150581,-2.4878781125134,101.858514591958));
#24834=CARTESIAN_POINT('Ctrl Pts',(-1.88449287681768,-2.42989283993802,
101.853526693197));
#24835=CARTESIAN_POINT('Ctrl Pts',(-1.95876915644562,-2.36846482806001,
101.848538794436));
#24836=CARTESIAN_POINT('Ctrl Pts',(-2.03308931209126,-2.30700052981237,
101.843547949255));
#24837=CARTESIAN_POINT('Ctrl Pts',(-2.10444721774311,-2.24208973812568,
101.838557104073));
#24838=CARTESIAN_POINT('Ctrl Pts',(-2.17252360987847,-2.17406150200968,
101.833566258892));
#24839=CARTESIAN_POINT('Ctrl Pts',(-2.24071001518281,-2.10592333054606,
101.828567348379));
#24840=CARTESIAN_POINT('Ctrl Pts',(-2.30560402268783,-2.03465797948598,
101.823568437866));
#24841=CARTESIAN_POINT('Ctrl Pts',(-2.36692594442134,-1.96062842569038,
101.818569527352));
#24842=CARTESIAN_POINT('Ctrl Pts',(-2.40252695910958,-1.91764987646137,
101.815667363142));
#24843=CARTESIAN_POINT('Ctrl Pts',(-2.436924794165,-1.87374023092859,101.812765198931));
#24844=CARTESIAN_POINT('Ctrl Pts',(-2.47007156829697,-1.82897476677261,
101.80986303472));
#24845=CARTESIAN_POINT('Ctrl Pts',(-2.52743545420021,-1.75150354836611,
101.804840542455));
#24846=CARTESIAN_POINT('Ctrl Pts',(-2.58125253037607,-1.67119415335716,
101.79981805019));
#24847=CARTESIAN_POINT('Ctrl Pts',(-2.63123135768058,-1.58840290617916,
101.794795557926));
#24848=CARTESIAN_POINT('Ctrl Pts',(-2.68114177306052,-1.50572498516071,
101.78977994054));
#24849=CARTESIAN_POINT('Ctrl Pts',(-2.72722415798737,-1.4205723301425,101.784764323154));
#24850=CARTESIAN_POINT('Ctrl Pts',(-2.76922841947647,-1.33333274570298,
101.779748705768));
#24851=CARTESIAN_POINT('Ctrl Pts',(-2.81118629016578,-1.24618951134681,
101.774738627784));
#24852=CARTESIAN_POINT('Ctrl Pts',(-2.84907480323806,-1.15696431708763,
101.7697285498));
#24853=CARTESIAN_POINT('Ctrl Pts',(-2.88268867979694,-1.06607139787659,
101.764718471816));
#24854=CARTESIAN_POINT('Ctrl Pts',(-2.91627301188171,-0.975258367799869,
101.759712797375));
#24855=CARTESIAN_POINT('Ctrl Pts',(-2.94559003048157,-0.882780933297525,
101.754707122933));
#24856=CARTESIAN_POINT('Ctrl Pts',(-2.97048212200563,-0.789074275873267,
101.749701448491));
#24857=CARTESIAN_POINT('Ctrl Pts',(-2.99536106342461,-0.695417122219762,
101.744698418469));
#24858=CARTESIAN_POINT('Ctrl Pts',(-3.01581961525058,-0.600532455110712,
101.739695388448));
#24859=CARTESIAN_POINT('Ctrl Pts',(-3.03174994754577,-0.504870781048189,
101.734692358426));
#24860=CARTESIAN_POINT('Ctrl Pts',(-3.04767925349586,-0.409215270189851,
101.729689650735));
#24861=CARTESIAN_POINT('Ctrl Pts',(-3.0590808394957,-0.312783277793817,
101.724686943044));
#24862=CARTESIAN_POINT('Ctrl Pts',(-3.06589809758779,-0.21603496292859,
101.719684235353));
#24863=CARTESIAN_POINT('Ctrl Pts',(-3.07101317419916,-0.143443455335405,
101.715930639294));
#24864=CARTESIAN_POINT('Ctrl Pts',(-3.07354846896932,-0.0706741086632016,
101.712177043236));
#24865=CARTESIAN_POINT('Ctrl Pts',(-3.07349929799898,0.0020773059017772,
101.708423447177));
#24866=CARTESIAN_POINT('Ctrl Pts',(-3.0734992979985,0.00207730659811786,
101.708423447141));
#24867=CARTESIAN_POINT('Ctrl Pts',(-3.0734250223512,0.111972567151077,101.702753421076));
#24868=CARTESIAN_POINT('Ctrl Pts',(-3.06745263996542,0.221638779434296,
101.697083395011));
#24869=CARTESIAN_POINT('Ctrl Pts',(-3.0556797259961,0.330490033338945,101.691413368946));
#24870=CARTESIAN_POINT('Ctrl Pts',(-3.04384899836201,0.439875826943855,
101.685715498884));
#24871=CARTESIAN_POINT('Ctrl Pts',(-3.0261607520244,0.548438458319583,101.680017628821));
#24872=CARTESIAN_POINT('Ctrl Pts',(-3.00276350587291,0.655601691423871,
101.674319758759));
#24873=CARTESIAN_POINT('Ctrl Pts',(-2.97923000797706,0.763388979912571,
101.668588707666));
#24874=CARTESIAN_POINT('Ctrl Pts',(-2.9499209313853,0.869760348838303,101.662857656573));
#24875=CARTESIAN_POINT('Ctrl Pts',(-2.91503564058411,0.974150637285826,
101.65712660548));
#24876=CARTESIAN_POINT('Ctrl Pts',(-2.90360721621242,1.00834890507326,101.655249112632));
#24877=CARTESIAN_POINT('Ctrl Pts',(-2.8915807188752,1.04233473933062,101.653371619784));
#24878=CARTESIAN_POINT('Ctrl Pts',(-2.87896424539991,1.07608880846747,101.651494126936));
#24879=CARTESIAN_POINT('Ctrl Pts',(-2.84536828312015,1.1659713287875,101.646494617443));
#24880=CARTESIAN_POINT('Ctrl Pts',(-2.80750002023446,1.25443689238554,101.64149510795));
#24881=CARTESIAN_POINT('Ctrl Pts',(-2.76549909601532,1.3410507074449,101.636495598457));
#24882=CARTESIAN_POINT('Ctrl Pts',(-2.72355514578312,1.42754703141422,101.631502870766));
#24883=CARTESIAN_POINT('Ctrl Pts',(-2.67748986552272,1.51219620745576,101.626510143076));
#24884=CARTESIAN_POINT('Ctrl Pts',(-2.62749176748756,1.5945812183094,101.621517415386));
#24885=CARTESIAN_POINT('Ctrl Pts',(-2.57754641618561,1.67687931505313,101.616529954898));
#24886=CARTESIAN_POINT('Ctrl Pts',(-2.52367672164694,1.75691762180815,101.61154249441));
#24887=CARTESIAN_POINT('Ctrl Pts',(-2.46611766424434,1.83430256939853,101.606555033921));
#24888=CARTESIAN_POINT('Ctrl Pts',(-2.40859979169278,1.91163214625,101.601571142078));
#24889=CARTESIAN_POINT('Ctrl Pts',(-2.34739806535233,1.98631178694058,101.596587250234));
#24890=CARTESIAN_POINT('Ctrl Pts',(-2.28279089484515,2.05797667149365,101.59160335839));
#24891=CARTESIAN_POINT('Ctrl Pts',(-2.21820725266931,2.12961545747072,101.586621281557));
#24892=CARTESIAN_POINT('Ctrl Pts',(-2.15022092404982,2.19824134301865,101.581639204723));
#24893=CARTESIAN_POINT('Ctrl Pts',(-2.07915011426144,2.26352315039335,101.576657127889));
#24894=CARTESIAN_POINT('Ctrl Pts',(-2.00808578449351,2.32879900557126,101.571675505306));
#24895=CARTESIAN_POINT('Ctrl Pts',(-1.93393785610523,2.39073109196675,101.566693882723));
#24896=CARTESIAN_POINT('Ctrl Pts',(-1.85706006057578,2.44902637417695,101.56171226014));
#24897=CARTESIAN_POINT('Ctrl Pts',(-1.78016828730857,2.50733225549657,101.55672973181));
#24898=CARTESIAN_POINT('Ctrl Pts',(-1.70054601096407,2.56199975421964,101.55174720348));
#24899=CARTESIAN_POINT('Ctrl Pts',(-1.618577702117,2.61277792248205,101.546764675151));
#24900=CARTESIAN_POINT('Ctrl Pts',(-1.53652104351337,2.66361082212624,101.54177677639));
#24901=CARTESIAN_POINT('Ctrl Pts',(-1.45211367791652,2.71054579056809,101.536788877628));
#24902=CARTESIAN_POINT('Ctrl Pts',(-1.36576635612371,2.75337692851534,101.531800978867));
#24903=CARTESIAN_POINT('Ctrl Pts',(-1.27936802778278,2.79623336740364,101.526810133686));
#24904=CARTESIAN_POINT('Ctrl Pts',(-1.19102786326029,2.83498097260156,101.521819288505));
#24905=CARTESIAN_POINT('Ctrl Pts',(-1.10117639046943,2.86946211110597,101.516828443323));
#24906=CARTESIAN_POINT('Ctrl Pts',(-1.01117971542946,2.90399897200098,101.51182953281));
#24907=CARTESIAN_POINT('Ctrl Pts',(-0.91966727185571,2.93425546127084,101.506830622297));
#24908=CARTESIAN_POINT('Ctrl Pts',(-0.827084463136288,2.96012390633206,
101.501831711784));
#24909=CARTESIAN_POINT('Ctrl Pts',(-0.773334648389712,2.97514207384128,
101.498929547573));
#24910=CARTESIAN_POINT('Ctrl Pts',(-0.719224272794842,2.98868220974381,
101.496027383362));
#24911=CARTESIAN_POINT('Ctrl Pts',(-0.664841586868186,3.00073122994556,
101.493125219151));
#24912=CARTESIAN_POINT('Ctrl Pts',(-0.571149477978079,3.02148964033897,
101.488125284326));
#24913=CARTESIAN_POINT('Ctrl Pts',(-0.476319646934513,3.03789227190172,
101.4831253495));
#24914=CARTESIAN_POINT('Ctrl Pts',(-0.380792933756225,3.04981950147895,
101.478125414674));
#24915=CARTESIAN_POINT('Ctrl Pts',(-0.282177760885511,3.06213234850879,
101.472963827713));
#24916=CARTESIAN_POINT('Ctrl Pts',(-0.182820307436638,3.06967528480989,
101.467802240753));
#24917=CARTESIAN_POINT('Ctrl Pts',(-0.0832206554129855,3.07237311739844,
101.462640653792));
#24918=CARTESIAN_POINT('Ctrl Pts',(0.013007602662867,3.07497962982396,101.457653783737));
#24919=CARTESIAN_POINT('Ctrl Pts',(0.109461444457588,3.07306372397927,101.452666913682));
#24920=CARTESIAN_POINT('Ctrl Pts',(0.205682849278356,3.06660998751272,101.447680043627));
#24921=CARTESIAN_POINT('Ctrl Pts',(0.301840877117753,3.0601605018502,101.442696458213));
#24922=CARTESIAN_POINT('Ctrl Pts',(0.397766335590615,3.04917915399254,101.437712872799));
#24923=CARTESIAN_POINT('Ctrl Pts',(0.493001817994154,3.03370259871571,101.432729287385));
#24924=CARTESIAN_POINT('Ctrl Pts',(0.588200572705452,3.0182320119933,101.427747623897));
#24925=CARTESIAN_POINT('Ctrl Pts',(0.682709447625377,2.99826973462336,101.42276596041));
#24926=CARTESIAN_POINT('Ctrl Pts',(0.77607783639723,2.97390407408393,101.417784296922));
#24927=CARTESIAN_POINT('Ctrl Pts',(0.869435706496847,2.9495411585249,101.412803194658));
#24928=CARTESIAN_POINT('Ctrl Pts',(0.961652921895574,2.92077595894579,101.407822092393));
#24929=CARTESIAN_POINT('Ctrl Pts',(1.05229176659022,2.88774726871422,101.402840990129));
#24930=CARTESIAN_POINT('Ctrl Pts',(1.14298146039165,2.85470004912692,101.397857093427));
#24931=CARTESIAN_POINT('Ctrl Pts',(1.23209060240693,2.81738471281017,101.392873196724));
#24932=CARTESIAN_POINT('Ctrl Pts',(1.31919976902284,2.77598887234983,101.387889300022));
#24933=CARTESIAN_POINT('Ctrl Pts',(1.40633871728044,2.73457887911848,101.382903699382));
#24934=CARTESIAN_POINT('Ctrl Pts',(1.49147593915523,2.68908580625506,101.377918098742));
#24935=CARTESIAN_POINT('Ctrl Pts',(1.57421657404744,2.6397432503928,101.372932498101));
#24936=CARTESIAN_POINT('Ctrl Pts',(1.65704434652747,2.59034872984233,101.367941646919));
#24937=CARTESIAN_POINT('Ctrl Pts',(1.7374701273175,2.53709687465271,101.362950795736));
#24938=CARTESIAN_POINT('Ctrl Pts',(1.81512839634102,2.48026433163816,101.357959944553));
#24939=CARTESIAN_POINT('Ctrl Pts',(1.83438465776063,2.46617204862451,101.356722405573));
#24940=CARTESIAN_POINT('Ctrl Pts',(1.85347092013274,2.45185979957568,101.355484866592));
#24941=CARTESIAN_POINT('Ctrl Pts',(1.8723819390353,2.43733217358127,101.354247327612));
#24942=CARTESIAN_POINT('',(-3.07349961014009,-0.00154805320464923,101.791576552789));
#24943=CARTESIAN_POINT('Ctrl Pts',(-3.07349961014009,-0.00154805320462876,
101.791576552789));
#24944=CARTESIAN_POINT('Ctrl Pts',(-3.07354741658701,0.0933667052458107,
101.786637087407));
#24945=CARTESIAN_POINT('Ctrl Pts',(-3.06919431499038,0.188457621467398,
101.781697622025));
#24946=CARTESIAN_POINT('Ctrl Pts',(-3.06041767066042,0.283277127755595,
101.776758156643));
#24947=CARTESIAN_POINT('Ctrl Pts',(-3.05165206442623,0.377977382681551,
101.771824903463));
#24948=CARTESIAN_POINT('Ctrl Pts',(-3.03847400796433,0.472406461110176,
101.766891650284));
#24949=CARTESIAN_POINT('Ctrl Pts',(-3.02091288803395,0.566116218554452,
101.761958397104));
#24950=CARTESIAN_POINT('Ctrl Pts',(-3.00336870097853,0.659735618685973,
101.757029900692));
#24951=CARTESIAN_POINT('Ctrl Pts',(-2.98144993236622,0.752636635881347,
101.75210140428));
#24952=CARTESIAN_POINT('Ctrl Pts',(-2.95523770915002,0.844376890030603,
101.747172907867));
#24953=CARTESIAN_POINT('Ctrl Pts',(-2.92903900427722,0.936069831281267,
101.742246953212));
#24954=CARTESIAN_POINT('Ctrl Pts',(-2.89855136438474,1.02660276607848,101.737320998557));
#24955=CARTESIAN_POINT('Ctrl Pts',(-2.86390665014472,1.11554513546376,101.732395043902));
#24956=CARTESIAN_POINT('Ctrl Pts',(-2.82926981023108,1.20446728931945,101.727470208857));
#24957=CARTESIAN_POINT('Ctrl Pts',(-2.79047793620527,1.29179917656985,101.722545373812));
#24958=CARTESIAN_POINT('Ctrl Pts',(-2.7477118276345,1.37712815753562,101.717620538767));
#24959=CARTESIAN_POINT('Ctrl Pts',(-2.70494310387406,1.46246235645267,101.712695402564));
#24960=CARTESIAN_POINT('Ctrl Pts',(-2.65819986601987,1.54579300403043,101.707770266361));
#24961=CARTESIAN_POINT('Ctrl Pts',(-2.60770930769473,1.62673120599633,101.702845130157));
#24962=CARTESIAN_POINT('Ctrl Pts',(-2.55716897446221,1.7077491989497,101.697915138626));
#24963=CARTESIAN_POINT('Ctrl Pts',(-2.50287418324929,1.78636965428595,101.692985147095));
#24964=CARTESIAN_POINT('Ctrl Pts',(-2.44509579674928,1.86223220751844,101.688055155565));
#24965=CARTESIAN_POINT('Ctrl Pts',(-2.38728790612099,1.93813349943226,101.683122646568));
#24966=CARTESIAN_POINT('Ctrl Pts',(-2.32599316896728,2.01127374135177,101.678190137571));
#24967=CARTESIAN_POINT('Ctrl Pts',(-2.26152165329072,2.08132699537992,101.673257628575));
#24968=CARTESIAN_POINT('Ctrl Pts',(-2.19694352932644,2.15149608750158,101.66831696332));
#24969=CARTESIAN_POINT('Ctrl Pts',(-2.1291784570876,2.21856768184379,101.663376298065));
#24970=CARTESIAN_POINT('Ctrl Pts',(-2.05857205794463,2.28225400257062,101.65843563281));
#24971=CARTESIAN_POINT('Ctrl Pts',(-2.00516974882912,2.33042239278971,101.654698819485));
#24972=CARTESIAN_POINT('Ctrl Pts',(-1.95014280537916,2.37665504166767,101.650962006159));
#24973=CARTESIAN_POINT('Ctrl Pts',(-1.89365173966774,2.42084393112264,101.647225192834));
#24974=CARTESIAN_POINT('Ctrl Pts',(-1.8180719355148,2.47996456495532,101.642225683341));
#24975=CARTESIAN_POINT('Ctrl Pts',(-1.73958806921937,2.53564619575051,101.637226173848));
#24976=CARTESIAN_POINT('Ctrl Pts',(-1.65854623503812,2.58759089429548,101.632226664355));
#24977=CARTESIAN_POINT('Ctrl Pts',(-1.57761433359045,2.63946513018664,101.627233936665));
#24978=CARTESIAN_POINT('Ctrl Pts',(-1.49413172679109,2.6876122735277,101.622241208975));
#24979=CARTESIAN_POINT('Ctrl Pts',(-1.40847691271125,2.73177507060142,101.617248481285));
#24980=CARTESIAN_POINT('Ctrl Pts',(-1.32291246230095,2.77589127703755,101.612261020797));
#24981=CARTESIAN_POINT('Ctrl Pts',(-1.23518074830207,2.81603129319022,101.607273560308));
#24982=CARTESIAN_POINT('Ctrl Pts',(-1.1456876594634,2.85198212423452,101.60228609982));
#24983=CARTESIAN_POINT('Ctrl Pts',(-1.0562586050218,2.88790723161882,101.597302207976));
#24984=CARTESIAN_POINT('Ctrl Pts',(-0.965071087323808,2.91964894954352,
101.592318316133));
#24985=CARTESIAN_POINT('Ctrl Pts',(-0.872553026345084,2.94704147684013,
101.587334424289));
#24986=CARTESIAN_POINT('Ctrl Pts',(-0.780068658152789,2.97442402845671,
101.582352347455));
#24987=CARTESIAN_POINT('Ctrl Pts',(-0.686255129900967,2.99746041192585,
101.577370270622));
#24988=CARTESIAN_POINT('Ctrl Pts',(-0.591556739153066,3.01603429595265,
101.572388193788));
#24989=CARTESIAN_POINT('Ctrl Pts',(-0.496866982716663,3.03460648646914,
101.567406571205));
#24990=CARTESIAN_POINT('Ctrl Pts',(-0.401292954979292,3.04871690218318,
101.562424948622));
#24991=CARTESIAN_POINT('Ctrl Pts',(-0.305289340276359,3.05830029080102,
101.557443326039));
#24992=CARTESIAN_POINT('Ctrl Pts',(-0.209268270424516,3.06788542184779,
101.552460797709));
#24993=CARTESIAN_POINT('Ctrl Pts',(-0.112817895278018,3.07294184756764,
101.547478269379));
#24994=CARTESIAN_POINT('Ctrl Pts',(-0.0163971433261428,3.07345626025339,
101.542495741049));
#24995=CARTESIAN_POINT('Ctrl Pts',(0.080127535985788,3.0739712274002,101.537507842288));
#24996=CARTESIAN_POINT('Ctrl Pts',(0.176622088674992,3.06993440551272,101.532519943527));
#24997=CARTESIAN_POINT('Ctrl Pts',(0.272628690951967,3.06138462903142,101.527532044766));
#24998=CARTESIAN_POINT('Ctrl Pts',(0.368692005646722,3.05282980207979,101.522541199585));
#24999=CARTESIAN_POINT('Ctrl Pts',(0.464266361288784,3.03975677182418,101.517550354404));
#25000=CARTESIAN_POINT('Ctrl Pts',(0.55890226517057,3.02225586408352,101.512559509222));
#25001=CARTESIAN_POINT('Ctrl Pts',(0.653691103062858,3.004726674434,101.507560598709));
#25002=CARTESIAN_POINT('Ctrl Pts',(0.747538033838945,2.9827554192197,101.502561688196));
#25003=CARTESIAN_POINT('Ctrl Pts',(0.840006960936336,2.95648280150223,101.497562777683));
#25004=CARTESIAN_POINT('Ctrl Pts',(0.893690660642837,2.94122998778069,101.494660613472));
#25005=CARTESIAN_POINT('Ctrl Pts',(0.946910229263901,2.92452832489818,101.491758449261));
#25006=CARTESIAN_POINT('Ctrl Pts',(0.999583567331903,2.9064127273875,101.48885628505));
#25007=CARTESIAN_POINT('Ctrl Pts',(1.09030709198469,2.87521077745148,101.48385765432));
#25008=CARTESIAN_POINT('Ctrl Pts',(1.17972758713199,2.83970206790258,101.478859023589));
#25009=CARTESIAN_POINT('Ctrl Pts',(1.26740695051557,2.80001461992341,101.473860392859));
#25010=CARTESIAN_POINT('Ctrl Pts',(1.35498197212341,2.76037440151613,101.468867710689));
#25011=CARTESIAN_POINT('Ctrl Pts',(1.44081958027821,2.71656549895826,101.463875028519));
#25012=CARTESIAN_POINT('Ctrl Pts',(1.52449792699141,2.66876531763265,101.458882346349));
#25013=CARTESIAN_POINT('Ctrl Pts',(1.60808320110302,2.62101830283586,101.453895217372));
#25014=CARTESIAN_POINT('Ctrl Pts',(1.68951361054567,2.56928905370452,101.448908088394));
#25015=CARTESIAN_POINT('Ctrl Pts',(1.76838958458584,2.51380200634981,101.443920959416));
#25016=CARTESIAN_POINT('Ctrl Pts',(1.80357290875261,2.48905151929853,101.441696406532));
#25017=CARTESIAN_POINT('Ctrl Pts',(1.83824829490535,2.46355396619335,101.439471853649));
#25018=CARTESIAN_POINT('Ctrl Pts',(1.8723819390353,2.43733217358127,101.437247300765));
#25019=CARTESIAN_POINT('Ctrl Pts',(1.87238193903529,2.43733217358128,102.437311095123));
#25020=CARTESIAN_POINT('Ctrl Pts',(1.94849411630402,2.37886206942259,102.432312458847));
#25021=CARTESIAN_POINT('Ctrl Pts',(2.02199547848817,2.31672298377835,102.427313822571));
#25022=CARTESIAN_POINT('Ctrl Pts',(2.09251173940791,2.25117677458704,102.422315186295));
#25023=CARTESIAN_POINT('Ctrl Pts',(2.16293483738044,2.18571716213166,102.417323153995));
#25024=CARTESIAN_POINT('Ctrl Pts',(2.23038035341126,2.11685966892024,102.412331121694));
#25025=CARTESIAN_POINT('Ctrl Pts',(2.2945054394344,2.04490758676424,102.407339089394));
#25026=CARTESIAN_POINT('Ctrl Pts',(2.35856514009273,1.97302887079661,102.402352147237));
#25027=CARTESIAN_POINT('Ctrl Pts',(2.41931085091136,1.89806216492121,102.39736520508));
#25028=CARTESIAN_POINT('Ctrl Pts',(2.47643586927194,1.82034821816687,102.392378262922));
#25029=CARTESIAN_POINT('Ctrl Pts',(2.53352270357738,1.74268621771757,102.387394654185));
#25030=CARTESIAN_POINT('Ctrl Pts',(2.58699339693294,1.66228097941049,102.382411045448));
#25031=CARTESIAN_POINT('Ctrl Pts',(2.63658154685445,1.57950625094888,102.37742743671));
#25032=CARTESIAN_POINT('Ctrl Pts',(2.68615322426235,1.49675901913402,102.372445483461));
#25033=CARTESIAN_POINT('Ctrl Pts',(2.73184469549272,1.41164423737551,102.367463530211));
#25034=CARTESIAN_POINT('Ctrl Pts',(2.7734334696027,1.32456371673375,102.362481576961));
#25035=CARTESIAN_POINT('Ctrl Pts',(2.81501978212943,1.23748835027014,102.357499918586));
#25036=CARTESIAN_POINT('Ctrl Pts',(2.85250369151814,1.14844787255197,102.352518260211));
#25037=CARTESIAN_POINT('Ctrl Pts',(2.88570965194885,1.05786674711386,102.347536601837));
#25038=CARTESIAN_POINT('Ctrl Pts',(2.91892271199686,0.967266254932028,102.342553878356));
#25039=CARTESIAN_POINT('Ctrl Pts',(2.9478558553953,0.875124872908682,102.337571154875));
#25040=CARTESIAN_POINT('Ctrl Pts',(2.97238283161512,0.781883976252037,102.332588431394));
#25041=CARTESIAN_POINT('Ctrl Pts',(2.99693666972406,0.688540962375334,102.327600250846));
#25042=CARTESIAN_POINT('Ctrl Pts',(3.01707459646963,0.594096455340248,102.322612070298));
#25043=CARTESIAN_POINT('Ctrl Pts',(3.03272116605009,0.499003586151244,102.317623889749));
#25044=CARTESIAN_POINT('Ctrl Pts',(3.04837742712118,0.403851816405978,102.31263261952));
#25045=CARTESIAN_POINT('Ctrl Pts',(3.05953674162776,0.308051320573856,102.307641349291));
#25046=CARTESIAN_POINT('Ctrl Pts',(3.06617561067201,0.212059837121748,102.302650079062));
#25047=CARTESIAN_POINT('Ctrl Pts',(3.07282498283358,0.115916488976235,102.297650912323));
#25048=CARTESIAN_POINT('Ctrl Pts',(3.07493962318002,0.0195819881951491,
102.292651745584));
#25049=CARTESIAN_POINT('Ctrl Pts',(3.07254813663131,-0.0764865876048893,
102.287652578845));
#25050=CARTESIAN_POINT('Ctrl Pts',(3.07143961667606,-0.121017021365781,
102.28533532722));
#25051=CARTESIAN_POINT('Ctrl Pts',(3.06936365093371,-0.16549039982456,102.283018075596));
#25052=CARTESIAN_POINT('Ctrl Pts',(3.06632683703467,-0.209861808056952,
102.280700823971));
#25053=CARTESIAN_POINT('Ctrl Pts',(3.05977485978896,-0.305593870265763,
102.275701314478));
#25054=CARTESIAN_POINT('Ctrl Pts',(3.04872388231001,-0.401186951466522,
102.270701804985));
#25055=CARTESIAN_POINT('Ctrl Pts',(3.03318367410548,-0.496184491031267,
102.265702295492));
#25056=CARTESIAN_POINT('Ctrl Pts',(3.01766454609472,-0.591053167036798,
102.260709567802));
#25057=CARTESIAN_POINT('Ctrl Pts',(2.9976683603208,-0.685327477452969,102.255716840112));
#25058=CARTESIAN_POINT('Ctrl Pts',(2.97325679924304,-0.778553951730414,
102.250724112422));
#25059=CARTESIAN_POINT('Ctrl Pts',(2.94887099174687,-0.871682074427455,
102.245736651934));
#25060=CARTESIAN_POINT('Ctrl Pts',(2.92007917959053,-0.963764136147713,
102.240749191445));
#25061=CARTESIAN_POINT('Ctrl Pts',(2.88699427219932,-1.05435588028347,102.235761730957));
#25062=CARTESIAN_POINT('Ctrl Pts',(2.85393303783272,-1.14488280390867,102.230777839114));
#25063=CARTESIAN_POINT('Ctrl Pts',(2.81658496499745,-1.23392111867382,102.22579394727));
#25064=CARTESIAN_POINT('Ctrl Pts',(2.77511279018437,-1.32104172975539,102.220810055426));
#25065=CARTESIAN_POINT('Ctrl Pts',(2.7336557185102,-1.40813061366815,102.215827978592));
#25066=CARTESIAN_POINT('Ctrl Pts',(2.68807771744261,-1.49330278556179,102.210845901759));
#25067=CARTESIAN_POINT('Ctrl Pts',(2.63858926419319,-1.57615003882385,102.205863824925));
#25068=CARTESIAN_POINT('Ctrl Pts',(2.58910532315058,-1.65898973832508,102.200882202342));
#25069=CARTESIAN_POINT('Ctrl Pts',(2.53571186406559,-1.73950456389468,102.195900579759));
#25070=CARTESIAN_POINT('Ctrl Pts',(2.47866429699143,-1.81731272840422,102.190918957176));
#25071=CARTESIAN_POINT('Ctrl Pts',(2.42160635766439,-1.89513503980904,102.185936428846));
#25072=CARTESIAN_POINT('Ctrl Pts',(2.36089325046359,-1.97024935882309,102.180953900516));
#25073=CARTESIAN_POINT('Ctrl Pts',(2.29682185592593,-2.0423054649442,102.175971372186));
#25074=CARTESIAN_POINT('Ctrl Pts',(2.23268140186773,-2.11443923692817,102.170983473425));
#25075=CARTESIAN_POINT('Ctrl Pts',(2.16517572616756,-2.18350788667534,102.165995574664));
#25076=CARTESIAN_POINT('Ctrl Pts',(2.09463975125441,-2.24919687054399,102.161007675903));
#25077=CARTESIAN_POINT('Ctrl Pts',(2.02406210977271,-2.31492465779704,102.156016830722));
#25078=CARTESIAN_POINT('Ctrl Pts',(1.95045093962948,-2.3772685204187,102.151025985541));
#25079=CARTESIAN_POINT('Ctrl Pts',(1.87417389055081,-2.43595453118026,102.146035140359));
#25080=CARTESIAN_POINT('Ctrl Pts',(1.79777357583458,-2.49473538001722,102.141036229846));
#25081=CARTESIAN_POINT('Ctrl Pts',(1.71869913968857,-2.54984632285046,102.136037319333));
#25082=CARTESIAN_POINT('Ctrl Pts',(1.63734674468351,-2.60105707120669,102.13103840882));
#25083=CARTESIAN_POINT('Ctrl Pts',(1.59011685156191,-2.63078794970622,102.128136244609));
#25084=CARTESIAN_POINT('Ctrl Pts',(1.54211964313373,-2.65920512779243,102.125234080398));
#25085=CARTESIAN_POINT('Ctrl Pts',(1.49343596752582,-2.6862708837532,102.122331916187));
#25086=CARTESIAN_POINT('Ctrl Pts',(1.40956941806112,-2.73289660649784,102.117332406694));
#25087=CARTESIAN_POINT('Ctrl Pts',(1.32336995709366,-2.77567293412901,102.112332897201));
#25088=CARTESIAN_POINT('Ctrl Pts',(1.23522586317959,-2.81435948608777,102.107333387708));
#25089=CARTESIAN_POINT('Ctrl Pts',(1.14720133616926,-2.85299355998444,102.102340660018));
#25090=CARTESIAN_POINT('Ctrl Pts',(1.05723781734186,-2.88754870909612,102.097347932328));
#25091=CARTESIAN_POINT('Ctrl Pts',(0.965749257407004,-2.9178297794453,102.092355204638));
#25092=CARTESIAN_POINT('Ctrl Pts',(0.874357215596731,-2.94807890402856,
102.08736774415));
#25093=CARTESIAN_POINT('Ctrl Pts',(0.781443745548439,-2.97406277636264,
102.082380283661));
#25094=CARTESIAN_POINT('Ctrl Pts',(0.687442959990188,-2.99563422779884,
102.077392823173));
#25095=CARTESIAN_POINT('Ctrl Pts',(0.593509434191262,-3.0171902443573,102.07240893133));
#25096=CARTESIAN_POINT('Ctrl Pts',(0.498490566123605,-3.03434001846278,
102.067425039486));
#25097=CARTESIAN_POINT('Ctrl Pts',(0.402834879351311,-3.04698643088183,
102.062441147642));
#25098=CARTESIAN_POINT('Ctrl Pts',(0.307214028011036,-3.05962823779069,
102.057459070809));
#25099=CARTESIAN_POINT('Ctrl Pts',(0.210957253484139,-3.0677698840657,102.052476993975));
#25100=CARTESIAN_POINT('Ctrl Pts',(0.114521550974326,-3.07136566764077,
102.047494917141));
#25101=CARTESIAN_POINT('Ctrl Pts',(0.0180946411787591,-3.07496112336322,
102.042513294558));
#25102=CARTESIAN_POINT('Ctrl Pts',(-0.0785107255000115,-3.07401152427165,
102.037531671975));
#25103=CARTESIAN_POINT('Ctrl Pts',(-0.17483525056192,-3.06852324175017,
102.032550049392));
#25104=CARTESIAN_POINT('Ctrl Pts',(-0.271177289119651,-3.06303396136222,
102.027567521062));
#25105=CARTESIAN_POINT('Ctrl Pts',(-0.367237946406401,-3.05300438367627,
102.022584992732));
#25106=CARTESIAN_POINT('Ctrl Pts',(-0.462561823095072,-3.0384928516972,
102.017602464402));
#25107=CARTESIAN_POINT('Ctrl Pts',(-0.55798844487411,-3.02396567842534,
102.012614565641));
#25108=CARTESIAN_POINT('Ctrl Pts',(-0.652676265943998,-3.00494697261566,
102.00762666688));
#25109=CARTESIAN_POINT('Ctrl Pts',(-0.746179100485398,-2.98154641084099,
102.002638768119));
#25110=CARTESIAN_POINT('Ctrl Pts',(-0.839737168434552,-2.95813202603329,
101.997647922938));
#25111=CARTESIAN_POINT('Ctrl Pts',(-0.932108435924485,-2.93033075773942,
101.992657077757));
#25112=CARTESIAN_POINT('Ctrl Pts',(-1.02286296744176,-2.89830184760598,
101.987666232575));
#25113=CARTESIAN_POINT('Ctrl Pts',(-1.11376416057381,-2.86622117794494,
101.982667322062));
#25114=CARTESIAN_POINT('Ctrl Pts',(-1.20304299444944,-2.82989938980636,
101.977668411549));
#25115=CARTESIAN_POINT('Ctrl Pts',(-1.29029061354383,-2.78954340037948,
101.972669501036));
#25116=CARTESIAN_POINT('Ctrl Pts',(-1.3409430340988,-2.76611435360915,101.969767336825));
#25117=CARTESIAN_POINT('Ctrl Pts',(-1.39091129889851,-2.74132644243857,
101.966865172614));
#25118=CARTESIAN_POINT('Ctrl Pts',(-1.44011974937299,-2.71522694400779,
101.963963008403));
#25119=CARTESIAN_POINT('Ctrl Pts',(-1.52489031967731,-2.67026577686473,
101.95896349891));
#25120=CARTESIAN_POINT('Ctrl Pts',(-1.60770220436728,-2.62125197237255,
101.953963989417));
#25121=CARTESIAN_POINT('Ctrl Pts',(-1.68814237521852,-2.56838034001811,
101.948964479924));
#25122=CARTESIAN_POINT('Ctrl Pts',(-1.76847342948877,-2.51558042769725,
101.943971752234));
#25123=CARTESIAN_POINT('Ctrl Pts',(-1.84643880023916,-2.45893332703264,
101.938979024544));
#25124=CARTESIAN_POINT('Ctrl Pts',(-1.92164941770891,-2.39868000479827,
101.933986296854));
#25125=CARTESIAN_POINT('Ctrl Pts',(-1.99678068987299,-2.3384902483001,101.928998836366));
#25126=CARTESIAN_POINT('Ctrl Pts',(-2.06916264533529,-2.27470210628814,
101.924011375877));
#25127=CARTESIAN_POINT('Ctrl Pts',(-2.13843548681621,-2.20759958296905,
101.919023915389));
#25128=CARTESIAN_POINT('Ctrl Pts',(-2.20765876195982,-2.1405450730739,101.914040023545));
#25129=CARTESIAN_POINT('Ctrl Pts',(-2.27377703121969,-2.07018120087511,
101.909056131702));
#25130=CARTESIAN_POINT('Ctrl Pts',(-2.33646463237743,-1.99683130775972,
101.904072239858));
#25131=CARTESIAN_POINT('Ctrl Pts',(-2.39912940426343,-1.92350812685873,
101.899090163024));
#25132=CARTESIAN_POINT('Ctrl Pts',(-2.45836570549932,-1.84720141901281,
101.894108086191));
#25133=CARTESIAN_POINT('Ctrl Pts',(-2.5138863897926,-1.76826962571196,101.889126009357));
#25134=CARTESIAN_POINT('Ctrl Pts',(-2.56940201187861,-1.68934502917217,
101.884144386774));
#25135=CARTESIAN_POINT('Ctrl Pts',(-2.62120243817953,-1.60779618218701,
101.879162764191));
#25136=CARTESIAN_POINT('Ctrl Pts',(-2.66904294717785,-1.52401180970496,
101.874181141608));
#25137=CARTESIAN_POINT('Ctrl Pts',(-2.71689215442356,-1.44021220374788,
101.869198613278));
#25138=CARTESIAN_POINT('Ctrl Pts',(-2.76077979685105,-1.35417664627861,
101.864216084948));
#25139=CARTESIAN_POINT('Ctrl Pts',(-2.80050686924816,-1.2663188876795,101.859233556618));
#25140=CARTESIAN_POINT('Ctrl Pts',(-2.84027676157447,-1.17836643136481,
101.854245657857));
#25141=CARTESIAN_POINT('Ctrl Pts',(-2.87587694986003,-1.08858825348359,
101.849257759096));
#25142=CARTESIAN_POINT('Ctrl Pts',(-2.90715650340211,-0.997418324840106,
101.844269860335));
#25143=CARTESIAN_POINT('Ctrl Pts',(-2.93845453420578,-0.906194540868447,
101.839279015154));
#25144=CARTESIAN_POINT('Ctrl Pts',(-2.9654267256226,-0.813577790403893,
101.834288169973));
#25145=CARTESIAN_POINT('Ctrl Pts',(-2.98797256925578,-0.720015399401322,
101.829297324791));
#25146=CARTESIAN_POINT('Ctrl Pts',(-3.01055484754163,-0.626301809212099,
101.824298414278));
#25147=CARTESIAN_POINT('Ctrl Pts',(-3.02869641233825,-0.531639957875307,
101.819299503765));
#25148=CARTESIAN_POINT('Ctrl Pts',(-3.04234822215892,-0.43648544663761,
101.814300593252));
#25149=CARTESIAN_POINT('Ctrl Pts',(-3.05027390792034,-0.381242605962414,
101.811398429041));
#25150=CARTESIAN_POINT('Ctrl Pts',(-3.05668729903727,-0.32583379401264,
101.80849626483));
#25151=CARTESIAN_POINT('Ctrl Pts',(-3.06158685878352,-0.270348212725789,
101.805594100619));
#25152=CARTESIAN_POINT('Ctrl Pts',(-3.06947520324294,-0.181015823615497,
101.800921584687));
#25153=CARTESIAN_POINT('Ctrl Pts',(-3.07345438733466,-0.0913332202229314,
101.796249068755));
#25154=CARTESIAN_POINT('Ctrl Pts',(-3.07349961013976,-0.00154805386522649,
101.791576552823));
#25155=CARTESIAN_POINT('Origin',(0.,0.,116.208423447177));
#25156=CARTESIAN_POINT('',(1.87238193903529,2.43733217358128,103.43740200794));
#25157=CARTESIAN_POINT('',(1.87238193903529,2.43733217358128,103.354077375525));
#25158=CARTESIAN_POINT('',(1.8723819390353,2.43733217358128,116.208423447177));
#25159=CARTESIAN_POINT('',(-3.07349905914929,-0.00240487181663789,102.708423447209));
#25160=CARTESIAN_POINT('Ctrl Pts',(1.87238193903529,2.43733217358128,103.354077375525));
#25161=CARTESIAN_POINT('Ctrl Pts',(1.9487790670956,2.37864316749308,103.349092480919));
#25162=CARTESIAN_POINT('Ctrl Pts',(2.02248072686417,2.3163076435992,103.344107586313));
#25163=CARTESIAN_POINT('Ctrl Pts',(2.09312461075592,2.25060694343723,103.339122691707));
#25164=CARTESIAN_POINT('Ctrl Pts',(2.16373572233126,2.18493672240546,103.334140109638));
#25165=CARTESIAN_POINT('Ctrl Pts',(2.2312915552962,2.11590472503888,103.329157527568));
#25166=CARTESIAN_POINT('Ctrl Pts',(2.29546369119003,2.0438318650095,103.324174945498));
#25167=CARTESIAN_POINT('Ctrl Pts',(2.35962357603549,1.97177276434909,103.319193314649));
#25168=CARTESIAN_POINT('Ctrl Pts',(2.42040075586888,1.89667428258958,103.3142116838));
#25169=CARTESIAN_POINT('Ctrl Pts',(2.47750517899769,1.81889261311372,103.30923005295));
#25170=CARTESIAN_POINT('Ctrl Pts',(2.53461428964495,1.74110455879074,103.304248013175));
#25171=CARTESIAN_POINT('Ctrl Pts',(2.58804978543248,1.66063323350006,103.2992659734));
#25172=CARTESIAN_POINT('Ctrl Pts',(2.63756390184625,1.5778653027675,103.294283933625));
#25173=CARTESIAN_POINT('Ctrl Pts',(2.68712858603362,1.49501284280801,103.289296805792));
#25174=CARTESIAN_POINT('Ctrl Pts',(2.73276366546207,1.40985946992048,103.28430967796));
#25175=CARTESIAN_POINT('Ctrl Pts',(2.77426657811826,1.32281790263664,103.279322550127));
#25176=CARTESIAN_POINT('Ctrl Pts',(2.81579029511711,1.23573270365381,103.274332922376));
#25177=CARTESIAN_POINT('Ctrl Pts',(2.85317754883889,1.14675782977441,103.269343294624));
#25178=CARTESIAN_POINT('Ctrl Pts',(2.8862741907344,1.05632549240301,103.264353666873));
#25179=CARTESIAN_POINT('Ctrl Pts',(2.91942798705916,0.965736987869896,103.259355422558));
#25180=CARTESIAN_POINT('Ctrl Pts',(2.94827623441644,0.873686410270901,103.254357178242));
#25181=CARTESIAN_POINT('Ctrl Pts',(2.9727148166892,0.780620822574235,103.249358933927));
#25182=CARTESIAN_POINT('Ctrl Pts',(2.99581857748097,0.692638424410125,103.244633690877));
#25183=CARTESIAN_POINT('Ctrl Pts',(3.01498160827294,0.603749276804136,103.239908447827));
#25184=CARTESIAN_POINT('Ctrl Pts',(3.03015849914792,0.514336193594856,103.235183204777));
#25185=CARTESIAN_POINT('Ctrl Pts',(3.04621629960374,0.419733322681253,103.230183695284));
#25186=CARTESIAN_POINT('Ctrl Pts',(3.05786774372334,0.324211570568872,103.225184185791));
#25187=CARTESIAN_POINT('Ctrl Pts',(3.06501536928885,0.228217080918866,103.220184676298));
#25188=CARTESIAN_POINT('Ctrl Pts',(3.07215329914567,0.132352807184519,103.215191948608));
#25189=CARTESIAN_POINT('Ctrl Pts',(3.07479952016353,0.0360175043912559,
103.210199220918));
#25190=CARTESIAN_POINT('Ctrl Pts',(3.07290776230444,-0.0603335260788791,
103.205206493228));
#25191=CARTESIAN_POINT('Ctrl Pts',(3.07101800020222,-0.156582908640208,
103.20021903274));
#25192=CARTESIAN_POINT('Ctrl Pts',(3.0645997849622,-0.25284754934986,103.195231572251));
#25193=CARTESIAN_POINT('Ctrl Pts',(3.05365880648709,-0.348669103253849,
103.190244111763));
#25194=CARTESIAN_POINT('Ctrl Pts',(3.04272565653778,-0.444422094596621,
103.18526021992));
#25195=CARTESIAN_POINT('Ctrl Pts',(3.02727622630706,-0.539732194514151,
103.180276328076));
#25196=CARTESIAN_POINT('Ctrl Pts',(3.00736819811512,-0.634144124758574,
103.175292436232));
#25197=CARTESIAN_POINT('Ctrl Pts',(2.98746741993402,-0.728521672516159,
103.170310359399));
#25198=CARTESIAN_POINT('Ctrl Pts',(2.96311136040599,-0.822001271416911,
103.165328282565));
#25199=CARTESIAN_POINT('Ctrl Pts',(2.93440900753257,-0.91413676575866,103.160346205731));
#25200=CARTESIAN_POINT('Ctrl Pts',(2.90570927165249,-1.00626385946593,103.155364583148));
#25201=CARTESIAN_POINT('Ctrl Pts',(2.87266416104216,-1.0970466732265,103.150382960565));
#25202=CARTESIAN_POINT('Ctrl Pts',(2.83543253547438,-1.18605420903656,103.145401337982));
#25203=CARTESIAN_POINT('Ctrl Pts',(2.79819414054104,-1.27507792798496,103.140418809652));
#25204=CARTESIAN_POINT('Ctrl Pts',(2.75676788836646,-1.36232532300432,103.135436281322));
#25205=CARTESIAN_POINT('Ctrl Pts',(2.71136035032806,-1.44738636882793,103.130453752993));
#25206=CARTESIAN_POINT('Ctrl Pts',(2.66590386965575,-1.53253909792276,103.125465854232));
#25207=CARTESIAN_POINT('Ctrl Pts',(2.61645774311736,-1.61550038528,103.12047795547));
#25208=CARTESIAN_POINT('Ctrl Pts',(2.56327388343518,-1.69588597744634,103.115490056709));
#25209=CARTESIAN_POINT('Ctrl Pts',(2.51005860731703,-1.77631905448543,103.110499211528));
#25210=CARTESIAN_POINT('Ctrl Pts',(2.45310146076836,-1.85417305267103,103.105508366347));
#25211=CARTESIAN_POINT('Ctrl Pts',(2.39269568836607,-1.92909553751866,103.100517521166));
#25212=CARTESIAN_POINT('Ctrl Pts',(2.33219229871011,-2.00413909899388,103.095518610652));
#25213=CARTESIAN_POINT('Ctrl Pts',(2.26822944612697,-2.07624135943845,103.090519700139));
#25214=CARTESIAN_POINT('Ctrl Pts',(2.20113831793372,-2.14508562890247,103.085520789626));
#25215=CARTESIAN_POINT('Ctrl Pts',(2.16218793652437,-2.1850538128589,103.082618625415));
#25216=CARTESIAN_POINT('Ctrl Pts',(2.12218382895401,-2.223924616875,103.079716461204));
#25217=CARTESIAN_POINT('Ctrl Pts',(2.08119575623365,-2.26164242846544,103.076814296993));
#25218=CARTESIAN_POINT('Ctrl Pts',(2.01058629248019,-2.32661826835245,103.0718147875));
#25219=CARTESIAN_POINT('Ctrl Pts',(1.93680703068045,-2.38839837684193,103.066815278007));
#25220=CARTESIAN_POINT('Ctrl Pts',(1.86017912923882,-2.44665809976472,103.061815768514));
#25221=CARTESIAN_POINT('Ctrl Pts',(1.78365517305878,-2.50483879374341,103.056823040824));
#25222=CARTESIAN_POINT('Ctrl Pts',(1.7042906034489,-2.55950832950711,103.051830313134));
#25223=CARTESIAN_POINT('Ctrl Pts',(1.62244213190147,-2.61038000655671,103.046837585444));
#25224=CARTESIAN_POINT('Ctrl Pts',(1.54068000842812,-2.6611980152695,103.041850124956));
#25225=CARTESIAN_POINT('Ctrl Pts',(1.45643956315767,-2.7082258997491,103.036862664467));
#25226=CARTESIAN_POINT('Ctrl Pts',(1.37010835017788,-2.75121888601631,103.031875203979));
#25227=CARTESIAN_POINT('Ctrl Pts',(1.2838389091994,-2.79418110979668,103.026891312135));
#25228=CARTESIAN_POINT('Ctrl Pts',(1.19548206628228,-2.83311397959143,103.021907420292));
#25229=CARTESIAN_POINT('Ctrl Pts',(1.10545111053773,-2.86781800193299,103.016923528448));
#25230=CARTESIAN_POINT('Ctrl Pts',(1.01545294183751,-2.9025093859291,103.011941451614));
#25231=CARTESIAN_POINT('Ctrl Pts',(0.923782280826692,-2.93297482464625,
103.006959374781));
#25232=CARTESIAN_POINT('Ctrl Pts',(0.830872698153815,-2.95906282621079,
103.001977297947));
#25233=CARTESIAN_POINT('Ctrl Pts',(0.737971586694478,-2.98514844915059,
102.996995675364));
#25234=CARTESIAN_POINT('Ctrl Pts',(0.64383220082838,-3.00685730997497,102.992014052781));
#25235=CARTESIAN_POINT('Ctrl Pts',(0.548902549807335,-3.02408800149979,
102.987032430198));
#25236=CARTESIAN_POINT('Ctrl Pts',(0.453955638903061,-3.04132182586794,
102.982049901868));
#25237=CARTESIAN_POINT('Ctrl Pts',(0.358218609394035,-3.05407578555463,
102.977067373538));
#25238=CARTESIAN_POINT('Ctrl Pts',(0.262147855419645,-3.06229991214102,
102.972084845208));
#25239=CARTESIAN_POINT('Ctrl Pts',(0.165973551331058,-3.07053290312382,
102.967096946447));
#25240=CARTESIAN_POINT('Ctrl Pts',(0.0694652427456439,-3.07422627605857,
102.962109047686));
#25241=CARTESIAN_POINT('Ctrl Pts',(-0.026917607229562,-3.07338212600077,
102.957121148925));
#25242=CARTESIAN_POINT('Ctrl Pts',(-0.123357391876979,-3.07253747729195,
102.952130303744));
#25243=CARTESIAN_POINT('Ctrl Pts',(-0.219671132276306,-3.06714999302605,
102.947139458563));
#25244=CARTESIAN_POINT('Ctrl Pts',(-0.315403551633273,-3.05727376098659,
102.942148613381));
#25245=CARTESIAN_POINT('Ctrl Pts',(-0.411290676997528,-3.04738156870675,
102.937149702868));
#25246=CARTESIAN_POINT('Ctrl Pts',(-0.506594171739937,-3.03298620967511,
102.932150792355));
#25247=CARTESIAN_POINT('Ctrl Pts',(-0.600868083321939,-3.01419305892058,
102.927151881842));
#25248=CARTESIAN_POINT('Ctrl Pts',(-0.655599683637761,-3.00328251963658,
102.924249717631));
#25249=CARTESIAN_POINT('Ctrl Pts',(-0.709984512979015,-2.99089065275652,
102.92134755342));
#25250=CARTESIAN_POINT('Ctrl Pts',(-0.763937942530679,-2.97704569497379,
102.918445389209));
#25251=CARTESIAN_POINT('Ctrl Pts',(-0.856882608515816,-2.95319521897278,
102.913445879716));
#25252=CARTESIAN_POINT('Ctrl Pts',(-0.948872521153678,-2.92494601987692,
102.908446370223));
#25253=CARTESIAN_POINT('Ctrl Pts',(-1.03946050783718,-2.89239072440894,
102.90344686073));
#25254=CARTESIAN_POINT('Ctrl Pts',(-1.12992561249208,-2.8598795899925,102.89845413304));
#25255=CARTESIAN_POINT('Ctrl Pts',(-1.21899216114037,-2.82307411537473,
102.89346140535));
#25256=CARTESIAN_POINT('Ctrl Pts',(-1.30622545948642,-2.78211741286911,
102.88846867766));
#25257=CARTESIAN_POINT('Ctrl Pts',(-1.39336672890185,-2.74120391865212,
102.883481217171));
#25258=CARTESIAN_POINT('Ctrl Pts',(-1.47867819752179,-2.69614808817625,
102.878493756683));
#25259=CARTESIAN_POINT('Ctrl Pts',(-1.5617435463928,-2.64714173124531,102.873506296195));
#25260=CARTESIAN_POINT('Ctrl Pts',(-1.64474946006473,-2.59817043950848,
102.868522404351));
#25261=CARTESIAN_POINT('Ctrl Pts',(-1.72551207194326,-2.545254463062,102.863538512507));
#25262=CARTESIAN_POINT('Ctrl Pts',(-1.80363903254509,-2.48863185109405,
102.858554620664));
#25263=CARTESIAN_POINT('Ctrl Pts',(-1.88173754124283,-2.43202985967902,
102.85357254383));
#25264=CARTESIAN_POINT('Ctrl Pts',(-1.95720195069231,-2.37172417211283,
102.848590466996));
#25265=CARTESIAN_POINT('Ctrl Pts',(-2.02966913246221,-2.30799598412347,
102.843608390163));
#25266=CARTESIAN_POINT('Ctrl Pts',(-2.10212970689473,-2.24427360667661,
102.83862676758));
#25267=CARTESIAN_POINT('Ctrl Pts',(-2.1715932674645,-2.17712963924436,102.833645144997));
#25268=CARTESIAN_POINT('Ctrl Pts',(-2.23773083527129,-2.10688465723115,
102.828663522413));
#25269=CARTESIAN_POINT('Ctrl Pts',(-2.30388042805295,-2.03662690344283,
102.823680994084));
#25270=CARTESIAN_POINT('Ctrl Pts',(-2.3667025262089,-1.96326733494541,102.818698465754));
#25271=CARTESIAN_POINT('Ctrl Pts',(-2.42590673211331,-1.88716156623838,
102.813715937424));
#25272=CARTESIAN_POINT('Ctrl Pts',(-2.48517475142643,-1.81097376672883,
102.808728038663));
#25273=CARTESIAN_POINT('Ctrl Pts',(-2.54081682341287,-1.73203420469134,
102.803740139902));
#25274=CARTESIAN_POINT('Ctrl Pts',(-2.59258454998316,-1.65072941489168,
102.798752241141));
#25275=CARTESIAN_POINT('Ctrl Pts',(-2.64438285646005,-1.56937659723677,
102.79376139596));
#25276=CARTESIAN_POINT('Ctrl Pts',(-2.69230204253118,-1.48565615061415,
102.788770550778));
#25277=CARTESIAN_POINT('Ctrl Pts',(-2.73613960045076,-1.39997940586465,
102.783779705597));
#25278=CARTESIAN_POINT('Ctrl Pts',(-2.78004800097105,-1.31416420533189,
102.778780795084));
#25279=CARTESIAN_POINT('Ctrl Pts',(-2.8198614213579,-1.22638679349449,102.773781884571));
#25280=CARTESIAN_POINT('Ctrl Pts',(-2.85542544981684,-1.13707860350034,
102.768782974058));
#25281=CARTESIAN_POINT('Ctrl Pts',(-2.87607247886867,-1.08522989925403,
102.765880809847));
#25282=CARTESIAN_POINT('Ctrl Pts',(-2.89528818176262,-1.03286555270384,
102.762978645636));
#25283=CARTESIAN_POINT('Ctrl Pts',(-2.91305016692883,-0.98007192335866,
102.760076481425));
#25284=CARTESIAN_POINT('Ctrl Pts',(-2.94920738770469,-0.872602465754107,
102.75416868502));
#25285=CARTESIAN_POINT('Ctrl Pts',(-2.97944169451475,-0.763046477913077,
102.748260888615));
#25286=CARTESIAN_POINT('Ctrl Pts',(-3.0035458119629,-0.652008286327827,
102.742353092211));
#25287=CARTESIAN_POINT('Ctrl Pts',(-3.02740835185899,-0.542082947538994,
102.736504505233));
#25288=CARTESIAN_POINT('Ctrl Pts',(-3.04526290787279,-0.430705059004667,
102.730655918256));
#25289=CARTESIAN_POINT('Ctrl Pts',(-3.05695463632165,-0.318481712931148,
102.724807331279));
#25290=CARTESIAN_POINT('Ctrl Pts',(-3.0678721407958,-0.213689774919587,
102.719346036589));
#25291=CARTESIAN_POINT('Ctrl Pts',(-3.0734163099308,-0.108160880676264,
102.713884741899));
#25292=CARTESIAN_POINT('Ctrl Pts',(-3.07349905914929,-0.00240487181666147,
102.708423447209));
#25293=CARTESIAN_POINT('Ctrl Pts',(-3.07349905914978,-0.00240487119184143,
102.708423447177));
#25294=CARTESIAN_POINT('Ctrl Pts',(-3.07357440903969,0.0938945965503393,
102.703450493134));
#25295=CARTESIAN_POINT('Ctrl Pts',(-3.06911954638383,0.190252789663529,
102.698477539092));
#25296=CARTESIAN_POINT('Ctrl Pts',(-3.06014462176969,0.28621171159479,102.693504585049));
#25297=CARTESIAN_POINT('Ctrl Pts',(-3.05117154752427,0.382150849584176,
102.688532656285));
#25298=CARTESIAN_POINT('Ctrl Pts',(-3.03768030403397,0.477690441648064,
102.683560727521));
#25299=CARTESIAN_POINT('Ctrl Pts',(-3.01973301736177,0.572376409240639,
102.678588798757));
#25300=CARTESIAN_POINT('Ctrl Pts',(-3.00178449415828,0.667068900502399,
102.673616527437));
#25301=CARTESIAN_POINT('Ctrl Pts',(-2.97937940044342,0.760907217840844,
102.668644256118));
#25302=CARTESIAN_POINT('Ctrl Pts',(-2.95263100332805,0.85344736696881,102.663671984798));
#25303=CARTESIAN_POINT('Ctrl Pts',(-2.92485280817885,0.949550259060835,
102.658508283868));
#25304=CARTESIAN_POINT('Ctrl Pts',(-2.89239026140684,1.044252510288,102.653344582938));
#25305=CARTESIAN_POINT('Ctrl Pts',(-2.85542656316374,1.13707580766585,102.648180882009));
#25306=CARTESIAN_POINT('Ctrl Pts',(-2.81977708586454,1.22659883133477,102.643200773204));
#25307=CARTESIAN_POINT('Ctrl Pts',(-2.77994134730074,1.31437386440563,102.638220664399));
#25308=CARTESIAN_POINT('Ctrl Pts',(-2.7361315529654,1.39999513387268,102.633240555594));
#25309=CARTESIAN_POINT('Ctrl Pts',(-2.69228901873091,1.48568038975574,102.628256725059));
#25310=CARTESIAN_POINT('Ctrl Pts',(-2.6444667369319,1.56920829804548,102.623272894523));
#25311=CARTESIAN_POINT('Ctrl Pts',(-2.59292101568691,1.65020085335366,102.618289063988));
#25312=CARTESIAN_POINT('Ctrl Pts',(-2.54129576608687,1.73131836965841,102.613297544049));
#25313=CARTESIAN_POINT('Ctrl Pts',(-2.48593587132566,1.80989237281012,102.60830602411));
#25314=CARTESIAN_POINT('Ctrl Pts',(-2.42713849798024,1.88557708981155,102.603314504171));
#25315=CARTESIAN_POINT('Ctrl Pts',(-2.42082891055332,1.89369886994614,102.602778860661));
#25316=CARTESIAN_POINT('Ctrl Pts',(-2.41447977355874,1.90178741316457,102.602243217151));
#25317=CARTESIAN_POINT('Ctrl Pts',(-2.40809147900626,1.909842317768,102.60170757364));
#25318=CARTESIAN_POINT('Ctrl Pts',(-2.34846536825855,1.98502398479989,102.596708064147));
#25319=CARTESIAN_POINT('Ctrl Pts',(-2.28521034726891,2.05754269684241,102.591708554654));
#25320=CARTESIAN_POINT('Ctrl Pts',(-2.21859308199756,2.12702773524761,102.586709045161));
#25321=CARTESIAN_POINT('Ctrl Pts',(-2.15206618262348,2.19641851763949,102.581716317471));
#25322=CARTESIAN_POINT('Ctrl Pts',(-2.0821864045681,2.26278349084756,102.576723589781));
#25323=CARTESIAN_POINT('Ctrl Pts',(-2.00926144500736,2.32578388841417,102.571730862091));
#25324=CARTESIAN_POINT('Ctrl Pts',(-1.93641341944093,2.38871782214924,102.566743401603));
#25325=CARTESIAN_POINT('Ctrl Pts',(-1.86052692920946,2.4482939510788,102.561755941115));
#25326=CARTESIAN_POINT('Ctrl Pts',(-1.78194666857239,2.50421011905227,102.556768480626));
#25327=CARTESIAN_POINT('Ctrl Pts',(-1.7034226339486,2.56008627770052,102.551784588783));
#25328=CARTESIAN_POINT('Ctrl Pts',(-1.62220901723995,2.61230742764789,102.546800696939));
#25329=CARTESIAN_POINT('Ctrl Pts',(-1.53868298702377,2.66061213171774,102.541816805095));
#25330=CARTESIAN_POINT('Ctrl Pts',(-1.45518737491906,2.70889924441075,102.536834728262));
#25331=CARTESIAN_POINT('Ctrl Pts',(-1.36938140211987,2.75327252554234,102.531852651428));
#25332=CARTESIAN_POINT('Ctrl Pts',(-1.2816697484747,2.79351479427706,102.526870574594));
#25333=CARTESIAN_POINT('Ctrl Pts',(-1.19396609211161,2.83375339384399,102.521888952011));
#25334=CARTESIAN_POINT('Ctrl Pts',(-1.10435749940877,2.86986154698673,102.516907329428));
#25335=CARTESIAN_POINT('Ctrl Pts',(-1.01327071436459,2.90166929704456,102.511925706845));
#25336=CARTESIAN_POINT('Ctrl Pts',(-0.922167368138048,2.93348283031177,
102.506943178515));
#25337=CARTESIAN_POINT('Ctrl Pts',(-0.829585710238195,2.96099426297923,
102.501960650185));
#25338=CARTESIAN_POINT('Ctrl Pts',(-0.735968779922514,2.98408314310767,
102.496978121856));
#25339=CARTESIAN_POINT('Ctrl Pts',(-0.642250944353016,3.0071969096461,102.491990223095));
#25340=CARTESIAN_POINT('Ctrl Pts',(-0.547496035532473,3.02587850176356,
102.487002324334));
#25341=CARTESIAN_POINT('Ctrl Pts',(-0.452158234261135,3.04005841739758,
102.482014425572));
#25342=CARTESIAN_POINT('Ctrl Pts',(-0.356764115641836,3.05424670930241,
102.477023580391));
#25343=CARTESIAN_POINT('Ctrl Pts',(-0.260786855511279,3.06392798578358,
102.47203273521));
#25344=CARTESIAN_POINT('Ctrl Pts',(-0.164684598476815,3.06908475494316,
102.467041890028));
#25345=CARTESIAN_POINT('Ctrl Pts',(-0.0684270377681817,3.07424985757193,
102.462042979515));
#25346=CARTESIAN_POINT('Ctrl Pts',(0.0279554845327262,3.07487585014498,
102.457044069002));
#25347=CARTESIAN_POINT('Ctrl Pts',(0.12400604513015,3.07099735440641,102.452045158489));
#25348=CARTESIAN_POINT('Ctrl Pts',(0.179769095633911,3.0687456574626,102.449142994278));
#25349=CARTESIAN_POINT('Ctrl Pts',(0.235420357734847,3.06497669821165,102.446240830067));
#25350=CARTESIAN_POINT('Ctrl Pts',(0.290871837190732,3.05970518585195,102.443338665856));
#25351=CARTESIAN_POINT('Ctrl Pts',(0.38638965175104,3.05062475472607,102.43833954977));
#25352=CARTESIAN_POINT('Ctrl Pts',(0.481649606642594,3.03705127955959,102.433340433685));
#25353=CARTESIAN_POINT('Ctrl Pts',(0.576195666898044,3.01900659215046,102.428341317599));
#25354=CARTESIAN_POINT('Ctrl Pts',(0.670619518355395,3.00098522902955,102.423348663294));
#25355=CARTESIAN_POINT('Ctrl Pts',(0.764330881220847,2.97850421807133,102.41835600899));
#25356=CARTESIAN_POINT('Ctrl Pts',(0.856878093999578,2.95163720365895,102.413363354686));
#25357=CARTESIAN_POINT('Ctrl Pts',(0.949320810009901,2.92480052528911,102.408376337679));
#25358=CARTESIAN_POINT('Ctrl Pts',(1.04060157080027,2.89358781392061,102.403389320673));
#25359=CARTESIAN_POINT('Ctrl Pts',(1.13027937671876,2.8581236468292,102.398402303667));
#25360=CARTESIAN_POINT('Ctrl Pts',(1.21989649384948,2.82268347984894,102.393418661588));
#25361=CARTESIAN_POINT('Ctrl Pts',(1.30791240494778,2.78299773560621,102.388435019508));
#25362=CARTESIAN_POINT('Ctrl Pts',(1.39390252845336,2.73924040404841,102.383451377429));
#25363=CARTESIAN_POINT('Ctrl Pts',(1.47987428090962,2.69549242086766,102.378468800061));
#25364=CARTESIAN_POINT('Ctrl Pts',(1.56382071038342,2.64767476874144,102.373486222694));
#25365=CARTESIAN_POINT('Ctrl Pts',(1.64533919289062,2.59600870382556,102.368503645327));
#25366=CARTESIAN_POINT('Ctrl Pts',(1.72335375591205,2.54656340806587,102.363735234727));
#25367=CARTESIAN_POINT('Ctrl Pts',(1.79914446256703,2.49359390502932,102.358966824128));
#25368=CARTESIAN_POINT('Ctrl Pts',(1.8723819390353,2.43733217358127,102.354198413529));
#25369=CARTESIAN_POINT('',(-3.07349876002173,0.00276082323149203,102.791576552849));
#25370=CARTESIAN_POINT('Ctrl Pts',(-3.07349876002127,0.00276082373854232,
102.791576552823));
#25371=CARTESIAN_POINT('Ctrl Pts',(-3.0733818456602,0.132916233066199,102.784832988938));
#25372=CARTESIAN_POINT('Ctrl Pts',(-3.06499365801856,0.262711138894001,
102.778089425052));
#25373=CARTESIAN_POINT('Ctrl Pts',(-3.04849240550272,0.391275227419569,
102.771345861166));
#25374=CARTESIAN_POINT('Ctrl Pts',(-3.03581851156285,0.490019708839072,
102.766166423219));
#25375=CARTESIAN_POINT('Ctrl Pts',(-3.01835961128476,0.588038888602218,
102.760986985271));
#25376=CARTESIAN_POINT('Ctrl Pts',(-2.99620562000435,0.684948270057185,
102.755807547324));
#25377=CARTESIAN_POINT('Ctrl Pts',(-2.97482123605449,0.778491117264577,
102.750808037831));
#25378=CARTESIAN_POINT('Ctrl Pts',(-2.94901442045459,0.871195861184662,
102.745808528338));
#25379=CARTESIAN_POINT('Ctrl Pts',(-2.91886594287446,0.962613036233973,
102.740809018845));
#25380=CARTESIAN_POINT('Ctrl Pts',(-2.88875836151275,1.05390620446576,102.735816291154));
#25381=CARTESIAN_POINT('Ctrl Pts',(-2.85432095934281,1.14391486172565,102.730823563464));
#25382=CARTESIAN_POINT('Ctrl Pts',(-2.81568530393745,1.23220068137891,102.725830835774));
#25383=CARTESIAN_POINT('Ctrl Pts',(-2.77709040817466,1.32039336171788,102.720843375286));
#25384=CARTESIAN_POINT('Ctrl Pts',(-2.7343062389121,1.40686641762785,102.715855914798));
#25385=CARTESIAN_POINT('Ctrl Pts',(-2.68751353008668,1.49119860367459,102.710868454309));
#25386=CARTESIAN_POINT('Ctrl Pts',(-2.64075430253822,1.57547044807092,102.705884562466));
#25387=CARTESIAN_POINT('Ctrl Pts',(-2.58999244964522,1.65760408509986,102.700900670622));
#25388=CARTESIAN_POINT('Ctrl Pts',(-2.53545556238873,1.73720100769947,102.695916778778));
#25389=CARTESIAN_POINT('Ctrl Pts',(-2.48093853611586,1.81676894307126,102.690934701945));
#25390=CARTESIAN_POINT('Ctrl Pts',(-2.42264945486254,1.89380163777317,102.685952625111));
#25391=CARTESIAN_POINT('Ctrl Pts',(-2.3608598137594,1.96792865464578,102.680970548277));
#25392=CARTESIAN_POINT('Ctrl Pts',(-2.29907580644797,2.04204891284224,102.675988925694));
#25393=CARTESIAN_POINT('Ctrl Pts',(-2.23379215506017,2.11326368287658,102.671007303111));
#25394=CARTESIAN_POINT('Ctrl Pts',(-2.16532062365469,2.18123562385535,102.666025680528));
#25395=CARTESIAN_POINT('Ctrl Pts',(-2.09683664291834,2.24921992333066,102.661043152198));
#25396=CARTESIAN_POINT('Ctrl Pts',(-2.02516394260194,2.31395991357074,102.656060623868));
#25397=CARTESIAN_POINT('Ctrl Pts',(-1.9506503338181,2.37515589492044,102.651078095538));
#25398=CARTESIAN_POINT('Ctrl Pts',(-1.87605641034575,2.43641783651903,102.646090196777));
#25399=CARTESIAN_POINT('Ctrl Pts',(-1.79861580503093,2.4941278640542,102.641102298016));
#25400=CARTESIAN_POINT('Ctrl Pts',(-1.71870834904133,2.54802744509073,102.636114399255));
#25401=CARTESIAN_POINT('Ctrl Pts',(-1.63875369062066,2.60195886534962,102.631123554074));
#25402=CARTESIAN_POINT('Ctrl Pts',(-1.55632965489344,2.65207512928547,102.626132708893));
#25403=CARTESIAN_POINT('Ctrl Pts',(-1.47184207391802,2.69816292307279,102.621141863711));
#25404=CARTESIAN_POINT('Ctrl Pts',(-1.38721795887821,2.74432519589871,102.616142953198));
#25405=CARTESIAN_POINT('Ctrl Pts',(-1.30052403441139,2.78644580762637,102.611144042685));
#25406=CARTESIAN_POINT('Ctrl Pts',(-1.21218749966317,2.82435899199453,102.606145132172));
#25407=CARTESIAN_POINT('Ctrl Pts',(-1.16090289895004,2.84636984546106,102.603242967961));
#25408=CARTESIAN_POINT('Ctrl Pts',(-1.10906498743717,2.86696350849769,102.60034080375));
#25409=CARTESIAN_POINT('Ctrl Pts',(-1.05675950233097,2.88611531374496,102.597438639539));
#25410=CARTESIAN_POINT('Ctrl Pts',(-0.96665372253602,2.91910780665049,102.592439130046));
#25411=CARTESIAN_POINT('Ctrl Pts',(-0.874843137497201,2.94793449136314,
102.587439620553));
#25412=CARTESIAN_POINT('Ctrl Pts',(-0.781748730651191,2.97241840462026,
102.58244011106));
#25413=CARTESIAN_POINT('Ctrl Pts',(-0.688780605776904,2.99686910560452,
102.57744738337));
#25414=CARTESIAN_POINT('Ctrl Pts',(-0.594532541098022,3.01698863229479,
102.57245465568));
#25415=CARTESIAN_POINT('Ctrl Pts',(-0.499443833784544,3.0326486949356,102.56746192799));
#25416=CARTESIAN_POINT('Ctrl Pts',(-0.40445544266044,3.04829223660506,102.562474467502));
#25417=CARTESIAN_POINT('Ctrl Pts',(-0.308628602744227,3.05948559577763,
102.557487007013));
#25418=CARTESIAN_POINT('Ctrl Pts',(-0.212415052330399,3.066151022951,102.552499546525));
#25419=CARTESIAN_POINT('Ctrl Pts',(-0.116270344960902,3.07281168085543,
102.547515654681));
#25420=CARTESIAN_POINT('Ctrl Pts',(-0.019739913818218,3.07495081716137,
102.542531762838));
#25421=CARTESIAN_POINT('Ctrl Pts',(0.0767180641836116,3.07254236563598,
102.537547870994));
#25422=CARTESIAN_POINT('Ctrl Pts',(0.173140914578841,3.07013479120897,102.53256579416));
#25423=CARTESIAN_POINT('Ctrl Pts',(0.269490925881531,3.06318293042476,102.527583717327));
#25424=CARTESIAN_POINT('Ctrl Pts',(0.365309562312508,3.05171282621466,102.522601640493));
#25425=CARTESIAN_POINT('Ctrl Pts',(0.461119462291404,3.0402437678138,102.51762001791));
#25426=CARTESIAN_POINT('Ctrl Pts',(0.556397647895687,3.02425733739534,102.512638395327));
#25427=CARTESIAN_POINT('Ctrl Pts',(0.650691419758013,3.00383137447049,102.507656772744));
#25428=CARTESIAN_POINT('Ctrl Pts',(0.745002335889377,2.98340169774571,102.502674244414));
#25429=CARTESIAN_POINT('Ctrl Pts',(0.838328053816558,2.95853097840997,102.497691716084));
#25430=CARTESIAN_POINT('Ctrl Pts',(0.930227821477748,2.92934778579614,102.492709187754));
#25431=CARTESIAN_POINT('Ctrl Pts',(1.0222266435445,2.90013313800163,102.487721288993));
#25432=CARTESIAN_POINT('Ctrl Pts',(1.11279602787013,2.86659687028279,102.482733390232));
#25433=CARTESIAN_POINT('Ctrl Pts',(1.20151231977035,2.8289168237048,102.477745491471));
#25434=CARTESIAN_POINT('Ctrl Pts',(1.29028101760189,2.79121451900611,102.47275464629));
#25435=CARTESIAN_POINT('Ctrl Pts',(1.37719404807226,2.7493637518578,102.467763801109));
#25436=CARTESIAN_POINT('Ctrl Pts',(1.4618515292926,2.70358879201421,102.462772955927));
#25437=CARTESIAN_POINT('Ctrl Pts',(1.54664581914047,2.65773985867956,102.457774045414));
#25438=CARTESIAN_POINT('Ctrl Pts',(1.62917690581338,2.60795429647158,102.452775134901));
#25439=CARTESIAN_POINT('Ctrl Pts',(1.70907315660856,2.55450018503817,102.447776224388));
#25440=CARTESIAN_POINT('Ctrl Pts',(1.75545767160221,2.52346690114089,102.444874060177));
#25441=CARTESIAN_POINT('Ctrl Pts',(1.80095470912527,2.49119791287163,102.441971895966));
#25442=CARTESIAN_POINT('Ctrl Pts',(1.84549689863107,2.4577517057553,102.439069731755));
#25443=CARTESIAN_POINT('Ctrl Pts',(1.854494037828,2.45099585957051,102.438483519544));
#25444=CARTESIAN_POINT('Ctrl Pts',(1.86345592697286,2.44418922160882,102.437897307334));
#25445=CARTESIAN_POINT('Ctrl Pts',(1.87238193903529,2.43733217358128,102.437311095123));
#25446=CARTESIAN_POINT('Ctrl Pts',(1.87238193903529,2.43733217358128,103.43740200794));
#25447=CARTESIAN_POINT('Ctrl Pts',(1.94890807686061,2.37854406095496,103.432413164395));
#25448=CARTESIAN_POINT('Ctrl Pts',(2.02261042630876,2.31618872145143,103.42742432085));
#25449=CARTESIAN_POINT('Ctrl Pts',(2.09315372916472,2.25057986218748,103.422435477304));
#25450=CARTESIAN_POINT('Ctrl Pts',(2.16374507961965,2.18492631621293,103.417443235819));
#25451=CARTESIAN_POINT('Ctrl Pts',(2.23117279423004,2.11601515269204,103.412450994333));
#25452=CARTESIAN_POINT('Ctrl Pts',(2.29514009236418,2.04419524664905,103.407458752847));
#25453=CARTESIAN_POINT('Ctrl Pts',(2.35920408615418,1.97226677461809,103.402458964879));
#25454=CARTESIAN_POINT('Ctrl Pts',(2.41979695160821,1.89742112725603,103.397459176911));
#25455=CARTESIAN_POINT('Ctrl Pts',(2.47666379764105,1.82003809945128,103.392459388943));
#25456=CARTESIAN_POINT('Ctrl Pts',(2.48870571312885,1.80365175229081,103.391400652115));
#25457=CARTESIAN_POINT('Ctrl Pts',(2.50058071237939,1.78715172008231,103.390341915288));
#25458=CARTESIAN_POINT('Ctrl Pts',(2.51228663814601,1.7705417526263,103.38928317846));
#25459=CARTESIAN_POINT('Ctrl Pts',(2.56756372444965,1.69210706724807,103.384283668967));
#25460=CARTESIAN_POINT('Ctrl Pts',(2.61926123270116,1.61094347370205,103.379284159474));
#25461=CARTESIAN_POINT('Ctrl Pts',(2.6670988678853,1.52741149626582,103.374284649981));
#25462=CARTESIAN_POINT('Ctrl Pts',(2.71487161162101,1.44399282942666,103.369291922291));
#25463=CARTESIAN_POINT('Ctrl Pts',(2.75879467199935,1.35821254138241,103.364299194601));
#25464=CARTESIAN_POINT('Ctrl Pts',(2.79862999518409,1.27046149097715,103.359306466911));
#25465=CARTESIAN_POINT('Ctrl Pts',(2.83842329310691,1.18280301571834,103.354319006423));
#25466=CARTESIAN_POINT('Ctrl Pts',(2.87413724626096,1.09317830881245,103.349331545934));
#25467=CARTESIAN_POINT('Ctrl Pts',(2.90557937086777,1.00200337803205,103.344344085446));
#25468=CARTESIAN_POINT('Ctrl Pts',(2.93699899789952,0.910893685045682,103.339360193603));
#25469=CARTESIAN_POINT('Ctrl Pts',(2.96415273004939,0.818236387054327,103.334376301759));
#25470=CARTESIAN_POINT('Ctrl Pts',(2.98689631737574,0.724467141592515,103.329392409915));
#25471=CARTESIAN_POINT('Ctrl Pts',(3.00963162205088,0.630732044567546,103.324410333082));
#25472=CARTESIAN_POINT('Ctrl Pts',(3.02795986961644,0.535886230808812,103.319428256248));
#25473=CARTESIAN_POINT('Ctrl Pts',(3.04178703534541,0.440379247472645,103.314446179414));
#25474=CARTESIAN_POINT('Ctrl Pts',(3.05561294035544,0.344880972172903,103.309464556831));
#25475=CARTESIAN_POINT('Ctrl Pts',(3.0649385167558,0.248722081609561,103.304482934248));
#25476=CARTESIAN_POINT('Ctrl Pts',(3.06972127333403,0.152359948938327,103.299501311665));
#25477=CARTESIAN_POINT('Ctrl Pts',(3.07450489950169,0.0559802959333553,
103.294518783335));
#25478=CARTESIAN_POINT('Ctrl Pts',(3.07474404375544,-0.0406022341483371,
103.289536255005));
#25479=CARTESIAN_POINT('Ctrl Pts',(3.07044830650883,-0.136928620299167,
103.284553726675));
#25480=CARTESIAN_POINT('Ctrl Pts',(3.06614793909059,-0.23335883209767,103.279565827914));
#25481=CARTESIAN_POINT('Ctrl Pts',(3.05730295145221,-0.329531909532675,
103.274577929153));
#25482=CARTESIAN_POINT('Ctrl Pts',(3.04397496614524,-0.424992535794552,
103.269590030392));
#25483=CARTESIAN_POINT('Ctrl Pts',(3.03063910781443,-0.520509551958479,
103.264599185211));
#25484=CARTESIAN_POINT('Ctrl Pts',(3.01281505994994,-0.615312847756394,
103.25960834003));
#25485=CARTESIAN_POINT('Ctrl Pts',(2.99061545682705,-0.708957995502657,
103.254617494848));
#25486=CARTESIAN_POINT('Ctrl Pts',(2.96837997858488,-0.802754476172602,
103.249618584335));
#25487=CARTESIAN_POINT('Ctrl Pts',(2.94175494702062,-0.895388650028548,
103.244619673822));
#25488=CARTESIAN_POINT('Ctrl Pts',(2.91090264273685,-0.986431981693414,
103.239620763309));
#25489=CARTESIAN_POINT('Ctrl Pts',(2.89299104918402,-1.03928803865039,103.236718599098));
#25490=CARTESIAN_POINT('Ctrl Pts',(2.8736555610664,-1.09160827303963,103.233816434887));
#25491=CARTESIAN_POINT('Ctrl Pts',(2.85293514461264,-1.14331242914353,103.230914270676));
#25492=CARTESIAN_POINT('Ctrl Pts',(2.81724043155436,-1.23238230957604,103.225914761183));
#25493=CARTESIAN_POINT('Ctrl Pts',(2.77730782451965,-1.3199354258661,103.22091525169));
#25494=CARTESIAN_POINT('Ctrl Pts',(2.73328712143254,-1.40554038071164,103.215915742197));
#25495=CARTESIAN_POINT('Ctrl Pts',(2.68932613214967,-1.49102921297946,103.210923014507));
#25496=CARTESIAN_POINT('Ctrl Pts',(2.64128826710602,-1.57457474889841,103.205930286817));
#25497=CARTESIAN_POINT('Ctrl Pts',(2.58937176690187,-1.65576450703942,103.200937559127));
#25498=CARTESIAN_POINT('Ctrl Pts',(2.53751003729684,-1.73686861203202,103.195950098639));
#25499=CARTESIAN_POINT('Ctrl Pts',(2.48177804212799,-1.81562151199361,103.19096263815));
#25500=CARTESIAN_POINT('Ctrl Pts',(2.42241992741185,-1.89163525693458,103.185975177662));
#25501=CARTESIAN_POINT('Ctrl Pts',(2.3631042848142,-1.96759461226434,103.180991285819));
#25502=CARTESIAN_POINT('Ctrl Pts',(2.30016794995018,-2.04081836383862,103.176007393975));
#25503=CARTESIAN_POINT('Ctrl Pts',(2.23389781189284,-2.11094832149449,103.171023502131));
#25504=CARTESIAN_POINT('Ctrl Pts',(2.16765180777847,-2.18105273955668,103.166041425298));
#25505=CARTESIAN_POINT('Ctrl Pts',(2.0980747139139,-2.24806528357457,103.161059348464));
#25506=CARTESIAN_POINT('Ctrl Pts',(2.02549241507628,-2.31166232968149,103.15607727163));
#25507=CARTESIAN_POINT('Ctrl Pts',(1.95291673407208,-2.37525357720303,103.151095649047));
#25508=CARTESIAN_POINT('Ctrl Pts',(1.87733672314457,-2.43542965681751,103.146114026464));
#25509=CARTESIAN_POINT('Ctrl Pts',(1.79911288896127,-2.49190590969511,103.141132403881));
#25510=CARTESIAN_POINT('Ctrl Pts',(1.72087483230664,-2.54839243095058,103.136149875551));
#25511=CARTESIAN_POINT('Ctrl Pts',(1.63999235365309,-2.60117753257764,103.131167347221));
#25512=CARTESIAN_POINT('Ctrl Pts',(1.55685570324067,-2.650019352625,103.126184818892));
#25513=CARTESIAN_POINT('Ctrl Pts',(1.47362944377158,-2.69891381695617,103.12119692013));
#25514=CARTESIAN_POINT('Ctrl Pts',(1.38814454104967,-2.743856291702,103.116209021369));
#25515=CARTESIAN_POINT('Ctrl Pts',(1.30081646179655,-2.78465056743555,103.111221122608));
#25516=CARTESIAN_POINT('Ctrl Pts',(1.21343679664838,-2.82546894090769,103.106230277427));
#25517=CARTESIAN_POINT('Ctrl Pts',(1.12421219283913,-2.86213406945711,103.101239432246));
#25518=CARTESIAN_POINT('Ctrl Pts',(1.03357675678986,-2.89449846049774,103.096248587064));
#25519=CARTESIAN_POINT('Ctrl Pts',(0.942794851587153,-2.92691515321157,
103.091249676551));
#25520=CARTESIAN_POINT('Ctrl Pts',(0.850597981214573,-2.95501710270414,
103.086250766038));
#25521=CARTESIAN_POINT('Ctrl Pts',(0.757433951767733,-2.97870711193791,
103.081251855525));
#25522=CARTESIAN_POINT('Ctrl Pts',(0.703346703896485,-2.99246056817105,
103.078349691314));
#25523=CARTESIAN_POINT('Ctrl Pts',(0.648933658242725,-3.00472794319488,
103.075447527103));
#25524=CARTESIAN_POINT('Ctrl Pts',(0.594283347907237,-3.01549822623064,
103.072545362892));
#25525=CARTESIAN_POINT('Ctrl Pts',(0.500138177112909,-3.03405201173855,
103.067545853399));
#25526=CARTESIAN_POINT('Ctrl Pts',(0.404957928388729,-3.04822527986852,
103.062546343906));
#25527=CARTESIAN_POINT('Ctrl Pts',(0.309186012177099,-3.05790880502902,
103.057546834413));
#25528=CARTESIAN_POINT('Ctrl Pts',(0.213544009961789,-3.06757919454913,
103.052554106723));
#25529=CARTESIAN_POINT('Ctrl Pts',(0.117312368359615,-3.07277190140275,
103.047561379033));
#25530=CARTESIAN_POINT('Ctrl Pts',(0.020945006015351,-3.07342863211805,
103.042568651343));
#25531=CARTESIAN_POINT('Ctrl Pts',(-0.0753206911909299,-3.074084669999,
103.037581190855));
#25532=CARTESIAN_POINT('Ctrl Pts',(-0.171721387884164,-3.07021424173392,
103.032593730366));
#25533=CARTESIAN_POINT('Ctrl Pts',(-0.267798748926218,-3.06181091514051,
103.027606269878));
#25534=CARTESIAN_POINT('Ctrl Pts',(-0.363807364370635,-3.0534136013237,
103.022622378035));
#25535=CARTESIAN_POINT('Ctrl Pts',(-0.459492668046105,-3.04048987503179,
103.017638486191));
#25536=CARTESIAN_POINT('Ctrl Pts',(-0.55439801560365,-3.02308535941259,
103.012654594347));
#25537=CARTESIAN_POINT('Ctrl Pts',(-0.64926880098422,-3.0056871820869,103.007672517514));
#25538=CARTESIAN_POINT('Ctrl Pts',(-0.743359763284123,-2.98381153672753,
103.00269044068));
#25539=CARTESIAN_POINT('Ctrl Pts',(-0.836222020825068,-2.957555575452,102.997708363846));
#25540=CARTESIAN_POINT('Ctrl Pts',(-0.929075811467547,-2.93130200811525,
102.992726741263));
#25541=CARTESIAN_POINT('Ctrl Pts',(-1.02070069773359,-2.90066903851846,
102.98774511868));
#25542=CARTESIAN_POINT('Ctrl Pts',(-1.11066163157496,-2.86580407392886,
102.982763496097));
#25543=CARTESIAN_POINT('Ctrl Pts',(-1.20063892189915,-2.8309327702744,102.977780967767));
#25544=CARTESIAN_POINT('Ctrl Pts',(-1.28895124968016,-2.79182810215373,
102.972798439437));
#25545=CARTESIAN_POINT('Ctrl Pts',(-1.37518327062679,-2.74868572634054,
102.967815911107));
#25546=CARTESIAN_POINT('Ctrl Pts',(-1.46150823698312,-2.70549684940454,
102.962828012346));
#25547=CARTESIAN_POINT('Ctrl Pts',(-1.545748026809,-2.65826177303416,102.957840113585));
#25548=CARTESIAN_POINT('Ctrl Pts',(-1.62751185964566,-2.60722216098144,
102.952852214824));
#25549=CARTESIAN_POINT('Ctrl Pts',(-1.70932399150057,-2.55615239912937,
102.947861369643));
#25550=CARTESIAN_POINT('Ctrl Pts',(-1.78865689328987,-2.50127387628021,
102.942870524462));
#25551=CARTESIAN_POINT('Ctrl Pts',(-1.86515049945167,-2.44287041498217,
102.93787967928));
#25552=CARTESIAN_POINT('Ctrl Pts',(-1.94176772121277,-2.38437257221578,
102.932880768767));
#25553=CARTESIAN_POINT('Ctrl Pts',(-2.01553614964289,-2.3223386988988,102.927881858254));
#25554=CARTESIAN_POINT('Ctrl Pts',(-2.086130447889,-2.25709149225068,102.922882947741));
#25555=CARTESIAN_POINT('Ctrl Pts',(-2.12711462740793,-2.21921161672516,
102.91998078353));
#25556=CARTESIAN_POINT('Ctrl Pts',(-2.1670296745846,-2.1802493652989,102.917078619319));
#25557=CARTESIAN_POINT('Ctrl Pts',(-2.2058181516778,-2.14027300401812,102.914176455108));
#25558=CARTESIAN_POINT('Ctrl Pts',(-2.27409282468423,-2.06990744189837,
102.909068125847));
#25559=CARTESIAN_POINT('Ctrl Pts',(-2.33913739562393,-1.996126757291,102.903959796586));
#25560=CARTESIAN_POINT('Ctrl Pts',(-2.4005870002092,-1.9192666058749,102.898851467326));
#25561=CARTESIAN_POINT('Ctrl Pts',(-2.45984031151225,-1.84515354185449,
102.89392571677));
#25562=CARTESIAN_POINT('Ctrl Pts',(-2.51575090150008,-1.76817775298914,
102.888999966214));
#25563=CARTESIAN_POINT('Ctrl Pts',(-2.56802759118943,-1.68867893363121,
102.884074215659));
#25564=CARTESIAN_POINT('Ctrl Pts',(-2.62025593278434,-1.60925363875328,
102.879153020683));
#25565=CARTESIAN_POINT('Ctrl Pts',(-2.66885679969573,-1.52731032102897,
102.874231825708));
#25566=CARTESIAN_POINT('Ctrl Pts',(-2.71357986674681,-1.44322089673978,
102.869310630733));
#25567=CARTESIAN_POINT('Ctrl Pts',(-2.75827455989699,-1.35918482176559,
102.864392557938));
#25568=CARTESIAN_POINT('Ctrl Pts',(-2.7990961280248,-1.27300574208554,102.859474485143));
#25569=CARTESIAN_POINT('Ctrl Pts',(-2.83583876812314,-1.18508258413067,
102.854556412349));
#25570=CARTESIAN_POINT('Ctrl Pts',(-2.87256876478253,-1.09718968124397,
102.849640031903));
#25571=CARTESIAN_POINT('Ctrl Pts',(-2.90522244952974,-1.00755430938457,
102.844723651456));
#25572=CARTESIAN_POINT('Ctrl Pts',(-2.93364152684788,-0.91659677173425,
102.83980727101));
#25573=CARTESIAN_POINT('Ctrl Pts',(-2.96206829382904,-0.825614622700294,
102.834889560285));
#25574=CARTESIAN_POINT('Ctrl Pts',(-2.98625802504285,-0.733310023163684,
102.82997184956));
#25575=CARTESIAN_POINT('Ctrl Pts',(-3.0061020888235,-0.640119115142639,
102.825054138834));
#25576=CARTESIAN_POINT('Ctrl Pts',(-3.02594955728513,-0.546912218193335,
102.820135584369));
#25577=CARTESIAN_POINT('Ctrl Pts',(-3.04144979336049,-0.452819154589259,
102.815217029903));
#25578=CARTESIAN_POINT('Ctrl Pts',(-3.05254548904124,-0.358285203900466,
102.810298475437));
#25579=CARTESIAN_POINT('Ctrl Pts',(-3.06365068804381,-0.263670286088727,
102.805375708292));
#25580=CARTESIAN_POINT('Ctrl Pts',(-3.07034378241226,-0.168614177656698,
102.800452941148));
#25581=CARTESIAN_POINT('Ctrl Pts',(-3.07261946386603,-0.0735654828818875,
102.795530174003));
#25582=CARTESIAN_POINT('Ctrl Pts',(-3.07322868642112,-0.0481200021036727,
102.794212300285));
#25583=CARTESIAN_POINT('Ctrl Pts',(-3.07352160822751,-0.0226750436337593,
102.792894426567));
#25584=CARTESIAN_POINT('Ctrl Pts',(-3.07349876002173,0.00276082323151584,
102.791576552849));
#25585=CARTESIAN_POINT('Origin',(0.,0.,116.208423447177));
#25586=CARTESIAN_POINT('',(1.8723819390353,2.43733217358127,104.437267724146));
#25587=CARTESIAN_POINT('',(1.87238193903531,2.43733217358127,104.354220317975));
#25588=CARTESIAN_POINT('',(1.8723819390353,2.43733217358128,116.208423447177));
#25589=CARTESIAN_POINT('',(-3.07349999209142,-0.000220485887778205,103.708423447147));
#25590=CARTESIAN_POINT('Ctrl Pts',(1.87238193903531,2.43733217358127,104.354220317975));
#25591=CARTESIAN_POINT('Ctrl Pts',(1.92554476800143,2.39649197877191,104.350735398405));
#25592=CARTESIAN_POINT('Ctrl Pts',(1.97731444018826,2.35395489326419,104.347250478836));
#25593=CARTESIAN_POINT('Ctrl Pts',(2.02758160247093,2.30983010096444,104.343765559266));
#25594=CARTESIAN_POINT('Ctrl Pts',(2.09969550639227,2.24652811835879,104.338766049773));
#25595=CARTESIAN_POINT('Ctrl Pts',(2.1689687585394,2.17973457216113,104.33376654028));
#25596=CARTESIAN_POINT('Ctrl Pts',(2.23504440315198,2.10973428799435,104.328767030787));
#25597=CARTESIAN_POINT('Ctrl Pts',(2.3010304165722,2.03982895876856,104.323774303097));
#25598=CARTESIAN_POINT('Ctrl Pts',(2.36382714428195,1.96672585323331,104.318781575407));
#25599=CARTESIAN_POINT('Ctrl Pts',(2.42311158959213,1.89074918336206,104.313788847717));
#25600=CARTESIAN_POINT('Ctrl Pts',(2.48233349130688,1.81485266696239,104.308801387229));
#25601=CARTESIAN_POINT('Ctrl Pts',(2.53805020806858,1.7360889569736,104.30381392674));
#25602=CARTESIAN_POINT('Ctrl Pts',(2.58997715335333,1.65481739026026,104.298826466252));
#25603=CARTESIAN_POINT('Ctrl Pts',(2.64186694369491,1.57360397525267,104.293842574408));
#25604=CARTESIAN_POINT('Ctrl Pts',(2.68997211756546,1.48988663960697,104.288858682565));
#25605=CARTESIAN_POINT('Ctrl Pts',(2.73405037656118,1.40405512300111,104.283874790721));
#25606=CARTESIAN_POINT('Ctrl Pts',(2.77811258334667,1.3182548641078,104.278892713887));
#25607=CARTESIAN_POINT('Ctrl Pts',(2.81815058871434,1.23034234410879,104.273910637054));
#25608=CARTESIAN_POINT('Ctrl Pts',(2.85396766778545,1.14073257218127,104.26892856022));
#25609=CARTESIAN_POINT('Ctrl Pts',(2.88978148116412,1.05113097060046,104.263946937637));
#25610=CARTESIAN_POINT('Ctrl Pts',(2.92137497065069,0.959832832439655,104.258965315054));
#25611=CARTESIAN_POINT('Ctrl Pts',(2.94859967732581,0.867272847997753,104.253983692471));
#25612=CARTESIAN_POINT('Ctrl Pts',(2.97582933393228,0.774696034519856,104.249001164141));
#25613=CARTESIAN_POINT('Ctrl Pts',(2.9986885063732,0.68085734025023,104.244018635811));
#25614=CARTESIAN_POINT('Ctrl Pts',(3.01707899164171,0.58620526114514,104.239036107481));
#25615=CARTESIAN_POINT('Ctrl Pts',(3.03548929914299,0.491451161048425,104.23404820872));
#25616=CARTESIAN_POINT('Ctrl Pts',(3.0494212197408,0.395882357466433,104.229060309959));
#25617=CARTESIAN_POINT('Ctrl Pts',(3.05882799262756,0.299955932626856,104.224072411198));
#25618=CARTESIAN_POINT('Ctrl Pts',(3.06824032222418,0.203972842731484,104.219081566017));
#25619=CARTESIAN_POINT('Ctrl Pts',(3.07312215939221,0.107632149136793,104.214090720836));
#25620=CARTESIAN_POINT('Ctrl Pts',(3.0734788864626,0.0113922986534843,104.209099875654));
#25621=CARTESIAN_POINT('Ctrl Pts',(3.07383619001295,-0.0850030778585972,
104.204100965141));
#25622=CARTESIAN_POINT('Ctrl Pts',(3.06965380067041,-0.181296847600807,
104.199102054628));
#25623=CARTESIAN_POINT('Ctrl Pts',(3.0609890886171,-0.277034383005151,104.194103144115));
#25624=CARTESIAN_POINT('Ctrl Pts',(3.05595870906673,-0.332615703808248,
104.191200979904));
#25625=CARTESIAN_POINT('Ctrl Pts',(3.04941853195809,-0.388009693650793,
104.188298815693));
#25626=CARTESIAN_POINT('Ctrl Pts',(3.04138763737108,-0.443129201527433,
104.185396651482));
#25627=CARTESIAN_POINT('Ctrl Pts',(3.02755295028724,-0.538082651037559,
104.180397141989));
#25628=CARTESIAN_POINT('Ctrl Pts',(3.00924296930636,-0.632554371002716,
104.175397632496));
#25629=CARTESIAN_POINT('Ctrl Pts',(2.9865022588426,-0.726089875929984,104.170398123003));
#25630=CARTESIAN_POINT('Ctrl Pts',(2.9637923960082,-0.81949850053874,104.165405395313));
#25631=CARTESIAN_POINT('Ctrl Pts',(2.93666385149201,-0.911973011201854,
104.160412667623));
#25632=CARTESIAN_POINT('Ctrl Pts',(2.90521271574455,-1.00306596307329,104.155419939933));
#25633=CARTESIAN_POINT('Ctrl Pts',(2.87379476015253,-1.09406281417667,104.150432479445));
#25634=CARTESIAN_POINT('Ctrl Pts',(2.83806342127841,-1.18368059120868,104.145445018956));
#25635=CARTESIAN_POINT('Ctrl Pts',(2.79816516453479,-1.27148494367176,104.140457558468));
#25636=CARTESIAN_POINT('Ctrl Pts',(2.75829545592651,-1.3592264700682,104.135473666624));
#25637=CARTESIAN_POINT('Ctrl Pts',(2.71426493765869,-1.44515675286649,104.130489774781));
#25638=CARTESIAN_POINT('Ctrl Pts',(2.66626860062224,-1.52886035965876,104.125505882937));
#25639=CARTESIAN_POINT('Ctrl Pts',(2.61828974266299,-1.61253348367056,104.120523806103));
#25640=CARTESIAN_POINT('Ctrl Pts',(2.56634815364014,-1.69398116243539,104.11554172927));
#25641=CARTESIAN_POINT('Ctrl Pts',(2.51068483288244,-1.77281243224828,104.110559652436));
#25642=CARTESIAN_POINT('Ctrl Pts',(2.45502658733718,-1.85163651446555,104.105578029853));
#25643=CARTESIAN_POINT('Ctrl Pts',(2.39564753806593,-1.92784430355049,104.10059640727));
#25644=CARTESIAN_POINT('Ctrl Pts',(2.33283147124749,-2.00107460549507,104.095614784687));
#25645=CARTESIAN_POINT('Ctrl Pts',(2.27000398336133,-2.07431822199882,104.090632256357));
#25646=CARTESIAN_POINT('Ctrl Pts',(2.20373852267581,-2.14458294306888,104.085649728027));
#25647=CARTESIAN_POINT('Ctrl Pts',(2.13435781735861,-2.21154221245723,104.080667199697));
#25648=CARTESIAN_POINT('Ctrl Pts',(2.06490232986631,-2.27857365406961,104.075679300936));
#25649=CARTESIAN_POINT('Ctrl Pts',(1.99232521063532,-2.34229222588164,104.070691402175));
#25650=CARTESIAN_POINT('Ctrl Pts',(1.91698439771724,-2.40240984615629,104.065703503414));
#25651=CARTESIAN_POINT('Ctrl Pts',(1.84159907994687,-2.46256297873438,104.060712658233));
#25652=CARTESIAN_POINT('Ctrl Pts',(1.76344717327735,-2.51911066710761,104.055721813052));
#25653=CARTESIAN_POINT('Ctrl Pts',(1.68291614977514,-2.57180782385194,104.05073096787));
#25654=CARTESIAN_POINT('Ctrl Pts',(1.60225498610525,-2.62459014053234,104.045732057357));
#25655=CARTESIAN_POINT('Ctrl Pts',(1.5192074065279,-2.67350927787263,104.040733146844));
#25656=CARTESIAN_POINT('Ctrl Pts',(1.43418598442494,-2.71836583484988,104.035734236331));
#25657=CARTESIAN_POINT('Ctrl Pts',(1.38482600333623,-2.74440772816731,104.03283207212));
#25658=CARTESIAN_POINT('Ctrl Pts',(1.33480114237456,-2.76908122230678,104.029929907909));
#25659=CARTESIAN_POINT('Ctrl Pts',(1.28419489131014,-2.79235487199119,104.027027743698));
#25660=CARTESIAN_POINT('Ctrl Pts',(1.19701635343025,-2.83244799700915,104.022028234205));
#25661=CARTESIAN_POINT('Ctrl Pts',(1.10780530582788,-2.86852500162958,104.017028724712));
#25662=CARTESIAN_POINT('Ctrl Pts',(1.01696723059307,-2.9003758208032,104.012029215219));
#25663=CARTESIAN_POINT('Ctrl Pts',(0.926252376630513,-2.93218343454286,
104.007036487529));
#25664=CARTESIAN_POINT('Ctrl Pts',(0.833915292099658,-2.95977611238127,
104.002043759839));
#25665=CARTESIAN_POINT('Ctrl Pts',(0.740383606881194,-2.9829908422021,103.997051032149));
#25666=CARTESIAN_POINT('Ctrl Pts',(0.646950595232957,-3.00618108106815,
103.992063571661));
#25667=CARTESIAN_POINT('Ctrl Pts',(0.552325912015178,-3.02500244828318,
103.987076111172));
#25668=CARTESIAN_POINT('Ctrl Pts',(0.456953630396812,-3.03934131509891,
103.982088650684));
#25669=CARTESIAN_POINT('Ctrl Pts',(0.361649589875361,-3.05366992212025,
103.97710475884));
#25670=CARTESIAN_POINT('Ctrl Pts',(0.265599447196298,-3.06352233969462,
103.972120866997));
#25671=CARTESIAN_POINT('Ctrl Pts',(0.169257826953313,-3.06883594185402,
103.967136975153));
#25672=CARTESIAN_POINT('Ctrl Pts',(0.0729512919423281,-3.07414760893112,
103.962154898319));
#25673=CARTESIAN_POINT('Ctrl Pts',(-0.0236460718779519,-3.07492372062509,
103.957172821486));
#25674=CARTESIAN_POINT('Ctrl Pts',(-0.120075114707274,-3.07115356451416,
103.952190744652));
#25675=CARTESIAN_POINT('Ctrl Pts',(-0.216495365429501,-3.06738375215461,
103.947209122069));
#25676=CARTESIAN_POINT('Ctrl Pts',(-0.312746887053481,-3.059068513455,103.942227499486));
#25677=CARTESIAN_POINT('Ctrl Pts',(-0.408372205003796,-3.04624923343123,
103.937245876903));
#25678=CARTESIAN_POINT('Ctrl Pts',(-0.504014909321746,-3.03342762263648,
103.932263348573));
#25679=CARTESIAN_POINT('Ctrl Pts',(-0.599030748788974,-3.01610040251193,
103.927280820243));
#25680=CARTESIAN_POINT('Ctrl Pts',(-0.692970100689274,-2.99436048089583,
103.922298291913));
#25681=CARTESIAN_POINT('Ctrl Pts',(-0.787010705366312,-2.97259712684821,
103.917310393152));
#25682=CARTESIAN_POINT('Ctrl Pts',(-0.879972077686123,-2.94641167504668,
103.912322494391));
#25683=CARTESIAN_POINT('Ctrl Pts',(-0.971417696979223,-2.91594751461606,
103.90733459563));
#25684=CARTESIAN_POINT('Ctrl Pts',(-1.06291733445483,-2.88546535858772,
103.902343750449));
#25685=CARTESIAN_POINT('Ctrl Pts',(-1.15289902679166,-2.85069961940891,
103.897352905268));
#25686=CARTESIAN_POINT('Ctrl Pts',(-1.24094623677775,-2.8118418674291,103.892362060086));
#25687=CARTESIAN_POINT('Ctrl Pts',(-1.32913573327866,-2.7729213203408,103.887363149573));
#25688=CARTESIAN_POINT('Ctrl Pts',(-1.41538411261891,-2.72989575197777,
103.88236423906));
#25689=CARTESIAN_POINT('Ctrl Pts',(-1.49929949253701,-2.68300266151159,
103.877365328547));
#25690=CARTESIAN_POINT('Ctrl Pts',(-1.54801735049982,-2.65577843964668,
103.874463164336));
#25691=CARTESIAN_POINT('Ctrl Pts',(-1.59594940067385,-2.62725149460519,
103.871561000125));
#25692=CARTESIAN_POINT('Ctrl Pts',(-1.64302381086752,-2.59747473653207,
103.868658835914));
#25693=CARTESIAN_POINT('Ctrl Pts',(-1.72411810585929,-2.54617881602781,
103.863659326421));
#25694=CARTESIAN_POINT('Ctrl Pts',(-1.80295031313648,-2.49099145902901,
103.858659816928));
#25695=CARTESIAN_POINT('Ctrl Pts',(-1.87912346639947,-2.43213841054058,
103.853660307435));
#25696=CARTESIAN_POINT('Ctrl Pts',(-1.95519329126374,-2.37336519583872,
103.848667579745));
#25697=CARTESIAN_POINT('Ctrl Pts',(-2.02861088637677,-2.31093643822026,
103.843674852055));
#25698=CARTESIAN_POINT('Ctrl Pts',(-2.0990066946769,-2.24512207812884,103.838682124365));
#25699=CARTESIAN_POINT('Ctrl Pts',(-2.16932823717359,-2.17937715052848,
103.833694663876));
#25700=CARTESIAN_POINT('Ctrl Pts',(-2.23663401128075,-2.11025401901876,
103.828707203388));
#25701=CARTESIAN_POINT('Ctrl Pts',(-2.30058692975088,-2.03806330339845,
103.8237197429));
#25702=CARTESIAN_POINT('Ctrl Pts',(-2.36449408841299,-1.9659242419226,103.818735851056));
#25703=CARTESIAN_POINT('Ctrl Pts',(-2.42505287038437,-1.89072228738107,
103.813751959213));
#25704=CARTESIAN_POINT('Ctrl Pts',(-2.48196322441649,-1.81280467856968,
103.808768067369));
#25705=CARTESIAN_POINT('Ctrl Pts',(-2.53885285310721,-1.73491544542158,
103.803785990535));
#25706=CARTESIAN_POINT('Ctrl Pts',(-2.59209643513275,-1.65431287710342,
103.798803913701));
#25707=CARTESIAN_POINT('Ctrl Pts',(-2.64143500017088,-1.57137627253062,
103.793821836868));
#25708=CARTESIAN_POINT('Ctrl Pts',(-2.69076906666857,-1.48844722986545,
103.788840214285));
#25709=CARTESIAN_POINT('Ctrl Pts',(-2.73619859979841,-1.40318495139973,
103.783858591702));
#25710=CARTESIAN_POINT('Ctrl Pts',(-2.77750924024574,-1.31599569541451,
103.778876969119));
#25711=CARTESIAN_POINT('Ctrl Pts',(-2.81882739169535,-1.22879058688639,
103.773894440789));
#25712=CARTESIAN_POINT('Ctrl Pts',(-2.85602497525254,-1.13965820172586,
103.768911912459));
#25713=CARTESIAN_POINT('Ctrl Pts',(-2.88893512350555,-1.0490262638161,103.763929384129));
#25714=CARTESIAN_POINT('Ctrl Pts',(-2.92188074404815,-0.958296638034406,
103.758941485368));
#25715=CARTESIAN_POINT('Ctrl Pts',(-2.95052955336883,-0.866064646002697,
103.753953586607));
#25716=CARTESIAN_POINT('Ctrl Pts',(-2.97476416079934,-0.772774506323692,
103.748965687846));
#25717=CARTESIAN_POINT('Ctrl Pts',(-2.99901308394508,-0.679429258878735,
103.743974842665));
#25718=CARTESIAN_POINT('Ctrl Pts',(-3.0188425229909,-0.585025048572415,
103.738983997483));
#25719=CARTESIAN_POINT('Ctrl Pts',(-3.03418638133272,-0.490015564380421,
103.733993152302));
#25720=CARTESIAN_POINT('Ctrl Pts',(-3.04955503573711,-0.394852542462566,
103.728994241789));
#25721=CARTESIAN_POINT('Ctrl Pts',(-3.06042358569747,-0.299082729402581,
103.723995331276));
#25722=CARTESIAN_POINT('Ctrl Pts',(-3.06677788277764,-0.203164139812822,
103.718996420763));
#25723=CARTESIAN_POINT('Ctrl Pts',(-3.07046692932559,-0.147477706310342,
103.716094256552));
#25724=CARTESIAN_POINT('Ctrl Pts',(-3.072635427446,-0.0917411326516463,
103.713192092341));
#25725=CARTESIAN_POINT('Ctrl Pts',(-3.07328864861143,-0.0360434781358497,
103.71028992813));
#25726=CARTESIAN_POINT('Ctrl Pts',(-3.07342868489404,-0.0241031233202659,
103.709667767812));
#25727=CARTESIAN_POINT('Ctrl Pts',(-3.07349913543572,-0.0121619508103782,
103.709045607495));
#25728=CARTESIAN_POINT('Ctrl Pts',(-3.07349999209138,-0.00022048645764921,
103.708423447177));
#25729=CARTESIAN_POINT('Ctrl Pts',(-3.07349999209142,-0.000220485887798679,
103.708423447147));
#25730=CARTESIAN_POINT('Ctrl Pts',(-3.07350686177119,0.0955405667047918,
103.703434215918));
#25731=CARTESIAN_POINT('Ctrl Pts',(-3.06903399632083,0.19147336895022,103.698444984688));
#25732=CARTESIAN_POINT('Ctrl Pts',(-3.06005921735193,0.287123381666347,
103.693455753459));
#25733=CARTESIAN_POINT('Ctrl Pts',(-3.05109660653681,0.382643710512995,
103.688473286711));
#25734=CARTESIAN_POINT('Ctrl Pts',(-3.03764425268558,0.477881576496013,
103.683490819964));
#25735=CARTESIAN_POINT('Ctrl Pts',(-3.01973198023759,0.572381880854357,
103.678508353217));
#25736=CARTESIAN_POINT('Ctrl Pts',(-3.00183853139196,0.66678287697818,103.673531122431));
#25737=CARTESIAN_POINT('Ctrl Pts',(-2.97949456191652,0.760447421190341,
103.668553891645));
#25738=CARTESIAN_POINT('Ctrl Pts',(-2.95278164141698,0.852926039062489,
103.66357666086));
#25739=CARTESIAN_POINT('Ctrl Pts',(-2.92608756204122,0.945339430031195,
103.658602940608));
#25740=CARTESIAN_POINT('Ctrl Pts',(-2.89503077887684,1.0365681348272,103.653629220357));
#25741=CARTESIAN_POINT('Ctrl Pts',(-2.85974361903482,1.12617435745519,103.648655500106));
#25742=CARTESIAN_POINT('Ctrl Pts',(-2.8244689530173,1.21574885397023,103.643683540857));
#25743=CARTESIAN_POINT('Ctrl Pts',(-2.78496704750032,1.30370159967069,103.638711581608));
#25744=CARTESIAN_POINT('Ctrl Pts',(-2.74141929053079,1.38961236447639,103.63373962236));
#25745=CARTESIAN_POINT('Ctrl Pts',(-2.6978749304007,1.47551642801675,103.628768050937));
#25746=CARTESIAN_POINT('Ctrl Pts',(-2.65028554591197,1.5593784341012,103.623796479514));
#25747=CARTESIAN_POINT('Ctrl Pts',(-2.59887915058709,1.64080145375475,103.618824908091));
#25748=CARTESIAN_POINT('Ctrl Pts',(-2.54746257395873,1.72224059966009,103.613852352023));
#25749=CARTESIAN_POINT('Ctrl Pts',(-2.49222772076612,1.80123942705036,103.608879795955));
#25750=CARTESIAN_POINT('Ctrl Pts',(-2.43344610934209,1.87742970119466,103.603907239887));
#25751=CARTESIAN_POINT('Ctrl Pts',(-2.37460080953994,1.95370252555952,103.598929296181));
#25752=CARTESIAN_POINT('Ctrl Pts',(-2.31220135081348,2.02716037302272,103.593951352474));
#25753=CARTESIAN_POINT('Ctrl Pts',(-2.24655957870032,2.09746807111571,103.588973408768));
#25754=CARTESIAN_POINT('Ctrl Pts',(-2.1808777071248,2.16781871900732,103.58399242412));
#25755=CARTESIAN_POINT('Ctrl Pts',(-2.11194989471064,2.23501507910632,103.579011439471));
#25756=CARTESIAN_POINT('Ctrl Pts',(-2.04012333245904,2.29876032642732,103.574030454822));
#25757=CARTESIAN_POINT('Ctrl Pts',(-1.96818290487756,2.36260662791807,103.56904157391));
#25758=CARTESIAN_POINT('Ctrl Pts',(-1.893334896855,2.42299061889371,103.564052692998));
#25759=CARTESIAN_POINT('Ctrl Pts',(-1.81595775176263,2.47965717263762,103.559063812085));
#25760=CARTESIAN_POINT('Ctrl Pts',(-1.77902970834285,2.50670113962046,103.556682881505));
#25761=CARTESIAN_POINT('Ctrl Pts',(-1.74152601481376,2.53289905886596,103.554301950925));
#25762=CARTESIAN_POINT('Ctrl Pts',(-1.70348979365066,2.55822688065935,103.551921020345));
#25763=CARTESIAN_POINT('Ctrl Pts',(-1.62362083384975,2.6114105755376,103.546921510852));
#25764=CARTESIAN_POINT('Ctrl Pts',(-1.54111857553593,2.66094378308383,103.541922001359));
#25765=CARTESIAN_POINT('Ctrl Pts',(-1.45635082880781,2.70655583970307,103.536922491866));
#25766=CARTESIAN_POINT('Ctrl Pts',(-1.37169806898992,2.75210602385711,103.531929764176));
#25767=CARTESIAN_POINT('Ctrl Pts',(-1.2847863116298,2.79374542205784,103.526937036486));
#25768=CARTESIAN_POINT('Ctrl Pts',(-1.19601257379427,2.83124639926058,103.521944308796));
#25769=CARTESIAN_POINT('Ctrl Pts',(-1.10733249001449,2.86870781387764,103.516956848308));
#25770=CARTESIAN_POINT('Ctrl Pts',(-1.01679473296656,2.90203931679329,103.51196938782));
#25771=CARTESIAN_POINT('Ctrl Pts',(-0.924820254834743,2.93105949210305,
103.506981927331));
#25772=CARTESIAN_POINT('Ctrl Pts',(-0.832911586591893,2.96005890279904,
103.501998035488));
#25773=CARTESIAN_POINT('Ctrl Pts',(-0.739568658313955,2.98475298673084,
103.497014143644));
#25774=CARTESIAN_POINT('Ctrl Pts',(-0.645230789620226,3.00500906456637,
103.4920302518));
#25775=CARTESIAN_POINT('Ctrl Pts',(-0.55092727644181,3.02525776564004,103.487048174967));
#25776=CARTESIAN_POINT('Ctrl Pts',(-0.455629971504973,3.04107157979625,
103.482066098133));
#25777=CARTESIAN_POINT('Ctrl Pts',(-0.35979075107977,3.05236840264039,103.477084021299));
#25778=CARTESIAN_POINT('Ctrl Pts',(-0.26396026898355,3.06366419547454,103.472102398716));
#25779=CARTESIAN_POINT('Ctrl Pts',(-0.167588405601255,3.07044376461798,
103.467120776133));
#25780=CARTESIAN_POINT('Ctrl Pts',(-0.0711334977560217,3.07267672811459,
103.46213915355));
#25781=CARTESIAN_POINT('Ctrl Pts',(0.0253389472912264,3.07491009760332,
103.45715662522));
#25782=CARTESIAN_POINT('Ctrl Pts',(0.121894027946905,3.07259520958721,103.45217409689));
#25783=CARTESIAN_POINT('Ctrl Pts',(0.218073137580161,3.06575379909508,103.447191568561));
#25784=CARTESIAN_POINT('Ctrl Pts',(0.314355914118666,3.05890501457074,103.4422036698));
#25785=CARTESIAN_POINT('Ctrl Pts',(0.410261472025794,3.04751999844626,103.437215771038));
#25786=CARTESIAN_POINT('Ctrl Pts',(0.505336283203782,3.03167239174647,103.432227872277));
#25787=CARTESIAN_POINT('Ctrl Pts',(0.600467256377786,3.01581542364788,103.427237027096));
#25788=CARTESIAN_POINT('Ctrl Pts',(0.694766076784185,2.99549070848587,103.422246181915));
#25789=CARTESIAN_POINT('Ctrl Pts',(0.787791450553388,2.97082259322818,103.417255336733));
#25790=CARTESIAN_POINT('Ctrl Pts',(0.880967155675705,2.9461146136733,103.41225642622));
#25791=CARTESIAN_POINT('Ctrl Pts',(0.972864886699481,2.91704935082481,103.407257515707));
#25792=CARTESIAN_POINT('Ctrl Pts',(1.0630605493129,2.88380036037423,103.402258605194));
#25793=CARTESIAN_POINT('Ctrl Pts',(1.11542448408092,2.86449734827132,103.399356440983));
#25794=CARTESIAN_POINT('Ctrl Pts',(1.16721513135695,2.84378510836311,103.396454276772));
#25795=CARTESIAN_POINT('Ctrl Pts',(1.21835329387811,2.82170471546836,103.393552112561));
#25796=CARTESIAN_POINT('Ctrl Pts',(1.30644831913931,2.78366711939642,103.388552593281));
#25797=CARTESIAN_POINT('Ctrl Pts',(1.39291504089482,2.74143320287493,103.383553074001));
#25798=CARTESIAN_POINT('Ctrl Pts',(1.47732617133322,2.69516411995521,103.37855355472));
#25799=CARTESIAN_POINT('Ctrl Pts',(1.56161153330858,2.64896397570998,103.37356148448));
#25800=CARTESIAN_POINT('Ctrl Pts',(1.64384701257246,2.59874082935472,103.368569414239));
#25801=CARTESIAN_POINT('Ctrl Pts',(1.72362567342723,2.54470367388867,103.363577343999));
#25802=CARTESIAN_POINT('Ctrl Pts',(1.77423225055539,2.51042589275549,103.360410687841));
#25803=CARTESIAN_POINT('Ctrl Pts',(1.82385063493909,2.47461438658962,103.357244031683));
#25804=CARTESIAN_POINT('Ctrl Pts',(1.87238193903529,2.43733217358128,103.354077375525));
#25805=CARTESIAN_POINT('',(-3.07349992841428,-0.000663353166432896,103.791576552855));
#25806=CARTESIAN_POINT('Ctrl Pts',(-3.07349992841441,-0.000663352542477041,
103.791576552823));
#25807=CARTESIAN_POINT('Ctrl Pts',(-3.07352145853115,0.0990917671334288,
103.786438116722));
#25808=CARTESIAN_POINT('Ctrl Pts',(-3.06868209475957,0.198789365247624,
103.781299680621));
#25809=CARTESIAN_POINT('Ctrl Pts',(-3.05902469152581,0.297943260765191,
103.77616124452));
#25810=CARTESIAN_POINT('Ctrl Pts',(-3.04935854635228,0.397186910988275,
103.771018157076));
#25811=CARTESIAN_POINT('Ctrl Pts',(-3.03486571256589,0.495885482213515,
103.765875069631));
#25812=CARTESIAN_POINT('Ctrl Pts',(-3.0156405532298,0.593560699268277,103.760731982187));
#25813=CARTESIAN_POINT('Ctrl Pts',(-2.99637806306914,0.691425579062894,
103.755578908053));
#25814=CARTESIAN_POINT('Ctrl Pts',(-2.97236496789568,0.788262743622209,
103.75042583392));
#25815=CARTESIAN_POINT('Ctrl Pts',(-2.94374630484731,0.883606214723414,
103.745272759786));
#25816=CARTESIAN_POINT('Ctrl Pts',(-2.91509738297958,0.979050493499077,
103.740114237251));
#25817=CARTESIAN_POINT('Ctrl Pts',(-2.88183331879042,1.07299755565158,103.734955714717));
#25818=CARTESIAN_POINT('Ctrl Pts',(-2.84414762681942,1.16500065530346,103.729797192183));
#25819=CARTESIAN_POINT('Ctrl Pts',(-2.80638226408419,1.25719825734807,103.724627764092));
#25820=CARTESIAN_POINT('Ctrl Pts',(-2.7641767638206,1.34744332420583,103.719458336002));
#25821=CARTESIAN_POINT('Ctrl Pts',(-2.71777125569243,1.43531238820405,103.714288907911));
#25822=CARTESIAN_POINT('Ctrl Pts',(-2.69303114014139,1.48215792194269,103.711532936617));
#25823=CARTESIAN_POINT('Ctrl Pts',(-2.66709802246462,1.52832860739875,103.708776965323));
#25824=CARTESIAN_POINT('Ctrl Pts',(-2.64001321119417,1.57376379889748,103.706020994028));
#25825=CARTESIAN_POINT('Ctrl Pts',(-2.59087961849347,1.65618616363491,103.701021484535));
#25826=CARTESIAN_POINT('Ctrl Pts',(-2.53779613328403,1.73645013360103,103.696021975042));
#25827=CARTESIAN_POINT('Ctrl Pts',(-2.4809779245829,1.81415291189368,103.691022465549));
#25828=CARTESIAN_POINT('Ctrl Pts',(-2.42423678942116,1.89175028686088,103.686029737859));
#25829=CARTESIAN_POINT('Ctrl Pts',(-2.36377125624717,1.96679302367079,103.681037010169));
#25830=CARTESIAN_POINT('Ctrl Pts',(-2.29984139884962,2.03890455640704,103.676044282479));
#25831=CARTESIAN_POINT('Ctrl Pts',(-2.23597898584013,2.11094001329399,103.671056821991));
#25832=CARTESIAN_POINT('Ctrl Pts',(-2.16865980372973,2.1800500867846,103.666069361503));
#25833=CARTESIAN_POINT('Ctrl Pts',(-2.09818545004237,2.24588959373129,103.661081901014));
#25834=CARTESIAN_POINT('Ctrl Pts',(-2.02776152240241,2.31168199097176,103.656098009171));
#25835=CARTESIAN_POINT('Ctrl Pts',(-1.95418723102758,2.37420817500229,103.651114117327));
#25836=CARTESIAN_POINT('Ctrl Pts',(-1.87780175898322,2.43315901740094,103.646130225483));
#25837=CARTESIAN_POINT('Ctrl Pts',(-1.80144410463589,2.49208839136287,103.64114814865));
#25838=CARTESIAN_POINT('Ctrl Pts',(-1.72227765087632,2.54744474280995,103.636166071816));
#25839=CARTESIAN_POINT('Ctrl Pts',(-1.6406747159887,2.59895916210998,103.631183994982));
#25840=CARTESIAN_POINT('Ctrl Pts',(-1.5590792214087,2.65046888448181,103.626202372399));
#25841=CARTESIAN_POINT('Ctrl Pts',(-1.47504805866327,2.69813713699048,103.621220749816));
#25842=CARTESIAN_POINT('Ctrl Pts',(-1.38898167563165,2.74173889252049,103.616239127233));
#25843=CARTESIAN_POINT('Ctrl Pts',(-1.30289964421533,2.78534857561781,103.611256598903));
#25844=CARTESIAN_POINT('Ctrl Pts',(-1.21478204920664,2.82489009502186,103.606274070573));
#25845=CARTESIAN_POINT('Ctrl Pts',(-1.12505205241748,2.86018533129432,103.601291542243));
#25846=CARTESIAN_POINT('Ctrl Pts',(-1.03522533991596,2.89551861062976,103.596303643482));
#25847=CARTESIAN_POINT('Ctrl Pts',(-0.943783165187995,2.92659630859235,
103.591315744721));
#25848=CARTESIAN_POINT('Ctrl Pts',(-0.851166487319248,2.95328932901343,
103.58632784596));
#25849=CARTESIAN_POINT('Ctrl Pts',(-0.758495099507587,2.97999811736808,
103.581337000779));
#25850=CARTESIAN_POINT('Ctrl Pts',(-0.664648253947756,3.0023169693754,103.576346155598));
#25851=CARTESIAN_POINT('Ctrl Pts',(-0.570077733164632,3.02016781456757,
103.571355310416));
#25852=CARTESIAN_POINT('Ctrl Pts',(-0.475354384031829,3.03804750717635,
103.566356399903));
#25853=CARTESIAN_POINT('Ctrl Pts',(-0.379905458896058,3.05144471442974,
103.56135748939));
#25854=CARTESIAN_POINT('Ctrl Pts',(-0.284188438080711,3.06033318147898,
103.556358578877));
#25855=CARTESIAN_POINT('Ctrl Pts',(-0.228619027213755,3.06549346408315,
103.553456414666));
#25856=CARTESIAN_POINT('Ctrl Pts',(-0.172959285597081,3.06913505583286,
103.550554250455));
#25857=CARTESIAN_POINT('Ctrl Pts',(-0.11729838078186,3.07126087134681,103.547652086244));
#25858=CARTESIAN_POINT('Ctrl Pts',(-0.0214331825123264,3.07492217952003,
103.542653666825));
#25859=CARTESIAN_POINT('Ctrl Pts',(0.0747719474817214,3.07409716580575,
103.537655247406));
#25860=CARTESIAN_POINT('Ctrl Pts',(0.170862295476754,3.06874702867219,103.532656827988));
#25861=CARTESIAN_POINT('Ctrl Pts',(0.266831636419484,3.06340362899289,103.527664703103));
#25862=CARTESIAN_POINT('Ctrl Pts',(0.362686048388711,3.05354645028764,103.522672578219));
#25863=CARTESIAN_POINT('Ctrl Pts',(0.457968239139363,3.03918859927113,103.517680453334));
#25864=CARTESIAN_POINT('Ctrl Pts',(0.553156462986874,3.02484490790801,103.512693251663));
#25865=CARTESIAN_POINT('Ctrl Pts',(0.647773155437854,3.00600942913244,103.507706049991));
#25866=CARTESIAN_POINT('Ctrl Pts',(0.741364642876875,2.98274717605969,103.50271884832));
#25867=CARTESIAN_POINT('Ctrl Pts',(0.834889386692949,2.95950151217779,103.49773520321));
#25868=CARTESIAN_POINT('Ctrl Pts',(0.927389954212311,2.931835455185,103.492751558101));
#25869=CARTESIAN_POINT('Ctrl Pts',(1.01842244305371,2.89986516539727,103.487767912991));
#25870=CARTESIAN_POINT('Ctrl Pts',(1.10942726221678,2.8679045931032,103.482785782679));
#25871=CARTESIAN_POINT('Ctrl Pts',(1.19896447432909,2.83164252900669,103.477803652368));
#25872=CARTESIAN_POINT('Ctrl Pts',(1.28660578901007,2.79124484660264,103.472821522057));
#25873=CARTESIAN_POINT('Ctrl Pts',(1.37423185213238,2.75085419430334,103.467840258748));
#25874=CARTESIAN_POINT('Ctrl Pts',(1.45996227740941,2.70632954305835,103.462858995439));
#25875=CARTESIAN_POINT('Ctrl Pts',(1.54339036598283,2.65788420142627,103.45787773213));
#25876=CARTESIAN_POINT('Ctrl Pts',(1.62684889623697,2.60942118280259,103.452894651232));
#25877=CARTESIAN_POINT('Ctrl Pts',(1.70800303472105,2.55703484133616,103.447911570334));
#25878=CARTESIAN_POINT('Ctrl Pts',(1.78647284537127,2.50098321120936,103.442928489435));
#25879=CARTESIAN_POINT('Ctrl Pts',(1.81548180357218,2.48026187415033,103.441086328937));
#25880=CARTESIAN_POINT('Ctrl Pts',(1.84412420216451,2.45904003791276,103.439244168439));
#25881=CARTESIAN_POINT('Ctrl Pts',(1.87238193903529,2.43733217358128,103.43740200794));
#25882=CARTESIAN_POINT('Ctrl Pts',(1.8723819390353,2.43733217358127,104.437267724146));
#25883=CARTESIAN_POINT('Ctrl Pts',(1.94887274963103,2.37857119967135,104.432285699447));
#25884=CARTESIAN_POINT('Ctrl Pts',(2.02262578910975,2.31618218202684,104.427303674749));
#25885=CARTESIAN_POINT('Ctrl Pts',(2.09328617694461,2.25045667174745,104.42232165005));
#25886=CARTESIAN_POINT('Ctrl Pts',(2.16394103458939,2.18473630543311,104.417340015266));
#25887=CARTESIAN_POINT('Ctrl Pts',(2.23150340058652,2.11568026483155,104.412358380483));
#25888=CARTESIAN_POINT('Ctrl Pts',(2.29565367489618,2.04361847098123,104.407376745699));
#25889=CARTESIAN_POINT('Ctrl Pts',(2.35981644119198,1.97154264453417,104.402394140841));
#25890=CARTESIAN_POINT('Ctrl Pts',(2.42056550434251,1.89646023024797,104.397411535984));
#25891=CARTESIAN_POINT('Ctrl Pts',(2.47762084770206,1.8187350508065,104.392428931126));
#25892=CARTESIAN_POINT('Ctrl Pts',(2.53473809046188,1.74092554723849,104.387440920635));
#25893=CARTESIAN_POINT('Ctrl Pts',(2.5881533535492,1.66046790932871,104.382452910145));
#25894=CARTESIAN_POINT('Ctrl Pts',(2.63762950377971,1.57775563722359,104.377464899654));
#25895=CARTESIAN_POINT('Ctrl Pts',(2.68713545317714,1.49499354804921,104.372473884916));
#25896=CARTESIAN_POINT('Ctrl Pts',(2.73269735870101,1.40997450756545,104.367482870179));
#25897=CARTESIAN_POINT('Ctrl Pts',(2.77412467651314,1.32311546327631,104.362491855442));
#25898=CARTESIAN_POINT('Ctrl Pts',(2.81561837012091,1.23611725144075,104.357492843986));
#25899=CARTESIAN_POINT('Ctrl Pts',(2.85296407966245,1.14727355392855,104.352493832531));
#25900=CARTESIAN_POINT('Ctrl Pts',(2.88601992722648,1.05701997599461,104.347494821076));
#25901=CARTESIAN_POINT('Ctrl Pts',(2.90364922234982,1.00888607296121,104.344828755772));
#25902=CARTESIAN_POINT('Ctrl Pts',(2.92005921202746,0.96035140393487,104.342162690469));
#25903=CARTESIAN_POINT('Ctrl Pts',(2.93523429559057,0.911483340488959,104.339496625165));
#25904=CARTESIAN_POINT('Ctrl Pts',(2.96369120331487,0.819844044641818,104.334497115672));
#25905=CARTESIAN_POINT('Ctrl Pts',(2.98790245202407,0.726709858047175,104.329497606179));
#25906=CARTESIAN_POINT('Ctrl Pts',(3.0077122975794,0.632510067105379,104.324498096686));
#25907=CARTESIAN_POINT('Ctrl Pts',(3.02749527120502,0.538438057581826,104.319505368996));
#25908=CARTESIAN_POINT('Ctrl Pts',(3.04288861803811,0.443303742409854,104.314512641306));
#25909=CARTESIAN_POINT('Ctrl Pts',(3.05378612035519,0.347552271070138,104.309519913616));
#25910=CARTESIAN_POINT('Ctrl Pts',(3.06467212608201,0.251901815119079,104.304532453128));
#25911=CARTESIAN_POINT('Ctrl Pts',(3.07107166672151,0.155635931143929,104.299544992639));
#25912=CARTESIAN_POINT('Ctrl Pts',(3.07292962245941,0.0592096732929988,
104.294557532151));
#25913=CARTESIAN_POINT('Ctrl Pts',(3.07478624878655,-0.0371475893164126,
104.289573640307));
#25914=CARTESIAN_POINT('Ctrl Pts',(3.07210774185138,-0.133664560059064,
104.284589748464));
#25915=CARTESIAN_POINT('Ctrl Pts',(3.06489092193472,-0.229882332166164,
104.27960585662));
#25916=CARTESIAN_POINT('Ctrl Pts',(3.05767673020514,-0.326065064143557,
104.274623779786));
#25917=CARTESIAN_POINT('Ctrl Pts',(3.04592754210997,-0.421948376693134,
104.269641702953));
#25918=CARTESIAN_POINT('Ctrl Pts',(3.02969224012889,-0.517075603855755,
104.264659626119));
#25919=CARTESIAN_POINT('Ctrl Pts',(3.01345841843328,-0.61219415760705,104.259678003536));
#25920=CARTESIAN_POINT('Ctrl Pts',(2.99273937010984,-0.706556330357332,
104.254696380953));
#25921=CARTESIAN_POINT('Ctrl Pts',(2.96763541861875,-0.79971386893033,104.24971475837));
#25922=CARTESIAN_POINT('Ctrl Pts',(2.94252690278692,-0.892888345185374,
104.24473223004));
#25923=CARTESIAN_POINT('Ctrl Pts',(2.91303201469197,-0.98485732845272,104.23974970171));
#25924=CARTESIAN_POINT('Ctrl Pts',(2.87930114853018,-1.07518702841544,104.23476717338));
#25925=CARTESIAN_POINT('Ctrl Pts',(2.84553392546594,-1.16561409048185,104.229779274619));
#25926=CARTESIAN_POINT('Ctrl Pts',(2.80752176303124,-1.25439792987099,104.224791375858));
#25927=CARTESIAN_POINT('Ctrl Pts',(2.76546341299628,-1.34112429005627,104.219803477097));
#25928=CARTESIAN_POINT('Ctrl Pts',(2.72338021851669,-1.42790188069288,104.214812631916));
#25929=CARTESIAN_POINT('Ctrl Pts',(2.67724628711548,-1.51261918677559,104.209821786735));
#25930=CARTESIAN_POINT('Ctrl Pts',(2.62730555565989,-1.59488801086429,104.204830941553));
#25931=CARTESIAN_POINT('Ctrl Pts',(2.57728411872113,-1.67728978345024,104.19983203104));
#25932=CARTESIAN_POINT('Ctrl Pts',(2.52344384281173,-1.75723480932283,104.194833120527));
#25933=CARTESIAN_POINT('Ctrl Pts',(2.4660710110759,-1.83436529032009,104.189834210014));
#25934=CARTESIAN_POINT('Ctrl Pts',(2.4327626774887,-1.87914411181223,104.186932045803));
#25935=CARTESIAN_POINT('Ctrl Pts',(2.39826444550648,-1.92297492309074,104.184029881592));
#25936=CARTESIAN_POINT('Ctrl Pts',(2.36263808832369,-1.96579335475583,104.181127717381));
#25937=CARTESIAN_POINT('Ctrl Pts',(2.30126516178033,-2.0395559470916,104.176128207888));
#25938=CARTESIAN_POINT('Ctrl Pts',(2.23632677673238,-2.11057120900105,104.171128698395));
#25939=CARTESIAN_POINT('Ctrl Pts',(2.16809822016109,-2.17847477785131,104.166129188902));
#25940=CARTESIAN_POINT('Ctrl Pts',(2.09996221519368,-2.24628623594147,104.161136461212));
#25941=CARTESIAN_POINT('Ctrl Pts',(2.02854521728431,-2.31099408291181,104.156143733522));
#25942=CARTESIAN_POINT('Ctrl Pts',(1.95416278397776,-2.37226686182568,104.151151005832));
#25943=CARTESIAN_POINT('Ctrl Pts',(1.87985882226302,-2.43347499950262,104.146163545344));
#25944=CARTESIAN_POINT('Ctrl Pts',(1.80259598134922,-2.49125499562497,104.141176084855));
#25945=CARTESIAN_POINT('Ctrl Pts',(1.72272594707639,-2.54531286117635,104.136188624367));
#25946=CARTESIAN_POINT('Ctrl Pts',(1.64291306168037,-2.59933204706112,104.131204732523));
#25947=CARTESIAN_POINT('Ctrl Pts',(1.56049705395011,-2.64963415149563,104.12622084068));
#25948=CARTESIAN_POINT('Ctrl Pts',(1.47586112013985,-2.69596665484934,104.121236948836));
#25949=CARTESIAN_POINT('Ctrl Pts',(1.39125600864048,-2.74228228505286,104.116254872002));
#25950=CARTESIAN_POINT('Ctrl Pts',(1.30443296199666,-2.78463097591669,104.111272795169));
#25951=CARTESIAN_POINT('Ctrl Pts',(1.21580164223415,-2.82280509719335,104.106290718335));
#25952=CARTESIAN_POINT('Ctrl Pts',(1.12717840360608,-2.86097573786962,104.101309095752));
#25953=CARTESIAN_POINT('Ctrl Pts',(1.03674762288719,-2.89497239223644,104.096327473169));
#25954=CARTESIAN_POINT('Ctrl Pts',(0.944939912648046,-2.92463515869667,
104.091345850586));
#25955=CARTESIAN_POINT('Ctrl Pts',(0.853115510149806,-2.95430331837041,
104.086363322256));
#25956=CARTESIAN_POINT('Ctrl Pts',(0.759914098643544,-2.97963589029097,
104.081380793926));
#25957=CARTESIAN_POINT('Ctrl Pts',(0.665781420455429,-3.00052284613471,
104.076398265596));
#25958=CARTESIAN_POINT('Ctrl Pts',(0.571547281113173,-3.02143231503861,
104.071410366835));
#25959=CARTESIAN_POINT('Ctrl Pts',(0.476380300408673,-3.03788650639572,
104.066422468074));
#25960=CARTESIAN_POINT('Ctrl Pts',(0.380736164232095,-3.049826589045,104.061434569313));
#25961=CARTESIAN_POINT('Ctrl Pts',(0.285035529751468,-3.06177372486498,
104.056443724132));
#25962=CARTESIAN_POINT('Ctrl Pts',(0.188857616019592,-3.06920140866425,
104.051452878951));
#25963=CARTESIAN_POINT('Ctrl Pts',(0.0926608518625408,-3.07210289810288,
104.046462033769));
#25964=CARTESIAN_POINT('Ctrl Pts',(-0.00369136869463417,-3.07500907642171,
104.041463123256));
#25965=CARTESIAN_POINT('Ctrl Pts',(-0.100062061900924,-3.07337446249044,
104.036464212743));
#25966=CARTESIAN_POINT('Ctrl Pts',(-0.195995242113639,-3.067244384634,104.03146530223));
#25967=CARTESIAN_POINT('Ctrl Pts',(-0.251690146338518,-3.06368551065163,
104.028563138019));
#25968=CARTESIAN_POINT('Ctrl Pts',(-0.307237708948579,-3.05861241343464,
104.025660973808));
#25969=CARTESIAN_POINT('Ctrl Pts',(-0.362550304875721,-3.05204186184176,
104.022758809597));
#25970=CARTESIAN_POINT('Ctrl Pts',(-0.457836383924149,-3.04072288308156,
104.017759300104));
#25971=CARTESIAN_POINT('Ctrl Pts',(-0.552759242854784,-3.02491743689527,
104.012759790611));
#25972=CARTESIAN_POINT('Ctrl Pts',(-0.646863376675473,-3.00465805407471,
104.007760281118));
#25973=CARTESIAN_POINT('Ctrl Pts',(-0.740839858836012,-2.98442615297834,
104.002767553428));
#25974=CARTESIAN_POINT('Ctrl Pts',(-0.833999397662042,-2.95975241439547,
103.997774825738));
#25975=CARTESIAN_POINT('Ctrl Pts',(-0.925892163834386,-2.93072106331361,
103.992782098048));
#25976=CARTESIAN_POINT('Ctrl Pts',(-1.01768798545516,-2.90172033957523,
103.98779463756));
#25977=CARTESIAN_POINT('Ctrl Pts',(-1.10821927478628,-2.86837127377104,
103.982807177071));
#25978=CARTESIAN_POINT('Ctrl Pts',(-1.19704796020428,-2.83080879449156,
103.977819716583));
#25979=CARTESIAN_POINT('Ctrl Pts',(-1.28581308662117,-2.79327319204417,
103.972835824739));
#25980=CARTESIAN_POINT('Ctrl Pts',(-1.37287762781264,-2.75153033986734,
103.967851932896));
#25981=CARTESIAN_POINT('Ctrl Pts',(-1.45782114046193,-2.70576417531578,
103.962868041052));
#25982=CARTESIAN_POINT('Ctrl Pts',(-1.54273371878766,-2.66001467766788,
103.957885964218));
#25983=CARTESIAN_POINT('Ctrl Pts',(-1.62552641725117,-2.61024498681573,
103.952903887385));
#25984=CARTESIAN_POINT('Ctrl Pts',(-1.70580203607325,-2.55668567949374,
103.947921810551));
#25985=CARTESIAN_POINT('Ctrl Pts',(-1.78607033560831,-2.50313125554665,
103.942940187968));
#25986=CARTESIAN_POINT('Ctrl Pts',(-1.86382164674154,-2.44578814587672,
103.937958565385));
#25987=CARTESIAN_POINT('Ctrl Pts',(-1.93868739756062,-2.38493048631184,
103.932976942802));
#25988=CARTESIAN_POINT('Ctrl Pts',(-2.01356676029249,-2.32406176175202,
103.927994414472));
#25989=CARTESIAN_POINT('Ctrl Pts',(-2.08555918016921,-2.25967749513936,
103.923011886142));
#25990=CARTESIAN_POINT('Ctrl Pts',(-2.15432968117646,-2.1920916666057,103.918029357812));
#25991=CARTESIAN_POINT('Ctrl Pts',(-2.22317430664848,-2.12443299050959,
103.913041459051));
#25992=CARTESIAN_POINT('Ctrl Pts',(-2.28878976662176,-2.05356617146032,
103.90805356029));
#25993=CARTESIAN_POINT('Ctrl Pts',(-2.35087861507805,-1.97984140454954,
103.903065661529));
#25994=CARTESIAN_POINT('Ctrl Pts',(-2.41300414026913,-1.90607308740727,
103.898074816348));
#25995=CARTESIAN_POINT('Ctrl Pts',(-2.47159863940539,-1.82944380940346,
103.893083971167));
#25996=CARTESIAN_POINT('Ctrl Pts',(-2.52640686477412,-1.75033442622323,
103.888093125985));
#25997=CARTESIAN_POINT('Ctrl Pts',(-2.5813036616193,-1.67109720028177,103.883094215472));
#25998=CARTESIAN_POINT('Ctrl Pts',(-2.6324017344191,-1.58937223819583,103.878095304959));
#25999=CARTESIAN_POINT('Ctrl Pts',(-2.67949084212781,-1.5055666962819,103.873096394446));
#26000=CARTESIAN_POINT('Ctrl Pts',(-2.70682886363425,-1.45691260579936,
103.870194230235));
#26001=CARTESIAN_POINT('Ctrl Pts',(-2.73281654600128,-1.40755768312279,
103.867292066024));
#26002=CARTESIAN_POINT('Ctrl Pts',(-2.75742024721313,-1.3575845573146,103.864389901813));
#26003=CARTESIAN_POINT('Ctrl Pts',(-2.80284919410827,-1.26531281092261,
103.859031266432));
#26004=CARTESIAN_POINT('Ctrl Pts',(-2.84369889987435,-1.17064478182644,
103.853672631051));
#26005=CARTESIAN_POINT('Ctrl Pts',(-2.87972873844127,-1.07404126689594,
103.84831399567));
#26006=CARTESIAN_POINT('Ctrl Pts',(-2.91564169345326,-0.977751141164306,
103.842972744112));
#26007=CARTESIAN_POINT('Ctrl Pts',(-2.94676582982252,-0.879538363778252,
103.837631492554));
#26008=CARTESIAN_POINT('Ctrl Pts',(-2.97290811057071,-0.779884360724638,
103.832290240997));
#26009=CARTESIAN_POINT('Ctrl Pts',(-2.99899763374524,-0.680431468792797,
103.826959768586));
#26010=CARTESIAN_POINT('Ctrl Pts',(-3.02012523611837,-0.579543470887511,
103.821629296174));
#26011=CARTESIAN_POINT('Ctrl Pts',(-3.03614664061705,-0.477719401604962,
103.816298823763));
#26012=CARTESIAN_POINT('Ctrl Pts',(-3.05212172792721,-0.376189701309465,
103.810983761518));
#26013=CARTESIAN_POINT('Ctrl Pts',(-3.06301998403236,-0.273729658401492,
103.805668699272));
#26014=CARTESIAN_POINT('Ctrl Pts',(-3.06874773143845,-0.170849673079425,
103.800353637026));
#26015=CARTESIAN_POINT('Ctrl Pts',(-3.0719005901615,-0.114219022990934,
103.797427942303));
#26016=CARTESIAN_POINT('Ctrl Pts',(-3.0734876697023,-0.057461379173942,
103.794502247579));
#26017=CARTESIAN_POINT('Ctrl Pts',(-3.07349992841428,-0.0006633531664633,
103.791576552855));
#26018=CARTESIAN_POINT('Origin',(0.,0.,116.208423447177));
#26019=CARTESIAN_POINT('',(1.87238193903528,2.43733217358128,105.437268236956));
#26020=CARTESIAN_POINT('',(1.87238193903528,2.43733217358129,105.354223092666));
#26021=CARTESIAN_POINT('',(1.8723819390353,2.43733217358128,116.208423447177));
#26022=CARTESIAN_POINT('',(-3.07349891831708,0.00257858561311968,104.70842344715));
#26023=CARTESIAN_POINT('Ctrl Pts',(1.87238193903529,2.43733217358128,105.354223092666));
#26024=CARTESIAN_POINT('Ctrl Pts',(1.94945953133495,2.37812042834175,105.349202752108));
#26025=CARTESIAN_POINT('Ctrl Pts',(2.02369320136329,2.3152738620541,105.34418241155));
#26026=CARTESIAN_POINT('Ctrl Pts',(2.09473553780151,2.24910766231219,105.339162070992));
#26027=CARTESIAN_POINT('Ctrl Pts',(2.16534023155336,2.18334906675188,105.334172657279));
#26028=CARTESIAN_POINT('Ctrl Pts',(2.23279253492672,2.11431198189643,105.329183243567));
#26029=CARTESIAN_POINT('Ctrl Pts',(2.29678984415326,2.04234146552296,105.324193829854));
#26030=CARTESIAN_POINT('Ctrl Pts',(2.36138218367118,1.96970178605737,105.319158025873));
#26031=CARTESIAN_POINT('Ctrl Pts',(2.42245466520873,1.89407420271472,105.314122221893));
#26032=CARTESIAN_POINT('Ctrl Pts',(2.47973990076263,1.8158447826193,105.309086417912));
#26033=CARTESIAN_POINT('Ctrl Pts',(2.53702513631653,1.73761536252389,105.304050613932));
#26034=CARTESIAN_POINT('Ctrl Pts',(2.59052292778912,1.65678451783041,105.299014809952));
#26035=CARTESIAN_POINT('Ctrl Pts',(2.64001321119421,1.57376379889741,105.293979005971));
#26036=CARTESIAN_POINT('Ctrl Pts',(2.68914680389491,1.49134143415999,105.288979496478));
#26037=CARTESIAN_POINT('Ctrl Pts',(2.73450310331458,1.40647113676653,105.283979986985));
#26038=CARTESIAN_POINT('Ctrl Pts',(2.77583012931114,1.31953375978355,105.278980477492));
#26039=CARTESIAN_POINT('Ctrl Pts',(2.8171010954593,1.23271431280053,105.273987749802));
#26040=CARTESIAN_POINT('Ctrl Pts',(2.85435346402324,1.14383375201073,105.268995022112));
#26041=CARTESIAN_POINT('Ctrl Pts',(2.8873796867055,1.0532999548089,105.264002294422));
#26042=CARTESIAN_POINT('Ctrl Pts',(2.92037106755534,0.962861668480981,105.259014833934));
#26043=CARTESIAN_POINT('Ctrl Pts',(2.94914501607307,0.870774023139204,105.254027373445));
#26044=CARTESIAN_POINT('Ctrl Pts',(2.97354133946183,0.777466496070115,105.249039912957));
#26045=CARTESIAN_POINT('Ctrl Pts',(2.99792020671094,0.684225732717753,105.244056021114));
#26046=CARTESIAN_POINT('Ctrl Pts',(3.01792756496112,0.58976724629874,105.23907212927));
#26047=CARTESIAN_POINT('Ctrl Pts',(3.03345281349624,0.494536427669112,105.234088237426));
#26048=CARTESIAN_POINT('Ctrl Pts',(3.04897240812038,0.399340289744977,105.229106160593));
#26049=CARTESIAN_POINT('Ctrl Pts',(3.06001306562101,0.303372811251732,105.224124083759));
#26050=CARTESIAN_POINT('Ctrl Pts',(3.06651532359486,0.20708940136545,105.219142006925));
#26051=CARTESIAN_POINT('Ctrl Pts',(3.07301698871259,0.110814770307922,105.214160384342));
#26052=CARTESIAN_POINT('Ctrl Pts',(3.07498104761558,0.0142247031053793,
105.209178761759));
#26053=CARTESIAN_POINT('Ctrl Pts',(3.07240001820998,-0.0822215184931722,
105.204197139176));
#26054=CARTESIAN_POINT('Ctrl Pts',(3.06981851952776,-0.178685275714061,
105.199214610846));
#26055=CARTESIAN_POINT('Ctrl Pts',(3.06269030312906,-0.275004696589989,
105.194232082516));
#26056=CARTESIAN_POINT('Ctrl Pts',(3.05105995248765,-0.370722829518265,
105.189249554186));
#26057=CARTESIAN_POINT('Ctrl Pts',(3.03941706604231,-0.466544132487117,
105.184261655425));
#26058=CARTESIAN_POINT('Ctrl Pts',(3.02326241054735,-0.561762417156996,
105.179273756664));
#26059=CARTESIAN_POINT('Ctrl Pts',(3.00269215754031,-0.655928393230473,
105.174285857903));
#26060=CARTESIAN_POINT('Ctrl Pts',(2.98210975340248,-0.750149994438522,
105.169295012722));
#26061=CARTESIAN_POINT('Ctrl Pts',(2.95710667181709,-0.84331762555405,105.164304167541));
#26062=CARTESIAN_POINT('Ctrl Pts',(2.92782911689693,-0.934996744513346,
105.159313322359));
#26063=CARTESIAN_POINT('Ctrl Pts',(2.89850424870867,-1.02682401924407,105.154314411846));
#26064=CARTESIAN_POINT('Ctrl Pts',(2.86489126710132,-1.117157567493,105.149315501333));
#26065=CARTESIAN_POINT('Ctrl Pts',(2.82718466573472,-1.20558247989693,105.14431659082));
#26066=CARTESIAN_POINT('Ctrl Pts',(2.80529374596009,-1.25691838908413,105.141414426609));
#26067=CARTESIAN_POINT('Ctrl Pts',(2.78202394842517,-1.30761143150604,105.138512262398));
#26068=CARTESIAN_POINT('Ctrl Pts',(2.75742024721298,-1.35758455731491,105.135610098187));
#26069=CARTESIAN_POINT('Ctrl Pts',(2.71503586478997,-1.44367242096148,105.130610588694));
#26070=CARTESIAN_POINT('Ctrl Pts',(2.66854162211707,-1.52792470090094,105.125611079201));
#26071=CARTESIAN_POINT('Ctrl Pts',(2.61811978482655,-1.6099226820875,105.120611569708));
#26072=CARTESIAN_POINT('Ctrl Pts',(2.56776634443807,-1.69180943353335,105.115618842018));
#26073=CARTESIAN_POINT('Ctrl Pts',(2.51349612596166,-1.77144759295787,105.110626114328));
#26074=CARTESIAN_POINT('Ctrl Pts',(2.45553825381476,-1.84844100096605,105.105633386638));
#26075=CARTESIAN_POINT('Ctrl Pts',(2.39764152576222,-1.9253531828693,105.10064592615));
#26076=CARTESIAN_POINT('Ctrl Pts',(2.33606514047656,-1.99962581115889,105.095658465661));
#26077=CARTESIAN_POINT('Ctrl Pts',(2.2710821229741,-2.07089068777361,105.090671005173));
#26078=CARTESIAN_POINT('Ctrl Pts',(2.20614560233962,-2.14210457270332,105.085687113329));
#26079=CARTESIAN_POINT('Ctrl Pts',(2.13780759009278,-2.21031466083467,105.080703221486));
#26080=CARTESIAN_POINT('Ctrl Pts',(2.06638145991496,-2.27518568739339,105.075719329642));
#26081=CARTESIAN_POINT('Ctrl Pts',(1.99498134136481,-2.34003308953083,105.070737252808));
#26082=CARTESIAN_POINT('Ctrl Pts',(1.92049566398737,-2.40154355134022,105.065755175975));
#26083=CARTESIAN_POINT('Ctrl Pts',(1.84327404708782,-2.45941924797959,105.060773099141));
#26084=CARTESIAN_POINT('Ctrl Pts',(1.76605947102081,-2.51728966768868,105.055791476558));
#26085=CARTESIAN_POINT('Ctrl Pts',(1.68610980276192,-2.57152571801325,105.050809853975));
#26086=CARTESIAN_POINT('Ctrl Pts',(1.60380621066126,-2.62187106636547,105.045828231392));
#26087=CARTESIAN_POINT('Ctrl Pts',(1.52148765431711,-2.67222556838925,105.040845703062));
#26088=CARTESIAN_POINT('Ctrl Pts',(1.43681469862724,-2.71868773452121,105.035863174732));
#26089=CARTESIAN_POINT('Ctrl Pts',(1.35019490461258,-2.76104617302178,105.030880646402));
#26090=CARTESIAN_POINT('Ctrl Pts',(1.26348174722592,-2.80345026767631,105.025892747641));
#26091=CARTESIAN_POINT('Ctrl Pts',(1.17481795723416,-2.84174161100527,105.02090484888));
#26092=CARTESIAN_POINT('Ctrl Pts',(1.08463275661632,-2.87575625414862,105.015916950119));
#26093=CARTESIAN_POINT('Ctrl Pts',(0.994394282362713,-2.90979099020851,
105.010926104938));
#26094=CARTESIAN_POINT('Ctrl Pts',(0.902633025354364,-2.93954386046796,
105.005935259757));
#26095=CARTESIAN_POINT('Ctrl Pts',(0.809793077179332,-2.9649009127039,105.000944414575));
#26096=CARTESIAN_POINT('Ctrl Pts',(0.716803097303502,-2.99029894257662,
104.995945504062));
#26097=CARTESIAN_POINT('Ctrl Pts',(0.622731373631855,-3.01128687428064,
104.990946593549));
#26098=CARTESIAN_POINT('Ctrl Pts',(0.528031821313986,-3.02780194954687,
104.985947683036));
#26099=CARTESIAN_POINT('Ctrl Pts',(0.473053111291294,-3.03738993081861,
104.983045518825));
#26100=CARTESIAN_POINT('Ctrl Pts',(0.417862900802648,-3.04547131024891,
104.980143354614));
#26101=CARTESIAN_POINT('Ctrl Pts',(0.362550304875634,-3.05204186184177,
104.977241190403));
#26102=CARTESIAN_POINT('Ctrl Pts',(0.267264225827233,-3.06336084060196,
104.97224168091));
#26103=CARTESIAN_POINT('Ctrl Pts',(0.171280200402446,-3.07023311387662,
104.967242171417));
#26104=CARTESIAN_POINT('Ctrl Pts',(0.0750486783593991,-3.07258359461163,
104.962242661924));
#26105=CARTESIAN_POINT('Ctrl Pts',(-0.0210523062352704,-3.07493088693445,
104.957249934234));
#26106=CARTESIAN_POINT('Ctrl Pts',(-0.117399685134141,-3.07276856657818,
104.952257206544));
#26107=CARTESIAN_POINT('Ctrl Pts',(-0.213536415746227,-3.06607313173549,
104.947264478854));
#26108=CARTESIAN_POINT('Ctrl Pts',(-0.309571724530516,-3.0593847604078,
104.942277018366));
#26109=CARTESIAN_POINT('Ctrl Pts',(-0.405396391232003,-3.04817281189546,
104.937289557877));
#26110=CARTESIAN_POINT('Ctrl Pts',(-0.500552925261181,-3.03246583146661,
104.932302097389));
#26111=CARTESIAN_POINT('Ctrl Pts',(-0.595641372565858,-3.01677008974942,
104.927318205546));
#26112=CARTESIAN_POINT('Ctrl Pts',(-0.690062205708036,-2.99658578125377,
104.922334313702));
#26113=CARTESIAN_POINT('Ctrl Pts',(-0.783363590391523,-2.97199322597628,
104.917350421858));
#26114=CARTESIAN_POINT('Ctrl Pts',(-0.876630997021813,-2.94740962669825,
104.912368345025));
#26115=CARTESIAN_POINT('Ctrl Pts',(-0.968779341168995,-2.91842108210969,
104.907386268191));
#26116=CARTESIAN_POINT('Ctrl Pts',(-1.05936845887682,-2.88515869898641,
104.902404191357));
#26117=CARTESIAN_POINT('Ctrl Pts',(-1.14994931694398,-2.85189934862622,
104.897422568774));
#26118=CARTESIAN_POINT('Ctrl Pts',(-1.23897081922333,-2.81436708595139,
104.892440946191));
#26119=CARTESIAN_POINT('Ctrl Pts',(-1.32601042821453,-2.77274207135578,
104.887459323608));
#26120=CARTESIAN_POINT('Ctrl Pts',(-1.41306586254063,-2.73110948859891,
104.882476795278));
#26121=CARTESIAN_POINT('Ctrl Pts',(-1.49813829194838,-2.6853828654822,104.877494266948));
#26122=CARTESIAN_POINT('Ctrl Pts',(-1.58082850544345,-2.63578896848314,
104.872511738619));
#26123=CARTESIAN_POINT('Ctrl Pts',(-1.66360784680152,-2.58614161657243,
104.867523839858));
#26124=CARTESIAN_POINT('Ctrl Pts',(-1.7439994690437,-2.53261889520195,104.862535941096));
#26125=CARTESIAN_POINT('Ctrl Pts',(-1.82163216255449,-2.47549157024359,
104.857548042335));
#26126=CARTESIAN_POINT('Ctrl Pts',(-1.89931071476291,-2.41833049939025,
104.852557197154));
#26127=CARTESIAN_POINT('Ctrl Pts',(-1.97422675241966,-2.35756086159102,
104.847566351973));
#26128=CARTESIAN_POINT('Ctrl Pts',(-2.04604290692081,-2.29349311597813,
104.842575506792));
#26129=CARTESIAN_POINT('Ctrl Pts',(-2.11797511814123,-2.2293218352704,104.837576596278));
#26130=CARTESIAN_POINT('Ctrl Pts',(-2.18679713013914,-2.1618421113799,104.832577685765));
#26131=CARTESIAN_POINT('Ctrl Pts',(-2.25220916695079,-2.09140051599469,
104.827578775252));
#26132=CARTESIAN_POINT('Ctrl Pts',(-2.29018473616726,-2.05050498954941,
104.824676611041));
#26133=CARTESIAN_POINT('Ctrl Pts',(-2.32701173114118,-2.00861178642058,
104.82177444683));
#26134=CARTESIAN_POINT('Ctrl Pts',(-2.36263808832381,-1.96579335475569,
104.818872282619));
#26135=CARTESIAN_POINT('Ctrl Pts',(-2.42366151100837,-1.89245082240576,
104.813901244114));
#26136=CARTESIAN_POINT('Ctrl Pts',(-2.48138149360842,-1.81612585312949,
104.808930205609));
#26137=CARTESIAN_POINT('Ctrl Pts',(-2.53549054025688,-1.73714995618337,
104.803959167104));
#26138=CARTESIAN_POINT('Ctrl Pts',(-2.58953001315165,-1.658275606944,104.798994520392));
#26139=CARTESIAN_POINT('Ctrl Pts',(-2.63996752204625,-1.57675746166274,
104.79402987368));
#26140=CARTESIAN_POINT('Ctrl Pts',(-2.68653487203633,-1.49296102806896,
104.789065226968));
#26141=CARTESIAN_POINT('Ctrl Pts',(-2.73305541744705,-1.40924881779533,
104.784105570194));
#26142=CARTESIAN_POINT('Ctrl Pts',(-2.77571331674056,-1.32326325384198,
104.77914591342));
#26143=CARTESIAN_POINT('Ctrl Pts',(-2.81428353238982,-1.23539890291333,
104.774186256646));
#26144=CARTESIAN_POINT('Ctrl Pts',(-2.85282580546769,-1.14759820617634,
104.769230192944));
#26145=CARTESIAN_POINT('Ctrl Pts',(-2.88728610213059,-1.05792183275072,
104.764274129242));
#26146=CARTESIAN_POINT('Ctrl Pts',(-2.91748575996682,-0.966788027641428,
104.75931806554));
#26147=CARTESIAN_POINT('Ctrl Pts',(-2.94767654771691,-0.875680989878505,
104.754363457507));
#26148=CARTESIAN_POINT('Ctrl Pts',(-2.97360903798759,-0.783117790220548,
104.749408849474));
#26149=CARTESIAN_POINT('Ctrl Pts',(-2.99515341736076,-0.689534811646325,
104.744454241442));
#26150=CARTESIAN_POINT('Ctrl Pts',(-3.01669409614081,-0.595967907451499,
104.739500484442));
#26151=CARTESIAN_POINT('Ctrl Pts',(-3.03384806794806,-0.50138200653861,
104.734546727443));
#26152=CARTESIAN_POINT('Ctrl Pts',(-3.04653625570149,-0.406225421036614,
104.729592970444));
#26153=CARTESIAN_POINT('Ctrl Pts',(-3.05922958420412,-0.311030281869517,
104.724637206379));
#26154=CARTESIAN_POINT('Ctrl Pts',(-3.06745346148863,-0.215264437470324,
104.719681442315));
#26155=CARTESIAN_POINT('Ctrl Pts',(-3.07118057186357,-0.119382347973822,
104.71472567825));
#26156=CARTESIAN_POINT('Ctrl Pts',(-3.07276049041973,-0.0787380210932937,
104.712624934559));
#26157=CARTESIAN_POINT('Ctrl Pts',(-3.07353302379519,-0.0380728361124389,
104.710524190868));
#26158=CARTESIAN_POINT('Ctrl Pts',(-3.07349891831751,0.00257858509384388,
104.708423447177));
#26159=CARTESIAN_POINT('Ctrl Pts',(-3.07349891831708,0.00257858561313954,
104.70842344715));
#26160=CARTESIAN_POINT('Ctrl Pts',(-3.07340190154726,0.11821598603669,104.702447652648));
#26161=CARTESIAN_POINT('Ctrl Pts',(-3.06677494859755,0.233572640495253,
104.696471858145));
#26162=CARTESIAN_POINT('Ctrl Pts',(-3.05373569317267,0.347995066406445,
104.690496063642));
#26163=CARTESIAN_POINT('Ctrl Pts',(-3.04052691899684,0.463905057833428,
104.684442579947));
#26164=CARTESIAN_POINT('Ctrl Pts',(-3.02073810232729,0.578856352949399,
104.678389096252));
#26165=CARTESIAN_POINT('Ctrl Pts',(-2.99454061664833,0.692191263483916,
104.672335612557));
#26166=CARTESIAN_POINT('Ctrl Pts',(-2.97747193939876,0.766033350191337,
104.668391533316));
#26167=CARTESIAN_POINT('Ctrl Pts',(-2.95768375771646,0.839189719506165,
104.664447454075));
#26168=CARTESIAN_POINT('Ctrl Pts',(-2.93523429559051,0.911483340489175,
104.660503374835));
#26169=CARTESIAN_POINT('Ctrl Pts',(-2.90677738786623,1.00312263633624,104.655503865342));
#26170=CARTESIAN_POINT('Ctrl Pts',(-2.87397485611257,1.09358895707076,104.650504355849));
#26171=CARTESIAN_POINT('Ctrl Pts',(-2.83694151691682,1.18244030698961,104.645504846356));
#26172=CARTESIAN_POINT('Ctrl Pts',(-2.7999584132105,1.27117113061657,104.640512118666));
#26173=CARTESIAN_POINT('Ctrl Pts',(-2.75875607550427,1.35829093558367,104.635519390975));
#26174=CARTESIAN_POINT('Ctrl Pts',(-2.71349912070783,1.4433727072097,104.630526663285));
#26175=CARTESIAN_POINT('Ctrl Pts',(-2.66828991085796,1.52836471971121,104.625539202797));
#26176=CARTESIAN_POINT('Ctrl Pts',(-2.61903479241562,1.61132258760283,104.620551742309));
#26177=CARTESIAN_POINT('Ctrl Pts',(-2.56594610259187,1.69184007772413,104.615564281821));
#26178=CARTESIAN_POINT('Ctrl Pts',(-2.51289539896664,1.77229995569914,104.610580389977));
#26179=CARTESIAN_POINT('Ctrl Pts',(-2.45601681787269,1.85032256174038,104.605596498133));
#26180=CARTESIAN_POINT('Ctrl Pts',(-2.39556768273871,1.92552790876109,104.60061260629));
#26181=CARTESIAN_POINT('Ctrl Pts',(-2.33514056168258,2.00070586785708,104.595630529456));
#26182=CARTESIAN_POINT('Ctrl Pts',(-2.27114574488193,2.0730682646461,104.590648452622));
#26183=CARTESIAN_POINT('Ctrl Pts',(-2.20388219103734,2.14226644888736,104.585666375788));
#26184=CARTESIAN_POINT('Ctrl Pts',(-2.13662477007921,2.21145832384844,104.580684753205));
#26185=CARTESIAN_POINT('Ctrl Pts',(-2.06609951071634,2.27748624522545,104.575703130622));
#26186=CARTESIAN_POINT('Ctrl Pts',(-1.99264299891211,2.34003763407484,104.570721508039));
#26187=CARTESIAN_POINT('Ctrl Pts',(-1.91917313141978,2.40260039586882,104.565738979709));
#26188=CARTESIAN_POINT('Ctrl Pts',(-1.84277128726752,2.4616850852312,104.560756451379));
#26189=CARTESIAN_POINT('Ctrl Pts',(-1.763807123446,2.51701940423214,104.55577392305));
#26190=CARTESIAN_POINT('Ctrl Pts',(-1.68475784789349,2.5724133654739,104.550786024289));
#26191=CARTESIAN_POINT('Ctrl Pts',(-1.6031410990681,2.62404863385521,104.545798125528));
#26192=CARTESIAN_POINT('Ctrl Pts',(-1.51935532078173,2.67169640101795,104.540810226766));
#26193=CARTESIAN_POINT('Ctrl Pts',(-1.43552004908622,2.71937231437069,104.535819381585));
#26194=CARTESIAN_POINT('Ctrl Pts',(-1.34951358789181,2.76305583768599,104.530828536404));
#26195=CARTESIAN_POINT('Ctrl Pts',(-1.26175685718869,2.80256523266405,104.525837691223));
#26196=CARTESIAN_POINT('Ctrl Pts',(-1.17385830939251,2.84213847582219,104.520838780709));
#26197=CARTESIAN_POINT('Ctrl Pts',(-1.08420425227333,2.8775239603299,104.515839870196));
#26198=CARTESIAN_POINT('Ctrl Pts',(-0.993233284057695,2.90858898668065,
104.510840959683));
#26199=CARTESIAN_POINT('Ctrl Pts',(-0.940419238377377,2.92662407801726,
104.507938795472));
#26200=CARTESIAN_POINT('Ctrl Pts',(-0.887161587446126,2.94320390445115,
104.505036631261));
#26201=CARTESIAN_POINT('Ctrl Pts',(-0.833547700173576,2.95831040993594,
104.50213446705));
#26202=CARTESIAN_POINT('Ctrl Pts',(-0.741183834711446,2.98433529474063,
104.497134734362));
#26203=CARTESIAN_POINT('Ctrl Pts',(-0.647437746391747,3.00607609265561,
104.492135001674));
#26204=CARTESIAN_POINT('Ctrl Pts',(-0.55274274831966,3.02338844745098,104.487135268986));
#26205=CARTESIAN_POINT('Ctrl Pts',(-0.458177294599245,3.04067711865351,
104.482142376016));
#26206=CARTESIAN_POINT('Ctrl Pts',(-0.362665939390717,3.05354930928601,
104.477149483047));
#26207=CARTESIAN_POINT('Ctrl Pts',(-0.266656530519557,3.06191060364787,
104.472156590077));
#26208=CARTESIAN_POINT('Ctrl Pts',(-0.170760147999297,3.07026205473915,
104.467169574953));
#26209=CARTESIAN_POINT('Ctrl Pts',(-0.0743673130760004,3.07411313495795,
104.462182559829));
#26210=CARTESIAN_POINT('Ctrl Pts',(0.0220657436718747,3.0734207900898,104.457195544705));
#26211=CARTESIAN_POINT('Ctrl Pts',(0.1184357663145,3.07272889777745,104.452211789376));
#26212=CARTESIAN_POINT('Ctrl Pts',(0.214845520986163,3.067499483887,104.447228034047));
#26213=CARTESIAN_POINT('Ctrl Pts',(0.310836215005677,3.05774150271748,104.442244278719));
#26214=CARTESIAN_POINT('Ctrl Pts',(0.40679036992339,3.0479872359483,104.437262420469));
#26215=CARTESIAN_POINT('Ctrl Pts',(0.502325345044623,3.03370787233216,104.43228056222));
#26216=CARTESIAN_POINT('Ctrl Pts',(0.596985986216576,3.01496434178931,104.42729870397));
#26217=CARTESIAN_POINT('Ctrl Pts',(0.691636436486133,2.99622282912303,104.422317382054));
#26218=CARTESIAN_POINT('Ctrl Pts',(0.785412309697513,2.97301819146454,104.417336060137));
#26219=CARTESIAN_POINT('Ctrl Pts',(0.877868241469313,2.94546254442652,104.412354738221));
#26220=CARTESIAN_POINT('Ctrl Pts',(0.970389740926265,2.91788735553809,104.407369883662));
#26221=CARTESIAN_POINT('Ctrl Pts',(1.06158900682457,2.88595511628965,104.402385029103));
#26222=CARTESIAN_POINT('Ctrl Pts',(1.15103577723119,2.84982787015879,104.397400174544));
#26223=CARTESIAN_POINT('Ctrl Pts',(1.24051289750611,2.81368836581942,104.392413628592));
#26224=CARTESIAN_POINT('Ctrl Pts',(1.3282359367672,2.77335119885068,104.387427082639));
#26225=CARTESIAN_POINT('Ctrl Pts',(1.41379637619271,2.72902584389821,104.382440536687));
#26226=CARTESIAN_POINT('Ctrl Pts',(1.49947820590929,2.68463760161399,104.37744691599));
#26227=CARTESIAN_POINT('Ctrl Pts',(1.58299092297891,2.63625008317744,104.372453295293));
#26228=CARTESIAN_POINT('Ctrl Pts',(1.66395228944447,2.58411784337567,104.367459674596));
#26229=CARTESIAN_POINT('Ctrl Pts',(1.73550200378447,2.53804590772833,104.363046555722));
#26230=CARTESIAN_POINT('Ctrl Pts',(1.80505932822455,2.48905004853368,104.358633436849));
#26231=CARTESIAN_POINT('Ctrl Pts',(1.87238193903531,2.43733217358127,104.354220317975));
#26232=CARTESIAN_POINT('',(-3.07349915681862,-0.00227662804431954,104.791576552792));
#26233=CARTESIAN_POINT('Ctrl Pts',(-3.07349915681862,-0.00227662804430111,
104.791576552792));
#26234=CARTESIAN_POINT('Ctrl Pts',(-3.07356931928976,0.0924442889047205,
104.786655194444));
#26235=CARTESIAN_POINT('Ctrl Pts',(-3.06925653593697,0.187328717419588,
104.781733836096));
#26236=CARTESIAN_POINT('Ctrl Pts',(-3.06054199775665,0.281930718382627,
104.776812477748));
#26237=CARTESIAN_POINT('Ctrl Pts',(-3.05164555568275,0.378507404860657,
104.771788392872));
#26238=CARTESIAN_POINT('Ctrl Pts',(-3.03816145777448,0.474789267800039,
104.766764307997));
#26239=CARTESIAN_POINT('Ctrl Pts',(-3.02012579510685,0.570300299605607,
104.761740223121));
#26240=CARTESIAN_POINT('Ctrl Pts',(-3.00249201978596,0.663683066103453,
104.75682808956));
#26241=CARTESIAN_POINT('Ctrl Pts',(-2.98050749991343,0.756328525787592,
104.751915955999));
#26242=CARTESIAN_POINT('Ctrl Pts',(-2.95425829823731,0.847797238315873,
104.747003822437));
#26243=CARTESIAN_POINT('Ctrl Pts',(-2.9280187265775,0.93923239381623,104.742093490985));
#26244=CARTESIAN_POINT('Ctrl Pts',(-2.89751770441931,1.02949122436819,104.737183159533));
#26245=CARTESIAN_POINT('Ctrl Pts',(-2.86289185257744,1.11814690020842,104.732272828081));
#26246=CARTESIAN_POINT('Ctrl Pts',(-2.82826859954847,1.20679592207478,104.72736286517));
#26247=CARTESIAN_POINT('Ctrl Pts',(-2.78952129756073,1.29384160663761,104.722452902258));
#26248=CARTESIAN_POINT('Ctrl Pts',(-2.74683521027429,1.37887583835434,104.717542939347));
#26249=CARTESIAN_POINT('Ctrl Pts',(-2.70241837912313,1.4673578556188,104.712433897796));
#26250=CARTESIAN_POINT('Ctrl Pts',(-2.65373679550002,1.55366136045947,104.707324856245));
#26251=CARTESIAN_POINT('Ctrl Pts',(-2.60105180294079,1.63735511371799,104.702215814693));
#26252=CARTESIAN_POINT('Ctrl Pts',(-2.55035354038939,1.71789280899892,104.697299433057));
#26253=CARTESIAN_POINT('Ctrl Pts',(-2.4959486828039,1.79601368823005,104.69238305142));
#26254=CARTESIAN_POINT('Ctrl Pts',(-2.43811316796268,1.87136485758576,104.687466669784));
#26255=CARTESIAN_POINT('Ctrl Pts',(-2.38023908112461,1.94676628058018,104.682547009285));
#26256=CARTESIAN_POINT('Ctrl Pts',(-2.31893007893897,2.01939397562079,104.677627348787));
#26257=CARTESIAN_POINT('Ctrl Pts',(-2.25450042655716,2.0889303666359,104.672707688289));
#26258=CARTESIAN_POINT('Ctrl Pts',(-2.18997614221535,2.15856889020535,104.66778080197));
#26259=CARTESIAN_POINT('Ctrl Pts',(-2.12232239149969,2.22510674253026,104.662853915651));
#26260=CARTESIAN_POINT('Ctrl Pts',(-2.05188761562412,2.28826560146509,104.657927029332));
#26261=CARTESIAN_POINT('Ctrl Pts',(-2.04382186572228,2.29549815887612,104.657362833132));
#26262=CARTESIAN_POINT('Ctrl Pts',(-2.03571967892865,2.30268645256438,104.656798636933));
#26263=CARTESIAN_POINT('Ctrl Pts',(-2.02758160247084,2.30983010096452,104.656234440734));
#26264=CARTESIAN_POINT('Ctrl Pts',(-1.95546769854954,2.37313208357013,104.651234931241));
#26265=CARTESIAN_POINT('Ctrl Pts',(-1.880259817106,2.43316487332258,104.646235421748));
#26266=CARTESIAN_POINT('Ctrl Pts',(-1.80228664223904,2.48961143739474,104.641235912255));
#26267=CARTESIAN_POINT('Ctrl Pts',(-1.72441923748872,2.54598143206114,104.636243184565));
#26268=CARTESIAN_POINT('Ctrl Pts',(-1.6437943469127,2.59877461409763,104.631250456875));
#26269=CARTESIAN_POINT('Ctrl Pts',(-1.56077530780112,2.64771272772526,104.626257729185));
#26270=CARTESIAN_POINT('Ctrl Pts',(-1.477843851683,2.69659921287667,104.621270268696));
#26271=CARTESIAN_POINT('Ctrl Pts',(-1.39252364424015,2.74163849284233,104.616282808208));
#26272=CARTESIAN_POINT('Ctrl Pts',(-1.30520787358299,2.78259495017456,104.61129534772));
#26273=CARTESIAN_POINT('Ctrl Pts',(-1.21795457940088,2.82352210220415,104.606311455876));
#26274=CARTESIAN_POINT('Ctrl Pts',(-1.12870895682206,2.86037205323864,104.601327564033));
#26275=CARTESIAN_POINT('Ctrl Pts',(-1.03788885994979,2.89295505744423,104.596343672189));
#26276=CARTESIAN_POINT('Ctrl Pts',(-0.947101837507401,2.92552619572669,
104.591361595355));
#26277=CARTESIAN_POINT('Ctrl Pts',(-0.854741892778729,2.9538333265618,104.586379518521));
#26278=CARTESIAN_POINT('Ctrl Pts',(-0.761246030056902,2.97773516816432,
104.581397441688));
#26279=CARTESIAN_POINT('Ctrl Pts',(-0.66775869200392,3.00163483046951,104.576415819105));
#26280=CARTESIAN_POINT('Ctrl Pts',(-0.573136067203588,3.02112989357356,
104.571434196522));
#26281=CARTESIAN_POINT('Ctrl Pts',(-0.477828419957685,3.03612948522963,
104.566452573938));
#26282=CARTESIAN_POINT('Ctrl Pts',(-0.382503444102034,3.05113180407578,
104.561470045609));
#26283=CARTESIAN_POINT('Ctrl Pts',(-0.286493632072055,3.06163695999534,
104.556487517279));
#26284=CARTESIAN_POINT('Ctrl Pts',(-0.190256424370767,3.06760570200697,
104.551504988949));
#26285=CARTESIAN_POINT('Ctrl Pts',(-0.0939154871429441,3.07358087744281,
104.546517090188));
#26286=CARTESIAN_POINT('Ctrl Pts',(0.00265289622678519,3.07500985014687,
104.541529191427));
#26287=CARTESIAN_POINT('Ctrl Pts',(0.0989894381430324,3.07190549026758,
104.536541292666));
#26288=CARTESIAN_POINT('Ctrl Pts',(0.195382887376889,3.06879929660031,104.531550447484));
#26289=CARTESIAN_POINT('Ctrl Pts',(0.291543785086276,3.0611544729812,104.526559602303));
#26290=CARTESIAN_POINT('Ctrl Pts',(0.387018248209097,3.04903576980546,104.521568757122));
#26291=CARTESIAN_POINT('Ctrl Pts',(0.482647000475417,3.03689748249934,104.516569846609));
#26292=CARTESIAN_POINT('Ctrl Pts',(0.577586671046384,3.02027095479029,104.511570936095));
#26293=CARTESIAN_POINT('Ctrl Pts',(0.67139390137743,2.99927199153281,104.506572025582));
#26294=CARTESIAN_POINT('Ctrl Pts',(0.725854565532475,2.98708084718782,104.503669861371));
#26295=CARTESIAN_POINT('Ctrl Pts',(0.779933812901155,2.97341691542069,104.50076769716));
#26296=CARTESIAN_POINT('Ctrl Pts',(0.833547700173759,2.95831040993589,104.497865532949));
#26297=CARTESIAN_POINT('Ctrl Pts',(0.926836818625348,2.93202482142043,104.492815715549));
#26298=CARTESIAN_POINT('Ctrl Pts',(1.01904687568902,2.90127553014951,104.487765898149));
#26299=CARTESIAN_POINT('Ctrl Pts',(1.10971947703148,2.86616903414592,104.482716080748));
#26300=CARTESIAN_POINT('Ctrl Pts',(1.19935676078363,2.8314633910164,104.477723923156));
#26301=CARTESIAN_POINT('Ctrl Pts',(1.28749108347536,2.79249965768734,104.472731765564));
#26302=CARTESIAN_POINT('Ctrl Pts',(1.37369152560868,2.74943154896988,104.467739607972));
#26303=CARTESIAN_POINT('Ctrl Pts',(1.46138540044595,2.70561728025063,104.462660960667));
#26304=CARTESIAN_POINT('Ctrl Pts',(1.54707730635654,2.65755518789107,104.457582313363));
#26305=CARTESIAN_POINT('Ctrl Pts',(1.63033297575459,2.60545900719378,104.452503666059));
#26306=CARTESIAN_POINT('Ctrl Pts',(1.71358864515264,2.55336282649648,104.447425018755));
#26307=CARTESIAN_POINT('Ctrl Pts',(1.79440764694954,2.49723277219189,104.44234637145));
#26308=CARTESIAN_POINT('Ctrl Pts',(1.8723819390353,2.43733217358127,104.437267724146));
#26309=CARTESIAN_POINT('Ctrl Pts',(1.87238193903528,2.43733217358128,105.437268236956));
#26310=CARTESIAN_POINT('Ctrl Pts',(1.94857858758612,2.37879717777398,105.432273767433));
#26311=CARTESIAN_POINT('Ctrl Pts',(2.02214284670669,2.31659717020739,105.42727929791));
#26312=CARTESIAN_POINT('Ctrl Pts',(2.09270312766355,2.25099886038781,105.422284828387));
#26313=CARTESIAN_POINT('Ctrl Pts',(2.16318302679711,2.18547527974557,105.417296048531));
#26314=CARTESIAN_POINT('Ctrl Pts',(2.23066543068644,2.11656138927756,105.412307268676));
#26315=CARTESIAN_POINT('Ctrl Pts',(2.2948108199587,2.04456488050648,105.407318488821));
#26316=CARTESIAN_POINT('Ctrl Pts',(2.35890300902193,1.97262808342098,105.402333846506));
#26317=CARTESIAN_POINT('Ctrl Pts',(2.41966339522959,1.89761407787516,105.397349204191));
#26318=CARTESIAN_POINT('Ctrl Pts',(2.47678916287568,1.81986749316031,105.392364561876));
#26319=CARTESIAN_POINT('Ctrl Pts',(2.53388976982813,1.74215515145138,105.387382115016));
#26320=CARTESIAN_POINT('Ctrl Pts',(2.58735867913724,1.66171297490895,105.382399668156));
#26321=CARTESIAN_POINT('Ctrl Pts',(2.63693383328984,1.57891805007459,105.377417221296));
#26322=CARTESIAN_POINT('Ctrl Pts',(2.68650068635184,1.4961369888012,105.37243560872));
#26323=CARTESIAN_POINT('Ctrl Pts',(2.73217485472712,1.41100433882768,105.367453996144));
#26324=CARTESIAN_POINT('Ctrl Pts',(2.77373862360918,1.32392458165057,105.362472383567));
#26325=CARTESIAN_POINT('Ctrl Pts',(2.81530677959038,1.2368356331143,105.357490245177));
#26326=CARTESIAN_POINT('Ctrl Pts',(2.85276348569194,1.14779956557037,105.352508106786));
#26327=CARTESIAN_POINT('Ctrl Pts',(2.88593830961203,1.05724279288801,105.347525968396));
#26328=CARTESIAN_POINT('Ctrl Pts',(2.9191474671539,0.966592300281464,105.34253867384));
#26329=CARTESIAN_POINT('Ctrl Pts',(2.94806574065103,0.8744183723187,105.337551379285));
#26330=CARTESIAN_POINT('Ctrl Pts',(2.97257200930894,0.781164450978793,105.33256408473));
#26331=CARTESIAN_POINT('Ctrl Pts',(2.99709107801706,0.687861821494363,105.327574185224));
#26332=CARTESIAN_POINT('Ctrl Pts',(3.01719346026177,0.593478504598446,105.322584285718));
#26333=CARTESIAN_POINT('Ctrl Pts',(3.03280925406294,0.498467931235499,105.317594386212));
#26334=CARTESIAN_POINT('Ctrl Pts',(3.0484515967511,0.403295827500985,105.312596003226));
#26335=CARTESIAN_POINT('Ctrl Pts',(3.05959206077699,0.307494773333855,105.30759762024));
#26336=CARTESIAN_POINT('Ctrl Pts',(3.06621267375895,0.211523259430255,105.302599237253));
#26337=CARTESIAN_POINT('Ctrl Pts',(3.071903459219,0.129030400024395,105.298302848792));
#26338=CARTESIAN_POINT('Ctrl Pts',(3.07425568275345,0.0464118010204372,
105.294006460331));
#26339=CARTESIAN_POINT('Ctrl Pts',(3.07328864861143,-0.0360434781360978,
105.28971007187));
#26340=CARTESIAN_POINT('Ctrl Pts',(3.07216335549216,-0.131992891140951,
105.284710562377));
#26341=CARTESIAN_POINT('Ctrl Pts',(3.0665384052831,-0.22805808365021,105.279711052884));
#26342=CARTESIAN_POINT('Ctrl Pts',(3.05639772121958,-0.323782673600333,
105.274711543391));
#26343=CARTESIAN_POINT('Ctrl Pts',(3.0462707929296,-0.419377413752011,105.269718815701));
#26344=CARTESIAN_POINT('Ctrl Pts',(3.03164035078638,-0.514632036803301,
105.264726088011));
#26345=CARTESIAN_POINT('Ctrl Pts',(3.01254232265201,-0.609090308764181,
105.259733360321));
#26346=CARTESIAN_POINT('Ctrl Pts',(2.99346444245592,-0.70344892962915,105.254745899833));
#26347=CARTESIAN_POINT('Ctrl Pts',(2.9699284323356,-0.797012441563642,105.249758439344));
#26348=CARTESIAN_POINT('Ctrl Pts',(2.94202188636012,-0.889330911516094,
105.244770978856));
#26349=CARTESIAN_POINT('Ctrl Pts',(2.91413530817061,-0.981583325445304,
105.239787087013));
#26350=CARTESIAN_POINT('Ctrl Pts',(2.88188453754418,-1.07259204939377,105.234803195169));
#26351=CARTESIAN_POINT('Ctrl Pts',(2.84540777360706,-1.16191946876559,105.229819303325));
#26352=CARTESIAN_POINT('Ctrl Pts',(2.80894429360394,-1.25121435730368,105.224837226492));
#26353=CARTESIAN_POINT('Ctrl Pts',(2.76825804389783,-1.33882875184732,105.219855149658));
#26354=CARTESIAN_POINT('Ctrl Pts',(2.72353606965056,-1.42434319154913,105.214873072824));
#26355=CARTESIAN_POINT('Ctrl Pts',(2.67881817301702,-1.50984983430417,105.209891450241));
#26356=CARTESIAN_POINT('Ctrl Pts',(2.63006548701451,-1.59325651399534,105.204909827658));
#26357=CARTESIAN_POINT('Ctrl Pts',(2.5775114123991,-1.6741676047972,105.199928205075));
#26358=CARTESIAN_POINT('Ctrl Pts',(2.52494778252695,-1.75509340666099,105.194945676745));
#26359=CARTESIAN_POINT('Ctrl Pts',(2.46858163053288,-1.8335223504018,105.189963148415));
#26360=CARTESIAN_POINT('Ctrl Pts',(2.40868954716271,-1.90908798000226,105.184980620085));
#26361=CARTESIAN_POINT('Ctrl Pts',(2.34873290895347,-1.98473505821468,105.179992721324));
#26362=CARTESIAN_POINT('Ctrl Pts',(2.2852430252631,-2.05751231632888,105.175004822563));
#26363=CARTESIAN_POINT('Ctrl Pts',(2.21853648627002,-2.12708676576408,105.170016923802));
#26364=CARTESIAN_POINT('Ctrl Pts',(2.15179054280878,-2.1967023137815,105.165026078621));
#26365=CARTESIAN_POINT('Ctrl Pts',(2.08182447882346,-2.26311098389953,105.16003523344));
#26366=CARTESIAN_POINT('Ctrl Pts',(2.00898985730555,-2.32601848729614,105.155044388258));
#26367=CARTESIAN_POINT('Ctrl Pts',(1.93603753319994,-2.38902765080688,105.150045477745));
#26368=CARTESIAN_POINT('Ctrl Pts',(1.86020774028786,-2.44852407909202,105.145046567232));
#26369=CARTESIAN_POINT('Ctrl Pts',(1.7818829776655,-2.50425543902892,105.140047656719));
#26370=CARTESIAN_POINT('Ctrl Pts',(1.73641080481555,-2.53661080082469,105.137145492508));
#26371=CARTESIAN_POINT('Ctrl Pts',(1.6900982210611,-2.56769797845902,105.134243328297));
#26372=CARTESIAN_POINT('Ctrl Pts',(1.64302381086744,-2.59747473653212,105.131341164086));
#26373=CARTESIAN_POINT('Ctrl Pts',(1.56192951587574,-2.64877065703635,105.126341654593));
#26374=CARTESIAN_POINT('Ctrl Pts',(1.47828826060228,-2.69635533621959,105.1213421451));
#26375=CARTESIAN_POINT('Ctrl Pts',(1.39247410178145,-2.73996681108877,105.116342635607));
#26376=CARTESIAN_POINT('Ctrl Pts',(1.30677634932212,-2.78351912726922,105.111349907917));
#26377=CARTESIAN_POINT('Ctrl Pts',(1.21891193931509,-2.82310875348712,105.106357180227));
#26378=CARTESIAN_POINT('Ctrl Pts',(1.12928311829205,-2.85851742844793,105.101364452537));
#26379=CARTESIAN_POINT('Ctrl Pts',(1.03974885341599,-2.89388874814918,105.096376992049));
#26380=CARTESIAN_POINT('Ctrl Pts',(0.948454283980141,-2.92508772456526,
105.09138953156));
#26381=CARTESIAN_POINT('Ctrl Pts',(0.855824501084636,-2.95194286417323,
105.086402071072));
#26382=CARTESIAN_POINT('Ctrl Pts',(0.763260996964004,-2.97877878830107,
105.081418179229));
#26383=CARTESIAN_POINT('Ctrl Pts',(0.669364599019418,-3.00127693253031,
105.076434287385));
#26384=CARTESIAN_POINT('Ctrl Pts',(0.574577617727836,-3.01931495727196,
105.071450395541));
#26385=CARTESIAN_POINT('Ctrl Pts',(0.479825155507194,-3.03734641301177,
105.066468318707));
#26386=CARTESIAN_POINT('Ctrl Pts',(0.384183185127693,-3.05092089452402,
105.061486241874));
#26387=CARTESIAN_POINT('Ctrl Pts',(0.288105384142396,-3.05996691773427,
105.05650416504));
#26388=CARTESIAN_POINT('Ctrl Pts',(0.192036343239045,-3.06901211615561,
105.051522542457));
#26389=CARTESIAN_POINT('Ctrl Pts',(0.0955319877824317,-3.07352963621368,
105.046540919874));
#26390=CARTESIAN_POINT('Ctrl Pts',(-0.000948758931243446,-3.07349985356377,
105.041559297291));
#26391=CARTESIAN_POINT('Ctrl Pts',(-0.0974470475446472,-3.07347006549885,
105.036576768961));
#26392=CARTESIAN_POINT('Ctrl Pts',(-0.193921279932462,-3.06889133291107,
105.031594240631));
#26393=CARTESIAN_POINT('Ctrl Pts',(-0.289913485351131,-3.05979614043347,
105.026611712301));
#26394=CARTESIAN_POINT('Ctrl Pts',(-0.386009156219984,-3.05069114467882,
105.02162381354));
#26395=CARTESIAN_POINT('Ctrl Pts',(-0.481621325148319,-3.03706001184057,
105.016635914779));
#26396=CARTESIAN_POINT('Ctrl Pts',(-0.576298315866676,-3.01898699916532,
105.011648016018));
#26397=CARTESIAN_POINT('Ctrl Pts',(-0.671031233582986,-3.00090331051342,
105.006657170837));
#26398=CARTESIAN_POINT('Ctrl Pts',(-0.764827446503814,-2.97837261993017,
105.001666325656));
#26399=CARTESIAN_POINT('Ctrl Pts',(-0.857248698416135,-2.95152958973205,
104.996675480474));
#26400=CARTESIAN_POINT('Ctrl Pts',(-0.949819305405491,-2.92464318051925,
104.991676569961));
#26401=CARTESIAN_POINT('Ctrl Pts',(-1.04101009957125,-2.89343065849364,
104.986677659448));
#26402=CARTESIAN_POINT('Ctrl Pts',(-1.13040117360682,-2.85807547778366,
104.981678748935));
#26403=CARTESIAN_POINT('Ctrl Pts',(-1.18229799695739,-2.83754969724429,
104.978776584724));
#26404=CARTESIAN_POINT('Ctrl Pts',(-1.23358864024603,-2.81562852167547,
104.975874420513));
#26405=CARTESIAN_POINT('Ctrl Pts',(-1.28419489131042,-2.79235487199106,
104.972972256302));
#26406=CARTESIAN_POINT('Ctrl Pts',(-1.37137342919031,-2.7522617469731,104.967972746809));
#26407=CARTESIAN_POINT('Ctrl Pts',(-1.456825702983,-2.70801166018953,104.962973237316));
#26408=CARTESIAN_POINT('Ctrl Pts',(-1.54012832437796,-2.65977574138286,
104.957973727823));
#26409=CARTESIAN_POINT('Ctrl Pts',(-1.62331794629595,-2.61160525429376,
104.952981000133));
#26410=CARTESIAN_POINT('Ctrl Pts',(-1.70436333452886,-2.55945989883298,
104.947988272443));
#26411=CARTESIAN_POINT('Ctrl Pts',(-1.78286240943459,-2.50355824358554,
104.942995544753));
#26412=CARTESIAN_POINT('Ctrl Pts',(-1.861278669795,-2.44771556317528,104.938008084265));
#26413=CARTESIAN_POINT('Ctrl Pts',(-1.93715360136216,-2.38812471406588,
104.933020623776));
#26414=CARTESIAN_POINT('Ctrl Pts',(-2.01011191517901,-2.32504888947638,
104.928033163288));
#26415=CARTESIAN_POINT('Ctrl Pts',(-2.0830180256169,-2.2620181971138,104.923049271445));
#26416=CARTESIAN_POINT('Ctrl Pts',(-2.15301133586417,-2.19550777265747,
104.918065379601));
#26417=CARTESIAN_POINT('Ctrl Pts',(-2.21974841178776,-2.12582201474293,
104.913081487757));
#26418=CARTESIAN_POINT('Ctrl Pts',(-2.28646118372119,-2.05616163465552,
104.908099410924));
#26419=CARTESIAN_POINT('Ctrl Pts',(-2.34991977416294,-1.98332853541114,
104.90311733409));
#26420=CARTESIAN_POINT('Ctrl Pts',(-2.40981721737087,-1.90766433862535,
104.898135257256));
#26421=CARTESIAN_POINT('Ctrl Pts',(-2.46970919931195,-1.8320070406711,104.893153634673));
#26422=CARTESIAN_POINT('Ctrl Pts',(-2.52604040726019,-1.75351950267518,
104.88817201209));
#26423=CARTESIAN_POINT('Ctrl Pts',(-2.57854451896164,-1.67257598145282,
104.883190389507));
#26424=CARTESIAN_POINT('Ctrl Pts',(-2.63105817683576,-1.59161774327204,
104.878207861177));
#26425=CARTESIAN_POINT('Ctrl Pts',(-2.6797431176888,-1.50820300332114,104.873225332847));
#26426=CARTESIAN_POINT('Ctrl Pts',(-2.72437724649409,-1.42273359023582,
104.868242804517));
#26427=CARTESIAN_POINT('Ctrl Pts',(-2.76905948431207,-1.33717205371965,
104.863254905756));
#26428=CARTESIAN_POINT('Ctrl Pts',(-2.80968198987636,-1.24955181250041,
104.858267006995));
#26429=CARTESIAN_POINT('Ctrl Pts',(-2.8460695216654,-1.16029760313778,104.853279108234));
#26430=CARTESIAN_POINT('Ctrl Pts',(-2.88247854806892,-1.07099067008858,
104.848288263053));
#26431=CARTESIAN_POINT('Ctrl Pts',(-2.9146474731721,-0.980048260651874,
104.843297417872));
#26432=CARTESIAN_POINT('Ctrl Pts',(-2.94245064140778,-0.887911297866479,
104.83830657269));
#26433=CARTESIAN_POINT('Ctrl Pts',(-2.97029874026546,-0.795625439422457,
104.833307662177));
#26434=CARTESIAN_POINT('Ctrl Pts',(-2.99376688782516,-0.7021415984557,104.828308751664));
#26435=CARTESIAN_POINT('Ctrl Pts',(-3.01278034480596,-0.607911871862083,
104.823309841151));
#26436=CARTESIAN_POINT('Ctrl Pts',(-3.0238187849283,-0.553205923554098,
104.82040767694));
#26437=CARTESIAN_POINT('Ctrl Pts',(-3.03335674278417,-0.498248709403444,
104.817505512729));
#26438=CARTESIAN_POINT('Ctrl Pts',(-3.04138763737114,-0.443129201527042,
104.814603348518));
#26439=CARTESIAN_POINT('Ctrl Pts',(-3.06262762190927,-0.297349988219478,
104.806927749953));
#26440=CARTESIAN_POINT('Ctrl Pts',(-3.07338972786299,-0.150008145579605,
104.799252151388));
#26441=CARTESIAN_POINT('Ctrl Pts',(-3.07349915681818,-0.0022766286332329,
104.791576552823));
#26442=CARTESIAN_POINT('Origin',(0.,0.,116.208423447177));
#26443=CARTESIAN_POINT('',(1.87238193903529,2.43733217358128,106.437412799624));
#26444=CARTESIAN_POINT('',(1.87238193903529,2.43733217358128,106.354088497349));
#26445=CARTESIAN_POINT('',(1.8723819390353,2.43733217358128,116.208423447177));
#26446=CARTESIAN_POINT('',(-3.07349947605365,-0.00179463031419764,105.708423447212));
#26447=CARTESIAN_POINT('Ctrl Pts',(1.87238193903529,2.43733217358128,106.354088497349));
#26448=CARTESIAN_POINT('Ctrl Pts',(1.94882610271153,2.37860703428205,106.349105157254));
#26449=CARTESIAN_POINT('Ctrl Pts',(2.02255624584631,2.31624258933613,106.344121817158));
#26450=CARTESIAN_POINT('Ctrl Pts',(2.09321314072919,2.25052460494851,106.339138477063));
#26451=CARTESIAN_POINT('Ctrl Pts',(2.16384886215988,2.1848263139907,106.334156630304));
#26452=CARTESIAN_POINT('Ctrl Pts',(2.23141284411495,2.11577677922113,106.329174783545));
#26453=CARTESIAN_POINT('Ctrl Pts',(2.29558034985051,2.04370083607661,106.324192936786));
#26454=CARTESIAN_POINT('Ctrl Pts',(2.35974614434464,1.97162681507849,106.319211222884));
#26455=CARTESIAN_POINT('Ctrl Pts',(2.42051535126871,1.89652687448059,106.314229508983));
#26456=CARTESIAN_POINT('Ctrl Pts',(2.47760212909524,1.81876055045812,106.309247795082));
#26457=CARTESIAN_POINT('Ctrl Pts',(2.53470296884459,1.74097507061556,106.304264854058));
#26458=CARTESIAN_POINT('Ctrl Pts',(2.58811931807684,1.66052225656373,106.299281913034));
#26459=CARTESIAN_POINT('Ctrl Pts',(2.63760806823708,1.57779147176382,106.29429897201));
#26460=CARTESIAN_POINT('Ctrl Pts',(2.68715187132221,1.49496865449862,106.289310487797));
#26461=CARTESIAN_POINT('Ctrl Pts',(2.73275912984867,1.40986318619962,106.284322003584));
#26462=CARTESIAN_POINT('Ctrl Pts',(2.77423234473112,1.32288969587326,106.279333519372));
#26463=CARTESIAN_POINT('Ctrl Pts',(2.81573245764219,1.23585979768369,106.274341799809));
#26464=CARTESIAN_POINT('Ctrl Pts',(2.85309301960049,1.14695986977429,106.269350080245));
#26465=CARTESIAN_POINT('Ctrl Pts',(2.8861651946821,1.05662326257075,106.264358360682));
#26466=CARTESIAN_POINT('Ctrl Pts',(2.91928857655281,0.966146784083211,106.259358912267));
#26467=CARTESIAN_POINT('Ctrl Pts',(2.94811018886722,0.874229604593374,106.254359463852));
#26468=CARTESIAN_POINT('Ctrl Pts',(2.97253147258493,0.781318689455259,106.249360015438));
#26469=CARTESIAN_POINT('Ctrl Pts',(2.98094563523119,0.749306959006453,106.247637494517));
#26470=CARTESIAN_POINT('Ctrl Pts',(2.98883788747533,0.71717733402477,106.245914973597));
#26471=CARTESIAN_POINT('Ctrl Pts',(2.99620562000438,0.684948270057071,106.244192452677));
#26472=CARTESIAN_POINT('Ctrl Pts',(3.01759000395423,0.591405422849737,106.239192943184));
#26473=CARTESIAN_POINT('Ctrl Pts',(3.03462707651195,0.496695869818655,106.234193433691));
#26474=CARTESIAN_POINT('Ctrl Pts',(3.04719429030025,0.401259525944931,106.229193924198));
#26475=CARTESIAN_POINT('Ctrl Pts',(3.05974445674285,0.305952640865651,106.224201196508));
#26476=CARTESIAN_POINT('Ctrl Pts',(3.06783675807475,0.20992135581178,106.219208468818));
#26477=CARTESIAN_POINT('Ctrl Pts',(3.07139923898995,0.113617625093908,106.214215741128));
#26478=CARTESIAN_POINT('Ctrl Pts',(3.07495796157757,0.0174154923846215,
106.209228280639));
#26479=CARTESIAN_POINT('Ctrl Pts',(3.0739963476656,-0.0790580782787412,
106.204240820151));
#26480=CARTESIAN_POINT('Ctrl Pts',(3.06849414646785,-0.175345154174617,
106.199253359663));
#26481=CARTESIAN_POINT('Ctrl Pts',(3.06299588222366,-0.271563334417186,
106.194269467819));
#26482=CARTESIAN_POINT('Ctrl Pts',(3.05296351431736,-0.367594848176605,
106.189285575975));
#26483=CARTESIAN_POINT('Ctrl Pts',(3.03842887460575,-0.462981882973846,
106.184301684132));
#26484=CARTESIAN_POINT('Ctrl Pts',(3.02389952804996,-0.558334180175458,
106.179319607298));
#26485=CARTESIAN_POINT('Ctrl Pts',(3.00487123348384,-0.653042031234897,
106.174337530464));
#26486=CARTESIAN_POINT('Ctrl Pts',(2.98142756238955,-0.746653828908618,
106.169355453631));
#26487=CARTESIAN_POINT('Ctrl Pts',(2.95798602881796,-0.840257091343089,
106.164373831048));
#26488=CARTESIAN_POINT('Ctrl Pts',(2.93013002593912,-0.932764073312985,
106.159392208464));
#26489=CARTESIAN_POINT('Ctrl Pts',(2.89799377469533,-1.02373547942185,106.154410585881));
#26490=CARTESIAN_POINT('Ctrl Pts',(2.86585168051494,-1.11472342573497,106.149428057552));
#26491=CARTESIAN_POINT('Ctrl Pts',(2.82942793865795,-1.20417482782572,106.144445529222));
#26492=CARTESIAN_POINT('Ctrl Pts',(2.78890559181497,-1.29166863008404,106.139463000892));
#26493=CARTESIAN_POINT('Ctrl Pts',(2.74833956785412,-1.37925673776671,106.134475102131));
#26494=CARTESIAN_POINT('Ctrl Pts',(2.70366630417707,-1.46488263421209,106.12948720337));
#26495=CARTESIAN_POINT('Ctrl Pts',(2.65511557027466,-1.54814842908717,106.124499304609));
#26496=CARTESIAN_POINT('Ctrl Pts',(2.60653615678729,-1.63146341021025,106.119508459427));
#26497=CARTESIAN_POINT('Ctrl Pts',(2.55407495097874,-1.71241514559357,106.114517614246));
#26498=CARTESIAN_POINT('Ctrl Pts',(2.49800478819914,-1.79063517449372,106.109526769065));
#26499=CARTESIAN_POINT('Ctrl Pts',(2.44184401462058,-1.86898160893583,106.104527858552));
#26500=CARTESIAN_POINT('Ctrl Pts',(2.38206291060169,-1.94458717800361,106.099528948038));
#26501=CARTESIAN_POINT('Ctrl Pts',(2.31897421576095,-2.01711696156567,106.094530037525));
#26502=CARTESIAN_POINT('Ctrl Pts',(2.28234748443543,-2.0592248051711,106.091627873314));
#26503=CARTESIAN_POINT('Ctrl Pts',(2.24460662877106,-2.10029664273728,106.088725709103));
#26504=CARTESIAN_POINT('Ctrl Pts',(2.20581815167771,-2.14027300401821,106.085823544892));
#26505=CARTESIAN_POINT('Ctrl Pts',(2.13899789432946,-2.20913960948482,106.080824035399));
#26506=CARTESIAN_POINT('Ctrl Pts',(2.06883211266339,-2.27499493850143,106.075824525906));
#26507=CARTESIAN_POINT('Ctrl Pts',(1.99562308286094,-2.33749668687521,106.070825016413));
#26508=CARTESIAN_POINT('Ctrl Pts',(1.92251336064241,-2.39991365202433,106.065832288723));
#26509=CARTESIAN_POINT('Ctrl Pts',(1.84636892569537,-2.45898579500717,106.060839561033));
#26510=CARTESIAN_POINT('Ctrl Pts',(1.76752969763012,-2.51440669303826,106.055846833343));
#26511=CARTESIAN_POINT('Ctrl Pts',(1.68877364296334,-2.5697691234188,106.050859372855));
#26512=CARTESIAN_POINT('Ctrl Pts',(1.60732880397115,-2.62148771523487,106.045871912366));
#26513=CARTESIAN_POINT('Ctrl Pts',(1.52356826551536,-2.66929616009811,106.040884451878));
#26514=CARTESIAN_POINT('Ctrl Pts',(1.43986765968277,-2.71707039690151,106.035900560035));
#26515=CARTESIAN_POINT('Ctrl Pts',(1.35385502843941,-2.76093983167477,106.030916668191));
#26516=CARTESIAN_POINT('Ctrl Pts',(1.26593171226487,-2.80068190801493,106.025932776347));
#26517=CARTESIAN_POINT('Ctrl Pts',(1.17804041558438,-2.84040951127523,106.020950699513));
#26518=CARTESIAN_POINT('Ctrl Pts',(1.08824021608889,-2.87601256194491,106.01596862268));
#26519=CARTESIAN_POINT('Ctrl Pts',(0.996955419074167,-2.90731528086973,
106.010986545846));
#26520=CARTESIAN_POINT('Ctrl Pts',(0.90567894513013,-2.93861514570767,106.006004923263));
#26521=CARTESIAN_POINT('Ctrl Pts',(0.812918558076705,-2.96561531613726,
106.00102330068));
#26522=CARTESIAN_POINT('Ctrl Pts',(0.719115812304894,-2.98818920058504,
105.996041678097));
#26523=CARTESIAN_POINT('Ctrl Pts',(0.625296011541326,-3.01076718936272,
105.991059149767));
#26524=CARTESIAN_POINT('Ctrl Pts',(0.530433902455986,-3.02891719120094,
105.986076621437));
#26525=CARTESIAN_POINT('Ctrl Pts',(0.434982321124866,-3.04256349651225,
105.981094093108));
#26526=CARTESIAN_POINT('Ctrl Pts',(0.339427857056205,-3.05622451052956,
105.976106194346));
#26527=CARTESIAN_POINT('Ctrl Pts',(0.24328308756026,-3.0653720745883,105.971118295585));
#26528=CARTESIAN_POINT('Ctrl Pts',(0.147006858336642,-3.06998228555182,
105.966130396824));
#26529=CARTESIAN_POINT('Ctrl Pts',(0.0506737574230522,-3.07459521983023,
105.961139551643));
#26530=CARTESIAN_POINT('Ctrl Pts',(-0.0457905190849338,-3.07466546382483,
105.956148706462));
#26531=CARTESIAN_POINT('Ctrl Pts',(-0.14192836352605,-3.07022126069552,
105.951157861281));
#26532=CARTESIAN_POINT('Ctrl Pts',(-0.238221569151672,-3.06576987562172,
105.946158950767));
#26533=CARTESIAN_POINT('Ctrl Pts',(-0.334186852606287,-3.05678951687311,
105.941160040254));
#26534=CARTESIAN_POINT('Ctrl Pts',(-0.429373013894057,-3.04336016024057,
105.936161129741));
#26535=CARTESIAN_POINT('Ctrl Pts',(-0.484634229301692,-3.03556362175623,
105.93325896553));
#26536=CARTESIAN_POINT('Ctrl Pts',(-0.539633037571687,-3.02626850926642,
105.930356801319));
#26537=CARTESIAN_POINT('Ctrl Pts',(-0.594283347907387,-3.01549822623062,
105.927454637108));
#26538=CARTESIAN_POINT('Ctrl Pts',(-0.688428518701941,-2.99694444072266,
105.922455127615));
#26539=CARTESIAN_POINT('Ctrl Pts',(-0.781869329979001,-2.9739449610631,
105.917455618122));
#26540=CARTESIAN_POINT('Ctrl Pts',(-0.874154084883601,-2.94656696612877,
105.912456108629));
#26541=CARTESIAN_POINT('Ctrl Pts',(-0.966313656103778,-2.91922610927084,
105.907463380939));
#26542=CARTESIAN_POINT('Ctrl Pts',(-1.05731987037793,-2.8875186651387,105.902470653249));
#26543=CARTESIAN_POINT('Ctrl Pts',(-1.14673063287514,-2.85156292331518,
105.897477925559));
#26544=CARTESIAN_POINT('Ctrl Pts',(-1.23604706927213,-2.81564511389276,
105.892490465071));
#26545=CARTESIAN_POINT('Ctrl Pts',(-1.32377099481605,-2.77548807932703,
105.887503004583));
#26546=CARTESIAN_POINT('Ctrl Pts',(-1.40947590544984,-2.73125976830406,
105.882515544094));
#26547=CARTESIAN_POINT('Ctrl Pts',(-1.49511949221646,-2.6870631036716,105.877531652251));
#26548=CARTESIAN_POINT('Ctrl Pts',(-1.57874654700909,-2.63880115440058,
105.872547760407));
#26549=CARTESIAN_POINT('Ctrl Pts',(-1.65995188078329,-2.58668939060801,
105.867563868563));
#26550=CARTESIAN_POINT('Ctrl Pts',(-1.7411276415861,-2.53459660462918,105.86258179173));
#26551=CARTESIAN_POINT('Ctrl Pts',(-1.81988306461357,-2.47865702659944,
105.857599714896));
#26552=CARTESIAN_POINT('Ctrl Pts',(-1.89583969398661,-2.4191308572925,105.852617638062));
#26553=CARTESIAN_POINT('Ctrl Pts',(-1.97178939786516,-2.35961011540067,
105.847636015479));
#26554=CARTESIAN_POINT('Ctrl Pts',(-2.04494047005417,-2.29650370330816,
105.842654392896));
#26555=CARTESIAN_POINT('Ctrl Pts',(-2.11494632154101,-2.23011307045185,
105.837672770313));
#26556=CARTESIAN_POINT('Ctrl Pts',(-2.18496490132493,-2.16371036660889,
105.832690241983));
#26557=CARTESIAN_POINT('Ctrl Pts',(-2.25183680621799,-2.09402255818539,
105.827707713654));
#26558=CARTESIAN_POINT('Ctrl Pts',(-2.31525198429387,-2.02138826038525,
105.822725185324));
#26559=CARTESIAN_POINT('Ctrl Pts',(-2.37873551458575,-1.94867567351673,
105.817737286563));
#26560=CARTESIAN_POINT('Ctrl Pts',(-2.4387545905842,-1.87301058813429,105.812749387802));
#26561=CARTESIAN_POINT('Ctrl Pts',(-2.49503934326516,-1.79476486637079,
105.807761489041));
#26562=CARTESIAN_POINT('Ctrl Pts',(-2.55135734412205,-1.71647292378551,
105.802770643859));
#26563=CARTESIAN_POINT('Ctrl Pts',(-2.60393639017204,-1.63559767730731,
105.797779798678));
#26564=CARTESIAN_POINT('Ctrl Pts',(-2.65255102635424,-1.5525383417446,105.792788953497));
#26565=CARTESIAN_POINT('Ctrl Pts',(-2.70124422501623,-1.46934478019803,
105.787790042983));
#26566=CARTESIAN_POINT('Ctrl Pts',(-2.74596001776208,-1.3839604704515,105.78279113247));
#26567=CARTESIAN_POINT('Ctrl Pts',(-2.78651983112612,-1.29680741852476,
105.777792221957));
#26568=CARTESIAN_POINT('Ctrl Pts',(-2.81006720978768,-1.24620989982293,
105.774890057746));
#26569=CARTESIAN_POINT('Ctrl Pts',(-2.83221472815899,-1.19501658524713,
105.771987893535));
#26570=CARTESIAN_POINT('Ctrl Pts',(-2.85293514461266,-1.14331242914346,
105.769085729324));
#26571=CARTESIAN_POINT('Ctrl Pts',(-2.893051927116,-1.04320805191886,105.763466851407));
#26572=CARTESIAN_POINT('Ctrl Pts',(-2.92793512895817,-0.940893018626475,
105.75784797349));
#26573=CARTESIAN_POINT('Ctrl Pts',(-2.95736499242841,-0.836895782973556,
105.752229095573));
#26574=CARTESIAN_POINT('Ctrl Pts',(-2.98669778170527,-0.733241581455836,
105.746628751485));
#26575=CARTESIAN_POINT('Ctrl Pts',(-3.01061301739709,-0.627916464693566,
105.741028407397));
#26576=CARTESIAN_POINT('Ctrl Pts',(-3.02893966727519,-0.521465954791764,
105.735428063308));
#26577=CARTESIAN_POINT('Ctrl Pts',(-3.04715867314249,-0.415640696090364,
105.729860613584));
#26578=CARTESIAN_POINT('Ctrl Pts',(-3.05985444442008,-0.308703449488098,
105.72429316386));
#26579=CARTESIAN_POINT('Ctrl Pts',(-3.0669067781481,-0.201209006133457,
105.718725714136));
#26580=CARTESIAN_POINT('Ctrl Pts',(-3.07125676650912,-0.134904773307905,
105.715291625161));
#26581=CARTESIAN_POINT('Ctrl Pts',(-3.07346059135322,-0.0683889062706779,
105.711857536187));
#26582=CARTESIAN_POINT('Ctrl Pts',(-3.07349947605365,-0.00179463031418164,
105.708423447212));
#26583=CARTESIAN_POINT('Ctrl Pts',(-3.07349947605404,-0.00179462963607823,
105.708423447177));
#26584=CARTESIAN_POINT('Ctrl Pts',(-3.07355640778969,0.095707192560317,
105.70339553858));
#26585=CARTESIAN_POINT('Ctrl Pts',(-3.06896936787619,0.193220771531798,
105.698367629983));
#26586=CARTESIAN_POINT('Ctrl Pts',(-3.0597615284335,0.2902785543548,105.693339721386));
#26587=CARTESIAN_POINT('Ctrl Pts',(-3.05055210965956,0.387352984556402,
105.688310950401));
#26588=CARTESIAN_POINT('Ctrl Pts',(-3.03672035558937,0.483971037494733,
105.683282179415));
#26589=CARTESIAN_POINT('Ctrl Pts',(-3.01834127070958,0.579670788923594,
105.67825340843));
#26590=CARTESIAN_POINT('Ctrl Pts',(-2.99995437574094,0.675411207424039,
105.673222500497));
#26591=CARTESIAN_POINT('Ctrl Pts',(-2.97701638775837,0.770232128781307,
105.668191592563));
#26592=CARTESIAN_POINT('Ctrl Pts',(-2.94965312222315,0.863683222344401,
105.66316068463));
#26593=CARTESIAN_POINT('Ctrl Pts',(-2.92225260677349,0.957261531909367,
105.658122928066));
#26594=CARTESIAN_POINT('Ctrl Pts',(-2.89041490754594,1.04946588014872,105.653085171503));
#26595=CARTESIAN_POINT('Ctrl Pts',(-2.85431530228173,1.13986245010542,105.648047414939));
#26596=CARTESIAN_POINT('Ctrl Pts',(-2.81818801472202,1.23032833895201,105.643005795268));
#26597=CARTESIAN_POINT('Ctrl Pts',(-2.77779248930952,1.31898330026846,105.637964175596));
#26598=CARTESIAN_POINT('Ctrl Pts',(-2.73335070314102,1.40541672952846,105.632922555925));
#26599=CARTESIAN_POINT('Ctrl Pts',(-2.68883063971646,1.49200239775673,105.627872056229));
#26600=CARTESIAN_POINT('Ctrl Pts',(-2.64025029773579,1.57635835094933,105.622821556533));
#26601=CARTESIAN_POINT('Ctrl Pts',(-2.58787585624958,1.65810156583984,105.617771056836));
#26602=CARTESIAN_POINT('Ctrl Pts',(-2.56349136256802,1.69615957372393,105.615419645071));
#26603=CARTESIAN_POINT('Ctrl Pts',(-2.53828502684479,1.7336516852532,105.613068233305));
#26604=CARTESIAN_POINT('Ctrl Pts',(-2.51228663814599,1.77054175262633,105.61071682154));
#26605=CARTESIAN_POINT('Ctrl Pts',(-2.4570095518424,1.84897643800449,105.605717312047));
#26606=CARTESIAN_POINT('Ctrl Pts',(-2.39795870705164,1.92495774495692,105.600717802554));
#26607=CARTESIAN_POINT('Ctrl Pts',(-2.33537936862426,1.99810046158949,105.595718293061));
#26608=CARTESIAN_POINT('Ctrl Pts',(-2.272884918672,2.07114396059151,105.590725565371));
#26609=CARTESIAN_POINT('Ctrl Pts',(-2.20687177062592,2.14135619125706,105.585732837681));
#26610=CARTESIAN_POINT('Ctrl Pts',(-2.13762796257577,2.20838152129883,105.58074010999));
#26611=CARTESIAN_POINT('Ctrl Pts',(-2.06845720499776,2.27533614130686,105.575752649502));
#26612=CARTESIAN_POINT('Ctrl Pts',(-1.99606287656792,2.33911024066632,105.570765189014));
#26613=CARTESIAN_POINT('Ctrl Pts',(-1.9207720244847,2.39938264558969,105.565777728526));
#26614=CARTESIAN_POINT('Ctrl Pts',(-1.84553504476623,2.45961192419833,105.560793836682));
#26615=CARTESIAN_POINT('Ctrl Pts',(-1.76740600318806,2.51634421573316,105.555809944838));
#26616=CARTESIAN_POINT('Ctrl Pts',(-1.68674667299025,2.56929716287477,105.550826052995));
#26617=CARTESIAN_POINT('Ctrl Pts',(-1.60611671692275,2.62223082586454,105.545843976161));
#26618=CARTESIAN_POINT('Ctrl Pts',(-1.52295866966958,2.67138763844867,105.540861899327));
#26619=CARTESIAN_POINT('Ctrl Pts',(-1.43766427554716,2.7165278722692,105.535879822494));
#26620=CARTESIAN_POINT('Ctrl Pts',(-1.35237765830835,2.76166399034043,105.530898199911));
#26621=CARTESIAN_POINT('Ctrl Pts',(-1.2649554695348,2.80278405259261,105.525916577328));
#26622=CARTESIAN_POINT('Ctrl Pts',(-1.17581415413273,2.83969423088845,105.520934954745));
#26623=CARTESIAN_POINT('Ctrl Pts',(-1.08665663126879,2.87661112010509,105.515952426415));
#26624=CARTESIAN_POINT('Ctrl Pts',(-0.995779766595947,2.90931643732089,
105.510969898085));
#26625=CARTESIAN_POINT('Ctrl Pts',(-0.903619074985017,2.93766485789704,
105.505987369755));
#26626=CARTESIAN_POINT('Ctrl Pts',(-0.811359047731229,2.96604383389256,
105.500999470994));
#26627=CARTESIAN_POINT('Ctrl Pts',(-0.717812851215745,2.99005640866325,
105.496011572233));
#26628=CARTESIAN_POINT('Ctrl Pts',(-0.623430006574469,3.00960749548883,
105.491023673472));
#26629=CARTESIAN_POINT('Ctrl Pts',(-0.528991408691466,3.02917013140974,
105.486032828291));
#26630=CARTESIAN_POINT('Ctrl Pts',(-0.433715611962334,3.04426596308788,
105.481041983109));
#26631=CARTESIAN_POINT('Ctrl Pts',(-0.338059037536675,3.05485160640247,
105.476051137928));
#26632=CARTESIAN_POINT('Ctrl Pts',(-0.242247879670979,3.065454356384,105.471052227415));
#26633=CARTESIAN_POINT('Ctrl Pts',(-0.14605515319154,3.07153233665974,105.466053316902));
#26634=CARTESIAN_POINT('Ctrl Pts',(-0.0499390083025376,3.07309426237624,
105.461054406389));
#26635=CARTESIAN_POINT('Ctrl Pts',(0.00586211777445551,3.07400105294644,
105.458152242178));
#26636=CARTESIAN_POINT('Ctrl Pts',(0.0616374759675003,3.07338668686073,
105.455250077967));
#26637=CARTESIAN_POINT('Ctrl Pts',(0.117298380782215,3.07126087134679,105.452347913756));
#26638=CARTESIAN_POINT('Ctrl Pts',(0.213170815550757,3.06759928679534,105.447349117025));
#26639=CARTESIAN_POINT('Ctrl Pts',(0.309040004977434,3.05943784159464,105.442350320295));
#26640=CARTESIAN_POINT('Ctrl Pts',(0.404449496958352,3.04677253079552,105.437351523564));
#26641=CARTESIAN_POINT('Ctrl Pts',(0.499737015301177,3.03412341161428,105.432359117408));
#26642=CARTESIAN_POINT('Ctrl Pts',(0.594565572604177,3.01698192325251,105.427366711251));
#26643=CARTESIAN_POINT('Ctrl Pts',(0.6884801318473,2.99539602691389,105.422374305095));
#26644=CARTESIAN_POINT('Ctrl Pts',(0.782300280046847,2.9738318305866,105.417386917737));
#26645=CARTESIAN_POINT('Ctrl Pts',(0.875207830789812,2.94783220335917,105.41239953038));
#26646=CARTESIAN_POINT('Ctrl Pts',(0.966755342263142,2.91749659095014,105.407412143022));
#26647=CARTESIAN_POINT('Ctrl Pts',(1.05823691733825,2.88718282753501,105.402428347792));
#26648=CARTESIAN_POINT('Ctrl Pts',(1.14835998508706,2.85253942515601,105.397444552562));
#26649=CARTESIAN_POINT('Ctrl Pts',(1.23669075990271,2.81371608631206,105.392460757332));
#26650=CARTESIAN_POINT('Ctrl Pts',(1.32498387377679,2.77490930028902,105.387479087007));
#26651=CARTESIAN_POINT('Ctrl Pts',(1.41148581328142,2.73192629887186,105.382497416681));
#26652=CARTESIAN_POINT('Ctrl Pts',(1.49578230549484,2.6849650918715,105.377515746355));
#26653=CARTESIAN_POINT('Ctrl Pts',(1.58008336359877,2.63800134123351,105.372533806199));
#26654=CARTESIAN_POINT('Ctrl Pts',(1.66217834910624,2.58705916249099,105.367551866042));
#26655=CARTESIAN_POINT('Ctrl Pts',(1.7416778638474,2.53238237013765,105.362569925886));
#26656=CARTESIAN_POINT('Ctrl Pts',(1.78607617520012,2.50184687242328,105.359787648146));
#26657=CARTESIAN_POINT('Ctrl Pts',(1.82966546057547,2.47014738179717,105.357005370406));
#26658=CARTESIAN_POINT('Ctrl Pts',(1.87238193903529,2.43733217358128,105.354223092666));
#26659=CARTESIAN_POINT('',(-3.07349899192526,0.00248930400748836,105.791576552872));
#26660=CARTESIAN_POINT('Ctrl Pts',(-3.07349899192449,0.00248930494811218,
105.791576552823));
#26661=CARTESIAN_POINT('Ctrl Pts',(-3.0733769618853,0.153157547793597,105.783754517199));
#26662=CARTESIAN_POINT('Ctrl Pts',(-3.06217291351732,0.303387429693875,
105.775932481575));
#26663=CARTESIAN_POINT('Ctrl Pts',(-3.04009617916299,0.451904272427881,
105.768110445952));
#26664=CARTESIAN_POINT('Ctrl Pts',(-3.0369975376803,0.472749767163985,105.767012562376));
#26665=CARTESIAN_POINT('Ctrl Pts',(-3.03368476415738,0.493561567928361,
105.765914678799));
#26666=CARTESIAN_POINT('Ctrl Pts',(-3.03015849914789,0.514336193594988,
105.764816795223));
#26667=CARTESIAN_POINT('Ctrl Pts',(-3.01410069869206,0.608939064508622,
105.75981728573));
#26668=CARTESIAN_POINT('Ctrl Pts',(-2.99358013316199,0.702955380470386,
105.754817776237));
#26669=CARTESIAN_POINT('Ctrl Pts',(-2.96865201364476,0.79593182615278,105.749818266744));
#26670=CARTESIAN_POINT('Ctrl Pts',(-2.94375770896337,0.888782149876992,
105.744825539054));
#26671=CARTESIAN_POINT('Ctrl Pts',(-2.91446784550576,0.980594986390127,
105.739832811364));
#26672=CARTESIAN_POINT('Ctrl Pts',(-2.88088898110049,1.07092526750179,105.734840083674));
#26673=CARTESIAN_POINT('Ctrl Pts',(-2.84734554155075,1.16116025244383,105.729852623186));
#26674=CARTESIAN_POINT('Ctrl Pts',(-2.80952224819633,1.24991538197292,105.724865162698));
#26675=CARTESIAN_POINT('Ctrl Pts',(-2.76757571287371,1.33675986007644,105.719877702209));
#26676=CARTESIAN_POINT('Ctrl Pts',(-2.72565919127763,1.42354219892586,105.714893810366));
#26677=CARTESIAN_POINT('Ctrl Pts',(-2.67962548309349,1.50841620997487,105.709909918522));
#26678=CARTESIAN_POINT('Ctrl Pts',(-2.62967926860791,1.59097114815252,105.704926026678));
#26679=CARTESIAN_POINT('Ctrl Pts',(-2.57975124329663,1.67349602186633,105.699943949845));
#26680=CARTESIAN_POINT('Ctrl Pts',(-2.52591376967499,1.75370312554444,105.694961873011));
#26681=CARTESIAN_POINT('Ctrl Pts',(-2.46841694995455,1.83120725511261,105.689979796177));
#26682=CARTESIAN_POINT('Ctrl Pts',(-2.41092537261941,1.90870431808977,105.684998173594));
#26683=CARTESIAN_POINT('Ctrl Pts',(-2.34977537422278,1.98349854450907,105.680016551011));
#26684=CARTESIAN_POINT('Ctrl Pts',(-2.28525913387661,2.05523549527385,105.675034928428));
#26685=CARTESIAN_POINT('Ctrl Pts',(-2.22073116334122,2.12698548908021,105.670052400098));
#26686=CARTESIAN_POINT('Ctrl Pts',(-2.15283602889522,2.19567677692278,105.665069871768));
#26687=CARTESIAN_POINT('Ctrl Pts',(-2.08190402857787,2.26099046123402,105.660087343438));
#26688=CARTESIAN_POINT('Ctrl Pts',(-2.01089557401804,2.32637454407111,105.655099444677));
#26689=CARTESIAN_POINT('Ctrl Pts',(-1.93684404221188,2.38837345750345,105.650111545916));
#26690=CARTESIAN_POINT('Ctrl Pts',(-1.86011402906525,2.44670759366023,105.645123647155));
#26691=CARTESIAN_POINT('Ctrl Pts',(-1.78333869044674,2.50507618859188,105.640132801974));
#26692=CARTESIAN_POINT('Ctrl Pts',(-1.70388208143739,2.55977544691557,105.635141956793));
#26693=CARTESIAN_POINT('Ctrl Pts',(-1.62213731550006,2.61056943590134,105.630151111611));
#26694=CARTESIAN_POINT('Ctrl Pts',(-1.54026044795657,2.66144550925608,105.625152201098));
#26695=CARTESIAN_POINT('Ctrl Pts',(-1.45608842304143,2.70840349785718,105.620153290585));
#26696=CARTESIAN_POINT('Ctrl Pts',(-1.37003837715734,2.75125373150426,105.615154380072));
#26697=CARTESIAN_POINT('Ctrl Pts',(-1.32008121892035,2.77613083506423,105.612252215861));
#26698=CARTESIAN_POINT('Ctrl Pts',(-1.26949145639921,2.79962432257363,105.60935005165));
#26699=CARTESIAN_POINT('Ctrl Pts',(-1.21835329387792,2.82170471546844,105.606447887439));
#26700=CARTESIAN_POINT('Ctrl Pts',(-1.13025844107435,2.85974223707676,105.601448377946));
#26701=CARTESIAN_POINT('Ctrl Pts',(-1.04022582662802,2.89371707501104,105.596448868453));
#26702=CARTESIAN_POINT('Ctrl Pts',(-0.948665747700957,2.92342873166749,
105.59144935896));
#26703=CARTESIAN_POINT('Ctrl Pts',(-0.857229869439561,2.95310008465035,
105.58645663127));
#26704=CARTESIAN_POINT('Ctrl Pts',(-0.764271058609443,2.97851961531101,
105.58146390358));
#26705=CARTESIAN_POINT('Ctrl Pts',(-0.670220650551179,2.99953438546298,
105.57647117589));
#26706=CARTESIAN_POINT('Ctrl Pts',(-0.57626946330279,3.02052698556213,105.571483715401));
#26707=CARTESIAN_POINT('Ctrl Pts',(-0.48122939427299,3.03712396771852,105.566496254913));
#26708=CARTESIAN_POINT('Ctrl Pts',(-0.385547059392509,3.0492221491708,105.561508794425));
#26709=CARTESIAN_POINT('Ctrl Pts',(-0.289933187459186,3.06131167409146,
105.556524902581));
#26710=CARTESIAN_POINT('Ctrl Pts',(-0.193678397497479,3.06890874261549,
105.551541010737));
#26711=CARTESIAN_POINT('Ctrl Pts',(-0.0972386578056601,3.07196140819317,
105.546557118894));
#26712=CARTESIAN_POINT('Ctrl Pts',(-0.000834039078500506,3.07501296206565,
105.54157504206));
#26713=CARTESIAN_POINT('Ctrl Pts',(0.0957549572592695,3.07352338734202,
105.536592965226));
#26714=CARTESIAN_POINT('Ctrl Pts',(0.192069056462435,3.06749274286829,105.531610888393));
#26715=CARTESIAN_POINT('Ctrl Pts',(0.288374374038715,3.0614626482504,105.52662926581));
#26716=CARTESIAN_POINT('Ctrl Pts',(0.384404406220011,3.05089233468703,105.521647643226));
#26717=CARTESIAN_POINT('Ctrl Pts',(0.479702774852875,3.03583390484368,105.516666020643));
#26718=CARTESIAN_POINT('Ctrl Pts',(0.575018470408214,3.02077273711248,105.511683492314));
#26719=CARTESIAN_POINT('Ctrl Pts',(0.669601804645896,3.00122190103336,105.506700963984));
#26720=CARTESIAN_POINT('Ctrl Pts',(0.763005457463406,2.97728482377502,105.501718435654));
#26721=CARTESIAN_POINT('Ctrl Pts',(0.856509785653021,2.95332194587519,105.496730536893));
#26722=CARTESIAN_POINT('Ctrl Pts',(0.948831468019021,2.92496349749113,105.491742638132));
#26723=CARTESIAN_POINT('Ctrl Pts',(1.03953746682639,2.89236306591413,105.486754739371));
#26724=CARTESIAN_POINT('Ctrl Pts',(1.13029704691229,2.85974337681472,105.481763894189));
#26725=CARTESIAN_POINT('Ctrl Pts',(1.21943863760954,2.82287688275281,105.476773049008));
#26726=CARTESIAN_POINT('Ctrl Pts',(1.30655030912593,2.7819648703251,105.471782203827));
#26727=CARTESIAN_POINT('Ctrl Pts',(1.39380275530329,2.74098674305216,105.466783293313));
#26728=CARTESIAN_POINT('Ctrl Pts',(1.47901834423043,2.6959502481222,105.4617843828));
#26729=CARTESIAN_POINT('Ctrl Pts',(1.56181087144092,2.64710201009499,105.456785472287));
#26730=CARTESIAN_POINT('Ctrl Pts',(1.60987684677172,2.61874270904359,105.453883308076));
#26731=CARTESIAN_POINT('Ctrl Pts',(1.65712667802367,2.58909947248047,105.450981143865));
#26732=CARTESIAN_POINT('Ctrl Pts',(1.70348979365083,2.55822688065923,105.448078979654));
#26733=CARTESIAN_POINT('Ctrl Pts',(1.76105829279885,2.5198927706255,105.444475398755));
#26734=CARTESIAN_POINT('Ctrl Pts',(1.81740497180485,2.4795660067949,105.440871817856));
#26735=CARTESIAN_POINT('Ctrl Pts',(1.87238193903528,2.43733217358128,105.437268236956));
#26736=CARTESIAN_POINT('Ctrl Pts',(1.87238193903529,2.43733217358128,106.437412799624));
#26737=CARTESIAN_POINT('Ctrl Pts',(1.94886548644755,2.37857677931852,106.432422059601));
#26738=CARTESIAN_POINT('Ctrl Pts',(2.02251314091683,2.31626985199124,106.427431319579));
#26739=CARTESIAN_POINT('Ctrl Pts',(2.09299380989473,2.25072858464595,106.422440579557));
#26740=CARTESIAN_POINT('Ctrl Pts',(2.16358899334487,2.18508082819166,106.417441730758));
#26741=CARTESIAN_POINT('Ctrl Pts',(2.23100660916304,2.11618855151676,106.41244288196));
#26742=CARTESIAN_POINT('Ctrl Pts',(2.29495385707934,2.04440432495059,106.407444033162));
#26743=CARTESIAN_POINT('Ctrl Pts',(2.33397751316687,2.00059817126444,106.404393497561));
#26744=CARTESIAN_POINT('Ctrl Pts',(2.37170959517796,1.95571568837146,106.40134296196));
#26745=CARTESIAN_POINT('Ctrl Pts',(2.40809147900642,1.9098423177678,106.398292426359));
#26746=CARTESIAN_POINT('Ctrl Pts',(2.46771758975408,1.83466065073596,106.393292916866));
#26747=CARTESIAN_POINT('Ctrl Pts',(2.52392424819075,1.75655192635719,106.388293407373));
#26748=CARTESIAN_POINT('Ctrl Pts',(2.57641121104068,1.67586023332016,106.38329389788));
#26749=CARTESIAN_POINT('Ctrl Pts',(2.62882697565878,1.59527799805237,106.37830117019));
#26750=CARTESIAN_POINT('Ctrl Pts',(2.67753283546953,1.51212012247802,106.3733084425));
#26751=CARTESIAN_POINT('Ctrl Pts',(2.72226900449198,1.42676337112439,106.36831571481));
#26752=CARTESIAN_POINT('Ctrl Pts',(2.7669579779838,1.34149666899182,106.363328254322));
#26753=CARTESIAN_POINT('Ctrl Pts',(2.80768538333752,1.2540360893513,106.358340793833));
#26754=CARTESIAN_POINT('Ctrl Pts',(2.84423550879917,1.16478608357325,106.353353333345));
#26755=CARTESIAN_POINT('Ctrl Pts',(2.88075948179168,1.07559993826061,106.348369441502));
#26756=CARTESIAN_POINT('Ctrl Pts',(2.91311195088674,0.984627317191522,106.343385549658));
#26757=CARTESIAN_POINT('Ctrl Pts',(2.9411242491937,0.892295018928603,106.338401657814));
#26758=CARTESIAN_POINT('Ctrl Pts',(2.9691263461154,0.799996345801883,106.333419580981));
#26759=CARTESIAN_POINT('Ctrl Pts',(2.99279128538639,0.706339398938902,106.328437504147));
#26760=CARTESIAN_POINT('Ctrl Pts',(3.01199975905624,0.61176768584582,106.323455427313));
#26761=CARTESIAN_POINT('Ctrl Pts',(3.03120648135583,0.517204595514167,106.31847380473));
#26762=CARTESIAN_POINT('Ctrl Pts',(3.04595745871357,0.421727334993363,106.313492182147));
#26763=CARTESIAN_POINT('Ctrl Pts',(3.05618439138251,0.325790140842114,106.308510559564));
#26764=CARTESIAN_POINT('Ctrl Pts',(3.066413183488,0.229835503618627,106.303528031234));
#26765=CARTESIAN_POINT('Ctrl Pts',(3.07211625082295,0.13342120317577,106.298545502904));
#26766=CARTESIAN_POINT('Ctrl Pts',(3.07327720859963,0.0370060684490628,
106.293562974574));
#26767=CARTESIAN_POINT('Ctrl Pts',(3.0744394177177,-0.0595129875833855,
106.288575075813));
#26768=CARTESIAN_POINT('Ctrl Pts',(3.07104973812129,-0.156032440036609,
106.283587177052));
#26769=CARTESIAN_POINT('Ctrl Pts',(3.06314393340568,-0.252094215006907,
106.278599278291));
#26770=CARTESIAN_POINT('Ctrl Pts',(3.05523345862272,-0.348212734986186,
106.27360843311));
#26771=CARTESIAN_POINT('Ctrl Pts',(3.04280160336489,-0.443872604060372,
106.268617587929));
#26772=CARTESIAN_POINT('Ctrl Pts',(3.02593567731295,-0.538623733941043,
106.263626742747));
#26773=CARTESIAN_POINT('Ctrl Pts',(3.0090424954986,-0.633527984040376,106.258627832234));
#26774=CARTESIAN_POINT('Ctrl Pts',(2.98770103195925,-0.727520134807199,
106.253628921721));
#26775=CARTESIAN_POINT('Ctrl Pts',(2.96204906231461,-0.820163155988569,
106.248630011208));
#26776=CARTESIAN_POINT('Ctrl Pts',(2.94715657163131,-0.873947927642731,
106.245727846997));
#26777=CARTESIAN_POINT('Ctrl Pts',(2.93081215209482,-0.927278294014138,
106.242825682786));
#26778=CARTESIAN_POINT('Ctrl Pts',(2.91305016692873,-0.980071923358931,
106.239923518575));
#26779=CARTESIAN_POINT('Ctrl Pts',(2.88245189371046,-1.07101862102652,106.234924009082));
#26780=CARTESIAN_POINT('Ctrl Pts',(2.84753670122269,-1.16069074941787,106.229924499589));
#26781=CARTESIAN_POINT('Ctrl Pts',(2.80842974048269,-1.24864912716596,106.224924990096));
#26782=CARTESIAN_POINT('Ctrl Pts',(2.76937582808664,-1.33648818993311,106.219932262406));
#26783=CARTESIAN_POINT('Ctrl Pts',(2.72614162500837,-1.42261772455469,106.214939534716));
#26784=CARTESIAN_POINT('Ctrl Pts',(2.67890171754383,-1.50661469451904,106.209946807026));
#26785=CARTESIAN_POINT('Ctrl Pts',(2.63171164699089,-1.5905230497974,106.204959346538));
#26786=CARTESIAN_POINT('Ctrl Pts',(2.5805244869527,-1.67230293231822,106.199971886049));
#26787=CARTESIAN_POINT('Ctrl Pts',(2.52556204351732,-1.75155320054648,106.194984425561));
#26788=CARTESIAN_POINT('Ctrl Pts',(2.47063892699498,-1.83074676335533,106.190000533718));
#26789=CARTESIAN_POINT('Ctrl Pts',(2.41194614658162,-1.90741395039175,106.185016641874));
#26790=CARTESIAN_POINT('Ctrl Pts',(2.34974986666697,-1.98118091402541,106.18003275003));
#26791=CARTESIAN_POINT('Ctrl Pts',(2.28757623709703,-2.05492101355793,106.175050673196));
#26792=CARTESIAN_POINT('Ctrl Pts',(2.22190192574255,-2.12576265296943,106.170068596363));
#26793=CARTESIAN_POINT('Ctrl Pts',(2.15303398587826,-2.19336428931748,106.165086519529));
#26794=CARTESIAN_POINT('Ctrl Pts',(2.08417232518346,-2.26095976195375,106.160104896946));
#26795=CARTESIAN_POINT('Ctrl Pts',(2.01211792829748,-2.32531551149458,106.155123274363));
#26796=CARTESIAN_POINT('Ctrl Pts',(1.93721461943756,-2.38612693883569,106.15014165178));
#26797=CARTESIAN_POINT('Ctrl Pts',(1.86229769183634,-2.44694942276576,106.14515912345));
#26798=CARTESIAN_POINT('Ctrl Pts',(1.78453116435678,-2.50422602803077,106.14017659512));
#26799=CARTESIAN_POINT('Ctrl Pts',(1.70429097844695,-2.557693201067,106.13519406679));
#26800=CARTESIAN_POINT('Ctrl Pts',(1.62396430544236,-2.61121800383586,106.130206168029));
#26801=CARTESIAN_POINT('Ctrl Pts',(1.54115901700683,-2.66092493329992,106.125218269268));
#26802=CARTESIAN_POINT('Ctrl Pts',(1.45627881354207,-2.70659458863504,106.120230370507));
#26803=CARTESIAN_POINT('Ctrl Pts',(1.37134847017607,-2.75229122166243,106.115239525326));
#26804=CARTESIAN_POINT('Ctrl Pts',(1.28434116699327,-2.79394564242786,106.110248680145));
#26805=CARTESIAN_POINT('Ctrl Pts',(1.19568197046962,-2.83138603434676,106.105257834963));
#26806=CARTESIAN_POINT('Ctrl Pts',(1.10687949844549,-2.86888693088448,106.10025892445));
#26807=CARTESIAN_POINT('Ctrl Pts',(1.01642021437568,-2.90216004912354,106.095260013937));
#26808=CARTESIAN_POINT('Ctrl Pts',(0.924745708015972,-2.93108301238741,
106.090261103424));
#26809=CARTESIAN_POINT('Ctrl Pts',(0.871523216691855,-2.94787450898232,
106.087358939213));
#26810=CARTESIAN_POINT('Ctrl Pts',(0.817891372082622,-2.96320073719099,
106.084456775002));
#26811=CARTESIAN_POINT('Ctrl Pts',(0.763937942530578,-2.97704569497382,
106.081554610791));
#26812=CARTESIAN_POINT('Ctrl Pts',(0.67099327654534,-3.00089617097485,106.076555101298));
#26813=CARTESIAN_POINT('Ctrl Pts',(0.576767356000774,-3.02043170716477,
106.071555591805));
#26814=CARTESIAN_POINT('Ctrl Pts',(0.481696701506079,-3.03551816627049,
106.066556082312));
#26815=CARTESIAN_POINT('Ctrl Pts',(0.386755009750507,-3.05058416069024,
106.061563354622));
#26816=CARTESIAN_POINT('Ctrl Pts',(0.290971291227217,-3.06121300426841,
106.056570626932));
#26817=CARTESIAN_POINT('Ctrl Pts',(0.194795439479901,-3.06732081575401,
106.051577899242));
#26818=CARTESIAN_POINT('Ctrl Pts',(0.0987210508319767,-3.07342218365244,
106.046590438754));
#26819=CARTESIAN_POINT('Ctrl Pts',(0.00225578710244156,-3.075011973412,
106.041602978265));
#26820=CARTESIAN_POINT('Ctrl Pts',(-0.0941431146129687,-3.07205783213321,
106.036615517777));
#26821=CARTESIAN_POINT('Ctrl Pts',(-0.190473040660873,-3.06910580461155,
106.031631625934));
#26822=CARTESIAN_POINT('Ctrl Pts',(-0.286736261591445,-3.0616163228673,
106.02664773409));
#26823=CARTESIAN_POINT('Ctrl Pts',(-0.382474283279055,-3.04960910161125,
106.021663842246));
#26824=CARTESIAN_POINT('Ctrl Pts',(-0.478177439550352,-3.03760625308779,
106.016681765413));
#26825=CARTESIAN_POINT('Ctrl Pts',(-0.573355341495525,-3.02108898855307,
106.011699688579));
#26826=CARTESIAN_POINT('Ctrl Pts',(-0.667554329894647,-3.00012890833693,
106.006717611745));
#26827=CARTESIAN_POINT('Ctrl Pts',(-0.761744729516232,-2.9791707391972,
106.001735989162));
#26828=CARTESIAN_POINT('Ctrl Pts',(-0.854955964602517,-2.95377065527505,
105.996754366579));
#26829=CARTESIAN_POINT('Ctrl Pts',(-0.946745344142949,-2.92405121421354,
105.991772743996));
#26830=CARTESIAN_POINT('Ctrl Pts',(-1.03855141260981,-2.89432636963401,
105.986790215666));
#26831=CARTESIAN_POINT('Ctrl Pts',(-1.12893469451034,-2.86028074348624,
105.981807687336));
#26832=CARTESIAN_POINT('Ctrl Pts',(-1.21746944124027,-2.82208618040734,
105.976825159007));
#26833=CARTESIAN_POINT('Ctrl Pts',(-1.30609961537912,-2.78385044921848,
105.971837260246));
#26834=CARTESIAN_POINT('Ctrl Pts',(-1.3928768728847,-2.74145702744756,105.966849361484));
#26835=CARTESIAN_POINT('Ctrl Pts',(-1.47739738672443,-2.69512508275587,
105.961861462723));
#26836=CARTESIAN_POINT('Ctrl Pts',(-1.56196782799178,-2.64876576914852,
105.956870617542));
#26837=CARTESIAN_POINT('Ctrl Pts',(-1.64427849681322,-2.59846352889413,
105.951879772361));
#26838=CARTESIAN_POINT('Ctrl Pts',(-1.72395384665673,-2.54448135866574,
105.94688892718));
#26839=CARTESIAN_POINT('Ctrl Pts',(-1.80375795387767,-2.49041195188703,
105.941890016666));
#26840=CARTESIAN_POINT('Ctrl Pts',(-1.88091788718286,-2.43265100345196,
105.936891106153));
#26841=CARTESIAN_POINT('Ctrl Pts',(-1.95509057372824,-2.37150228726834,
105.93189219564));
#26842=CARTESIAN_POINT('Ctrl Pts',(-1.99815222001252,-2.33600182868072,
105.928990031429));
#26843=CARTESIAN_POINT('Ctrl Pts',(-2.04020768351381,-2.29936024005541,
105.926087867218));
#26844=CARTESIAN_POINT('Ctrl Pts',(-2.08119575623374,-2.26164242846535,
105.923185703007));
#26845=CARTESIAN_POINT('Ctrl Pts',(-2.15075950934304,-2.19762886649083,
105.918260235151));
#26846=CARTESIAN_POINT('Ctrl Pts',(-2.21750681602361,-2.13027396279245,
105.913334767295));
#26847=CARTESIAN_POINT('Ctrl Pts',(-2.28109244639444,-2.05985909736619,
105.90840929944));
#26848=CARTESIAN_POINT('Ctrl Pts',(-2.34457578858639,-1.98955750609177,
105.903491755027));
#26849=CARTESIAN_POINT('Ctrl Pts',(-2.40490726497281,-1.91620607231139,
105.898574210615));
#26850=CARTESIAN_POINT('Ctrl Pts',(-2.4617762523236,-1.84012497768374,105.893656666202));
#26851=CARTESIAN_POINT('Ctrl Pts',(-2.51859341366884,-1.76411321749329,
105.88874360326));
#26852=CARTESIAN_POINT('Ctrl Pts',(-2.57195407934606,-1.68537709464359,
105.883830540318));
#26853=CARTESIAN_POINT('Ctrl Pts',(-2.62158640063781,-1.60427148388011,
105.878917477376));
#26854=CARTESIAN_POINT('Ctrl Pts',(-2.67118799605383,-1.52321608315823,
105.874007455963));
#26855=CARTESIAN_POINT('Ctrl Pts',(-2.71706559402625,-1.43979449251477,
105.86909743455));
#26856=CARTESIAN_POINT('Ctrl Pts',(-2.75899012028278,-1.35439128990925,
105.864187413137));
#26857=CARTESIAN_POINT('Ctrl Pts',(-2.80090094098928,-1.26901600647109,
105.85927899686));
#26858=CARTESIAN_POINT('Ctrl Pts',(-2.83886105818303,-1.18166080472102,
105.854370580583));
#26859=CARTESIAN_POINT('Ctrl Pts',(-2.87268751225107,-1.09273450890725,
105.849462164305));
#26860=CARTESIAN_POINT('Ctrl Pts',(-2.90652877058643,-1.00376929418545,
105.844551599842));
#26861=CARTESIAN_POINT('Ctrl Pts',(-2.93623258264752,-0.913232033075345,
105.839641035379));
#26862=CARTESIAN_POINT('Ctrl Pts',(-2.96166455066047,-0.821550570178788,
105.834730470916));
#26863=CARTESIAN_POINT('Ctrl Pts',(-2.9871011391851,-0.729852450479684,
105.829819014295));
#26864=CARTESIAN_POINT('Ctrl Pts',(-3.00826423064648,-0.637010155946073,
105.824907557675));
#26865=CARTESIAN_POINT('Ctrl Pts',(-3.02507014949399,-0.543463743630075,
105.819996101054));
#26866=CARTESIAN_POINT('Ctrl Pts',(-3.0418970487393,-0.449800548592378,
105.815078513004));
#26867=CARTESIAN_POINT('Ctrl Pts',(-3.05435584318723,-0.355431929188649,
105.810160924953));
#26868=CARTESIAN_POINT('Ctrl Pts',(-3.06241458140855,-0.260804872608452,
105.805243336903));
#26869=CARTESIAN_POINT('Ctrl Pts',(-3.06988009998551,-0.173143500643975,
105.800687742226));
#26870=CARTESIAN_POINT('Ctrl Pts',(-3.07357006283488,-0.0852606728696437,
105.796132147549));
#26871=CARTESIAN_POINT('Ctrl Pts',(-3.07349899192525,0.00248930400749208,
105.791576552872));
#26872=CARTESIAN_POINT('Origin',(0.,0.,116.208423447177));
#26873=CARTESIAN_POINT('',(1.8723819390353,2.43733217358127,107.437292535812));
#26874=CARTESIAN_POINT('',(1.8723819390353,2.43733217358127,107.354176765664));
#26875=CARTESIAN_POINT('',(1.8723819390353,2.43733217358128,116.208423447177));
#26876=CARTESIAN_POINT('',(-3.07349975246569,-0.00123352880650566,106.708423447146));
#26877=CARTESIAN_POINT('Ctrl Pts',(1.8723819390353,2.43733217358127,107.354176765664));
#26878=CARTESIAN_POINT('Ctrl Pts',(1.87949704018099,2.43186628467864,107.353709446164));
#26879=CARTESIAN_POINT('Ctrl Pts',(1.88658706336632,2.42637011824953,107.353242126665));
#26880=CARTESIAN_POINT('Ctrl Pts',(1.89365173966783,2.42084393112257,107.352774807166));
#26881=CARTESIAN_POINT('Ctrl Pts',(1.96923154382078,2.36172329728988,107.347775297673));
#26882=CARTESIAN_POINT('Ctrl Pts',(2.04217278678712,2.29895597815628,107.34277578818));
#26883=CARTESIAN_POINT('Ctrl Pts',(2.11210297010482,2.23280614780468,107.337776278687));
#26884=CARTESIAN_POINT('Ctrl Pts',(2.18193829357291,2.1667460492779,107.332783550997));
#26885=CARTESIAN_POINT('Ctrl Pts',(2.24877035886731,2.09731285765864,107.327790823307));
#26886=CARTESIAN_POINT('Ctrl Pts',(2.31225834386002,2.02481199158088,107.322798095617));
#26887=CARTESIAN_POINT('Ctrl Pts',(2.3756793506289,1.95238761208931,107.317810635128));
#26888=CARTESIAN_POINT('Ctrl Pts',(2.43576300273951,1.87690232023088,107.31282317464));
#26889=CARTESIAN_POINT('Ctrl Pts',(2.49220483946106,1.79869877638443,107.307835714152));
#26890=CARTESIAN_POINT('Ctrl Pts',(2.54860629072909,1.72055118900166,107.302851822308));
#26891=CARTESIAN_POINT('Ctrl Pts',(2.60137085066683,1.63968957106517,107.297867930464));
#26892=CARTESIAN_POINT('Ctrl Pts',(2.65023455884298,1.55648932958578,107.292884038621));
#26893=CARTESIAN_POINT('Ctrl Pts',(2.69908047206682,1.4733193875737,107.287901961787));
#26894=CARTESIAN_POINT('Ctrl Pts',(2.7440281340211,1.3878128923161,107.282919884953));
#26895=CARTESIAN_POINT('Ctrl Pts',(2.78485765514179,1.30037305824067,107.27793780812));
#26896=CARTESIAN_POINT('Ctrl Pts',(2.82568345355081,1.2129411966636,107.272956185537));
#26897=CARTESIAN_POINT('Ctrl Pts',(2.86239167209386,1.12357674455337,107.267974562953));
#26898=CARTESIAN_POINT('Ctrl Pts',(2.89480949636708,1.03270529665679,107.26299294037));
#26899=CARTESIAN_POINT('Ctrl Pts',(2.92723321477193,0.941817326729887,107.258010412041));
#26900=CARTESIAN_POINT('Ctrl Pts',(2.95536484223045,0.849422230304534,107.253027883711));
#26901=CARTESIAN_POINT('Ctrl Pts',(2.97908095867815,0.755962228977924,107.248045355381));
#26902=CARTESIAN_POINT('Ctrl Pts',(3.00282263760414,0.66240149154387,107.24305745662));
#26903=CARTESIAN_POINT('Ctrl Pts',(3.02213919592931,0.567773983893576,107.238069557859));
#26904=CARTESIAN_POINT('Ctrl Pts',(3.03695808761004,0.472533410564768,107.233081659098));
#26905=CARTESIAN_POINT('Ctrl Pts',(3.05178573301348,0.377236577322067,107.228090813916));
#26906=CARTESIAN_POINT('Ctrl Pts',(3.06211037462238,0.281326393545326,107.223099968735));
#26907=CARTESIAN_POINT('Ctrl Pts',(3.06791144880873,0.18526087624835,107.218109123554));
#26908=CARTESIAN_POINT('Ctrl Pts',(3.07372189767746,0.0890401146494389,
107.21311021304));
#26909=CARTESIAN_POINT('Ctrl Pts',(3.07499417648102,-0.00733604307861015,
107.208111302527));
#26910=CARTESIAN_POINT('Ctrl Pts',(3.07175984225134,-0.103410451754141,
107.203112392014));
#26911=CARTESIAN_POINT('Ctrl Pts',(3.06988211929091,-0.159187347482755,
107.200210227803));
#26912=CARTESIAN_POINT('Ctrl Pts',(3.06648641852976,-0.214862631439177,
107.197308063592));
#26913=CARTESIAN_POINT('Ctrl Pts',(3.06158685878352,-0.270348212725877,
107.194405899381));
#26914=CARTESIAN_POINT('Ctrl Pts',(3.0531464695836,-0.365932290744841,107.189406389888));
#26915=CARTESIAN_POINT('Ctrl Pts',(3.04021070012985,-0.461288607501185,
107.184406880395));
#26916=CARTESIAN_POINT('Ctrl Pts',(3.0227983302358,-0.555960884166899,107.179407370902));
#26917=CARTESIAN_POINT('Ctrl Pts',(3.00540958011095,-0.650504738490473,
107.174414643212));
#26918=CARTESIAN_POINT('Ctrl Pts',(2.98355637692206,-0.744365968827277,
107.169421915522));
#26919=CARTESIAN_POINT('Ctrl Pts',(2.95730934232343,-0.837092410553675,
107.164429187832));
#26920=CARTESIAN_POINT('Ctrl Pts',(2.93108999768471,-0.92972102822135,107.159441727344));
#26921=CARTESIAN_POINT('Ctrl Pts',(2.90048615541362,-1.02121681706509,107.154454266855));
#26922=CARTESIAN_POINT('Ctrl Pts',(2.86561947227221,-1.1111378357946,107.149466806367));
#26923=CARTESIAN_POINT('Ctrl Pts',(2.83077773705761,-1.20099451393331,107.144482914524));
#26924=CARTESIAN_POINT('Ctrl Pts',(2.7916793827907,-1.2892782538538,107.13949902268));
#26925=CARTESIAN_POINT('Ctrl Pts',(2.74849558430707,-1.37556325664964,107.134515130836));
#26926=CARTESIAN_POINT('Ctrl Pts',(2.7053275122933,-1.4618168365845,107.129533054003));
#26927=CARTESIAN_POINT('Ctrl Pts',(2.65807714845424,-1.54607273349073,107.124550977169));
#26928=CARTESIAN_POINT('Ctrl Pts',(2.6069629867247,-1.62792697497383,107.119568900335));
#26929=CARTESIAN_POINT('Ctrl Pts',(2.5558534854291,-1.70977375323593,107.114587277752));
#26930=CARTESIAN_POINT('Ctrl Pts',(2.50088111931813,-1.78921893920546,107.109605655169));
#26931=CARTESIAN_POINT('Ctrl Pts',(2.44230878491009,-1.86588586176941,107.104624032586));
#26932=CARTESIAN_POINT('Ctrl Pts',(2.38372580101967,-1.94256672373068,107.099641504256));
#26933=CARTESIAN_POINT('Ctrl Pts',(2.32154181543371,-2.01646797029362,107.094658975926));
#26934=CARTESIAN_POINT('Ctrl Pts',(2.2560605639695,-2.0872453094214,107.089676447596));
#26935=CARTESIAN_POINT('Ctrl Pts',(2.19050873336672,-2.15809893608972,107.084688548835));
#26936=CARTESIAN_POINT('Ctrl Pts',(2.12165284031759,-2.22582161044657,107.079700650074));
#26937=CARTESIAN_POINT('Ctrl Pts',(2.04983395088141,-2.29010546128642,107.074712751313));
#26938=CARTESIAN_POINT('Ctrl Pts',(1.97797263704148,-2.35442728547931,107.069721906132));
#26939=CARTESIAN_POINT('Ctrl Pts',(1.90314518206019,-2.4153059644849,107.064731060951));
#26940=CARTESIAN_POINT('Ctrl Pts',(1.82572457117581,-2.47247488161253,107.059740215769));
#26941=CARTESIAN_POINT('Ctrl Pts',(1.74817884662911,-2.52973618515395,107.054741305256));
#26942=CARTESIAN_POINT('Ctrl Pts',(1.6680319632319,-2.58327551232093,107.049742394743));
#26943=CARTESIAN_POINT('Ctrl Pts',(1.58568455211106,-2.63287043950065,107.04474348423));
#26944=CARTESIAN_POINT('Ctrl Pts',(1.5378769930855,-2.66166323791702,107.041841320019));
#26945=CARTESIAN_POINT('Ctrl Pts',(1.48932819984732,-2.68912744557709,107.038939155808));
#26946=CARTESIAN_POINT('Ctrl Pts',(1.44011974937296,-2.7152269440078,107.036036991597));
#26947=CARTESIAN_POINT('Ctrl Pts',(1.35534917906867,-2.76018811115085,107.031037482104));
#26948=CARTESIAN_POINT('Ctrl Pts',(1.26832213635766,-2.80125458304302,107.026037972611));
#26949=CARTESIAN_POINT('Ctrl Pts',(1.17943156909956,-2.83819369032689,107.021038463118));
#26950=CARTESIAN_POINT('Ctrl Pts',(1.09066158133155,-2.87508268994626,107.016045735428));
#26951=CARTESIAN_POINT('Ctrl Pts',(1.00003349485742,-2.90785528508275,107.011053007738));
#26952=CARTESIAN_POINT('Ctrl Pts',(0.90796503194505,-2.93632453089999,107.006060280048));
#26953=CARTESIAN_POINT('Ctrl Pts',(0.815993698940238,-2.96476374238052,
107.00107281956));
#26954=CARTESIAN_POINT('Ctrl Pts',(0.722585427433058,-2.98890850065104,
106.996085359071));
#26955=CARTESIAN_POINT('Ctrl Pts',(0.628177150582328,-3.0086202348396,106.991097898583));
#26956=CARTESIAN_POINT('Ctrl Pts',(0.533836425060517,-3.02831786482157,
106.98611400674));
#26957=CARTESIAN_POINT('Ctrl Pts',(0.438497545093442,-3.04358868691319,
106.981130114896));
#26958=CARTESIAN_POINT('Ctrl Pts',(0.342610863925298,-3.05434445436666,
106.976146223052));
#26959=CARTESIAN_POINT('Ctrl Pts',(0.246759102311604,-3.06509630483601,
106.971164146219));
#26960=CARTESIAN_POINT('Ctrl Pts',(0.150360371653682,-3.07133631877303,
106.966182069385));
#26961=CARTESIAN_POINT('Ctrl Pts',(0.0538724802433375,-3.07302782380382,
106.961199992551));
#26962=CARTESIAN_POINT('Ctrl Pts',(-0.0426066136942767,-3.07471917460832,
106.956218369968));
#26963=CARTESIAN_POINT('Ctrl Pts',(-0.139174413323532,-3.07186283353432,
106.951236747385));
#26964=CARTESIAN_POINT('Ctrl Pts',(-0.235371835401016,-3.06447423697768,
106.946255124802));
#26965=CARTESIAN_POINT('Ctrl Pts',(-0.331586747864818,-3.05708429704401,
106.941272596472));
#26966=CARTESIAN_POINT('Ctrl Pts',(-0.427430711371173,-3.04516049872647,
106.936290068142));
#26967=CARTESIAN_POINT('Ctrl Pts',(-0.522449566975857,-3.02877016294844,
106.931307539812));
#26968=CARTESIAN_POINT('Ctrl Pts',(-0.617570838903127,-3.01236216080403,
106.926319641051));
#26969=CARTESIAN_POINT('Ctrl Pts',(-0.711864794142939,-2.99147808469634,
106.92133174229));
#26970=CARTESIAN_POINT('Ctrl Pts',(-0.804887498754871,-2.9662363972462,
106.916343843529));
#26971=CARTESIAN_POINT('Ctrl Pts',(-0.897965153155196,-2.94097979918483,
106.911352998348));
#26972=CARTESIAN_POINT('Ctrl Pts',(-0.989769644110338,-2.91136059904522,
106.906362153167));
#26973=CARTESIAN_POINT('Ctrl Pts',(-1.07987426320182,-2.87754649409429,
106.901371307985));
#26974=CARTESIAN_POINT('Ctrl Pts',(-1.1701244936332,-2.84367774469583,106.896372397472));
#26975=CARTESIAN_POINT('Ctrl Pts',(-1.25866896399276,-2.80560072747383,
106.891373486959));
#26976=CARTESIAN_POINT('Ctrl Pts',(-1.34510298282755,-2.76353038984348,
106.886374576446));
#26977=CARTESIAN_POINT('Ctrl Pts',(-1.39528306014903,-2.73910606220384,
106.883472412235));
#26978=CARTESIAN_POINT('Ctrl Pts',(-1.44475229191811,-2.71333663971388,
106.880570248024));
#26979=CARTESIAN_POINT('Ctrl Pts',(-1.49343596752607,-2.68627088375306,
106.877668083813));
#26980=CARTESIAN_POINT('Ctrl Pts',(-1.5773025169908,-2.6396451610084,106.87266857432));
#26981=CARTESIAN_POINT('Ctrl Pts',(-1.65913076605024,-2.58900625370816,
106.867669064827));
#26982=CARTESIAN_POINT('Ctrl Pts',(-1.73851161236678,-2.53455708629059,
106.862669555334));
#26983=CARTESIAN_POINT('Ctrl Pts',(-1.81778477906938,-2.48018177882287,
106.857676827644));
#26984=CARTESIAN_POINT('Ctrl Pts',(-1.89461678219015,-2.42200672964877,
106.852684099954));
#26985=CARTESIAN_POINT('Ctrl Pts',(-1.96862338430176,-2.36028053857593,
106.847691372264));
#26986=CARTESIAN_POINT('Ctrl Pts',(-2.04255191131358,-2.29861946707879,
106.842703911776));
#26987=CARTESIAN_POINT('Ctrl Pts',(-2.11366062751448,-2.23341498089758,
106.837716451288));
#26988=CARTESIAN_POINT('Ctrl Pts',(-2.18159541178576,-2.16495813106751,
106.832728990799));
#26989=CARTESIAN_POINT('Ctrl Pts',(-2.24948158713089,-2.0965502637137,106.827745098956));
#26990=CARTESIAN_POINT('Ctrl Pts',(-2.31419803691549,-2.02489496964545,
106.822761207112));
#26991=CARTESIAN_POINT('Ctrl Pts',(-2.37542554492148,-1.95032195561001,
106.817777315268));
#26992=CARTESIAN_POINT('Ctrl Pts',(-2.43663075538551,-1.87577609921931,
106.812795238435));
#26993=CARTESIAN_POINT('Ctrl Pts',(-2.49434927032418,-1.79831497297089,
106.807813161601));
#26994=CARTESIAN_POINT('Ctrl Pts',(-2.54830107479406,-1.71830261659681,
106.802831084767));
#26995=CARTESIAN_POINT('Ctrl Pts',(-2.60224796010231,-1.6382975555063,106.797849462184));
#26996=CARTESIAN_POINT('Ctrl Pts',(-2.65242857249977,-1.55574209082362,
106.792867839601));
#26997=CARTESIAN_POINT('Ctrl Pts',(-2.6986059113277,-1.47102970240142,106.787886217018));
#26998=CARTESIAN_POINT('Ctrl Pts',(-2.74479164600945,-1.38630191177441,
106.782903688688));
#26999=CARTESIAN_POINT('Ctrl Pts',(-2.78697245151776,-1.29941680399648,
106.777921160359));
#27000=CARTESIAN_POINT('Ctrl Pts',(-2.82495752857764,-1.21079197706811,
106.772938632029));
#27001=CARTESIAN_POINT('Ctrl Pts',(-2.86298354795241,-1.1220716256377,106.767950733268));
#27002=CARTESIAN_POINT('Ctrl Pts',(-2.89680463715693,-1.0316082156055,106.762962834507));
#27003=CARTESIAN_POINT('Ctrl Pts',(-2.92627846119675,-0.939838612494707,
106.757974935746));
#27004=CARTESIAN_POINT('Ctrl Pts',(-2.95576969582899,-0.848014799819735,
106.752984090564));
#27005=CARTESIAN_POINT('Ctrl Pts',(-2.98090843766949,-0.754883681308667,
106.747993245383));
#27006=CARTESIAN_POINT('Ctrl Pts',(-3.00160302782743,-0.660894479729704,
106.743002400202));
#27007=CARTESIAN_POINT('Ctrl Pts',(-3.02233106096569,-0.566753389227413,
106.738003489688));
#27008=CARTESIAN_POINT('Ctrl Pts',(-3.0386005277857,-0.471751879127948,
106.733004579175));
#27009=CARTESIAN_POINT('Ctrl Pts',(-3.05037138962777,-0.37634642995565,
106.728005668662));
#27010=CARTESIAN_POINT('Ctrl Pts',(-3.05720507346357,-0.320957904917864,
106.725103504451));
#27011=CARTESIAN_POINT('Ctrl Pts',(-3.06252348114542,-0.265433292654388,
106.72220134024));
#27012=CARTESIAN_POINT('Ctrl Pts',(-3.0663268370347,-0.209861808056603,
106.719299176029));
#27013=CARTESIAN_POINT('Ctrl Pts',(-3.07107780497571,-0.140444601398931,
106.715673933079));
#27014=CARTESIAN_POINT('Ctrl Pts',(-3.07347180662027,-0.0708642553406025,
106.712048690128));
#27015=CARTESIAN_POINT('Ctrl Pts',(-3.07349975246545,-0.0012335294098428,
106.708423447177));
#27016=CARTESIAN_POINT('Ctrl Pts',(-3.07349975246569,-0.00123352880650975,
106.708423447146));
#27017=CARTESIAN_POINT('Ctrl Pts',(-3.07353790671295,0.0938328116699644,
106.703473928438));
#27018=CARTESIAN_POINT('Ctrl Pts',(-3.06916108330069,0.18907672144084,106.69852440973));
#27019=CARTESIAN_POINT('Ctrl Pts',(-3.06034609058113,0.28404938983357,106.693574891022));
#27020=CARTESIAN_POINT('Ctrl Pts',(-3.05154252364177,0.378898956952153,
106.68863178776));
#27021=CARTESIAN_POINT('Ctrl Pts',(-3.03831225657513,0.473477538391671,
106.683688684499));
#27022=CARTESIAN_POINT('Ctrl Pts',(-3.02068411174001,0.567335656451707,
106.678745581237));
#27023=CARTESIAN_POINT('Ctrl Pts',(-3.00307397543663,0.661097891086995,
106.673807527743));
#27024=CARTESIAN_POINT('Ctrl Pts',(-2.98107497399975,0.75414068679251,106.668869474249));
#27025=CARTESIAN_POINT('Ctrl Pts',(-2.95476767376119,0.846020238585289,
106.663931420755));
#27026=CARTESIAN_POINT('Ctrl Pts',(-2.92847497441744,0.937848796028246,
106.658996107945));
#27027=CARTESIAN_POINT('Ctrl Pts',(-2.89787884709398,1.02851496137343,106.654060795135));
#27028=CARTESIAN_POINT('Ctrl Pts',(-2.86311061951497,1.11758660980731,106.649125482325));
#27029=CARTESIAN_POINT('Ctrl Pts',(-2.82835173619897,1.20663431946239,106.644191495923));
#27030=CARTESIAN_POINT('Ctrl Pts',(-2.7894231428698,1.29408794592081,106.639257509521));
#27031=CARTESIAN_POINT('Ctrl Pts',(-2.74650516220389,1.37953312536792,106.634323523119));
#27032=CARTESIAN_POINT('Ctrl Pts',(-2.70358643071273,1.46497979962902,106.6293894504));
#27033=CARTESIAN_POINT('Ctrl Pts',(-2.65667837574756,1.54841755690931,106.624455377681));
#27034=CARTESIAN_POINT('Ctrl Pts',(-2.60600780319389,1.62945560838354,106.619521304962));
#27035=CARTESIAN_POINT('Ctrl Pts',(-2.55528842710113,1.71057171194034,106.614582479974));
#27036=CARTESIAN_POINT('Ctrl Pts',(-2.50079953325928,1.78928311198955,106.609643654985));
#27037=CARTESIAN_POINT('Ctrl Pts',(-2.44281174149959,1.86522734421081,106.604704829997));
#27038=CARTESIAN_POINT('Ctrl Pts',(-2.38479683706134,1.94120708479504,106.599763695819));
#27039=CARTESIAN_POINT('Ctrl Pts',(-2.32328006610208,2.0144167378847,106.594822561642));
#27040=CARTESIAN_POINT('Ctrl Pts',(-2.25857142803395,2.0845280891532,106.589881427464));
#27041=CARTESIAN_POINT('Ctrl Pts',(-2.19375173689868,2.15475976563379,106.584931813304));
#27042=CARTESIAN_POINT('Ctrl Pts',(-2.12572955460516,2.2218822018932,106.579982199144));
#27043=CARTESIAN_POINT('Ctrl Pts',(-2.05485076363564,2.28560508163288,106.575032584985));
#27044=CARTESIAN_POINT('Ctrl Pts',(-1.98753540476063,2.34612429280382,106.570331812738));
#27045=CARTESIAN_POINT('Ctrl Pts',(-1.91764398370614,2.40357730667361,106.565631040491));
#27046=CARTESIAN_POINT('Ctrl Pts',(-1.84549689863096,2.45775170575539,106.560930268245));
#27047=CARTESIAN_POINT('Ctrl Pts',(-1.76876481764489,2.5153689244328,106.555930758752));
#27048=CARTESIAN_POINT('Ctrl Pts',(-1.68919712402311,2.56949048583303,106.550931249259));
#27049=CARTESIAN_POINT('Ctrl Pts',(-1.60714572551787,2.61982535046702,106.545931739766));
#27050=CARTESIAN_POINT('Ctrl Pts',(-1.52520562921355,2.67009193617684,106.540939012076));
#27051=CARTESIAN_POINT('Ctrl Pts',(-1.4407888949156,2.71658180626101,106.535946284386));
#27052=CARTESIAN_POINT('Ctrl Pts',(-1.35427902496947,2.75904522843098,106.530953556696));
#27053=CARTESIAN_POINT('Ctrl Pts',(-1.26786042075562,2.80146385276085,106.525966096207));
#27054=CARTESIAN_POINT('Ctrl Pts',(-1.17935346262849,2.83986428115655,106.520978635719));
#27055=CARTESIAN_POINT('Ctrl Pts',(-1.08916816463259,2.87404157227255,106.515991175231));
#27056=CARTESIAN_POINT('Ctrl Pts',(-0.999047396325561,2.90819440873783,
106.511007283387));
#27057=CARTESIAN_POINT('Ctrl Pts',(-0.907251084763536,2.93812995991572,
106.506023391544));
#27058=CARTESIAN_POINT('Ctrl Pts',(-0.81421033935335,2.96369090380392,106.5010394997));
#27059=CARTESIAN_POINT('Ctrl Pts',(-0.721203477078128,2.98924253902948,
106.496057422866));
#27060=CARTESIAN_POINT('Ctrl Pts',(-0.626953504244634,3.01042261616097,
106.491075346033));
#27061=CARTESIAN_POINT('Ctrl Pts',(-0.531906928153377,3.02712359671396,
106.486093269199));
#27062=CARTESIAN_POINT('Ctrl Pts',(-0.436869018120279,3.04382305452225,
106.481111646616));
#27063=CARTESIAN_POINT('Ctrl Pts',(-0.341035081605433,3.05604415192055,
106.476130024033));
#27064=CARTESIAN_POINT('Ctrl Pts',(-0.244861002391348,3.06373062450143,
106.47114840145));
#27065=CARTESIAN_POINT('Ctrl Pts',(-0.148669437035249,3.07141849461844,
106.46616587312));
#27066=CARTESIAN_POINT('Ctrl Pts',(-0.0521380437231236,3.07457006757433,
106.46118334479));
#27067=CARTESIAN_POINT('Ctrl Pts',(0.0442740757878782,3.07318109720419,
106.45620081646));
#27068=CARTESIAN_POINT('Ctrl Pts',(0.140790113354838,3.07179062972869,106.451212917699));
#27069=CARTESIAN_POINT('Ctrl Pts',(0.237186180818789,3.06584985476902,106.446225018938));
#27070=CARTESIAN_POINT('Ctrl Pts',(0.333005310159123,3.05540663634251,106.441237120177));
#27071=CARTESIAN_POINT('Ctrl Pts',(0.42888104117435,3.04495724896352,106.436246274996));
#27072=CARTESIAN_POINT('Ctrl Pts',(0.524178722015902,3.0300001903401,106.431255429815));
#27073=CARTESIAN_POINT('Ctrl Pts',(0.61845073052815,3.0106346413853,106.426264584633));
#27074=CARTESIAN_POINT('Ctrl Pts',(0.712875084986894,2.99123779721434,106.42126567412));
#27075=CARTESIAN_POINT('Ctrl Pts',(0.8062700323702,2.96741834560313,106.416266763607));
#27076=CARTESIAN_POINT('Ctrl Pts',(0.898202338471354,2.93932557046078,106.411267853094));
#27077=CARTESIAN_POINT('Ctrl Pts',(0.95157449784442,2.92301604733754,106.408365688883));
#27078=CARTESIAN_POINT('Ctrl Pts',(1.00445401722475,2.90526711899224,106.405463524672));
#27079=CARTESIAN_POINT('Ctrl Pts',(1.05675950233112,2.88611531374491,106.402561360461));
#27080=CARTESIAN_POINT('Ctrl Pts',(1.14685315663654,2.85312726062258,106.397562523749));
#27081=CARTESIAN_POINT('Ctrl Pts',(1.23555890822217,2.81585865486352,106.392563687038));
#27082=CARTESIAN_POINT('Ctrl Pts',(1.32244121367734,2.77444615849139,106.387564850326));
#27083=CARTESIAN_POINT('Ctrl Pts',(1.4092199524657,2.73308302722519,106.382571972399));
#27084=CARTESIAN_POINT('Ctrl Pts',(1.49417916876701,2.6875860016328,106.377579094471));
#27085=CARTESIAN_POINT('Ctrl Pts',(1.57690055060915,2.63814080433334,106.372586216543));
#27086=CARTESIAN_POINT('Ctrl Pts',(1.65952934396238,2.58875095011447,106.367598927049));
#27087=CARTESIAN_POINT('Ctrl Pts',(1.73992490908725,2.5354219361422,106.362611637556));
#27088=CARTESIAN_POINT('Ctrl Pts',(1.81769214758397,2.47838606891896,106.357624348063));
#27089=CARTESIAN_POINT('Ctrl Pts',(1.83607042340513,2.46490711660189,106.356445731158));
#27090=CARTESIAN_POINT('Ctrl Pts',(1.85430202037919,2.45122134039976,106.355267114254));
#27091=CARTESIAN_POINT('Ctrl Pts',(1.87238193903529,2.43733217358128,106.354088497349));
#27092=CARTESIAN_POINT('',(-3.07349998753216,0.000276838910911489,106.791576552796));
#27093=CARTESIAN_POINT('Ctrl Pts',(-3.07349998753216,0.000276838910921114,
106.791576552796));
#27094=CARTESIAN_POINT('Ctrl Pts',(-3.07349079945254,0.102284040620658,
106.786322773875));
#27095=CARTESIAN_POINT('Ctrl Pts',(-3.06839901409353,0.204179977417602,
106.781068994954));
#27096=CARTESIAN_POINT('Ctrl Pts',(-3.05828337165257,0.305458783919216,
106.775815216034));
#27097=CARTESIAN_POINT('Ctrl Pts',(-3.04813772460372,0.407037999504475,
106.770545853567));
#27098=CARTESIAN_POINT('Ctrl Pts',(-3.03293845951957,0.507996061930611,
106.765276491101));
#27099=CARTESIAN_POINT('Ctrl Pts',(-3.01279594210241,0.607834567338209,
106.760007128635));
#27100=CARTESIAN_POINT('Ctrl Pts',(-2.99262318887305,0.707822939728093,
106.75472985636));
#27101=CARTESIAN_POINT('Ctrl Pts',(-2.96749246796359,0.806688050718487,
106.749452584086));
#27102=CARTESIAN_POINT('Ctrl Pts',(-2.93756412737037,0.903946484913101,
106.744175311811));
#27103=CARTESIAN_POINT('Ctrl Pts',(-2.90755169174042,1.00147820360776,106.738883211036));
#27104=CARTESIAN_POINT('Ctrl Pts',(-2.87271479946202,1.09739387420478,106.733591110261));
#27105=CARTESIAN_POINT('Ctrl Pts',(-2.83326264746127,1.19122836622571,106.728299009486));
#27106=CARTESIAN_POINT('Ctrl Pts',(-2.80029014392485,1.26965141701237,106.723876086967));
#27107=CARTESIAN_POINT('Ctrl Pts',(-2.76409481162807,1.34662108790702,106.719453164447));
#27108=CARTESIAN_POINT('Ctrl Pts',(-2.72482273064761,1.42188021174292,106.715030241928));
#27109=CARTESIAN_POINT('Ctrl Pts',(-2.68043100983037,1.50695036669438,106.710030732435));
#27110=CARTESIAN_POINT('Ctrl Pts',(-2.63197360866318,1.59008905533461,106.705031222942));
#27111=CARTESIAN_POINT('Ctrl Pts',(-2.57964256266102,1.67088195241546,106.700031713449));
#27112=CARTESIAN_POINT('Ctrl Pts',(-2.52738250339044,1.75156525444448,106.695038985759));
#27113=CARTESIAN_POINT('Ctrl Pts',(-2.47125947900096,1.82990872375329,106.690046258069));
#27114=CARTESIAN_POINT('Ctrl Pts',(-2.41151184191223,1.90552168350745,106.685053530379));
#27115=CARTESIAN_POINT('Ctrl Pts',(-2.35182723707464,1.98105487349497,106.680066069891));
#27116=CARTESIAN_POINT('Ctrl Pts',(-2.288525891873,2.05386293783921,106.675078609403));
#27117=CARTESIAN_POINT('Ctrl Pts',(-2.2218893914809,2.12358418293804,106.670091148914));
#27118=CARTESIAN_POINT('Ctrl Pts',(-2.15530057106246,2.19325554085627,106.665107257071));
#27119=CARTESIAN_POINT('Ctrl Pts',(-2.08538164189137,2.25984415387907,106.660123365227));
#27120=CARTESIAN_POINT('Ctrl Pts',(-2.01245375433242,2.32302219891962,106.655139473383));
#27121=CARTESIAN_POINT('Ctrl Pts',(-1.93955242530391,2.38617723608091,106.65015739655));
#27122=CARTESIAN_POINT('Ctrl Pts',(-1.86364464653832,2.44592388593905,106.645175319716));
#27123=CARTESIAN_POINT('Ctrl Pts',(-1.78508692598574,2.50197260510078,106.640193242882));
#27124=CARTESIAN_POINT('Ctrl Pts',(-1.70653636808742,2.55801621391061,106.635211620299));
#27125=CARTESIAN_POINT('Ctrl Pts',(-1.62533670621702,2.61036230757285,106.630229997716));
#27126=CARTESIAN_POINT('Ctrl Pts',(-1.54187501558476,2.6587635634474,106.625248375133));
#27127=CARTESIAN_POINT('Ctrl Pts',(-1.45839815014669,2.70717361952301,106.620265846803));
#27128=CARTESIAN_POINT('Ctrl Pts',(-1.37265881889352,2.75163719318902,106.615283318473));
#27129=CARTESIAN_POINT('Ctrl Pts',(-1.28506942846085,2.79195250927291,106.610300790143));
#27130=CARTESIAN_POINT('Ctrl Pts',(-1.19738562957399,2.83231127932597,106.605312891382));
#27131=CARTESIAN_POINT('Ctrl Pts',(-1.10784818990129,2.86851268159844,106.600324992621));
#27132=CARTESIAN_POINT('Ctrl Pts',(-1.01689005841298,2.90040287875682,106.59533709386));
#27133=CARTESIAN_POINT('Ctrl Pts',(-0.925878196707886,2.93231191389239,
106.590346248679));
#27134=CARTESIAN_POINT('Ctrl Pts',(-0.833444392583745,2.95990454753966,
106.585355403498));
#27135=CARTESIAN_POINT('Ctrl Pts',(-0.740035287971699,2.98307727398347,
106.580364558316));
#27136=CARTESIAN_POINT('Ctrl Pts',(-0.646475231887759,3.00628744813838,
106.575365647803));
#27137=CARTESIAN_POINT('Ctrl Pts',(-0.551937158434959,3.02506336727993,
106.57036673729));
#27138=CARTESIAN_POINT('Ctrl Pts',(-0.45687632976544,3.03935293595529,106.565367826777));
#27139=CARTESIAN_POINT('Ctrl Pts',(-0.401687877380712,3.04764887857936,
106.562465662566));
#27140=CARTESIAN_POINT('Ctrl Pts',(-0.346323316646575,3.05443367349225,
106.559563498355));
#27141=CARTESIAN_POINT('Ctrl Pts',(-0.29087183719041,3.05970518585198,106.556661334144));
#27142=CARTESIAN_POINT('Ctrl Pts',(-0.195371922038768,3.06878391536491,
106.551663154859));
#27143=CARTESIAN_POINT('Ctrl Pts',(-0.0992788561140445,3.07340316998083,
106.546664975575));
#27144=CARTESIAN_POINT('Ctrl Pts',(-0.00304436420393871,3.07349849224733,
106.541666796291));
#27145=CARTESIAN_POINT('Ctrl Pts',(0.0930703047400408,3.07359369582668,
106.536674840312));
#27146=CARTESIAN_POINT('Ctrl Pts',(0.189325615191599,3.0691761555212,106.531682884333));
#27147=CARTESIAN_POINT('Ctrl Pts',(0.28526431249711,3.06023308295554,106.526690928355));
#27148=CARTESIAN_POINT('Ctrl Pts',(0.381109755113251,3.05129870326853,106.521703824676));
#27149=CARTESIAN_POINT('Ctrl Pts',(0.476638761596079,3.03784757214109,106.516716720997));
#27150=CARTESIAN_POINT('Ctrl Pts',(0.571394733447213,3.01991892417475,106.511729617318));
#27151=CARTESIAN_POINT('Ctrl Pts',(0.66608447301117,3.00200280792898,106.506745999512));
#27152=CARTESIAN_POINT('Ctrl Pts',(0.760001822005656,2.97961547692256,106.501762381706));
#27153=CARTESIAN_POINT('Ctrl Pts',(0.852697023548337,2.9528477840945,106.4967787639));
#27154=CARTESIAN_POINT('Ctrl Pts',(0.945373875724465,2.92608539003271,106.49179613262));
#27155=CARTESIAN_POINT('Ctrl Pts',(1.03682863681075,2.89494446814416,106.48681350134));
#27156=CARTESIAN_POINT('Ctrl Pts',(1.12662418519526,2.85956643485216,106.48183087006));
#27157=CARTESIAN_POINT('Ctrl Pts',(1.21640461430721,2.82419435831569,106.476849077727));
#27158=CARTESIAN_POINT('Ctrl Pts',(1.30452597941365,2.78458675430858,106.471867285395));
#27159=CARTESIAN_POINT('Ctrl Pts',(1.39057003262799,2.74093364282264,106.466885493063));
#27160=CARTESIAN_POINT('Ctrl Pts',(1.47666861947242,2.69725286454806,106.461900543334));
#27161=CARTESIAN_POINT('Ctrl Pts',(1.56068687181946,2.64952165515339,106.456915593604));
#27162=CARTESIAN_POINT('Ctrl Pts',(1.64223042811163,2.59797641848118,106.451930643875));
#27163=CARTESIAN_POINT('Ctrl Pts',(1.72139114950026,2.54793741718352,106.447091362458));
#27164=CARTESIAN_POINT('Ctrl Pts',(1.7982195086045,2.49430446352957,106.442252081041));
#27165=CARTESIAN_POINT('Ctrl Pts',(1.87238193903529,2.43733217358128,106.437412799624));
#27166=CARTESIAN_POINT('Ctrl Pts',(1.8723819390353,2.43733217358127,107.437292535812));
#27167=CARTESIAN_POINT('Ctrl Pts',(1.94889495900041,2.37855413822091,107.432310908554));
#27168=CARTESIAN_POINT('Ctrl Pts',(2.02265352062151,2.31615755441516,107.427329281296));
#27169=CARTESIAN_POINT('Ctrl Pts',(2.09330611117521,2.25043812954645,107.422347654038));
#27170=CARTESIAN_POINT('Ctrl Pts',(2.16396476603174,2.18471306380185,107.417365599194));
#27171=CARTESIAN_POINT('Ctrl Pts',(2.23151659924619,2.11566488992335,107.412383544349));
#27172=CARTESIAN_POINT('Ctrl Pts',(2.29564594777291,2.04362715104145,107.407401489504));
#27173=CARTESIAN_POINT('Ctrl Pts',(2.35984093096381,1.97151568347046,107.402414335661));
#27174=CARTESIAN_POINT('Ctrl Pts',(2.42060614030575,1.89640886787032,107.397427181817));
#27175=CARTESIAN_POINT('Ctrl Pts',(2.477665453007,1.81867428446537,107.392440027973));
#27176=CARTESIAN_POINT('Ctrl Pts',(2.53475355975952,1.7409004735711,107.387450357443));
#27177=CARTESIAN_POINT('Ctrl Pts',(2.58813180152419,1.66049661928838,107.382460686914));
#27178=CARTESIAN_POINT('Ctrl Pts',(2.6375679743032,1.57785849521752,107.377471016384));
#27179=CARTESIAN_POINT('Ctrl Pts',(2.68708930554924,1.49507801918921,107.372472750677));
#27180=CARTESIAN_POINT('Ctrl Pts',(2.73265479140424,1.41005597060174,107.367474484969));
#27181=CARTESIAN_POINT('Ctrl Pts',(2.7740786078095,1.32321204940618,107.362476219262));
#27182=CARTESIAN_POINT('Ctrl Pts',(2.81267233143673,1.24230134189105,107.357819437196));
#27183=CARTESIAN_POINT('Ctrl Pts',(2.84767136059942,1.15980968333125,107.353162655131));
#27184=CARTESIAN_POINT('Ctrl Pts',(2.87896424539992,1.07608880846743,107.348505873065));
#27185=CARTESIAN_POINT('Ctrl Pts',(2.91256020767963,0.986206288147527,107.343506363572));
#27186=CARTESIAN_POINT('Ctrl Pts',(2.94200188712549,0.894591066769858,107.338506854079));
#27187=CARTESIAN_POINT('Ctrl Pts',(2.96710950151711,0.801662931665718,107.333507344586));
#27188=CARTESIAN_POINT('Ctrl Pts',(2.99218305758924,0.708860852986766,107.328514616896));
#27189=CARTESIAN_POINT('Ctrl Pts',(3.01293411947688,0.614749820262306,107.323521889206));
#27190=CARTESIAN_POINT('Ctrl Pts',(3.02923145456839,0.51976826052911,107.318529161516));
#27191=CARTESIAN_POINT('Ctrl Pts',(3.04551159638223,0.424886903947011,107.313541701027));
#27192=CARTESIAN_POINT('Ctrl Pts',(3.05734727803285,0.329137276387487,107.308554240539));
#27193=CARTESIAN_POINT('Ctrl Pts',(3.0646577226006,0.232970584633594,107.303566780051));
#27194=CARTESIAN_POINT('Ctrl Pts',(3.07196293637436,0.136872702395668,107.298582888207));
#27195=CARTESIAN_POINT('Ctrl Pts',(3.0747493167053,0.0403587856510456,107.293598996363));
#27196=CARTESIAN_POINT('Ctrl Pts',(3.07298772560659,-0.0561131737763518,
107.28861510452));
#27197=CARTESIAN_POINT('Ctrl Pts',(3.07122677603572,-0.152550000505387,
107.283633027686));
#27198=CARTESIAN_POINT('Ctrl Pts',(3.06492115384708,-0.248944461835907,
107.278650950852));
#27199=CARTESIAN_POINT('Ctrl Pts',(3.05409382664008,-0.344837857664972,
107.273668874019));
#27200=CARTESIAN_POINT('Ctrl Pts',(3.04326748663586,-0.440722510225716,
107.268687251436));
#27201=CARTESIAN_POINT('Ctrl Pts',(3.0279203107254,-0.536105751946442,107.263705628852));
#27202=CARTESIAN_POINT('Ctrl Pts',(3.00812710105997,-0.630534371678943,
107.258724006269));
#27203=CARTESIAN_POINT('Ctrl Pts',(2.98833029264029,-0.724980160198237,
107.25374147794));
#27204=CARTESIAN_POINT('Ctrl Pts',(2.96408593513475,-0.818470552410832,
107.24875894961));
#27205=CARTESIAN_POINT('Ctrl Pts',(2.93551963948931,-0.910563944032784,
107.24377642128));
#27206=CARTESIAN_POINT('Ctrl Pts',(2.90692255358723,-1.00275659875831,107.238788522519));
#27207=CARTESIAN_POINT('Ctrl Pts',(2.87399435971913,-1.09354882683002,107.233800623758));
#27208=CARTESIAN_POINT('Ctrl Pts',(2.83691005410327,-1.18251579056172,107.228812724997));
#27209=CARTESIAN_POINT('Ctrl Pts',(2.79980384227905,-1.27153530830008,107.223821879815));
#27210=CARTESIAN_POINT('Ctrl Pts',(2.75853681795548,-1.35872701822674,107.218831034634));
#27211=CARTESIAN_POINT('Ctrl Pts',(2.71333056440642,-1.44368954358544,107.213840189453));
#27212=CARTESIAN_POINT('Ctrl Pts',(2.66805125641002,-1.5287893705307,107.208841278939));
#27213=CARTESIAN_POINT('Ctrl Pts',(2.61882023196572,-1.61165244254687,107.203842368426));
#27214=CARTESIAN_POINT('Ctrl Pts',(2.56590307268301,-1.69190533765807,107.198843457913));
#27215=CARTESIAN_POINT('Ctrl Pts',(2.53518152137457,-1.7384969058418,107.195941293702));
#27216=CARTESIAN_POINT('Ctrl Pts',(2.50321834242864,-1.78420930261705,107.193039129491));
#27217=CARTESIAN_POINT('Ctrl Pts',(2.47007156829692,-1.82897476677269,107.19013696528));
#27218=CARTESIAN_POINT('Ctrl Pts',(2.41297017778752,-1.90609147924455,107.185137455787));
#27219=CARTESIAN_POINT('Ctrl Pts',(2.35215360522443,-1.98066698312061,107.180137946294));
#27220=CARTESIAN_POINT('Ctrl Pts',(2.28787608227205,-2.05232192459358,107.175138436801));
#27221=CARTESIAN_POINT('Ctrl Pts',(2.22368575137137,-2.12387966659348,107.170145709111));
#27222=CARTESIAN_POINT('Ctrl Pts',(2.15604409120931,-2.19252439589207,107.165152981421));
#27223=CARTESIAN_POINT('Ctrl Pts',(2.08524740120169,-2.25790733330258,107.160160253731));
#27224=CARTESIAN_POINT('Ctrl Pts',(2.01452539991748,-2.32322129336222,107.155172793243));
#27225=CARTESIAN_POINT('Ctrl Pts',(1.94065530636213,-2.38528000601421,107.150185332754));
#27226=CARTESIAN_POINT('Ctrl Pts',(1.86397161018428,-2.44377005596415,107.145197872266));
#27227=CARTESIAN_POINT('Ctrl Pts',(1.78734278298354,-2.50221825491614,107.140213980423));
#27228=CARTESIAN_POINT('Ctrl Pts',(1.70790470332619,-2.55710260187487,107.135230088579));
#27229=CARTESIAN_POINT('Ctrl Pts',(1.6260256669984,-2.60814930175832,107.130246196735));
#27230=CARTESIAN_POINT('Ctrl Pts',(1.54417644898777,-2.65917741169793,107.125264119902));
#27231=CARTESIAN_POINT('Ctrl Pts',(1.45988841264542,-2.7063704193997,107.120282043068));
#27232=CARTESIAN_POINT('Ctrl Pts',(1.37355881682426,-2.74949784992175,107.115299966234));
#27233=CARTESIAN_POINT('Ctrl Pts',(1.28723709227335,-2.79262134821572,107.110318343651));
#27234=CARTESIAN_POINT('Ctrl Pts',(1.19887457110041,-2.8316798103144,107.105336721068));
#27235=CARTESIAN_POINT('Ctrl Pts',(1.10889212946815,-2.86648922816807,107.100355098485));
#27236=CARTESIAN_POINT('Ctrl Pts',(1.01889332744257,-2.90130497498723,107.095372570155));
#27237=CARTESIAN_POINT('Ctrl Pts',(0.927274429425749,-2.93186998493461,
107.090390041825));
#27238=CARTESIAN_POINT('Ctrl Pts',(0.834474238759778,-2.95804918736087,
107.085407513495));
#27239=CARTESIAN_POINT('Ctrl Pts',(0.741574023164935,-2.98425660710911,
107.080419614734));
#27240=CARTESIAN_POINT('Ctrl Pts',(0.64749039615016,-3.00606866243138,107.075431715973));
#27241=CARTESIAN_POINT('Ctrl Pts',(0.552674985253281,-3.02340083526404,
107.070443817212));
#27242=CARTESIAN_POINT('Ctrl Pts',(0.457803565591821,-3.04074324644908,
107.065452972031));
#27243=CARTESIAN_POINT('Ctrl Pts',(0.362199936161149,-3.05360044739323,
107.06046212685));
#27244=CARTESIAN_POINT('Ctrl Pts',(0.266321410047234,-3.0619397702356,107.055471281668));
#27245=CARTESIAN_POINT('Ctrl Pts',(0.170287941813845,-3.07029256963429,
107.050472371155));
#27246=CARTESIAN_POINT('Ctrl Pts',(0.0739791281699808,-3.07411289505045,
107.045473460642));
#27247=CARTESIAN_POINT('Ctrl Pts',(-0.0221472110899903,-3.07342020411153,
107.040474550129));
#27248=CARTESIAN_POINT('Ctrl Pts',(-0.07795425560488,-3.07301805591405,
107.037572385918));
#27249=CARTESIAN_POINT('Ctrl Pts',(-0.133699864030437,-3.07109577378738,
107.034670221707));
#27250=CARTESIAN_POINT('Ctrl Pts',(-0.189295602926625,-3.06766514220712,
107.031768057496));
#27251=CARTESIAN_POINT('Ctrl Pts',(-0.285069447607009,-3.06175525086209,
107.026768548003));
#27252=CARTESIAN_POINT('Ctrl Pts',(-0.380734482790873,-3.05134552848548,
107.02176903851));
#27253=CARTESIAN_POINT('Ctrl Pts',(-0.475834092604759,-3.03644268286345,
107.016769529017));
#27254=CARTESIAN_POINT('Ctrl Pts',(-0.570804700401915,-3.02156005285686,
107.011776801327));
#27255=CARTESIAN_POINT('Ctrl Pts',(-0.665210977222577,-3.00219648017965,
107.006784073637));
#27256=CARTESIAN_POINT('Ctrl Pts',(-0.7585990490962,-2.9784106051232,107.001791345947));
#27257=CARTESIAN_POINT('Ctrl Pts',(-0.851888598907823,-2.95464982356542,
106.996803885459));
#27258=CARTESIAN_POINT('Ctrl Pts',(-0.944161656058873,-2.92647612196491,
106.99181642497));
#27259=CARTESIAN_POINT('Ctrl Pts',(-1.03497321680699,-2.89399942821214,
106.986828964482));
#27260=CARTESIAN_POINT('Ctrl Pts',(-1.12571979976071,-2.86154597229288,
106.981845072639));
#27261=CARTESIAN_POINT('Ctrl Pts',(-1.21500655304231,-2.82479579230485,
106.976861180795));
#27262=CARTESIAN_POINT('Ctrl Pts',(-1.30240330023355,-2.78390874375235,
106.971877288951));
#27263=CARTESIAN_POINT('Ctrl Pts',(-1.38976821969396,-2.7430365852503,106.966895212118));
#27264=CARTESIAN_POINT('Ctrl Pts',(-1.47524410343219,-2.69803073734652,
106.961913135284));
#27265=CARTESIAN_POINT('Ctrl Pts',(-1.55842134264245,-2.64909893526016,
106.95693105845));
#27266=CARTESIAN_POINT('Ctrl Pts',(-1.64159099800491,-2.60017159462675,
106.951949435867));
#27267=CARTESIAN_POINT('Ctrl Pts',(-1.7224620472744,-2.54731923422894,106.946967813284));
#27268=CARTESIAN_POINT('Ctrl Pts',(-1.80065099923461,-2.49079469827511,
106.941986190701));
#27269=CARTESIAN_POINT('Ctrl Pts',(-1.87885416732379,-2.43425988516481,
106.937003662371));
#27270=CARTESIAN_POINT('Ctrl Pts',(-1.95437391391006,-2.37405182771042,
106.932021134041));
#27271=CARTESIAN_POINT('Ctrl Pts',(-2.02685803561019,-2.31046505134408,
106.927038605712));
#27272=CARTESIAN_POINT('Ctrl Pts',(-2.09942028451098,-2.24680973780409,
106.922050706951));
#27273=CARTESIAN_POINT('Ctrl Pts',(-2.16894004583562,-2.17976872487179,
106.91706280819));
#27274=CARTESIAN_POINT('Ctrl Pts',(-2.23510053716642,-2.10967481825005,
106.912074909429));
#27275=CARTESIAN_POINT('Ctrl Pts',(-2.30130011040751,-2.03953950619562,
106.907084064247));
#27276=CARTESIAN_POINT('Ctrl Pts',(-2.36413617665296,-1.9663480425184,106.902093219066));
#27277=CARTESIAN_POINT('Ctrl Pts',(-2.42333234952958,-1.89046623183897,
106.897102373885));
#27278=CARTESIAN_POINT('Ctrl Pts',(-2.4826241849165,-1.81446179423718,106.892103463372));
#27279=CARTESIAN_POINT('Ctrl Pts',(-2.53826412833264,-1.73575868649417,
106.887104552858));
#27280=CARTESIAN_POINT('Ctrl Pts',(-2.59001923998408,-1.6547515180571,106.882105642345));
#27281=CARTESIAN_POINT('Ctrl Pts',(-2.6200661536819,-1.60772204944488,106.879203478134));
#27282=CARTESIAN_POINT('Ctrl Pts',(-2.64880454179271,-1.55991647365968,
106.876301313923));
#27283=CARTESIAN_POINT('Ctrl Pts',(-2.67619614131924,-1.51141538406488,
106.873399149712));
#27284=CARTESIAN_POINT('Ctrl Pts',(-2.72544131435984,-1.42421914174836,
106.868181580047));
#27285=CARTESIAN_POINT('Ctrl Pts',(-2.77049117203041,-1.33449006635661,
106.862964010382));
#27286=CARTESIAN_POINT('Ctrl Pts',(-2.81108935767527,-1.24264993991263,
106.857746440717));
#27287=CARTESIAN_POINT('Ctrl Pts',(-2.85161438327567,-1.15097531415855,
106.852538273385));
#27288=CARTESIAN_POINT('Ctrl Pts',(-2.88770355110402,-1.05719755939782,
106.847330106052));
#27289=CARTESIAN_POINT('Ctrl Pts',(-2.91914588564462,-0.961763769500647,
106.842121938719));
#27290=CARTESIAN_POINT('Ctrl Pts',(-2.95051943878282,-0.86653874495124,
106.836925164467));
#27291=CARTESIAN_POINT('Ctrl Pts',(-2.97726629363181,-0.769665267032493,
106.831728390215));
#27292=CARTESIAN_POINT('Ctrl Pts',(-2.99922360632994,-0.67161001275536,
106.826531615963));
#27293=CARTESIAN_POINT('Ctrl Pts',(-3.02115180119315,-0.573684790634065,
106.821341733211));
#27294=CARTESIAN_POINT('Ctrl Pts',(-3.03830301001062,-0.47458128423278,
106.816151850459));
#27295=CARTESIAN_POINT('Ctrl Pts',(-3.05056405627992,-0.374781521066573,
106.810961967706));
#27296=CARTESIAN_POINT('Ctrl Pts',(-3.06280647431927,-0.275133383862565,
106.805779969952));
#27297=CARTESIAN_POINT('Ctrl Pts',(-3.07017348425895,-0.174791477730663,
106.800597972198));
#27298=CARTESIAN_POINT('Ctrl Pts',(-3.07260306387733,-0.0742473019824065,
106.795415974444));
#27299=CARTESIAN_POINT('Ctrl Pts',(-3.07320310147932,-0.0494157279708957,
106.794136167237));
#27300=CARTESIAN_POINT('Ctrl Pts',(-3.07350222572077,-0.0245718569904162,
106.79285636003));
#27301=CARTESIAN_POINT('Ctrl Pts',(-3.07349998753221,0.000276838377306025,
106.791576552823));
#27302=CARTESIAN_POINT('Origin',(0.,0.,116.208423447177));
#27303=CARTESIAN_POINT('',(1.87238193903529,2.43733217358128,108.437241832237));
#27304=CARTESIAN_POINT('',(1.8723819390353,2.43733217358127,108.354243299745));
#27305=CARTESIAN_POINT('',(1.8723819390353,2.43733217358128,116.208423447177));
#27306=CARTESIAN_POINT('',(-3.07349874901725,0.00277304695061168,107.708423447135));
#27307=CARTESIAN_POINT('Ctrl Pts',(1.8723819390353,2.43733217358127,108.354243299745));
#27308=CARTESIAN_POINT('Ctrl Pts',(1.9489202414689,2.37853471598626,108.349255013332));
#27309=CARTESIAN_POINT('Ctrl Pts',(2.02263916084149,2.31616481968597,108.344266726919));
#27310=CARTESIAN_POINT('Ctrl Pts',(2.09320201927132,2.25053494896624,108.339278440506));
#27311=CARTESIAN_POINT('Ctrl Pts',(2.16380931523457,2.18486374730219,108.334287012678));
#27312=CARTESIAN_POINT('Ctrl Pts',(2.23125628667876,2.11592879743876,108.329295584851));
#27313=CARTESIAN_POINT('Ctrl Pts',(2.29524455677507,2.04407795218148,108.324304157024));
#27314=CARTESIAN_POINT('Ctrl Pts',(2.35933328799668,1.97211430161227,108.319304892691));
#27315=CARTESIAN_POINT('Ctrl Pts',(2.41995220306546,1.89722595814191,108.314305628358));
#27316=CARTESIAN_POINT('Ctrl Pts',(2.47684458529493,1.81979206237834,108.309306364025));
#27317=CARTESIAN_POINT('Ctrl Pts',(2.50081160083218,1.78717153727201,108.307200327307));
#27318=CARTESIAN_POINT('Ctrl Pts',(2.52411782113852,1.75409958665616,108.305094290589));
#27319=CARTESIAN_POINT('Ctrl Pts',(2.54674648514769,1.7206058788659,108.302988253871));
#27320=CARTESIAN_POINT('Ctrl Pts',(2.60046455167701,1.6410953420237,108.297988744378));
#27321=CARTESIAN_POINT('Ctrl Pts',(2.6505498707295,1.55892708725271,108.292989234885));
#27322=CARTESIAN_POINT('Ctrl Pts',(2.69672931841694,1.47446710142698,108.287989725392));
#27323=CARTESIAN_POINT('Ctrl Pts',(2.74284612397695,1.39012168503551,108.282996997702));
#27324=CARTESIAN_POINT('Ctrl Pts',(2.7850673793875,1.30349109781853,108.278004270012));
#27325=CARTESIAN_POINT('Ctrl Pts',(2.82316279249373,1.21497082149284,108.273011542322));
#27326=CARTESIAN_POINT('Ctrl Pts',(2.8612180158994,1.12654393182736,108.268024081834));
#27327=CARTESIAN_POINT('Ctrl Pts',(2.89515587722372,1.03623171722334,108.263036621345));
#27328=CARTESIAN_POINT('Ctrl Pts',(2.92479214191414,0.944453903902824,108.258049160857));
#27329=CARTESIAN_POINT('Ctrl Pts',(2.95440720116434,0.852741759753303,108.253065269013));
#27330=CARTESIAN_POINT('Ctrl Pts',(2.97972664798471,0.759566518119873,108.24808137717));
#27331=CARTESIAN_POINT('Ctrl Pts',(3.00061486013517,0.665366599053461,108.243097485326));
#27332=CARTESIAN_POINT('Ctrl Pts',(3.02149546531612,0.57120098526449,108.238115408492));
#27333=CARTESIAN_POINT('Ctrl Pts',(3.03794794723341,0.476011863589975,108.233133331659));
#27334=CARTESIAN_POINT('Ctrl Pts',(3.04988717324782,0.380250549583362,108.228151254825));
#27335=CARTESIAN_POINT('Ctrl Pts',(3.06182531067985,0.284497966802541,108.223169632242));
#27336=CARTESIAN_POINT('Ctrl Pts',(3.06925095623096,0.188173731027255,108.218188009659));
#27337=CARTESIAN_POINT('Ctrl Pts',(3.07213065521582,0.0917359650475105,
108.213206387076));
#27338=CARTESIAN_POINT('Ctrl Pts',(3.0750108777807,-0.0047193350173881,
108.208223858746));
#27339=CARTESIAN_POINT('Ctrl Pts',(3.07334349921686,-0.101287767518089,
108.203241330416));
#27340=CARTESIAN_POINT('Ctrl Pts',(3.06714717884297,-0.197510590388534,
108.198258802086));
#27341=CARTESIAN_POINT('Ctrl Pts',(3.06094417974892,-0.293837127280852,
108.193270903325));
#27342=CARTESIAN_POINT('Ctrl Pts',(3.05020252157301,-0.389816872067273,
108.188283004564));
#27343=CARTESIAN_POINT('Ctrl Pts',(3.03499280251743,-0.484995813041077,
108.183295105803));
#27344=CARTESIAN_POINT('Ctrl Pts',(3.01977409887207,-0.580230977521588,
108.178304260622));
#27345=CARTESIAN_POINT('Ctrl Pts',(3.00008216854657,-0.674663966759862,
108.173313415441));
#27346=CARTESIAN_POINT('Ctrl Pts',(2.97603839658355,-0.767852662989717,
108.168322570259));
#27347=CARTESIAN_POINT('Ctrl Pts',(2.9519557692778,-0.861191954506244,108.163323659746));
#27348=CARTESIAN_POINT('Ctrl Pts',(2.92350738708946,-0.953282518749631,
108.158324749233));
#27349=CARTESIAN_POINT('Ctrl Pts',(2.89086395801154,-1.04369910715199,108.15332583872));
#27350=CARTESIAN_POINT('Ctrl Pts',(2.87191251022242,-1.0961913024507,108.150423674509));
#27351=CARTESIAN_POINT('Ctrl Pts',(2.85154802208845,-1.14811967283023,108.147521510298));
#27352=CARTESIAN_POINT('Ctrl Pts',(2.82981103644169,-1.19940474737797,108.144619346087));
#27353=CARTESIAN_POINT('Ctrl Pts',(2.79236509672558,-1.28775268306042,108.139619836594));
#27354=CARTESIAN_POINT('Ctrl Pts',(2.75071202868001,-1.37450049686041,108.134620327101));
#27355=CARTESIAN_POINT('Ctrl Pts',(2.70501011654409,-1.45921983244271,108.129620817608));
#27356=CARTESIAN_POINT('Ctrl Pts',(2.6593701987617,-1.54382424678441,108.124628089918));
#27357=CARTESIAN_POINT('Ctrl Pts',(2.60969255896058,-1.62640526853741,108.119635362228));
#27358=CARTESIAN_POINT('Ctrl Pts',(2.55618354123051,-1.70655440978078,108.114642634538));
#27359=CARTESIAN_POINT('Ctrl Pts',(2.50273097416546,-1.78661899570029,108.109655174049));
#27360=CARTESIAN_POINT('Ctrl Pts',(2.44545530687436,-1.86425643817653,108.104667713561));
#27361=CARTESIAN_POINT('Ctrl Pts',(2.38460829568444,-1.93908368209135,108.099680253073));
#27362=CARTESIAN_POINT('Ctrl Pts',(2.32380482195331,-2.01385738536408,108.094696361229));
#27363=CARTESIAN_POINT('Ctrl Pts',(2.25943536044716,-2.0858245477796,108.089712469385));
#27364=CARTESIAN_POINT('Ctrl Pts',(2.19179381478206,-2.15463271196812,108.084728577542));
#27365=CARTESIAN_POINT('Ctrl Pts',(2.12417690249259,-2.22341581792744,108.079746500708));
#27366=CARTESIAN_POINT('Ctrl Pts',(2.05329058106153,-2.2890418987214,108.074764423874));
#27367=CARTESIAN_POINT('Ctrl Pts',(1.97946705989498,-2.35119382629139,108.069782347041));
#27368=CARTESIAN_POINT('Ctrl Pts',(1.90565026973289,-2.41334008703737,108.064800724458));
#27369=CARTESIAN_POINT('Ctrl Pts',(1.82889714820048,-2.47201254177189,108.059819101874));
#27370=CARTESIAN_POINT('Ctrl Pts',(1.74957375070406,-2.52693370329483,108.054837479291));
#27371=CARTESIAN_POINT('Ctrl Pts',(1.67023593081595,-2.58186485045288,108.049854950962));
#27372=CARTESIAN_POINT('Ctrl Pts',(1.58832726777996,-2.63304309999932,108.044872422632));
#27373=CARTESIAN_POINT('Ctrl Pts',(1.50424270999716,-2.68023434039272,108.039889894302));
#27374=CARTESIAN_POINT('Ctrl Pts',(1.42006752145364,-2.72747644598811,108.034901995541));
#27375=CARTESIAN_POINT('Ctrl Pts',(1.33371213943096,-2.77072274785716,108.02991409678));
#27376=CARTESIAN_POINT('Ctrl Pts',(1.2455958227475,-2.80978527584475,108.024926198019));
#27377=CARTESIAN_POINT('Ctrl Pts',(1.15742745454628,-2.8488708786038,108.019935352837));
#27378=CARTESIAN_POINT('Ctrl Pts',(1.06749648950074,-2.8837676277708,108.014944507656));
#27379=CARTESIAN_POINT('Ctrl Pts',(0.976239860858216,-2.91433662847509,
108.009953662475));
#27380=CARTESIAN_POINT('Ctrl Pts',(0.884835759199264,-2.94495502945648,
108.004954751961));
#27381=CARTESIAN_POINT('Ctrl Pts',(0.792102138282386,-2.9712315974102,107.999955841448));
#27382=CARTESIAN_POINT('Ctrl Pts',(0.698488635558885,-2.99307799363717,
107.994956930935));
#27383=CARTESIAN_POINT('Ctrl Pts',(0.644140441777194,-3.00576112311136,
107.992054766724));
#27384=CARTESIAN_POINT('Ctrl Pts',(0.589495847966339,-3.01695202988825,
107.989152602513));
#27385=CARTESIAN_POINT('Ctrl Pts',(0.534643587322916,-3.02664145292013,
107.986250438302));
#27386=CARTESIAN_POINT('Ctrl Pts',(0.44015052012765,-3.04333325907169,107.981250928809));
#27387=CARTESIAN_POINT('Ctrl Pts',(0.344709045236271,-3.05562496958097,
107.976251419316));
#27388=CARTESIAN_POINT('Ctrl Pts',(0.248764642739155,-3.0634161327712,107.971251909823));
#27389=CARTESIAN_POINT('Ctrl Pts',(0.152950388214801,-3.07119672729804,
107.966259182133));
#27390=CARTESIAN_POINT('Ctrl Pts',(0.0566349957276155,-3.07448887249237,
107.961266454443));
#27391=CARTESIAN_POINT('Ctrl Pts',(-0.039726553843952,-3.07324324629856,
107.956273726753));
#27392=CARTESIAN_POINT('Ctrl Pts',(-0.135986444409814,-3.07199893420898,
107.951286266265));
#27393=CARTESIAN_POINT('Ctrl Pts',(-0.232291958666501,-3.06622637310776,
107.946298805777));
#27394=CARTESIAN_POINT('Ctrl Pts',(-0.328184723810764,-3.05592817930285,
107.941311345288));
#27395=CARTESIAN_POINT('Ctrl Pts',(-0.424008875439887,-3.04563735409636,
107.936327453445));
#27396=CARTESIAN_POINT('Ctrl Pts',(-0.519420429860693,-3.03082738030431,
107.931343561601));
#27397=CARTESIAN_POINT('Ctrl Pts',(-0.613963732267965,-3.01155288604726,
107.926359669757));
#27398=CARTESIAN_POINT('Ctrl Pts',(-0.70847260434631,-2.9922854110836,107.921377592924));
#27399=CARTESIAN_POINT('Ctrl Pts',(-0.802113422982623,-2.96855673367534,
107.91639551609));
#27400=CARTESIAN_POINT('Ctrl Pts',(-0.894439311678201,-2.94047284764281,
107.911413439256));
#27401=CARTESIAN_POINT('Ctrl Pts',(-0.98675678237983,-2.91239152221366,
107.906431816673));
#27402=CARTESIAN_POINT('Ctrl Pts',(-1.07775914159711,-2.87995590557865,
107.90145019409));
#27403=CARTESIAN_POINT('Ctrl Pts',(-1.16701433576996,-2.84332196384922,
107.896468571507));
#27404=CARTESIAN_POINT('Ctrl Pts',(-1.25628575811,-2.80668136142361,107.891486043177));
#27405=CARTESIAN_POINT('Ctrl Pts',(-1.34380897845139,-2.76584108463607,
107.886503514848));
#27406=CARTESIAN_POINT('Ctrl Pts',(-1.42917259556581,-2.72100495076428,
107.881520986518));
#27407=CARTESIAN_POINT('Ctrl Pts',(-1.51462822207821,-2.67612049014831,
107.876533087757));
#27408=CARTESIAN_POINT('Ctrl Pts',(-1.59791920899493,-2.62723177848541,
107.871545188996));
#27409=CARTESIAN_POINT('Ctrl Pts',(-1.6786596222819,-2.57458814619356,107.866557290235));
#27410=CARTESIAN_POINT('Ctrl Pts',(-1.7594477300391,-2.52191341658562,107.861566445053));
#27411=CARTESIAN_POINT('Ctrl Pts',(-1.83768190832291,-2.46547960646562,
107.856575599872));
#27412=CARTESIAN_POINT('Ctrl Pts',(-1.91300776419879,-2.40557759054144,
107.851584754691));
#27413=CARTESIAN_POINT('Ctrl Pts',(-1.98845534856018,-2.34557877144665,
107.846585844178));
#27414=CARTESIAN_POINT('Ctrl Pts',(-2.06098489570981,-2.28210084408562,
107.841586933664));
#27415=CARTESIAN_POINT('Ctrl Pts',(-2.13027750201616,-2.21547286474103,
107.836588023151));
#27416=CARTESIAN_POINT('Ctrl Pts',(-2.17050597211508,-2.17679136872447,
107.83368585894));
#27417=CARTESIAN_POINT('Ctrl Pts',(-2.20964415278631,-2.13704881167315,
107.830783694729));
#27418=CARTESIAN_POINT('Ctrl Pts',(-2.24763596500707,-2.09631458011596,
107.827881530518));
#27419=CARTESIAN_POINT('Ctrl Pts',(-2.31279465263703,-2.02645244628409,
107.822904110379));
#27420=CARTESIAN_POINT('Ctrl Pts',(-2.37482199766329,-1.95341089458772,
107.81792669024));
#27421=CARTESIAN_POINT('Ctrl Pts',(-2.43338709172439,-1.87750619488434,
107.812949270101));
#27422=CARTESIAN_POINT('Ctrl Pts',(-2.49142726776055,-1.80228182782095,
107.808016462501));
#27423=CARTESIAN_POINT('Ctrl Pts',(-2.54606669154666,-1.72424576440769,
107.803083654901));
#27424=CARTESIAN_POINT('Ctrl Pts',(-2.59701940177456,-1.64374343399647,
107.7981508473));
#27425=CARTESIAN_POINT('Ctrl Pts',(-2.64792390878895,-1.56331726187013,
107.793222706325));
#27426=CARTESIAN_POINT('Ctrl Pts',(-2.69514838800659,-1.48042983355373,
107.78829456535));
#27427=CARTESIAN_POINT('Ctrl Pts',(-2.73844827237939,-1.39545810023172,
107.783366424374));
#27428=CARTESIAN_POINT('Ctrl Pts',(-2.78171969930191,-1.31054221183658,
107.77844152226));
#27429=CARTESIAN_POINT('Ctrl Pts',(-2.82107145100596,-1.22354513949691,
107.773516620146));
#27430=CARTESIAN_POINT('Ctrl Pts',(-2.85630392453019,-1.13487009860753,
107.768591718033));
#27431=CARTESIAN_POINT('Ctrl Pts',(-2.89217396080832,-1.04459040446457,
107.763577695461));
#27432=CARTESIAN_POINT('Ctrl Pts',(-2.92377393693999,-0.952571834193836,
107.75856367289));
#27433=CARTESIAN_POINT('Ctrl Pts',(-2.95094401222761,-0.859262292142507,
107.753549650319));
#27434=CARTESIAN_POINT('Ctrl Pts',(-2.97762656940174,-0.767627021929973,
107.748625595361));
#27435=CARTESIAN_POINT('Ctrl Pts',(-3.00003679617018,-0.67474718207457,
107.743701540403));
#27436=CARTESIAN_POINT('Ctrl Pts',(-3.01807379931678,-0.581061779742557,
107.738777485445));
#27437=CARTESIAN_POINT('Ctrl Pts',(-3.03660513471701,-0.484808782578329,
107.733718479067));
#27438=CARTESIAN_POINT('Ctrl Pts',(-3.05051992970566,-0.387705913687277,
107.728659472689));
#27439=CARTESIAN_POINT('Ctrl Pts',(-3.05976537292283,-0.29023802759536,
107.723600466311));
#27440=CARTESIAN_POINT('Ctrl Pts',(-3.06901081613999,-0.192770141503442,
107.718541459933));
#27441=CARTESIAN_POINT('Ctrl Pts',(-3.07358690801022,-0.0949377524641238,
107.713482453555));
#27442=CARTESIAN_POINT('Ctrl Pts',(-3.07349874901799,0.00277304613428424,
107.708423447177));
#27443=CARTESIAN_POINT('Ctrl Pts',(-3.07349874901725,0.00277304695062745,
107.708423447135));
#27444=CARTESIAN_POINT('Ctrl Pts',(-3.07338535343165,0.128454723711174,
107.701916240015));
#27445=CARTESIAN_POINT('Ctrl Pts',(-3.06555916854414,0.253796631394034,
107.695409032895));
#27446=CARTESIAN_POINT('Ctrl Pts',(-3.050166873552,0.378000388208786,107.688901825776));
#27447=CARTESIAN_POINT('Ctrl Pts',(-3.03487898698839,0.501361650835883,
107.682438758095));
#27448=CARTESIAN_POINT('Ctrl Pts',(-3.01212748935548,0.623600593083645,
107.675975690415));
#27449=CARTESIAN_POINT('Ctrl Pts',(-2.98210140691276,0.743957961775346,
107.669512622734));
#27450=CARTESIAN_POINT('Ctrl Pts',(-2.95887471463155,0.837060469293967,
107.664513113241));
#27451=CARTESIAN_POINT('Ctrl Pts',(-2.93124299597944,0.929237740901595,
107.659513603748));
#27452=CARTESIAN_POINT('Ctrl Pts',(-2.89929587704686,1.02004199292926,107.654514094255));
#27453=CARTESIAN_POINT('Ctrl Pts',(-2.86739209417824,1.11072306956569,107.649521366565));
#27454=CARTESIAN_POINT('Ctrl Pts',(-2.83118468953308,1.20003441766224,107.644528638875));
#27455=CARTESIAN_POINT('Ctrl Pts',(-2.7908138573318,1.2875403930459,107.639535911185));
#27456=CARTESIAN_POINT('Ctrl Pts',(-2.75048561534092,1.37495405183118,107.634548450696));
#27457=CARTESIAN_POINT('Ctrl Pts',(-2.70600286035394,1.46056572770928,107.629560990208));
#27458=CARTESIAN_POINT('Ctrl Pts',(-2.65755460620401,1.54395782489155,107.62457352972));
#27459=CARTESIAN_POINT('Ctrl Pts',(-2.6091410179124,1.62729025307901,107.619589637876));
#27460=CARTESIAN_POINT('Ctrl Pts',(-2.5567677909679,1.70840588129053,107.614605746033));
#27461=CARTESIAN_POINT('Ctrl Pts',(-2.50067033827754,1.78691077260698,107.609621854189));
#27462=CARTESIAN_POINT('Ctrl Pts',(-2.44459331489007,1.86538707438638,107.604639777355));
#27463=CARTESIAN_POINT('Ctrl Pts',(-2.38479501546821,1.94125417155407,107.599657700522));
#27464=CARTESIAN_POINT('Ctrl Pts',(-2.32155419443271,2.01414705826359,107.594675623688));
#27465=CARTESIAN_POINT('Ctrl Pts',(-2.25831913950307,2.08703329882124,107.589694001105));
#27466=CARTESIAN_POINT('Ctrl Pts',(-2.1916424748109,2.15694553662771,107.584712378522));
#27467=CARTESIAN_POINT('Ctrl Pts',(-2.12184256256027,2.22355265053644,107.579730755939));
#27468=CARTESIAN_POINT('Ctrl Pts',(-2.05202995945583,2.29017187479201,107.574748227609));
#27469=CARTESIAN_POINT('Ctrl Pts',(-1.97909329861193,2.35348447868616,107.569765699279));
#27470=CARTESIAN_POINT('Ctrl Pts',(-1.90338623924964,2.41319768652199,107.564783170949));
#27471=CARTESIAN_POINT('Ctrl Pts',(-1.82759757883496,2.47297525639543,107.559795272188));
#27472=CARTESIAN_POINT('Ctrl Pts',(-1.74903290369471,2.52914541261508,107.554807373427));
#27473=CARTESIAN_POINT('Ctrl Pts',(-1.66807707425214,2.58145717073796,107.549819474666));
#27474=CARTESIAN_POINT('Ctrl Pts',(-1.58707342308996,2.63379983013437,107.544828629485));
#27475=CARTESIAN_POINT('Ctrl Pts',(-1.50367618445484,2.68227933265321,107.539837784304));
#27476=CARTESIAN_POINT('Ctrl Pts',(-1.41829532200881,2.7266904168915,107.534846939122));
#27477=CARTESIAN_POINT('Ctrl Pts',(-1.33277648193289,2.77117327056345,107.529848028609));
#27478=CARTESIAN_POINT('Ctrl Pts',(-1.24526801546849,2.81157439392441,107.524849118096));
#27479=CARTESIAN_POINT('Ctrl Pts',(-1.1562003106438,2.84773648564385,107.519850207583));
#27480=CARTESIAN_POINT('Ctrl Pts',(-1.10449122231035,2.86873072590998,107.516948043372));
#27481=CARTESIAN_POINT('Ctrl Pts',(-1.05225690540002,2.88829712987677,107.514045879161));
#27482=CARTESIAN_POINT('Ctrl Pts',(-0.999583567331795,2.90641272738753,
107.51114371495));
#27483=CARTESIAN_POINT('Ctrl Pts',(-0.90884356227205,2.93762034532239,107.506144176192));
#27484=CARTESIAN_POINT('Ctrl Pts',(-0.816481295459383,2.96462926578446,
107.501144637434));
#27485=CARTESIAN_POINT('Ctrl Pts',(-0.722921168961461,2.9872708671072,107.496145098676));
#27486=CARTESIAN_POINT('Ctrl Pts',(-0.6294881007632,3.00988172025255,107.491152349486));
#27487=CARTESIAN_POINT('Ctrl Pts',(-0.534860828948531,3.0281369394181,107.486159600297));
#27488=CARTESIAN_POINT('Ctrl Pts',(-0.439481103284817,3.04191693013724,
107.481166851107));
#27489=CARTESIAN_POINT('Ctrl Pts',(-0.344202148071791,3.05568236204039,
107.47617937685));
#27490=CARTESIAN_POINT('Ctrl Pts',(-0.248172751548078,3.06498190244422,
107.471191902593));
#27491=CARTESIAN_POINT('Ctrl Pts',(-0.151846102580116,3.06974673403707,
107.466204428336));
#27492=CARTESIAN_POINT('Ctrl Pts',(-0.0555890490807236,3.07450812306557,
107.461220557501));
#27493=CARTESIAN_POINT('Ctrl Pts',(0.0409643927297265,3.07474129518815,
107.456236686666));
#27494=CARTESIAN_POINT('Ctrl Pts',(0.137355626442126,3.07042923414377,107.451252815831));
#27495=CARTESIAN_POINT('Ctrl Pts',(0.233711544263408,3.06611875295548,107.44627077099));
#27496=CARTESIAN_POINT('Ctrl Pts',(0.32990493400896,3.05726636708296,107.44128872615));
#27497=CARTESIAN_POINT('Ctrl Pts',(0.425477872150161,3.04390716519255,107.436306681309));
#27498=CARTESIAN_POINT('Ctrl Pts',(0.521041885408221,3.03054921082386,107.431325101707));
#27499=CARTESIAN_POINT('Ctrl Pts',(0.615985127581939,3.01268533826579,107.426343522104));
#27500=CARTESIAN_POINT('Ctrl Pts',(0.709856535661639,2.99040230550648,107.421361942502));
#27501=CARTESIAN_POINT('Ctrl Pts',(0.803744804035921,2.96811527047955,107.416379468155));
#27502=CARTESIAN_POINT('Ctrl Pts',(0.896560428964477,2.94140760047606,107.411396993808));
#27503=CARTESIAN_POINT('Ctrl Pts',(0.987865296181821,2.91041653489661,107.406414519461));
#27504=CARTESIAN_POINT('Ctrl Pts',(1.07926604503664,2.8793929247858,107.401426812888));
#27505=CARTESIAN_POINT('Ctrl Pts',(1.16915245293809,2.84407708124595,107.396439106314));
#27506=CARTESIAN_POINT('Ctrl Pts',(1.2571045059371,2.80465515013034,107.39145139974));
#27507=CARTESIAN_POINT('Ctrl Pts',(1.3451084356226,2.76520996680979,107.386460751271));
#27508=CARTESIAN_POINT('Ctrl Pts',(1.43117534722427,2.72165407165248,107.381470102802));
#27509=CARTESIAN_POINT('Ctrl Pts',(1.51490990831687,2.67421955338064,107.376479454334));
#27510=CARTESIAN_POINT('Ctrl Pts',(1.59877453701659,2.62671135353448,107.371481053729));
#27511=CARTESIAN_POINT('Ctrl Pts',(1.68029921137597,2.57531273623145,107.366482653124));
#27512=CARTESIAN_POINT('Ctrl Pts',(1.75911776996604,2.52029897460395,107.36148425252));
#27513=CARTESIAN_POINT('Ctrl Pts',(1.79752776191253,2.49348957617218,107.359048423568));
#27514=CARTESIAN_POINT('Ctrl Pts',(1.83529560004653,2.46582225468724,107.356612594616));
#27515=CARTESIAN_POINT('Ctrl Pts',(1.8723819390353,2.43733217358127,107.354176765664));
#27516=CARTESIAN_POINT('',(-3.07349882217909,-0.00269073665490008,107.791576552773));
#27517=CARTESIAN_POINT('Ctrl Pts',(-3.07349882217909,-0.00269073665491237,
107.791576552773));
#27518=CARTESIAN_POINT('Ctrl Pts',(-3.07358187200602,0.0921730787232002,
107.786657377012));
#27519=CARTESIAN_POINT('Ctrl Pts',(-3.06926874327697,0.187176666217751,
107.781738201252));
#27520=CARTESIAN_POINT('Ctrl Pts',(-3.06054730741393,0.281873072643216,
107.776819025491));
#27521=CARTESIAN_POINT('Ctrl Pts',(-3.05183388741077,0.376482443729889,
107.771904370938));
#27522=CARTESIAN_POINT('Ctrl Pts',(-3.03872025258485,0.470784745941165,
107.766989716385));
#27523=CARTESIAN_POINT('Ctrl Pts',(-3.02124633039514,0.564333997800871,
107.762075061832));
#27524=CARTESIAN_POINT('Ctrl Pts',(-3.00378085462675,0.657838030482692,
107.75716278289));
#27525=CARTESIAN_POINT('Ctrl Pts',(-2.98195935853931,0.750589291234735,
107.752250503948));
#27526=CARTESIAN_POINT('Ctrl Pts',(-2.95587337232113,0.842148951672397,
107.747338225007));
#27527=CARTESIAN_POINT('Ctrl Pts',(-2.92979239116969,0.933691044738551,
107.742426888574));
#27528=CARTESIAN_POINT('Ctrl Pts',(-2.89944866934983,1.02404155637932,107.737515552141));
#27529=CARTESIAN_POINT('Ctrl Pts',(-2.86498409547437,1.11277508180176,107.732604215709));
#27530=CARTESIAN_POINT('Ctrl Pts',(-2.83051608758398,1.20151744854199,107.727692389916));
#27531=CARTESIAN_POINT('Ctrl Pts',(-2.7919265779177,1.28864208775896,107.722780564123));
#27532=CARTESIAN_POINT('Ctrl Pts',(-2.7494057890288,1.37374308269594,107.71786873833));
#27533=CARTESIAN_POINT('Ctrl Pts',(-2.70684237480604,1.45892938786388,107.712951988634));
#27534=CARTESIAN_POINT('Ctrl Pts',(-2.66034001805582,1.5420875940516,107.708035238939));
#27535=CARTESIAN_POINT('Ctrl Pts',(-2.61013494930664,1.62283634307593,107.703118489243));
#27536=CARTESIAN_POINT('Ctrl Pts',(-2.55990223283484,1.70362956010058,107.698199031914));
#27537=CARTESIAN_POINT('Ctrl Pts',(-2.5059630043373,1.78201030768138,107.693279574585));
#27538=CARTESIAN_POINT('Ctrl Pts',(-2.44859557061089,1.85762805254032,107.688360117256));
#27539=CARTESIAN_POINT('Ctrl Pts',(-2.39113686525471,1.93336610528762,107.683432833066));
#27540=CARTESIAN_POINT('Ctrl Pts',(-2.33023935839614,2.00633203475412,107.678505548877));
#27541=CARTESIAN_POINT('Ctrl Pts',(-2.26621999102241,2.07621029818523,107.673578264687));
#27542=CARTESIAN_POINT('Ctrl Pts',(-2.23012341355619,2.11561034621164,107.670800072669));
#27543=CARTESIAN_POINT('Ctrl Pts',(-2.1930350019475,2.1540294738056,107.668021880651));
#27544=CARTESIAN_POINT('Ctrl Pts',(-2.15501616577193,2.19141679633557,107.665243688633));
#27545=CARTESIAN_POINT('Ctrl Pts',(-2.08659917690485,2.25869734162871,107.66024417914));
#27546=CARTESIAN_POINT('Ctrl Pts',(-2.01490820660401,2.32288897701853,107.655244669647));
#27547=CARTESIAN_POINT('Ctrl Pts',(-1.94025347588031,2.38365658166909,107.650245160154));
#27548=CARTESIAN_POINT('Ctrl Pts',(-1.86570001382474,2.44434175544985,107.645252432464));
#27549=CARTESIAN_POINT('Ctrl Pts',(-1.78819111899622,2.50161185473757,107.640259704774));
#27550=CARTESIAN_POINT('Ctrl Pts',(-1.70807380396321,2.55516851307593,107.635266977084));
#27551=CARTESIAN_POINT('Ctrl Pts',(-1.62804101067826,2.60866867048961,107.630279516596));
#27552=CARTESIAN_POINT('Ctrl Pts',(-1.54540563062879,2.65846293222671,107.625292056108));
#27553=CARTESIAN_POINT('Ctrl Pts',(-1.46054689172002,2.70429381301052,107.620304595619));
#27554=CARTESIAN_POINT('Ctrl Pts',(-1.37574887122236,2.75009190072792,107.615320703776));
#27555=CARTESIAN_POINT('Ctrl Pts',(-1.28873103955456,2.79193203711114,107.610336811932));
#27556=CARTESIAN_POINT('Ctrl Pts',(-1.19989984636383,2.82960113950643,107.605352920088));
#27557=CARTESIAN_POINT('Ctrl Pts',(-1.1111010032936,2.86725652374756,107.600370843255));
#27558=CARTESIAN_POINT('Ctrl Pts',(-1.02049051452175,2.90074372086698,107.595388766421));
#27559=CARTESIAN_POINT('Ctrl Pts',(-0.928496691140395,2.92989695118128,
107.590406689587));
#27560=CARTESIAN_POINT('Ctrl Pts',(-0.836511255476247,2.95904752339264,
107.585425067004));
#27561=CARTESIAN_POINT('Ctrl Pts',(-0.743143154476894,2.98386478201134,
107.580443444421));
#27562=CARTESIAN_POINT('Ctrl Pts',(-0.648836790001705,3.00423252594407,
107.575461821838));
#27563=CARTESIAN_POINT('Ctrl Pts',(-0.55451327896797,3.02460397309149,107.570479293508));
#27564=CARTESIAN_POINT('Ctrl Pts',(-0.459251594733273,3.04052420624508,
107.565496765178));
#27565=CARTESIAN_POINT('Ctrl Pts',(-0.363506224416851,3.05192815688872,
107.560514236849));
#27566=CARTESIAN_POINT('Ctrl Pts',(-0.267657654701984,3.06334439931047,
107.555526338088));
#27567=CARTESIAN_POINT('Ctrl Pts',(-0.171324794697769,3.07023458893297,
107.550538439326));
#27568=CARTESIAN_POINT('Ctrl Pts',(-0.0749669244908475,3.07258559038351,
107.545550540565));
#27569=CARTESIAN_POINT('Ctrl Pts',(0.0214478656326629,3.07493798060288,
107.540559695384));
#27570=CARTESIAN_POINT('Ctrl Pts',(0.117887256732058,3.0727458535934,107.535568850203));
#27571=CARTESIAN_POINT('Ctrl Pts',(0.213894429392107,3.06604817690052,107.530578005021));
#27572=CARTESIAN_POINT('Ctrl Pts',(0.310056752067661,3.05933967659297,107.525579094508));
#27573=CARTESIAN_POINT('Ctrl Pts',(0.405785025922154,3.04811113899372,107.520580183995));
#27574=CARTESIAN_POINT('Ctrl Pts',(0.500630050715323,3.03245309977265,107.515581273482));
#27575=CARTESIAN_POINT('Ctrl Pts',(0.555693216143185,3.02336267878551,107.512679109271));
#27576=CARTESIAN_POINT('Ctrl Pts',(0.610458900941498,3.01278025014732,107.50977694506));
#27577=CARTESIAN_POINT('Ctrl Pts',(0.664841586868444,3.0007312299455,107.506874780849));
#27578=CARTESIAN_POINT('Ctrl Pts',(0.758533573162282,2.9799728467145,107.501874852566));
#27579=CARTESIAN_POINT('Ctrl Pts',(0.851416994428939,2.95478576871685,107.496874924283));
#27580=CARTESIAN_POINT('Ctrl Pts',(0.94304174075739,2.92524777158949,107.491874996));
#27581=CARTESIAN_POINT('Ctrl Pts',(1.03451892702328,2.89575734489346,107.486883120014));
#27582=CARTESIAN_POINT('Ctrl Pts',(1.12474105646772,2.86193007146443,107.481891244029));
#27583=CARTESIAN_POINT('Ctrl Pts',(1.21326915473125,2.82389451080909,107.476899368043));
#27584=CARTESIAN_POINT('Ctrl Pts',(1.3017145830081,2.78589446881228,107.47191215361));
#27585=CARTESIAN_POINT('Ctrl Pts',(1.38846872151956,2.74369411797663,107.466924939176));
#27586=CARTESIAN_POINT('Ctrl Pts',(1.4731091828196,2.69747133172765,107.461937724742));
#27587=CARTESIAN_POINT('Ctrl Pts',(1.55769020176563,2.65128100739089,107.456954012792));
#27588=CARTESIAN_POINT('Ctrl Pts',(1.6401601100366,2.60107407253766,107.451970300841));
#27589=CARTESIAN_POINT('Ctrl Pts',(1.72011892292524,2.54707540936552,107.44698658889));
#27590=CARTESIAN_POINT('Ctrl Pts',(1.77196280848986,2.5120636275118,107.443755237864));
#27591=CARTESIAN_POINT('Ctrl Pts',(1.82275148441596,2.47545876455751,107.440523886838));
#27592=CARTESIAN_POINT('Ctrl Pts',(1.8723819390353,2.43733217358127,107.437292535812));
#27593=CARTESIAN_POINT('Ctrl Pts',(1.87238193903529,2.43733217358128,108.437241832237));
#27594=CARTESIAN_POINT('Ctrl Pts',(1.94865272942512,2.37874022130256,108.432250974061));
#27595=CARTESIAN_POINT('Ctrl Pts',(2.02227039622087,2.31648811211804,108.427260115884));
#27596=CARTESIAN_POINT('Ctrl Pts',(2.09286615451889,2.25084728697202,108.422269257707));
#27597=CARTESIAN_POINT('Ctrl Pts',(2.16568347076244,2.18314082927003,108.417121343627));
#27598=CARTESIAN_POINT('Ctrl Pts',(2.23528511606183,2.11182907458801,108.411973429546));
#27599=CARTESIAN_POINT('Ctrl Pts',(2.30130181357665,2.03725604989378,108.406825515465));
#27600=CARTESIAN_POINT('Ctrl Pts',(2.36520480718796,1.96507068316075,108.401842425838));
#27601=CARTESIAN_POINT('Ctrl Pts',(2.4257486140982,1.88983006461674,108.396859336211));
#27602=CARTESIAN_POINT('Ctrl Pts',(2.48263561520456,1.8118837302978,108.391876246583));
#27603=CARTESIAN_POINT('Ctrl Pts',(2.53950742813583,1.73395820675374,108.386894487384));
#27604=CARTESIAN_POINT('Ctrl Pts',(2.59272411674773,1.65332875733658,108.381912728184));
#27605=CARTESIAN_POINT('Ctrl Pts',(2.64202944337277,1.57037660144036,108.376930968984));
#27606=CARTESIAN_POINT('Ctrl Pts',(2.69133506624758,1.48742394712827,108.371949179852));
#27607=CARTESIAN_POINT('Ctrl Pts',(2.73672905683115,1.40214893640555,108.36696739072));
#27608=CARTESIAN_POINT('Ctrl Pts',(2.77800003571611,1.31495933456563,108.361985601587));
#27609=CARTESIAN_POINT('Ctrl Pts',(2.81928252927881,1.22774540666913,108.357002422527));
#27610=CARTESIAN_POINT('Ctrl Pts',(2.85643953838532,1.13861622323021,108.352019243466));
#27611=CARTESIAN_POINT('Ctrl Pts',(2.88930736521566,1.04800057219,108.347036064405));
#27612=CARTESIAN_POINT('Ctrl Pts',(2.92221231123304,0.957282584621167,108.342047257606));
#27613=CARTESIAN_POINT('Ctrl Pts',(2.95081825925177,0.865075192659291,108.337058450806));
#27614=CARTESIAN_POINT('Ctrl Pts',(2.97501113763128,0.771823153947734,108.332069644006));
#27615=CARTESIAN_POINT('Ctrl Pts',(2.99922041557854,0.678507902703052,108.327077455456));
#27616=CARTESIAN_POINT('Ctrl Pts',(3.01901057937577,0.584147023968748,108.322085266906));
#27617=CARTESIAN_POINT('Ctrl Pts',(3.03431890787338,0.489194251113101,108.317093078356));
#27618=CARTESIAN_POINT('Ctrl Pts',(3.04965043232491,0.394097601011497,108.312093325389));
#27619=CARTESIAN_POINT('Ctrl Pts',(3.06048652234468,0.298407702000529,108.307093572422));
#27620=CARTESIAN_POINT('Ctrl Pts',(3.06681640165786,0.202581856350362,108.302093819456));
#27621=CARTESIAN_POINT('Ctrl Pts',(3.06824048373387,0.181023172138915,108.300968986227));
#27622=CARTESIAN_POINT('Ctrl Pts',(3.0694366926648,0.159457597829568,108.299844152998));
#27623=CARTESIAN_POINT('Ctrl Pts',(3.07040526815994,0.137890316033002,108.29871931977));
#27624=CARTESIAN_POINT('Ctrl Pts',(3.07471026401134,0.0420309234243816,
108.293719810277));
#27625=CARTESIAN_POINT('Ctrl Pts',(3.07452936043881,-0.0541986383047818,
108.288720300784));
#27626=CARTESIAN_POINT('Ctrl Pts',(3.06982068590681,-0.150343627662216,
108.283720791291));
#27627=CARTESIAN_POINT('Ctrl Pts',(3.06511839866191,-0.24635819695208,108.278728063601));
#27628=CARTESIAN_POINT('Ctrl Pts',(3.05590056835112,-0.342287987185902,
108.273735335911));
#27629=CARTESIAN_POINT('Ctrl Pts',(3.04217725314545,-0.437675462465506,
108.268742608221));
#27630=CARTESIAN_POINT('Ctrl Pts',(3.02846841569141,-0.532962306363106,
108.263755147732));
#27631=CARTESIAN_POINT('Ctrl Pts',(3.01026360454042,-0.627707540485188,
108.258767687244));
#27632=CARTESIAN_POINT('Ctrl Pts',(2.98762481780021,-0.721456996683966,
108.253780226756));
#27633=CARTESIAN_POINT('Ctrl Pts',(2.96500222964111,-0.815139372955408,
108.248796334912));
#27634=CARTESIAN_POINT('Ctrl Pts',(2.93795207564211,-0.907826962250595,
108.243812443068));
#27635=CARTESIAN_POINT('Ctrl Pts',(2.90658757484791,-0.999075032087041,
108.238828551225));
#27636=CARTESIAN_POINT('Ctrl Pts',(2.87523449622809,-1.09028987163643,108.233846474391));
#27637=CARTESIAN_POINT('Ctrl Pts',(2.83957033511733,-1.18006581863036,108.228864397557));
#27638=CARTESIAN_POINT('Ctrl Pts',(2.79975810543389,-1.2679735017173,108.223882320724));
#27639=CARTESIAN_POINT('Ctrl Pts',(2.75994950570858,-1.35587316964881,108.218900698141));
#27640=CARTESIAN_POINT('Ctrl Pts',(2.7159937706197,-1.44190451255567,108.213919075557));
#27641=CARTESIAN_POINT('Ctrl Pts',(2.66810154393361,-1.52565933329138,108.208937452974));
#27642=CARTESIAN_POINT('Ctrl Pts',(2.62020060959689,-1.60942938212918,108.203954924645));
#27643=CARTESIAN_POINT('Ctrl Pts',(2.56836198016065,-1.69092170572518,108.198972396315));
#27644=CARTESIAN_POINT('Ctrl Pts',(2.51284107052908,-1.76975478647814,108.193989867985));
#27645=CARTESIAN_POINT('Ctrl Pts',(2.45726031753948,-1.84867283767389,108.189001969224));
#27646=CARTESIAN_POINT('Ctrl Pts',(2.39798961388014,-1.92492556429635,108.184014070463));
#27647=CARTESIAN_POINT('Ctrl Pts',(2.33532620329136,-1.99816259954508,108.179026171702));
#27648=CARTESIAN_POINT('Ctrl Pts',(2.2726257765659,-2.07144289691571,108.17403532652));
#27649=CARTESIAN_POINT('Ctrl Pts',(2.20652895301756,-2.14170363626027,108.169044481339));
#27650=CARTESIAN_POINT('Ctrl Pts',(2.13737008268124,-2.2086311099093,108.164053636158));
#27651=CARTESIAN_POINT('Ctrl Pts',(2.06809944986392,-2.27566674004593,108.159054725645));
#27652=CARTESIAN_POINT('Ctrl Pts',(1.99575721875222,-2.33935805868163,108.154055815131));
#27653=CARTESIAN_POINT('Ctrl Pts',(1.92071099964292,-2.39943149638632,108.149056904618));
#27654=CARTESIAN_POINT('Ctrl Pts',(1.87714221586565,-2.4343076920052,108.146154740407));
#27655=CARTESIAN_POINT('Ctrl Pts',(1.83266261781819,-2.46796528230611,108.143252576196));
#27656=CARTESIAN_POINT('Ctrl Pts',(1.78734827456117,-2.50035765350143,108.140350411985));
#27657=CARTESIAN_POINT('Ctrl Pts',(1.70928601729026,-2.55615944675534,108.135350902492));
#27658=CARTESIAN_POINT('Ctrl Pts',(1.62847091007281,-2.60840004133588,108.130351392999));
#27659=CARTESIAN_POINT('Ctrl Pts',(1.54526158954139,-2.65679673100672,108.125351883506));
#27660=CARTESIAN_POINT('Ctrl Pts',(1.4621651419249,-2.70512777087534,108.120359155816));
#27661=CARTESIAN_POINT('Ctrl Pts',(1.37668131185539,-2.74962504996746,108.115366428126));
#27662=CARTESIAN_POINT('Ctrl Pts',(1.28919935310137,-2.79004789886536,108.110373700436));
#27663=CARTESIAN_POINT('Ctrl Pts',(1.20180968560867,-2.83042810267661,108.105386239948));
#27664=CARTESIAN_POINT('Ctrl Pts',(1.11242647631956,-2.86674223814872,108.100398779459));
#27665=CARTESIAN_POINT('Ctrl Pts',(1.02146443293911,-2.8987950362591,108.095411318971));
#27666=CARTESIAN_POINT('Ctrl Pts',(0.930567475027023,-2.93082489984317,
108.090427427128));
#27667=CARTESIAN_POINT('Ctrl Pts',(0.838094341622891,-2.95859934203647,
108.085443535284));
#27668=CARTESIAN_POINT('Ctrl Pts',(0.744479713187609,-2.98197119480589,
108.08045964344));
#27669=CARTESIAN_POINT('Ctrl Pts',(0.650899176881401,-3.0053345361254,108.075477566607));
#27670=CARTESIAN_POINT('Ctrl Pts',(0.556178396957965,-3.02429836741274,
108.070495489773));
#27671=CARTESIAN_POINT('Ctrl Pts',(0.460766279976702,-3.03876565158231,
108.065513412939));
#27672=CARTESIAN_POINT('Ctrl Pts',(0.365362862382369,-3.05323161666886,
108.060531790356));
#27673=CARTESIAN_POINT('Ctrl Pts',(0.269268667082403,-3.06320178413063,
108.055550167773));
#27674=CARTESIAN_POINT('Ctrl Pts',(0.172940772021517,-3.06863059676016,
108.05056854519));
#27675=CARTESIAN_POINT('Ctrl Pts',(0.0765953628520557,-3.07406039644347,
108.04558601686));
#27676=CARTESIAN_POINT('Ctrl Pts',(-0.019983392200641,-3.07494717679239,
108.04060348853));
#27677=CARTESIAN_POINT('Ctrl Pts',(-0.116336418072692,-3.07129746000449,
108.0356209602));
#27678=CARTESIAN_POINT('Ctrl Pts',(-0.212793298306262,-3.06764380935978,
108.030633061439));
#27679=CARTESIAN_POINT('Ctrl Pts',(-0.309023524252548,-3.05944391643599,
108.025645162678));
#27680=CARTESIAN_POINT('Ctrl Pts',(-0.404571376123934,-3.04675634923786,
108.020657263917));
#27681=CARTESIAN_POINT('Ctrl Pts',(-0.500175669422909,-3.03406128731963,
108.015666418736));
#27682=CARTESIAN_POINT('Ctrl Pts',(-0.595096354297082,-3.01687335086801,
108.010675573555));
#27683=CARTESIAN_POINT('Ctrl Pts',(-0.688888257775055,-2.99530219148246,
108.005684728373));
#27684=CARTESIAN_POINT('Ctrl Pts',(-0.782831731337599,-2.97369617255861,
108.00068581786));
#27685=CARTESIAN_POINT('Ctrl Pts',(-0.875642358700166,-2.94769290506496,
107.995686907347));
#27686=CARTESIAN_POINT('Ctrl Pts',(-0.966890525935409,-2.91745179237916,
107.990687996834));
#27687=CARTESIAN_POINT('Ctrl Pts',(-1.01986550209675,-2.89989503181987,
107.987785832623));
#27688=CARTESIAN_POINT('Ctrl Pts',(-1.07231421576993,-2.88091081570988,
107.984883668412));
#27689=CARTESIAN_POINT('Ctrl Pts',(-1.12415615175069,-2.86053757124095,
107.981981504201));
#27690=CARTESIAN_POINT('Ctrl Pts',(-1.21346338326081,-2.82544092552398,
107.976981994708));
#27691=CARTESIAN_POINT('Ctrl Pts',(-1.30128230224839,-2.78609631033271,
107.971982485215));
#27692=CARTESIAN_POINT('Ctrl Pts',(-1.387180516629,-2.74265062745602,107.966982975722));
#27693=CARTESIAN_POINT('Ctrl Pts',(-1.4729622106272,-2.6992638783723,107.961990248032));
#27694=CARTESIAN_POINT('Ctrl Pts',(-1.55682798976619,-2.6517873142658,107.956997520342));
#27695=CARTESIAN_POINT('Ctrl Pts',(-1.63836405257318,-2.60041640535434,
107.952004792652));
#27696=CARTESIAN_POINT('Ctrl Pts',(-1.71981409688917,-2.54909969145688,
107.947017332164));
#27697=CARTESIAN_POINT('Ctrl Pts',(-1.79893894139432,-2.49389703282588,
107.942029871675));
#27698=CARTESIAN_POINT('Ctrl Pts',(-1.87534900768155,-2.43504996856078,
107.937042411187));
#27699=CARTESIAN_POINT('Ctrl Pts',(-1.95170440078025,-2.37624501074571,
107.932058519344));
#27700=CARTESIAN_POINT('Ctrl Pts',(-2.0253485304533,-2.31380109826874,107.9270746275));
#27701=CARTESIAN_POINT('Ctrl Pts',(-2.09592129083439,-2.24800271188162,
107.922090735656));
#27702=CARTESIAN_POINT('Ctrl Pts',(-2.16646835036403,-2.18222828763719,
107.917108658823));
#27703=CARTESIAN_POINT('Ctrl Pts',(-2.23394594223746,-2.11310211573858,
107.912126581989));
#27704=CARTESIAN_POINT('Ctrl Pts',(-2.29802826461889,-2.04094790355185,
107.907144505155));
#27705=CARTESIAN_POINT('Ctrl Pts',(-2.36210474416887,-1.96880027016696,
107.902162882572));
#27706=CARTESIAN_POINT('Ctrl Pts',(-2.4227862783556,-1.89362547373688,107.897181259989));
#27707=CARTESIAN_POINT('Ctrl Pts',(-2.47978579734442,-1.81578210402265,
107.892199637406));
#27708=CARTESIAN_POINT('Ctrl Pts',(-2.53679567985015,-1.73792458101216,
107.887217109076));
#27709=CARTESIAN_POINT('Ctrl Pts',(-2.59012195831713,-1.65739787530658,
107.882234580746));
#27710=CARTESIAN_POINT('Ctrl Pts',(-2.63952015937921,-1.57459060654849,
107.877252052417));
#27711=CARTESIAN_POINT('Ctrl Pts',(-2.68897160442178,-1.49169408375873,
107.872264153656));
#27712=CARTESIAN_POINT('Ctrl Pts',(-2.73448629423355,-1.40651246813084,
107.867276254895));
#27713=CARTESIAN_POINT('Ctrl Pts',(-2.7758652378553,-1.31945990134849,107.862288356134));
#27714=CARTESIAN_POINT('Ctrl Pts',(-2.81726862458697,-1.23235591142012,
107.857297510952));
#27715=CARTESIAN_POINT('Ctrl Pts',(-2.85453123114773,-1.1433791744113,107.852306665771));
#27716=CARTESIAN_POINT('Ctrl Pts',(-2.88750265733404,-1.05296279796052,
107.84731582059));
#27717=CARTESIAN_POINT('Ctrl Pts',(-2.92052736617773,-0.962400306362025,
107.842316910077));
#27718=CARTESIAN_POINT('Ctrl Pts',(-2.94924691696304,-0.870393948568264,
107.837317999563));
#27719=CARTESIAN_POINT('Ctrl Pts',(-2.97356111204,-0.777390868844901,107.83231908905));
#27720=CARTESIAN_POINT('Ctrl Pts',(-2.98767694519709,-0.723397061839775,
107.829416924839));
#27721=CARTESIAN_POINT('Ctrl Pts',(-3.0003089152176,-0.669067499346808,
107.826514760628));
#27722=CARTESIAN_POINT('Ctrl Pts',(-3.01144541790491,-0.614490638642712,
107.823612596417));
#27723=CARTESIAN_POINT('Ctrl Pts',(-3.03868361335523,-0.481003920176118,
107.816514343202));
#27724=CARTESIAN_POINT('Ctrl Pts',(-3.057053505008,-0.345651342796672,107.809416089987));
#27725=CARTESIAN_POINT('Ctrl Pts',(-3.06635784075599,-0.209408315103014,
107.802317836772));
#27726=CARTESIAN_POINT('Ctrl Pts',(-3.07105103823203,-0.140686006383854,
107.798737408789));
#27727=CARTESIAN_POINT('Ctrl Pts',(-3.07343837424032,-0.0717374795268788,
107.795156980806));
#27728=CARTESIAN_POINT('Ctrl Pts',(-3.07349882217824,-0.00269073762031292,
107.791576552823));
#27729=CARTESIAN_POINT('Origin',(0.,0.,116.208423447177));
#27730=CARTESIAN_POINT('',(1.87238193903529,2.43733217358128,109.437414079767));
#27731=CARTESIAN_POINT('',(1.8723819390353,2.43733217358128,109.354106889186));
#27732=CARTESIAN_POINT('',(1.8723819390353,2.43733217358128,116.208423447177));
#27733=CARTESIAN_POINT('',(-3.07349984408606,-0.00097898058431413,108.708423447223));
#27734=CARTESIAN_POINT('Ctrl Pts',(1.8723819390353,2.43733217358128,109.354106889186));
#27735=CARTESIAN_POINT('Ctrl Pts',(1.9488625296069,2.37857905079185,109.349124610237));
#27736=CARTESIAN_POINT('Ctrl Pts',(2.02261135197631,2.31619480280882,109.344142331288));
#27737=CARTESIAN_POINT('Ctrl Pts',(2.09327238020598,2.25046950485155,109.339160052339));
#27738=CARTESIAN_POINT('Ctrl Pts',(2.16392383385049,2.18475311268688,109.33417844849));
#27739=CARTESIAN_POINT('Ctrl Pts',(2.23148800372025,2.11569686945201,109.32919684464));
#27740=CARTESIAN_POINT('Ctrl Pts',(2.29564394264312,2.04362940344035,109.324215240791));
#27741=CARTESIAN_POINT('Ctrl Pts',(2.35980870268412,1.97155202851547,109.319232951996));
#27742=CARTESIAN_POINT('Ctrl Pts',(2.42056400940447,1.89646293660758,109.314250663202));
#27743=CARTESIAN_POINT('Ctrl Pts',(2.47762832376815,1.81872486629007,109.309268374407));
#27744=CARTESIAN_POINT('Ctrl Pts',(2.53475273694755,1.74090492403534,109.304280838381));
#27745=CARTESIAN_POINT('Ctrl Pts',(2.58817813514947,1.66043078696199,109.299293302355));
#27746=CARTESIAN_POINT('Ctrl Pts',(2.6376656962614,1.57769513048809,109.294305766329));
#27747=CARTESIAN_POINT('Ctrl Pts',(2.68718052328823,1.49491388956193,109.289315482345));
#27748=CARTESIAN_POINT('Ctrl Pts',(2.73275298501038,1.40986903470771,109.284325198361));
#27749=CARTESIAN_POINT('Ctrl Pts',(2.77419073716893,1.3229769475717,109.279334914377));
#27750=CARTESIAN_POINT('Ctrl Pts',(2.81569745690376,1.23594024022016,109.274336324736));
#27751=CARTESIAN_POINT('Ctrl Pts',(2.85305555124296,1.14705056442657,109.269337735094));
#27752=CARTESIAN_POINT('Ctrl Pts',(2.88612121697342,1.0567433798874,109.264339145452));
#27753=CARTESIAN_POINT('Ctrl Pts',(2.91067927939797,0.989671708221202,109.260626663827));
#27754=CARTESIAN_POINT('Ctrl Pts',(2.93287061027351,0.921818508434118,109.256914182201));
#27755=CARTESIAN_POINT('Ctrl Pts',(2.95265448210382,0.853366134383247,109.253201700576));
#27756=CARTESIAN_POINT('Ctrl Pts',(2.97929694528728,0.761182972709294,109.248202191083));
#27757=CARTESIAN_POINT('Ctrl Pts',(3.00166506851,0.667589018095253,109.24320268159));
#27758=CARTESIAN_POINT('Ctrl Pts',(3.01961161181223,0.573016547587191,109.238203172097));
#27759=CARTESIAN_POINT('Ctrl Pts',(3.03753381074247,0.478572364034679,109.233210444407));
#27760=CARTESIAN_POINT('Ctrl Pts',(3.05104626893321,0.383152730186458,109.228217716717));
#27761=CARTESIAN_POINT('Ctrl Pts',(3.06005157631718,0.28720480545898,109.223224989027));
#27762=CARTESIAN_POINT('Ctrl Pts',(3.06904738332882,0.191358103373958,109.218237528538));
#27763=CARTESIAN_POINT('Ctrl Pts',(3.07354545124736,0.0949846530728144,
109.21325006805));
#27764=CARTESIAN_POINT('Ctrl Pts',(3.0734996534705,-0.00145949192962973,
109.208262607562));
#27765=CARTESIAN_POINT('Ctrl Pts',(3.07345388846303,-0.0978346288922086,
109.203278715718));
#27766=CARTESIAN_POINT('Ctrl Pts',(3.0688707212837,-0.194279922294424,109.198294823875));
#27767=CARTESIAN_POINT('Ctrl Pts',(3.05975603135353,-0.290336492015243,
109.193310932031));
#27768=CARTESIAN_POINT('Ctrl Pts',(3.05064466076767,-0.386358080312533,
109.188328855197));
#27769=CARTESIAN_POINT('Ctrl Pts',(3.03700508775893,-0.481990789647019,
109.183346778363));
#27770=CARTESIAN_POINT('Ctrl Pts',(3.01889519957126,-0.576779007944624,
109.17836470153));
#27771=CARTESIAN_POINT('Ctrl Pts',(3.00078696258817,-0.671558583740493,
109.173383078947));
#27772=CARTESIAN_POINT('Ctrl Pts',(2.97820930334661,-0.765493390456918,
109.168401456363));
#27773=CARTESIAN_POINT('Ctrl Pts',(2.95127137398542,-0.858137242574983,
109.16341983378));
#27774=CARTESIAN_POINT('Ctrl Pts',(2.92432854683401,-0.950797938977824,
109.158437305451));
#27775=CARTESIAN_POINT('Ctrl Pts',(2.89302399770608,-1.04216679314023,109.153454777121));
#27776=CARTESIAN_POINT('Ctrl Pts',(2.8575166542334,-1.1318130679484,109.148472248791));
#27777=CARTESIAN_POINT('Ctrl Pts',(2.82197103907754,-1.22155596822871,109.14348435003));
#27778=CARTESIAN_POINT('Ctrl Pts',(2.78221374777995,-1.3095721736594,109.138496451269));
#27779=CARTESIAN_POINT('Ctrl Pts',(2.73845167054005,-1.39545143165802,109.133508552508));
#27780=CARTESIAN_POINT('Ctrl Pts',(2.69466374244047,-1.48138141971308,109.128517707326));
#27781=CARTESIAN_POINT('Ctrl Pts',(2.64686653533936,-1.565171565732,109.123526862145));
#27782=CARTESIAN_POINT('Ctrl Pts',(2.59531160133992,-1.64643856306587,109.118536016963));
#27783=CARTESIAN_POINT('Ctrl Pts',(2.5436733532652,-1.72783688991971,109.11353710645));
#27784=CARTESIAN_POINT('Ctrl Pts',(2.48826550486169,-1.80670356733909,109.108538195937));
#27785=CARTESIAN_POINT('Ctrl Pts',(2.42938134619686,-1.88268651791815,109.103539285424));
#27786=CARTESIAN_POINT('Ctrl Pts',(2.39519559764185,-1.92679912989836,109.100637121213));
#27787=CARTESIAN_POINT('Ctrl Pts',(2.35983889563577,-1.96994042855624,109.097734957003));
#27788=CARTESIAN_POINT('Ctrl Pts',(2.32337427194717,-2.01204727639635,109.094832792792));
#27789=CARTESIAN_POINT('Ctrl Pts',(2.26055727778196,-2.08458403524721,109.089833283299));
#27790=CARTESIAN_POINT('Ctrl Pts',(2.19422975031862,-2.15430361913334,109.084833773806));
#27791=CARTESIAN_POINT('Ctrl Pts',(2.12467411518251,-2.22084717039994,109.079834264313));
#27792=CARTESIAN_POINT('Ctrl Pts',(2.05521283182369,-2.28730045576188,109.074841536623));
#27793=CARTESIAN_POINT('Ctrl Pts',(1.98253245805288,-2.35058597004816,109.069848808933));
#27794=CARTESIAN_POINT('Ctrl Pts',(1.90695503267566,-2.41037854980353,109.064856081243));
#27795=CARTESIAN_POINT('Ctrl Pts',(1.83145733957744,-2.4701080498942,109.059868620754));
#27796=CARTESIAN_POINT('Ctrl Pts',(1.75306901306894,-2.52635167002143,109.054881160266));
#27797=CARTESIAN_POINT('Ctrl Pts',(1.6721474736194,-2.57882242049899,109.049893699778));
#27798=CARTESIAN_POINT('Ctrl Pts',(1.59128383542269,-2.6312556269282,109.044909807934));
#27799=CARTESIAN_POINT('Ctrl Pts',(1.50789095485014,-2.67992109220403,109.039925916091));
#27800=CARTESIAN_POINT('Ctrl Pts',(1.42235693806705,-2.72457390994125,109.034942024247));
#27801=CARTESIAN_POINT('Ctrl Pts',(1.33685407065436,-2.7692104662282,109.029959947413));
#27802=CARTESIAN_POINT('Ctrl Pts',(1.24921200503772,-2.80983707549881,109.024977870579));
#27803=CARTESIAN_POINT('Ctrl Pts',(1.15984442191021,-2.84625423442175,109.019995793746));
#27804=CARTESIAN_POINT('Ctrl Pts',(1.07048498704748,-2.88266807293876,109.015014171163));
#27805=CARTESIAN_POINT('Ctrl Pts',(0.979400754045785,-2.9148730587022,109.01003254858));
#27806=CARTESIAN_POINT('Ctrl Pts',(0.887025407928533,-2.94271782128175,
109.005050925997));
#27807=CARTESIAN_POINT('Ctrl Pts',(0.794633266345759,-2.97056764652974,
109.000068397667));
#27808=CARTESIAN_POINT('Ctrl Pts',(0.700949965729004,-2.9940555475094,108.995085869337));
#27809=CARTESIAN_POINT('Ctrl Pts',(0.606423333443464,-3.01308031599812,
108.990103341007));
#27810=CARTESIAN_POINT('Ctrl Pts',(0.51179481537949,-3.03212559038343,108.985115442246));
#27811=CARTESIAN_POINT('Ctrl Pts',(0.416321581984284,-3.04669804160713,
108.980127543485));
#27812=CARTESIAN_POINT('Ctrl Pts',(0.320460391650988,-3.05674784491343,
108.975139644724));
#27813=CARTESIAN_POINT('Ctrl Pts',(0.224542574796665,-3.0668035847765,108.970148799543));
#27814=CARTESIAN_POINT('Ctrl Pts',(0.128236782722721,-3.07233133200704,
108.965157954361));
#27815=CARTESIAN_POINT('Ctrl Pts',(0.0320014880243871,-3.07333339466518,
108.96016710918));
#27816=CARTESIAN_POINT('Ctrl Pts',(-0.0643893253401735,-3.07433707668188,
108.955168198667));
#27817=CARTESIAN_POINT('Ctrl Pts',(-0.160708975473842,-3.07080048653805,
108.950169288154));
#27818=CARTESIAN_POINT('Ctrl Pts',(-0.256502460329738,-3.06277794458638,
108.945170377641));
#27819=CARTESIAN_POINT('Ctrl Pts',(-0.312116263111785,-3.05812038288913,
108.942268213429));
#27820=CARTESIAN_POINT('Ctrl Pts',(-0.36755286320686,-3.05195180141579,
108.939366049218));
#27821=CARTESIAN_POINT('Ctrl Pts',(-0.422724983626062,-3.0442906954196,
108.936463885007));
#27822=CARTESIAN_POINT('Ctrl Pts',(-0.517769067875486,-3.03109303692445,
108.931464375514));
#27823=CARTESIAN_POINT('Ctrl Pts',(-0.612361442832732,-3.01341695487468,
108.926464866021));
#27824=CARTESIAN_POINT('Ctrl Pts',(-0.706047334392842,-2.99130396509562,
108.921465356528));
#27825=CARTESIAN_POINT('Ctrl Pts',(-0.799606141635985,-2.96922097144676,
108.916472628838));
#27826=CARTESIAN_POINT('Ctrl Pts',(-0.89226048573956,-2.94271313168788,
108.911479901148));
#27827=CARTESIAN_POINT('Ctrl Pts',(-0.983562287575478,-2.91187353373379,
108.906487173458));
#27828=CARTESIAN_POINT('Ctrl Pts',(-1.07476776831182,-2.8810664707782,108.90149971297));
#27829=CARTESIAN_POINT('Ctrl Pts',(-1.16462312970035,-2.84593687403104,
108.896512252482));
#27830=CARTESIAN_POINT('Ctrl Pts',(-1.25269304887393,-2.80662829304184,
108.891524791993));
#27831=CARTESIAN_POINT('Ctrl Pts',(-1.34069995196168,-2.76734783826118,
108.88654090015));
#27832=CARTESIAN_POINT('Ctrl Pts',(-1.42692355279716,-2.72389452193577,
108.881557008306));
#27833=CARTESIAN_POINT('Ctrl Pts',(-1.51094712078631,-2.67646054485911,
108.876573116463));
#27834=CARTESIAN_POINT('Ctrl Pts',(-1.59494008947298,-2.62904384206214,
108.871591039629));
#27835=CARTESIAN_POINT('Ctrl Pts',(-1.67673423533987,-2.57764957440248,
108.866608962795));
#27836=CARTESIAN_POINT('Ctrl Pts',(-1.75593698743265,-2.52251611415387,
108.861626885961));
#27837=CARTESIAN_POINT('Ctrl Pts',(-1.83513251805927,-2.46738768080657,
108.856645263378));
#27838=CARTESIAN_POINT('Ctrl Pts',(-1.91173676450594,-2.40852098363493,
108.851663640795));
#27839=CARTESIAN_POINT('Ctrl Pts',(-1.98538663793553,-2.34619738042371,
108.846682018212));
#27840=CARTESIAN_POINT('Ctrl Pts',(-2.05904990220975,-2.28386244568333,
108.841699489883));
#27841=CARTESIAN_POINT('Ctrl Pts',(-2.12975739161074,-2.21806964022926,
108.836716961553));
#27842=CARTESIAN_POINT('Ctrl Pts',(-2.19718039315411,-2.14913949522575,
108.831734433223));
#27843=CARTESIAN_POINT('Ctrl Pts',(-2.26467606675646,-2.08013505368472,
108.826746534462));
#27844=CARTESIAN_POINT('Ctrl Pts',(-2.32887987737857,-2.00798683588808,
108.821758635701));
#27845=CARTESIAN_POINT('Ctrl Pts',(-2.38950134957952,-1.93305084008612,
108.81677073694));
#27846=CARTESIAN_POINT('Ctrl Pts',(-2.45015863171617,-1.85807057856289,
108.811779891758));
#27847=CARTESIAN_POINT('Ctrl Pts',(-2.50722910227927,-1.78029961376144,
108.806789046577));
#27848=CARTESIAN_POINT('Ctrl Pts',(-2.56046508113166,-1.70012376558457,
108.801798201396));
#27849=CARTESIAN_POINT('Ctrl Pts',(-2.61378709067025,-1.61981835121235,
108.796799290883));
#27850=CARTESIAN_POINT('Ctrl Pts',(-2.66326201001578,-1.53710066974384,
108.79180038037));
#27851=CARTESIAN_POINT('Ctrl Pts',(-2.70868767608633,-1.45238194818652,
108.786801469856));
#27852=CARTESIAN_POINT('Ctrl Pts',(-2.73505997100621,-1.40319770272766,
108.783899305645));
#27853=CARTESIAN_POINT('Ctrl Pts',(-2.76006835591568,-1.35333941643973,
108.780997141434));
#27854=CARTESIAN_POINT('Ctrl Pts',(-2.7836808263976,-1.30289036635719,108.778094977223));
#27855=CARTESIAN_POINT('Ctrl Pts',(-2.82776458090748,-1.20870354499948,
108.772676726104));
#27856=CARTESIAN_POINT('Ctrl Pts',(-2.8671157375435,-1.11216731993342,108.767258474984));
#27857=CARTESIAN_POINT('Ctrl Pts',(-2.90149899609407,-1.01375826786523,
108.761840223864));
#27858=CARTESIAN_POINT('Ctrl Pts',(-2.93575895679424,-0.915702109184439,
108.756441402512));
#27859=CARTESIAN_POINT('Ctrl Pts',(-2.96508642595566,-0.815786813333184,
108.75104258116));
#27860=CARTESIAN_POINT('Ctrl Pts',(-2.98929429006591,-0.714508150673832,
108.745643759808));
#27861=CARTESIAN_POINT('Ctrl Pts',(-3.0134461323165,-0.613463867181533,
108.740257432413));
#27862=CARTESIAN_POINT('Ctrl Pts',(-3.03250189335562,-0.511062811241492,
108.734871105017));
#27863=CARTESIAN_POINT('Ctrl Pts',(-3.04632357483707,-0.407817272061727,
108.729484777622));
#27864=CARTESIAN_POINT('Ctrl Pts',(-3.06009921045474,-0.30491568741747,
108.72411639436));
#27865=CARTESIAN_POINT('Ctrl Pts',(-3.06867547241194,-0.201175543042106,
108.718748011098));
#27866=CARTESIAN_POINT('Ctrl Pts',(-3.07196518096963,-0.0971193951289094,
108.713379627836));
#27867=CARTESIAN_POINT('Ctrl Pts',(-3.07297755216737,-0.0650972736407699,
108.711727567632));
#27868=CARTESIAN_POINT('Ctrl Pts',(-3.07348963021813,-0.0330453177270445,
108.710075507427));
#27869=CARTESIAN_POINT('Ctrl Pts',(-3.07349984408606,-0.000978980584313824,
108.708423447223));
#27870=CARTESIAN_POINT('Ctrl Pts',(-3.07349984408634,-0.000978979696610955,
108.708423447177));
#27871=CARTESIAN_POINT('Ctrl Pts',(-3.07353140800572,0.0981157223006356,
108.703318080358));
#27872=CARTESIAN_POINT('Ctrl Pts',(-3.0687661617826,0.19717128811251,108.69821271354));
#27873=CARTESIAN_POINT('Ctrl Pts',(-3.05924166423145,0.295707101420337,
108.693107346721));
#27874=CARTESIAN_POINT('Ctrl Pts',(-3.04971067839837,0.394310039333225,
108.687998502022));
#27875=CARTESIAN_POINT('Ctrl Pts',(-3.03541402516345,0.492392114361571,
108.682889657324));
#27876=CARTESIAN_POINT('Ctrl Pts',(-3.01644086918857,0.589480052833778,
108.677780812625));
#27877=CARTESIAN_POINT('Ctrl Pts',(-2.99743484423122,0.686736185872648,
108.672663117394));
#27878=CARTESIAN_POINT('Ctrl Pts',(-2.97373621135201,0.782994341219481,
108.667545422163));
#27879=CARTESIAN_POINT('Ctrl Pts',(-2.94548493282318,0.877793119426008,
108.662427726933));
#27880=CARTESIAN_POINT('Ctrl Pts',(-2.91720806099992,0.972677777393298,
108.657305395498));
#27881=CARTESIAN_POINT('Ctrl Pts',(-2.88437045851986,1.06610003899986,108.652183064064));
#27882=CARTESIAN_POINT('Ctrl Pts',(-2.84716073907503,1.15761737023496,108.647060732629));
#27883=CARTESIAN_POINT('Ctrl Pts',(-2.80987280649384,1.24932706673416,108.641927634287));
#27884=CARTESIAN_POINT('Ctrl Pts',(-2.76819456226925,1.33912346049446,108.636794535945));
#27885=CARTESIAN_POINT('Ctrl Pts',(-2.7223614801067,1.42658691345156,108.631661437603));
#27886=CARTESIAN_POINT('Ctrl Pts',(-2.68683811953932,1.4943762836895,108.627682981549));
#27887=CARTESIAN_POINT('Ctrl Pts',(-2.64881983239274,1.56076469042194,108.623704525494));
#27888=CARTESIAN_POINT('Ctrl Pts',(-2.60843375910547,1.62556930776849,108.619726069439));
#27889=CARTESIAN_POINT('Ctrl Pts',(-2.55768277580638,1.70700574822815,108.614726559946));
#27890=CARTESIAN_POINT('Ctrl Pts',(-2.50302527490195,1.78620624615312,108.609727050453));
#27891=CARTESIAN_POINT('Ctrl Pts',(-2.44468433443415,1.86277233041837,108.604727540961));
#27892=CARTESIAN_POINT('Ctrl Pts',(-2.38642253308163,1.9392345532765,108.59973481327));
#27893=CARTESIAN_POINT('Ctrl Pts',(-2.32448748627122,2.01306911853243,108.59474208558));
#27894=CARTESIAN_POINT('Ctrl Pts',(-2.25914665028472,2.08390466732702,108.58974935789));
#27895=CARTESIAN_POINT('Ctrl Pts',(-2.19387474723318,2.15466548640313,108.584761897402));
#27896=CARTESIAN_POINT('Ctrl Pts',(-2.1252044937598,2.22243325769432,108.579774436914));
#27897=CARTESIAN_POINT('Ctrl Pts',(-2.05344424231571,2.28686881864711,108.574786976426));
#27898=CARTESIAN_POINT('Ctrl Pts',(-1.98173533700892,2.35125827444988,108.569803084582));
#27899=CARTESIAN_POINT('Ctrl Pts',(-1.90694115470479,2.41231996730369,108.564819192738));
#27900=CARTESIAN_POINT('Ctrl Pts',(-1.82940691437592,2.46975152426992,108.559835300895));
#27901=CARTESIAN_POINT('Ctrl Pts',(-1.75190091009697,2.52716216608558,108.554853224061));
#27902=CARTESIAN_POINT('Ctrl Pts',(-1.67165718280875,2.58094503768329,108.549871147227));
#27903=CARTESIAN_POINT('Ctrl Pts',(-1.58905328635393,2.63083863114555,108.544889070393));
#27904=CARTESIAN_POINT('Ctrl Pts',(-1.50645692147157,2.68072767546145,108.53990744781));
#27905=CARTESIAN_POINT('Ctrl Pts',(-1.42150119110167,2.72672791988308,108.534925825227));
#27906=CARTESIAN_POINT('Ctrl Pts',(-1.3345909069889,2.76862228571948,108.529944202644));
#27907=CARTESIAN_POINT('Ctrl Pts',(-1.24766482105507,2.81052426868978,108.524961674314));
#27908=CARTESIAN_POINT('Ctrl Pts',(-1.15878387103893,2.84831869990831,108.519979145985));
#27909=CARTESIAN_POINT('Ctrl Pts',(-1.06837465226522,2.88183584758001,108.514996617655));
#27910=CARTESIAN_POINT('Ctrl Pts',(-0.977867985678008,2.9153891217972,108.510008718894));
#27911=CARTESIAN_POINT('Ctrl Pts',(-0.885830174024775,2.94465575562677,
108.505020820133));
#27912=CARTESIAN_POINT('Ctrl Pts',(-0.792704638749025,2.96951538229823,
108.500032921372));
#27913=CARTESIAN_POINT('Ctrl Pts',(-0.699524092941319,2.99438969389238,
108.49504207619));
#27914=CARTESIAN_POINT('Ctrl Pts',(-0.605254972895097,3.01485172170391,
108.490051231009));
#27915=CARTESIAN_POINT('Ctrl Pts',(-0.510350514170142,3.03083232836894,
108.485060385828));
#27916=CARTESIAN_POINT('Ctrl Pts',(-0.415292687443233,3.0468387600979,108.480061475314));
#27917=CARTESIAN_POINT('Ctrl Pts',(-0.319597907425214,3.05834925744096,
108.475062564801));
#27918=CARTESIAN_POINT('Ctrl Pts',(-0.223724083557654,3.06534660102839,
108.470063654288));
#27919=CARTESIAN_POINT('Ctrl Pts',(-0.1680636392132,3.06940897423512,108.467161490077));
#27920=CARTESIAN_POINT('Ctrl Pts',(-0.112342859687147,3.07195116941884,
108.464259325866));
#27921=CARTESIAN_POINT('Ctrl Pts',(-0.0566508376245821,3.07297786073971,
108.461357161655));
#27922=CARTESIAN_POINT('Ctrl Pts',(0.0392697134137614,3.07474617141685,
108.456358650558));
#27923=CARTESIAN_POINT('Ctrl Pts',(0.135441582109926,3.0720221593444,108.45136013946));
#27924=CARTESIAN_POINT('Ctrl Pts',(0.231409352307455,3.06477600513719,108.446361628363));
#27925=CARTESIAN_POINT('Ctrl Pts',(0.327255795233389,3.05753901188179,108.441369436634));
#27926=CARTESIAN_POINT('Ctrl Pts',(0.422898218666516,3.04579126670438,108.436377244905));
#27927=CARTESIAN_POINT('Ctrl Pts',(0.51787965982746,3.02955490261144,108.431385053176));
#27928=CARTESIAN_POINT('Ctrl Pts',(0.612766961614202,3.01333463093757,108.42639780938));
#27929=CARTESIAN_POINT('Ctrl Pts',(0.70699415276511,2.99263465446948,108.421410565584));
#27930=CARTESIAN_POINT('Ctrl Pts',(0.800108920153355,2.96752893261229,108.416423321788));
#27931=CARTESIAN_POINT('Ctrl Pts',(0.896853710889718,2.94144447924914,108.411241653284));
#27932=CARTESIAN_POINT('Ctrl Pts',(0.992397085932376,2.91060379138493,108.406059984781));
#27933=CARTESIAN_POINT('Ctrl Pts',(1.08624307984464,2.87514838251691,108.400878316277));
#27934=CARTESIAN_POINT('Ctrl Pts',(1.17647157100917,2.84105968131169,108.395896386721));
#27935=CARTESIAN_POINT('Ctrl Pts',(1.26513068520286,2.80270564861303,108.390914457165));
#27936=CARTESIAN_POINT('Ctrl Pts',(1.35179631350352,2.76026248331536,108.385932527609));
#27937=CARTESIAN_POINT('Ctrl Pts',(1.43844753217521,2.71782637491299,108.380951426383));
#27938=CARTESIAN_POINT('Ctrl Pts',(1.52310553228236,2.67130268361139,108.375970325157));
#27939=CARTESIAN_POINT('Ctrl Pts',(1.60536895169007,2.62091449287258,108.370989223932));
#27940=CARTESIAN_POINT('Ctrl Pts',(1.68765633080886,2.57051162627296,108.36600667193));
#27941=CARTESIAN_POINT('Ctrl Pts',(1.76754736597993,2.51624224784611,108.361024119929));
#27942=CARTESIAN_POINT('Ctrl Pts',(1.84466863322337,2.4583734223266,108.356041567928));
#27943=CARTESIAN_POINT('Ctrl Pts',(1.85394665788643,2.45141155033483,108.3554421452));
#27944=CARTESIAN_POINT('Ctrl Pts',(1.86318463274705,2.4443976324336,108.354842722473));
#27945=CARTESIAN_POINT('Ctrl Pts',(1.8723819390353,2.43733217358127,108.354243299745));
#27946=CARTESIAN_POINT('',(-3.07349942256353,0.00188401212038324,108.791576552858));
#27947=CARTESIAN_POINT('Ctrl Pts',(-3.07349942256311,0.00188401280239466,
108.791576552823));
#27948=CARTESIAN_POINT('Ctrl Pts',(-3.07342968576284,0.115649702238102,
108.785659716256));
#27949=CARTESIAN_POINT('Ctrl Pts',(-3.06704369053512,0.229219670324852,
108.779742879689));
#27950=CARTESIAN_POINT('Ctrl Pts',(-3.05440435245984,0.342076455890201,
108.773826043122));
#27951=CARTESIAN_POINT('Ctrl Pts',(-3.04372457620121,0.437436292926549,
108.768826533629));
#27952=CARTESIAN_POINT('Ctrl Pts',(-3.02855599778406,0.532463002358434,
108.763827024136));
#27953=CARTESIAN_POINT('Ctrl Pts',(-3.00892809284563,0.626700871296976,
108.758827514643));
#27954=CARTESIAN_POINT('Ctrl Pts',(-2.98932681303559,0.720810907164757,
108.753834786953));
#27955=CARTESIAN_POINT('Ctrl Pts',(-2.96527831752782,0.814133803142816,
108.748842059263));
#27956=CARTESIAN_POINT('Ctrl Pts',(-2.93686381305166,0.906219175248276,
108.743849331573));
#27957=CARTESIAN_POINT('Ctrl Pts',(-2.90847928516147,0.998207399607386,
108.738861871085));
#27958=CARTESIAN_POINT('Ctrl Pts',(-2.87573803355059,1.08896027824398,108.733874410597));
#27959=CARTESIAN_POINT('Ctrl Pts',(-2.83877204625355,1.17803884460972,108.728886950109));
#27960=CARTESIAN_POINT('Ctrl Pts',(-2.80183250898455,1.26705367317891,108.723903058265));
#27961=CARTESIAN_POINT('Ctrl Pts',(-2.76067441317311,1.35439616678808,108.718919166421));
#27962=CARTESIAN_POINT('Ctrl Pts',(-2.715478872724,1.43964465816727,108.713935274578));
#27963=CARTESIAN_POINT('Ctrl Pts',(-2.67029979137136,1.5248621041573,108.708953197744));
#27964=CARTESIAN_POINT('Ctrl Pts',(-2.62108639218397,1.60798667565565,108.70397112091));
#27965=CARTESIAN_POINT('Ctrl Pts',(-2.56806658325906,1.68861963566344,108.698989044076));
#27966=CARTESIAN_POINT('Ctrl Pts',(-2.51505160851921,1.76924524380298,108.694007421493));
#27967=CARTESIAN_POINT('Ctrl Pts',(-2.45823115537972,1.84737932544832,108.68902579891));
#27968=CARTESIAN_POINT('Ctrl Pts',(-2.39787688201833,1.92265147873504,108.684044176327));
#27969=CARTESIAN_POINT('Ctrl Pts',(-2.33751163518674,1.99793731782536,108.679061647997));
#27970=CARTESIAN_POINT('Ctrl Pts',(-2.27361156672695,2.07035985270018,108.674079119668));
#27971=CARTESIAN_POINT('Ctrl Pts',(-2.20648840350465,2.13958200945874,108.669096591338));
#27972=CARTESIAN_POINT('Ctrl Pts',(-2.1392928914048,2.20887877750054,108.664108692577));
#27973=CARTESIAN_POINT('Ctrl Pts',(-2.06886765506542,2.27496796508934,108.659120793816));
#27974=CARTESIAN_POINT('Ctrl Pts',(-1.99556088715803,2.33754978463455,108.654132895055));
#27975=CARTESIAN_POINT('Ctrl Pts',(-1.92221081593672,2.4001685721195,108.649142049873));
#27976=CARTESIAN_POINT('Ctrl Pts',(-1.84597617061308,2.45927559732614,108.644151204692));
#27977=CARTESIAN_POINT('Ctrl Pts',(-1.76723608672674,2.51461306442378,108.639160359511));
#27978=CARTESIAN_POINT('Ctrl Pts',(-1.68836875687637,2.57003995826571,108.634161448998));
#27979=CARTESIAN_POINT('Ctrl Pts',(-1.60698827418052,2.62168489517077,108.629162538484));
#27980=CARTESIAN_POINT('Ctrl Pts',(-1.52350037601449,2.66933490860246,108.624163627971));
#27981=CARTESIAN_POINT('Ctrl Pts',(-1.47503069657559,2.69699856916918,108.62126146376));
#27982=CARTESIAN_POINT('Ctrl Pts',(-1.42585114589775,2.7233166204389,108.618359299549));
#27983=CARTESIAN_POINT('Ctrl Pts',(-1.37604412559659,2.74825486707676,108.615457135338));
#27984=CARTESIAN_POINT('Ctrl Pts',(-1.29024240911845,2.79121556527847,108.610457625845));
#27985=CARTESIAN_POINT('Ctrl Pts',(-1.20227618216251,2.8302297190156,108.605458116352));
#27986=CARTESIAN_POINT('Ctrl Pts',(-1.11254374124092,2.86507393863154,108.600458606859));
#27987=CARTESIAN_POINT('Ctrl Pts',(-1.02293302180566,2.89987089228483,108.595465879169));
#27988=CARTESIAN_POINT('Ctrl Pts',(-0.931561255708334,2.93050899617858,
108.590473151479));
#27989=CARTESIAN_POINT('Ctrl Pts',(-0.838850434689728,2.95681115362832,
108.585480423789));
#27990=CARTESIAN_POINT('Ctrl Pts',(-0.746237421250267,2.98308556296498,
108.580492963301));
#27991=CARTESIAN_POINT('Ctrl Pts',(-0.652288581241642,3.00503300014899,
108.575505502812));
#27992=CARTESIAN_POINT('Ctrl Pts',(-0.557443977509493,3.02252517970296,
108.570518042324));
#27993=CARTESIAN_POINT('Ctrl Pts',(-0.462667237308462,3.04000484319355,
108.56553415048));
#27994=CARTESIAN_POINT('Ctrl Pts',(-0.366996437986369,3.05303550694457,
108.560550258637));
#27995=CARTESIAN_POINT('Ctrl Pts',(-0.270883878544352,3.06153951049872,
108.555566366793));
#27996=CARTESIAN_POINT('Ctrl Pts',(-0.174806320916051,3.07004041710541,
108.550584289959));
#27997=CARTESIAN_POINT('Ctrl Pts',(-0.0782877596223771,3.07401790025227,
108.545602213126));
#27998=CARTESIAN_POINT('Ctrl Pts',(0.0182132628988892,3.07344603451152,
108.540620136292));
#27999=CARTESIAN_POINT('Ctrl Pts',(0.114705486750156,3.07287422091175,108.535638513709));
#28000=CARTESIAN_POINT('Ctrl Pts',(0.211179736054938,3.06775388589978,108.530656891126));
#28001=CARTESIAN_POINT('Ctrl Pts',(0.307177415868004,3.05811122838602,108.525675268543));
#28002=CARTESIAN_POINT('Ctrl Pts',(0.403192549750659,3.04846681766723,108.520692740213));
#28003=CARTESIAN_POINT('Ctrl Pts',(0.498730505300663,3.03429849538734,108.515710211883));
#28004=CARTESIAN_POINT('Ctrl Pts',(0.593338827351907,3.01568421522491,108.510727683553));
#28005=CARTESIAN_POINT('Ctrl Pts',(0.688049123231148,2.99704987161179,108.505739784792));
#28006=CARTESIAN_POINT('Ctrl Pts',(0.781827353776249,2.97396008803848,108.500751886031));
#28007=CARTESIAN_POINT('Ctrl Pts',(0.874232485425454,2.94654370600995,108.49576398727));
#28008=CARTESIAN_POINT('Ctrl Pts',(0.966692202054234,2.91911112874824,108.490773142089));
#28009=CARTESIAN_POINT('Ctrl Pts',(1.05777679044951,2.88734700852904,108.485782296908));
#28010=CARTESIAN_POINT('Ctrl Pts',(1.14706359252094,2.85142900397554,108.480791451726));
#28011=CARTESIAN_POINT('Ctrl Pts',(1.2364946843193,2.81545295501964,108.475792541213));
#28012=CARTESIAN_POINT('Ctrl Pts',(1.32412178980594,2.77530980048739,108.4707936307));
#28013=CARTESIAN_POINT('Ctrl Pts',(1.40954536994573,2.73122391979577,108.465794720187));
#28014=CARTESIAN_POINT('Ctrl Pts',(1.45913882764104,2.70562944979741,108.462892555976));
#28015=CARTESIAN_POINT('Ctrl Pts',(1.50799008914338,2.67870692619813,108.459990391765));
#28016=CARTESIAN_POINT('Ctrl Pts',(1.55602560798143,2.65050684913396,108.457088227554));
#28017=CARTESIAN_POINT('Ctrl Pts',(1.63877545032361,2.60192713171767,108.45208872642));
#28018=CARTESIAN_POINT('Ctrl Pts',(1.71939343985904,2.54938315058608,108.447089225286));
#28019=CARTESIAN_POINT('Ctrl Pts',(1.7974753479185,2.49308736782835,108.442089724152));
#28020=CARTESIAN_POINT('Ctrl Pts',(1.82271337604429,2.47489116099998,108.44047376018));
#28021=CARTESIAN_POINT('Ctrl Pts',(1.84768661711419,2.45630335660053,108.438857796209));
#28022=CARTESIAN_POINT('Ctrl Pts',(1.87238193903529,2.43733217358128,108.437241832237));
#28023=CARTESIAN_POINT('Ctrl Pts',(1.87238193903529,2.43733217358128,109.437414079767));
#28024=CARTESIAN_POINT('Ctrl Pts',(1.94920407382002,2.37831667325343,109.432395345516));
#28025=CARTESIAN_POINT('Ctrl Pts',(2.02314962296453,2.31573001139801,109.427376611265));
#28026=CARTESIAN_POINT('Ctrl Pts',(2.09388683944776,2.24989780958769,109.422357877013));
#28027=CARTESIAN_POINT('Ctrl Pts',(2.16462405593099,2.18406560777736,109.417339142762));
#28028=CARTESIAN_POINT('Ctrl Pts',(2.2321526722981,2.11498822739159,109.41232040851));
#28029=CARTESIAN_POINT('Ctrl Pts',(2.29618206789388,2.04302475782419,109.407301674259));
#28030=CARTESIAN_POINT('Ctrl Pts',(2.35996619255337,1.97133695144861,109.402302164766));
#28031=CARTESIAN_POINT('Ctrl Pts',(2.42050194475992,1.89653331529101,109.397302655273));
#28032=CARTESIAN_POINT('Ctrl Pts',(2.47747009479805,1.81894040017295,109.392303145779));
#28033=CARTESIAN_POINT('Ctrl Pts',(2.53436096790243,1.7414527393515,109.387310418089));
#28034=CARTESIAN_POINT('Ctrl Pts',(2.58769359932268,1.6611836701117,109.382317690399));
#28035=CARTESIAN_POINT('Ctrl Pts',(2.63718730315004,1.57849465570975,109.377324962708));
#28036=CARTESIAN_POINT('Ctrl Pts',(2.68662879236747,1.49589287613361,109.37233750222));
#28037=CARTESIAN_POINT('Ctrl Pts',(2.73223918084695,1.41087660121226,109.367350041732));
#28038=CARTESIAN_POINT('Ctrl Pts',(2.77378021988544,1.32383743026562,109.362362581243));
#28039=CARTESIAN_POINT('Ctrl Pts',(2.81529153533949,1.2368605378803,109.357378689399));
#28040=CARTESIAN_POINT('Ctrl Pts',(2.85273910117318,1.14786402191088,109.352394797555));
#28041=CARTESIAN_POINT('Ctrl Pts',(2.88593037386635,1.05726445471115,109.347410905711));
#28042=CARTESIAN_POINT('Ctrl Pts',(2.91910955912007,0.966697881629828,109.342428828877));
#28043=CARTESIAN_POINT('Ctrl Pts',(2.94803538014164,0.874529829000709,109.337446752044));
#28044=CARTESIAN_POINT('Ctrl Pts',(2.97256362795683,0.781196343916247,109.33246467521));
#28045=CARTESIAN_POINT('Ctrl Pts',(2.99708963936092,0.687871368695325,109.327483052626));
#28046=CARTESIAN_POINT('Ctrl Pts',(3.01721876334168,0.593381596877724,109.322501430043));
#28047=CARTESIAN_POINT('Ctrl Pts',(3.03285711041393,0.498176673291401,109.31751980746));
#28048=CARTESIAN_POINT('Ctrl Pts',(3.04849830081322,0.402954439772503,109.31253727913));
#28049=CARTESIAN_POINT('Ctrl Pts',(3.05964702161439,0.307017229409604,109.3075547508));
#28050=CARTESIAN_POINT('Ctrl Pts',(3.06626095531663,0.210822209220869,109.30257222247));
#28051=CARTESIAN_POINT('Ctrl Pts',(3.07288201786465,0.114523504977408,109.297584323708));
#28052=CARTESIAN_POINT('Ctrl Pts',(3.07495850504839,0.0179668747989478,
109.292596424947));
#28053=CARTESIAN_POINT('Ctrl Pts',(3.07250020693919,-0.0783883177433252,
109.287608526186));
#28054=CARTESIAN_POINT('Ctrl Pts',(3.07004045667956,-0.174800428620378,
109.282617681004));
#28055=CARTESIAN_POINT('Ctrl Pts',(3.06304061911616,-0.271010427328123,
109.277626835823));
#28056=CARTESIAN_POINT('Ctrl Pts',(3.05156239964119,-0.366564006820237,
109.272635990641));
#28057=CARTESIAN_POINT('Ctrl Pts',(3.04006563107369,-0.462272003309829,
109.267637080128));
#28058=CARTESIAN_POINT('Ctrl Pts',(3.02407610232081,-0.557321029832261,
109.262638169614));
#28059=CARTESIAN_POINT('Ctrl Pts',(3.00370664265917,-0.651266961272567,
109.257639259101));
#28060=CARTESIAN_POINT('Ctrl Pts',(2.99188096251942,-0.705808149605373,
109.254737094892));
#28061=CARTESIAN_POINT('Ctrl Pts',(2.97857997045296,-0.759977805615262,
109.251834930684));
#28062=CARTESIAN_POINT('Ctrl Pts',(2.96383331659665,-0.813691785279715,
109.248932766475));
#28063=CARTESIAN_POINT('Ctrl Pts',(2.93842950390934,-0.906223955043927,
109.243933256982));
#28064=CARTESIAN_POINT('Ctrl Pts',(2.9086435757866,-0.997727833444311,109.238933747489));
#28065=CARTESIAN_POINT('Ctrl Pts',(2.87457563542129,-1.08775786195378,109.233934237996));
#28066=CARTESIAN_POINT('Ctrl Pts',(2.84055390800077,-1.17766576530123,109.228941510306));
#28067=CARTESIAN_POINT('Ctrl Pts',(2.80226186641799,-1.26610338513085,109.223948782616));
#28068=CARTESIAN_POINT('Ctrl Pts',(2.75984988338236,-1.35263848503375,109.218956054926));
#28069=CARTESIAN_POINT('Ctrl Pts',(2.71748264391977,-1.43908229258749,109.213968594438));
#28070=CARTESIAN_POINT('Ctrl Pts',(2.67100429561214,-1.52362717815871,109.20898113395));
#28071=CARTESIAN_POINT('Ctrl Pts',(2.62061359406956,-1.60586009371234,109.203993673462));
#28072=CARTESIAN_POINT('Ctrl Pts',(2.57025894825183,-1.68803416969268,109.199009781618));
#28073=CARTESIAN_POINT('Ctrl Pts',(2.51599774292866,-1.76789919105604,109.194025889775));
#28074=CARTESIAN_POINT('Ctrl Pts',(2.45807456515645,-1.84506685031489,109.189041997931));
#28075=CARTESIAN_POINT('Ctrl Pts',(2.40017248157099,-1.92220640702348,109.184059921097));
#28076=CARTESIAN_POINT('Ctrl Pts',(2.33861133850038,-1.99665020266829,109.179077844264));
#28077=CARTESIAN_POINT('Ctrl Pts',(2.27367837408059,-2.06803986935413,109.17409576743));
#28078=CARTESIAN_POINT('Ctrl Pts',(2.20875133005119,-2.13942302694709,109.169114144847));
#28079=CARTESIAN_POINT('Ctrl Pts',(2.14045337140159,-2.20775228461636,109.164132522264));
#28080=CARTESIAN_POINT('Ctrl Pts',(2.06911053846775,-2.27270407875766,109.159150899681));
#28081=CARTESIAN_POINT('Ctrl Pts',(1.99775473414986,-2.33766768227955,109.154168371351));
#28082=CARTESIAN_POINT('Ctrl Pts',(1.92335328068573,-2.39925230722043,109.149185843022));
#28083=CARTESIAN_POINT('Ctrl Pts',(1.84626660641381,-2.45717355269042,109.144203314692));
#28084=CARTESIAN_POINT('Ctrl Pts',(1.76909684406792,-2.51515722872669,109.139215415931));
#28085=CARTESIAN_POINT('Ctrl Pts',(1.68923643428642,-2.56946937818642,109.13422751717));
#28086=CARTESIAN_POINT('Ctrl Pts',(1.6070760179085,-2.61986811169253,109.129239618409));
#28087=CARTESIAN_POINT('Ctrl Pts',(1.5248670682449,-2.67029661642228,109.124248773228));
#28088=CARTESIAN_POINT('Ctrl Pts',(1.44035579108999,-2.71680689066201,109.119257928046));
#28089=CARTESIAN_POINT('Ctrl Pts',(1.35395685128638,-2.75920334423809,109.114267082865));
#28090=CARTESIAN_POINT('Ctrl Pts',(1.26741828861416,-2.80166831155383,109.109268172352));
#28091=CARTESIAN_POINT('Ctrl Pts',(1.17898637457032,-2.84000600906012,109.104269261839));
#28092=CARTESIAN_POINT('Ctrl Pts',(1.0890950679507,-2.87406927247161,109.099270351326));
#28093=CARTESIAN_POINT('Ctrl Pts',(1.03690782988644,-2.89384501835573,109.096368187114));
#28094=CARTESIAN_POINT('Ctrl Pts',(0.984228994385734,-2.91218100262128,
109.093466022903));
#28095=CARTESIAN_POINT('Ctrl Pts',(0.931145283869106,-2.92905628322986,
109.090563858691));
#28096=CARTESIAN_POINT('Ctrl Pts',(0.839698868264912,-2.95812704540814,
109.085564349198));
#28097=CARTESIAN_POINT('Ctrl Pts',(0.74672912593414,-2.9829622681281,109.080564839705));
#28098=CARTESIAN_POINT('Ctrl Pts',(0.652664289271526,-3.00340333214001,
109.075565330212));
#28099=CARTESIAN_POINT('Ctrl Pts',(0.558727050962504,-3.02381666797839,
109.070572602522));
#28100=CARTESIAN_POINT('Ctrl Pts',(0.463698095913494,-3.03984759908562,
109.065579874832));
#28101=CARTESIAN_POINT('Ctrl Pts',(0.368021851346044,-3.0513869251427,109.060587147142));
#28102=CARTESIAN_POINT('Ctrl Pts',(0.272446542804956,-3.06291407750166,
109.055599686653));
#28103=CARTESIAN_POINT('Ctrl Pts',(0.176225735744696,-3.0699589924401,109.050612226165));
#28104=CARTESIAN_POINT('Ctrl Pts',(0.0798141044726736,-3.07246349998291,
109.045624765677));
#28105=CARTESIAN_POINT('Ctrl Pts',(-0.0165285420234597,-3.07496621549203,
109.040640873833));
#28106=CARTESIAN_POINT('Ctrl Pts',(-0.113061303741829,-3.07293497063558,
109.03565698199));
#28107=CARTESIAN_POINT('Ctrl Pts',(-0.209325305552926,-3.06636350853175,
109.030673090146));
#28108=CARTESIAN_POINT('Ctrl Pts',(-0.305554250398746,-3.05979443959168,
109.025691013312));
#28109=CARTESIAN_POINT('Ctrl Pts',(-0.401514192310171,-3.04868846846501,
109.020708936479));
#28110=CARTESIAN_POINT('Ctrl Pts',(-0.496748147809946,-3.03309141432424,
109.015726859645));
#28111=CARTESIAN_POINT('Ctrl Pts',(-0.591973420167034,-3.01749578227547,
109.010745237062));
#28112=CARTESIAN_POINT('Ctrl Pts',(-0.686472404555486,-2.99740995246849,
109.005763614479));
#28113=CARTESIAN_POINT('Ctrl Pts',(-0.77979618515038,-2.97293124031231,
109.000781991896));
#28114=CARTESIAN_POINT('Ctrl Pts',(-0.873136933652916,-2.94844807749496,
108.995799463566));
#28115=CARTESIAN_POINT('Ctrl Pts',(-0.965301629421924,-2.91957055750715,
108.990816935236));
#28116=CARTESIAN_POINT('Ctrl Pts',(-1.05585548341354,-2.88644616235009,
108.985834406906));
#28117=CARTESIAN_POINT('Ctrl Pts',(-1.14650694111404,-2.85328606397688,
108.980846508145));
#28118=CARTESIAN_POINT('Ctrl Pts',(-1.23554367784378,-2.81587010291647,
108.975858609384));
#28119=CARTESIAN_POINT('Ctrl Pts',(-1.32255011364468,-2.77439424864211,
108.970870710623));
#28120=CARTESIAN_POINT('Ctrl Pts',(-1.40960794534142,-2.73289389401136,
108.965879865442));
#28121=CARTESIAN_POINT('Ctrl Pts',(-1.49463270132819,-2.68732907813605,
108.960889020261));
#28122=CARTESIAN_POINT('Ctrl Pts',(-1.57723455715542,-2.63794112931178,
108.955898175079));
#28123=CARTESIAN_POINT('Ctrl Pts',(-1.65996989966767,-2.58847336831499,
108.950899264566));
#28124=CARTESIAN_POINT('Ctrl Pts',(-1.7402741582147,-2.53517038030392,108.945900354053));
#28125=CARTESIAN_POINT('Ctrl Pts',(-1.8177876229855,-2.47831604274369,108.94090144354));
#28126=CARTESIAN_POINT('Ctrl Pts',(-1.86278878929052,-2.44530872579205,
108.937999279329));
#28127=CARTESIAN_POINT('Ctrl Pts',(-1.90684994564932,-2.41110518024289,
108.935097115118));
#28128=CARTESIAN_POINT('Ctrl Pts',(-1.94990630988446,-2.37576674626798,
108.932194950906));
#28129=CARTESIAN_POINT('Ctrl Pts',(-2.0231004133922,-2.31569281666177,108.927261387392));
#28130=CARTESIAN_POINT('Ctrl Pts',(-2.09366081744235,-2.25211385752092,
108.922327823877));
#28131=CARTESIAN_POINT('Ctrl Pts',(-2.16122630733891,-2.18529245147331,
108.917394260362));
#28132=CARTESIAN_POINT('Ctrl Pts',(-2.22869969055363,-2.11856213775694,
108.912467422383));
#28133=CARTESIAN_POINT('Ctrl Pts',(-2.29318595057505,-2.04859847115879,
108.907540584405));
#28134=CARTESIAN_POINT('Ctrl Pts',(-2.35435603555813,-1.97570491415875,
108.902613746427));
#28135=CARTESIAN_POINT('Ctrl Pts',(-2.41545719841484,-1.90289348846435,
108.897692459661));
#28136=CARTESIAN_POINT('Ctrl Pts',(-2.47324932477289,-1.82715907853984,
108.892771172895));
#28137=CARTESIAN_POINT('Ctrl Pts',(-2.52744035696434,-1.74884175727478,
108.887849886129));
#28138=CARTESIAN_POINT('Ctrl Pts',(-2.58159824008911,-1.67057234331099,
108.882931609752));
#28139=CARTESIAN_POINT('Ctrl Pts',(-2.63215914615633,-1.58972352521532,
108.878013333375));
#28140=CARTESIAN_POINT('Ctrl Pts',(-2.6788720486264,-1.50666744741107,108.873095056998));
#28141=CARTESIAN_POINT('Ctrl Pts',(-2.72556993900543,-1.42363806127736,
108.868178361204));
#28142=CARTESIAN_POINT('Ctrl Pts',(-2.76842206102694,-1.33840321788697,
108.863261665409));
#28143=CARTESIAN_POINT('Ctrl Pts',(-2.807222054207,-1.25136189344803,108.858344969615));
#28144=CARTESIAN_POINT('Ctrl Pts',(-2.8460208426018,-1.1643232717442,108.85342842649));
#28145=CARTESIAN_POINT('Ctrl Pts',(-2.88076757017542,-1.07547869384789,
108.848511883365));
#28146=CARTESIAN_POINT('Ctrl Pts',(-2.91130349058054,-0.985248311713113,
108.84359534024));
#28147=CARTESIAN_POINT('Ctrl Pts',(-2.94186355431931,-0.894946588607045,
108.838674909832));
#28148=CARTESIAN_POINT('Ctrl Pts',(-2.96820601882626,-0.803257302207185,
108.833754479425));
#28149=CARTESIAN_POINT('Ctrl Pts',(-2.99022180531312,-0.710616496452175,
108.828834049017));
#28150=CARTESIAN_POINT('Ctrl Pts',(-3.01224721691765,-0.617935188911903,
108.823911467439));
#28151=CARTESIAN_POINT('Ctrl Pts',(-3.02994210090026,-0.52430197769036,
108.818988885861));
#28152=CARTESIAN_POINT('Ctrl Pts',(-3.04324877593042,-0.430161757712154,
108.814066304282));
#28153=CARTESIAN_POINT('Ctrl Pts',(-3.05657391129479,-0.33589093712039,
108.809136893612));
#28154=CARTESIAN_POINT('Ctrl Pts',(-3.06549864354241,-0.241112153077702,
108.804207482942));
#28155=CARTESIAN_POINT('Ctrl Pts',(-3.07001730613623,-0.146273681925572,
108.799278072273));
#28156=CARTESIAN_POINT('Ctrl Pts',(-3.07237056700401,-0.0968830362889882,
108.796710899135));
#28157=CARTESIAN_POINT('Ctrl Pts',(-3.07352967967365,-0.0474761854540675,
108.794143725996));
#28158=CARTESIAN_POINT('Ctrl Pts',(-3.07349942256353,0.00188401212038081,
108.791576552858));
#28159=CARTESIAN_POINT('Origin',(0.,0.,116.208423447177));
#28160=CARTESIAN_POINT('',(1.8723819390353,2.43733217358127,110.437319612009));
#28161=CARTESIAN_POINT('',(1.8723819390353,2.43733217358127,110.35412809305));
#28162=CARTESIAN_POINT('',(1.8723819390353,2.43733217358128,116.208423447177));
#28163=CARTESIAN_POINT('',(-3.07349931288414,-0.0020551643988658,109.708423447143));
#28164=CARTESIAN_POINT('Ctrl Pts',(1.8723819390353,2.43733217358127,110.35412809305));
#28165=CARTESIAN_POINT('Ctrl Pts',(1.94855031136323,2.37881889983944,110.349132233708));
#28166=CARTESIAN_POINT('Ctrl Pts',(2.02209372129131,2.31663912935644,110.344136374365));
#28167=CARTESIAN_POINT('Ctrl Pts',(2.09263962734076,2.2510578935432,110.339140515023));
#28168=CARTESIAN_POINT('Ctrl Pts',(2.1631006932861,2.18555552720921,110.334150663814));
#28169=CARTESIAN_POINT('Ctrl Pts',(2.23057110136168,2.11666012335588,110.329160812605));
#28170=CARTESIAN_POINT('Ctrl Pts',(2.29471016091284,2.04467785418715,110.324170961396));
#28171=CARTESIAN_POINT('Ctrl Pts',(2.35938447039662,1.97209488234221,110.319139469141));
#28172=CARTESIAN_POINT('Ctrl Pts',(2.42067120798129,1.8963735556705,110.314107976887));
#28173=CARTESIAN_POINT('Ctrl Pts',(2.47825785808659,1.81786694750526,110.309076484632));
#28174=CARTESIAN_POINT('Ctrl Pts',(2.53528697316547,1.74012041452718,110.304093705632));
#28175=CARTESIAN_POINT('Ctrl Pts',(2.58868707596905,1.65964266323822,110.299110926632));
#28176=CARTESIAN_POINT('Ctrl Pts',(2.63819497902644,1.57680991328685,110.294128147632));
#28177=CARTESIAN_POINT('Ctrl Pts',(2.68769187402954,1.49399558115065,110.28914647655));
#28178=CARTESIAN_POINT('Ctrl Pts',(2.73329806407065,1.40882766764537,110.284164805469));
#28179=CARTESIAN_POINT('Ctrl Pts',(2.77479458668175,1.32170997261943,110.279183134387));
#28180=CARTESIAN_POINT('Ctrl Pts',(2.81629321096451,1.2345878653493,110.274201210999));
#28181=CARTESIAN_POINT('Ctrl Pts',(2.85368156621807,1.14551617705663,110.269219287611));
#28182=CARTESIAN_POINT('Ctrl Pts',(2.88678788139234,1.05492083961135,110.264237364222));
#28183=CARTESIAN_POINT('Ctrl Pts',(2.92046964321373,0.962750794050624,110.259168846144));
#28184=CARTESIAN_POINT('Ctrl Pts',(2.94971892598634,0.86900406897538,110.254100328066));
#28185=CARTESIAN_POINT('Ctrl Pts',(2.97440751960176,0.774146082685,110.249031809987));
#28186=CARTESIAN_POINT('Ctrl Pts',(2.99871037369669,0.680770176529102,110.244042483448));
#28187=CARTESIAN_POINT('Ctrl Pts',(3.0185940050598,0.586317934023058,110.239053156909));
#28188=CARTESIAN_POINT('Ctrl Pts',(3.033987916313,0.491242886632159,110.23406383037));
#28189=CARTESIAN_POINT('Ctrl Pts',(3.04974833019519,0.39390426540047,110.228955716522));
#28190=CARTESIAN_POINT('Ctrl Pts',(3.06080246555741,0.295913295032107,110.223847602674));
#28191=CARTESIAN_POINT('Ctrl Pts',(3.06713112097644,0.19775979555466,110.218739488825));
#28192=CARTESIAN_POINT('Ctrl Pts',(3.07345977639546,0.0996062960772201,
110.213631374977));
#28193=CARTESIAN_POINT('Ctrl Pts',(3.07506301017686,0.00129075512507518,
110.208523261129));
#28194=CARTESIAN_POINT('Ctrl Pts',(3.07197837451437,-0.0967011712238769,
110.203415147281));
#28195=CARTESIAN_POINT('Ctrl Pts',(3.06895932174052,-0.192609676936675,
110.198415637786));
#28196=CARTESIAN_POINT('Ctrl Pts',(3.06143920317429,-0.288545119294609,
110.193416128292));
#28197=CARTESIAN_POINT('Ctrl Pts',(3.04941095386831,-0.384050887810424,
110.188416618797));
#28198=CARTESIAN_POINT('Ctrl Pts',(3.03739902080607,-0.479427103358187,
110.183423891105));
#28199=CARTESIAN_POINT('Ctrl Pts',(3.02089116504168,-0.574374371642853,
110.178431163413));
#28200=CARTESIAN_POINT('Ctrl Pts',(2.99993231319909,-0.66843725675933,110.173438435721));
#28201=CARTESIAN_POINT('Ctrl Pts',(2.9789955724168,-0.762400907903461,110.168450975231));
#28202=CARTESIAN_POINT('Ctrl Pts',(2.95361726526135,-0.855481604453911,
110.163463514741));
#28203=CARTESIAN_POINT('Ctrl Pts',(2.92389385012061,-0.947231230073669,
110.158476054251));
#28204=CARTESIAN_POINT('Ctrl Pts',(2.89419170277803,-1.03891520669213,110.153492162406));
#28205=CARTESIAN_POINT('Ctrl Pts',(2.86015076294477,-1.1292695893327,110.14850827056));
#28206=CARTESIAN_POINT('Ctrl Pts',(2.8219178410477,-1.21785957662479,110.143524378715));
#28207=CARTESIAN_POINT('Ctrl Pts',(2.78369884263373,-1.30641730163792,110.138542301879));
#28208=CARTESIAN_POINT('Ctrl Pts',(2.74129106913517,-1.39321150535876,110.133560225044));
#28209=CARTESIAN_POINT('Ctrl Pts',(2.69488980915411,-1.4778265008171,110.128578148208));
#28210=CARTESIAN_POINT('Ctrl Pts',(2.64849277989884,-1.56243378133746,110.123596525624));
#28211=CARTESIAN_POINT('Ctrl Pts',(2.59810319931333,-1.64486186383458,110.118614903039));
#28212=CARTESIAN_POINT('Ctrl Pts',(2.54396223207421,-1.72471980674543,110.113633280454));
#28213=CARTESIAN_POINT('Ctrl Pts',(2.48981142105321,-1.80459226923751,110.108650752122));
#28214=CARTESIAN_POINT('Ctrl Pts',(2.43190811514426,-1.88189330078221,110.10366822379));
#28215=CARTESIAN_POINT('Ctrl Pts',(2.37053608480555,-1.95626197648341,110.098685695459));
#28216=CARTESIAN_POINT('Ctrl Pts',(2.30909790446301,-2.03071081065673,110.093697796696));
#28217=CARTESIAN_POINT('Ctrl Pts',(2.24418381543414,-2.10222063992062,110.088709897933));
#28218=CARTESIAN_POINT('Ctrl Pts',(2.17611691919086,-2.17046478985753,110.08372199917));
#28219=CARTESIAN_POINT('Ctrl Pts',(2.10800981489766,-2.23874925255054,110.078731153987));
#28220=CARTESIAN_POINT('Ctrl Pts',(2.03674651916761,-2.30376389908778,110.073740308804));
#28221=CARTESIAN_POINT('Ctrl Pts',(1.96268433556355,-2.36522143761075,110.068749463621));
#28222=CARTESIAN_POINT('Ctrl Pts',(1.88850246560064,-2.42677829306784,110.063750553106));
#28223=CARTESIAN_POINT('Ctrl Pts',(1.81151302658086,-2.48476629835775,110.058751642591));
#28224=CARTESIAN_POINT('Ctrl Pts',(1.73210342396602,-2.53894071980525,110.053752732076));
#28225=CARTESIAN_POINT('Ctrl Pts',(1.68600143742526,-2.57039218620459,110.050850567883));
#28226=CARTESIAN_POINT('Ctrl Pts',(1.63908423686524,-2.60055912638756,110.04794840369));
#28227=CARTESIAN_POINT('Ctrl Pts',(1.5914312251376,-2.62940086439041,110.045046239497));
#28228=CARTESIAN_POINT('Ctrl Pts',(1.50934018250595,-2.67908604184562,110.040046730004));
#28229=CARTESIAN_POINT('Ctrl Pts',(1.42477593332819,-2.72501042574185,110.035047220512));
#28230=CARTESIAN_POINT('Ctrl Pts',(1.33811763243627,-2.76691948776309,110.030047711019));
#28231=CARTESIAN_POINT('Ctrl Pts',(1.25157688297926,-2.80877170040781,110.02505498333));
#28232=CARTESIAN_POINT('Ctrl Pts',(1.16294811904434,-2.8466192267724,110.02006225564));
#28233=CARTESIAN_POINT('Ctrl Pts',(1.0726378171252,-2.88025178817285,110.01506952795));
#28234=CARTESIAN_POINT('Ctrl Pts',(0.982422790298312,-2.91384886806872,
110.010082067462));
#28235=CARTESIAN_POINT('Ctrl Pts',(0.89053016122757,-2.94323967035396,110.005094606974));
#28236=CARTESIAN_POINT('Ctrl Pts',(0.797388323358748,-2.96826112594076,
110.000107146487));
#28237=CARTESIAN_POINT('Ctrl Pts',(0.704313130652064,-2.99326467809123,
109.995123254643));
#28238=CARTESIAN_POINT('Ctrl Pts',(0.609990928771594,-3.01390498506074,
109.9901393628));
#28239=CARTESIAN_POINT('Ctrl Pts',(0.514866356918277,-3.0300684620176,109.985155470957));
#28240=CARTESIAN_POINT('Ctrl Pts',(0.419776427078054,-3.04622605263648,
109.980173394123));
#28241=CARTESIAN_POINT('Ctrl Pts',(0.323885140158247,-3.05790997911342,
109.97519131729));
#28242=CARTESIAN_POINT('Ctrl Pts',(0.227647496366421,-3.06505772660126,
109.970209240457));
#28243=CARTESIAN_POINT('Ctrl Pts',(0.13141862723048,-3.07220482237921,109.965227617874));
#28244=CARTESIAN_POINT('Ctrl Pts',(0.0348439017790225,-3.07481652914136,
109.960245995291));
#28245=CARTESIAN_POINT('Ctrl Pts',(-0.0616174587366106,-3.07288228521348,
109.955264372709));
#28246=CARTESIAN_POINT('Ctrl Pts',(-0.158096357627207,-3.07094768960598,
109.950281844379));
#28247=CARTESIAN_POINT('Ctrl Pts',(-0.25446141177816,-3.06446551064649,
109.94529931605));
#28248=CARTESIAN_POINT('Ctrl Pts',(-0.350255380902445,-3.05347726668284,
109.94031678772));
#28249=CARTESIAN_POINT('Ctrl Pts',(-0.44615260180752,-3.04247717901161,
109.93532888896));
#28250=CARTESIAN_POINT('Ctrl Pts',(-0.541477071980438,-3.02696138014293,
109.930340990199));
#28251=CARTESIAN_POINT('Ctrl Pts',(-0.635778866339523,-3.007023026702,109.925353091438));
#28252=CARTESIAN_POINT('Ctrl Pts',(-0.730136366062876,-2.98707289540202,
109.920362246258));
#28253=CARTESIAN_POINT('Ctrl Pts',(-0.823469562577525,-2.96269511856725,
109.915371401077));
#28254=CARTESIAN_POINT('Ctrl Pts',(-0.915342943206711,-2.93403298316868,
109.910380555896));
#28255=CARTESIAN_POINT('Ctrl Pts',(-1.00736479353926,-2.90532452903543,
109.905381645383));
#28256=CARTESIAN_POINT('Ctrl Pts',(-1.09792170524262,-2.87231804159566,
109.90038273487));
#28257=CARTESIAN_POINT('Ctrl Pts',(-1.18659747408996,-2.83520522793031,
109.895383824357));
#28258=CARTESIAN_POINT('Ctrl Pts',(-1.2380790204009,-2.81365903712443,109.892481660143));
#28259=CARTESIAN_POINT('Ctrl Pts',(-1.28892696056755,-2.79072968876361,
109.889579495928));
#28260=CARTESIAN_POINT('Ctrl Pts',(-1.33906394489701,-2.76646163925634,
109.886677331713));
#28261=CARTESIAN_POINT('Ctrl Pts',(-1.42543408474452,-2.72465547843908,
109.88167782222));
#28262=CARTESIAN_POINT('Ctrl Pts',(-1.5099962411333,-2.67872724112716,109.876678312727));
#28263=CARTESIAN_POINT('Ctrl Pts',(-1.59233048623538,-2.62885638112952,
109.871678803235));
#28264=CARTESIAN_POINT('Ctrl Pts',(-1.67455304545668,-2.57905317063686,
109.866686075545));
#28265=CARTESIAN_POINT('Ctrl Pts',(-1.75455332746351,-2.5253181920119,109.861693347855));
#28266=CARTESIAN_POINT('Ctrl Pts',(-1.83193364535642,-2.4678779080439,109.856700620165));
#28267=CARTESIAN_POINT('Ctrl Pts',(-1.90923232896429,-2.41049822212773,
109.851713159677));
#28268=CARTESIAN_POINT('Ctrl Pts',(-1.98391619252336,-2.34942126198035,
109.846725699189));
#28269=CARTESIAN_POINT('Ctrl Pts',(-2.05561521546054,-2.28491757749971,
109.841738238701));
#28270=CARTESIAN_POINT('Ctrl Pts',(-2.12726293607088,-2.22046004691305,
109.836754346858));
#28271=CARTESIAN_POINT('Ctrl Pts',(-2.19592973637622,-2.15258095900171,
109.831770455014));
#28272=CARTESIAN_POINT('Ctrl Pts',(-2.26127825778897,-2.08159143225824,
109.826786563171));
#28273=CARTESIAN_POINT('Ctrl Pts',(-2.32660298088865,-2.01062775814225,
109.821804486337));
#28274=CARTESIAN_POINT('Ctrl Pts',(-2.38861152913235,-1.93655621846444,
109.816822409504));
#28275=CARTESIAN_POINT('Ctrl Pts',(-2.44700373997525,-1.85972442758253,
109.811840332671));
#28276=CARTESIAN_POINT('Ctrl Pts',(-2.50539062679372,-1.78289964198995,
109.806858710088));
#28277=CARTESIAN_POINT('Ctrl Pts',(-2.56016156630613,-1.70331545515841,
109.801877087505));
#28278=CARTESIAN_POINT('Ctrl Pts',(-2.61105767573447,-1.62135130801073,
109.796895464922));
#28279=CARTESIAN_POINT('Ctrl Pts',(-2.66196303897232,-1.53937225833684,
109.791912936592));
#28280=CARTESIAN_POINT('Ctrl Pts',(-2.70899194143188,-1.45501276189719,
109.786930408263));
#28281=CARTESIAN_POINT('Ctrl Pts',(-2.75193026319493,-1.36867895304629,
109.781947879933));
#28282=CARTESIAN_POINT('Ctrl Pts',(-2.79491486614059,-1.28225208907334,
109.776959981172));
#28283=CARTESIAN_POINT('Ctrl Pts',(-2.83379989034128,-1.19384705798507,
109.771972082412));
#28284=CARTESIAN_POINT('Ctrl Pts',(-2.86841851244245,-1.10389197273894,
109.766984183651));
#28285=CARTESIAN_POINT('Ctrl Pts',(-2.90305758423886,-1.01388374978925,
109.76199333847));
#28286=CARTESIAN_POINT('Ctrl Pts',(-2.93342509763796,-0.922324065945445,
109.757002493289));
#28287=CARTESIAN_POINT('Ctrl Pts',(-2.95940412508885,-0.829656238695951,
109.752011648108));
#28288=CARTESIAN_POINT('Ctrl Pts',(-2.98542513530414,-0.736838657897498,
109.747012737595));
#28289=CARTESIAN_POINT('Ctrl Pts',(-3.00704340021671,-0.642909785376251,
109.742013827082));
#28290=CARTESIAN_POINT('Ctrl Pts',(-3.02419311920603,-0.548323105246242,
109.737014916569));
#28291=CARTESIAN_POINT('Ctrl Pts',(-3.03414954883091,-0.493409924175956,
109.734112752355));
#28292=CARTESIAN_POINT('Ctrl Pts',(-3.04260082871646,-0.438275144761581,
109.731210588142));
#28293=CARTESIAN_POINT('Ctrl Pts',(-3.04954213539411,-0.383007851689662,
109.728308423928));
#28294=CARTESIAN_POINT('Ctrl Pts',(-3.06539555968381,-0.256781495889267,
109.721680098345));
#28295=CARTESIAN_POINT('Ctrl Pts',(-3.07341405992647,-0.129550961238268,
109.715051772761));
#28296=CARTESIAN_POINT('Ctrl Pts',(-3.0734993128837,-0.00205516505886973,
109.708423447177));
#28297=CARTESIAN_POINT('Ctrl Pts',(-3.07349931288414,-0.0020551643988658,
109.708423447143));
#28298=CARTESIAN_POINT('Ctrl Pts',(-3.07356266900829,0.0926939486859775,
109.70349757516));
#28299=CARTESIAN_POINT('Ctrl Pts',(-3.06924046811866,0.187612347631797,
109.698571703178));
#28300=CARTESIAN_POINT('Ctrl Pts',(-3.0605122154393,0.282253838143699,109.693645831195));
#28301=CARTESIAN_POINT('Ctrl Pts',(-3.05137897652877,0.381286642926907,
109.688491401402));
#28302=CARTESIAN_POINT('Ctrl Pts',(-3.03742083355291,0.480015730082625,
109.683336971608));
#28303=CARTESIAN_POINT('Ctrl Pts',(-3.01867547972599,0.577927848525294,
109.678182541814));
#28304=CARTESIAN_POINT('Ctrl Pts',(-3.00079765234977,0.671308638651749,
109.673266656687));
#28305=CARTESIAN_POINT('Ctrl Pts',(-2.97856592490908,0.763945887153016,
109.66835077156));
#28306=CARTESIAN_POINT('Ctrl Pts',(-2.95206600206826,0.855399654800428,
109.663434886433));
#28307=CARTESIAN_POINT('Ctrl Pts',(-2.92557704384696,0.946815582497475,
109.658521035305));
#28308=CARTESIAN_POINT('Ctrl Pts',(-2.89482352222469,1.03704856765137,109.653607184177));
#28309=CARTESIAN_POINT('Ctrl Pts',(-2.85994172243619,1.12567117501904,109.648693333049));
#28310=CARTESIAN_POINT('Ctrl Pts',(-2.82506420199237,1.21428291004966,109.643780084758));
#28311=CARTESIAN_POINT('Ctrl Pts',(-2.78605957572621,1.30128423906308,109.638866836468));
#28312=CARTESIAN_POINT('Ctrl Pts',(-2.74311281379706,1.38626633111476,109.633953588177));
#28313=CARTESIAN_POINT('Ctrl Pts',(-2.70015881922103,1.47126273496634,109.629039512449));
#28314=CARTESIAN_POINT('Ctrl Pts',(-2.65326157639766,1.55423882374924,109.62412543672));
#28315=CARTESIAN_POINT('Ctrl Pts',(-2.6026520919461,1.63481018417692,109.619211360991));
#28316=CARTESIAN_POINT('Ctrl Pts',(-2.55198980139593,1.71546561302084,109.6142921579));
#28317=CARTESIAN_POINT('Ctrl Pts',(-2.49760778202127,1.79371092387224,109.609372954809));
#28318=CARTESIAN_POINT('Ctrl Pts',(-2.43978020987164,1.86919094196358,109.604453751718));
#28319=CARTESIAN_POINT('Ctrl Pts',(-2.38191726870418,1.94471712581991,109.5995315399));
#28320=CARTESIAN_POINT('Ctrl Pts',(-2.32060487432343,2.01747430775393,109.594609328082));
#28321=CARTESIAN_POINT('Ctrl Pts',(-2.25615582270311,2.08714234150018,109.589687116264));
#28322=CARTESIAN_POINT('Ctrl Pts',(-2.19160825703757,2.15691686680301,109.584757380564));
#28323=CARTESIAN_POINT('Ctrl Pts',(-2.1239147913646,2.22359250862423,109.579827644865));
#28324=CARTESIAN_POINT('Ctrl Pts',(-2.05342285426502,2.28688802340257,109.574897909166));
#28325=CARTESIAN_POINT('Ctrl Pts',(-2.02978894835492,2.30810917723027,109.573245111492));
#28326=CARTESIAN_POINT('Ctrl Pts',(-2.00584072734789,2.32895073584105,109.571592313818));
#28327=CARTESIAN_POINT('Ctrl Pts',(-1.9815920072361,2.34940319376177,109.569939516144));
#28328=CARTESIAN_POINT('Ctrl Pts',(-1.90824261408625,2.41126936113027,109.564940006651));
#28329=CARTESIAN_POINT('Ctrl Pts',(-1.83186437798168,2.46980589951436,109.559940497158));
#28330=CARTESIAN_POINT('Ctrl Pts',(-1.75279217700187,2.52470232586756,109.554940987665));
#28331=CARTESIAN_POINT('Ctrl Pts',(-1.67382723696063,2.57952428556696,109.549948259975));
#28332=CARTESIAN_POINT('Ctrl Pts',(-1.59217595231317,2.63071569856871,109.544955532285));
#28333=CARTESIAN_POINT('Ctrl Pts',(-1.5082070821448,2.67800553535056,109.539962804595));
#28334=CARTESIAN_POINT('Ctrl Pts',(-1.42432679701802,2.72524548254656,109.534975344107));
#28335=CARTESIAN_POINT('Ctrl Pts',(-1.33813416731467,2.76859182175116,109.529987883619));
#28336=CARTESIAN_POINT('Ctrl Pts',(-1.25002695547136,2.80781674270153,109.525000423131));
#28337=CARTESIAN_POINT('Ctrl Pts',(-1.16198278639743,2.84701359730415,109.520016531287));
#28338=CARTESIAN_POINT('Ctrl Pts',(-1.07202715840337,2.88209471804872,109.515032639443));
#28339=CARTESIAN_POINT('Ctrl Pts',(-0.980581589636902,2.91287864423926,
109.5100487476));
#28340=CARTESIAN_POINT('Ctrl Pts',(-0.889169323081802,2.94365135968629,
109.505066670766));
#28341=CARTESIAN_POINT('Ctrl Pts',(-0.796268609437589,2.97012985002376,
109.500084593933));
#28342=CARTESIAN_POINT('Ctrl Pts',(-0.702319156661911,2.99218148717382,
109.495102517099));
#28343=CARTESIAN_POINT('Ctrl Pts',(-0.608378269911635,3.01423111372265,
109.490120894516));
#28344=CARTESIAN_POINT('Ctrl Pts',(-0.513389261531923,3.03185458944141,
109.485139271933));
#28345=CARTESIAN_POINT('Ctrl Pts',(-0.417804101854027,3.04496994771278,
109.48015764935));
#28346=CARTESIAN_POINT('Ctrl Pts',(-0.322201563110231,3.05808769058732,
109.47517512102));
#28347=CARTESIAN_POINT('Ctrl Pts',(-0.226003092691896,3.06669562854235,
109.47019259269));
#28348=CARTESIAN_POINT('Ctrl Pts',(-0.129666816763162,3.0707635478217,109.465210064361));
#28349=CARTESIAN_POINT('Ctrl Pts',(-0.0332267045267823,3.07483585171851,
109.4602221656));
#28350=CARTESIAN_POINT('Ctrl Pts',(0.0633510704557592,3.07435834902676,
109.455234266839));
#28351=CARTESIAN_POINT('Ctrl Pts',(0.159607564124986,3.0693529734252,109.450246368078));
#28352=CARTESIAN_POINT('Ctrl Pts',(0.255920917826297,3.06434464107956,109.445255522897));
#28353=CARTESIAN_POINT('Ctrl Pts',(0.351912175715045,3.05480315350409,109.440264677715));
#28354=CARTESIAN_POINT('Ctrl Pts',(0.447128821294317,3.04080220783397,109.435273832534));
#28355=CARTESIAN_POINT('Ctrl Pts',(0.542499339377329,3.02677863628209,109.430274922021));
#28356=CARTESIAN_POINT('Ctrl Pts',(0.63709231508409,3.00828130083954,109.425276011508));
#28357=CARTESIAN_POINT('Ctrl Pts',(0.73046676216636,2.98543473540625,109.420277100995));
#28358=CARTESIAN_POINT('Ctrl Pts',(0.784676169975338,2.97217094834986,109.417374936783));
#28359=CARTESIAN_POINT('Ctrl Pts',(0.83847516344876,2.95744218974732,109.414472772572));
#28360=CARTESIAN_POINT('Ctrl Pts',(0.891780412031208,2.94128032440253,109.41157060836));
#28361=CARTESIAN_POINT('Ctrl Pts',(0.983586075158197,2.91344533995343,109.406572318003));
#28362=CARTESIAN_POINT('Ctrl Pts',(1.0742484876445,2.8812590886785,109.401574027646));
#28363=CARTESIAN_POINT('Ctrl Pts',(1.16332521637671,2.84483333271777,109.39657573729));
#28364=CARTESIAN_POINT('Ctrl Pts',(1.25229627227011,2.8084507890875,109.391583376467));
#28365=CARTESIAN_POINT('Ctrl Pts',(1.33968497736054,2.76783889229763,109.386591015645));
#28366=CARTESIAN_POINT('Ctrl Pts',(1.42506331255238,2.72315934260507,109.381598654823));
#28367=CARTESIAN_POINT('Ctrl Pts',(1.51035007260189,2.6785277153288,109.37661164871));
#28368=CARTESIAN_POINT('Ctrl Pts',(1.59363036303518,2.62983731152457,109.371624642597));
#28369=CARTESIAN_POINT('Ctrl Pts',(1.67449663930034,2.57729766518574,109.366637636483));
#28370=CARTESIAN_POINT('Ctrl Pts',(1.7422269802255,2.53329257031841,109.362460720718));
#28371=CARTESIAN_POINT('Ctrl Pts',(1.80826409501652,2.48658811596448,109.358283804952));
#28372=CARTESIAN_POINT('Ctrl Pts',(1.8723819390353,2.43733217358128,109.354106889186));
#28373=CARTESIAN_POINT('',(-3.07349977118745,0.0011859640259134,109.791576552796));
#28374=CARTESIAN_POINT('Ctrl Pts',(-3.07349977118745,0.0011859640259162,
109.791576552796));
#28375=CARTESIAN_POINT('Ctrl Pts',(-3.07345762578049,0.110408415828411,
109.785948464215));
#28376=CARTESIAN_POINT('Ctrl Pts',(-3.06758844717733,0.219451566251278,
109.780320375635));
#28377=CARTESIAN_POINT('Ctrl Pts',(-3.05597865567814,0.327714366544475,
109.774692287054));
#28378=CARTESIAN_POINT('Ctrl Pts',(-3.04477419212563,0.43219743155575,109.769260689649));
#28379=CARTESIAN_POINT('Ctrl Pts',(-3.02822341391354,0.535953470050506,
109.763829092245));
#28380=CARTESIAN_POINT('Ctrl Pts',(-3.00645543748823,0.638457478926707,
109.758397494841));
#28381=CARTESIAN_POINT('Ctrl Pts',(-2.98350625736496,0.746523700476025,
109.752671160672));
#28382=CARTESIAN_POINT('Ctrl Pts',(-2.95475800377033,0.85319780148342,109.746944826503));
#28383=CARTESIAN_POINT('Ctrl Pts',(-2.9204200294292,0.957887833573822,109.741218492334));
#28384=CARTESIAN_POINT('Ctrl Pts',(-2.88608205508808,1.06257786566422,109.735492158165));
#28385=CARTESIAN_POINT('Ctrl Pts',(-2.84615458915357,1.16528350101537,109.729765823996));
#28386=CARTESIAN_POINT('Ctrl Pts',(-2.80090335864964,1.26544167210708,109.724039489827));
#28387=CARTESIAN_POINT('Ctrl Pts',(-2.76139571732356,1.3528870974646,109.719039980335));
#28388=CARTESIAN_POINT('Ctrl Pts',(-2.71771963209727,1.43863417236837,109.714040470842));
#28389=CARTESIAN_POINT('Ctrl Pts',(-2.67004338980336,1.5222583705033,109.70904096135));
#28390=CARTESIAN_POINT('Ctrl Pts',(-2.62243182002944,1.60576913294437,109.70404823366));
#28391=CARTESIAN_POINT('Ctrl Pts',(-2.57083109292843,1.68716236368984,109.69905550597));
#28392=CARTESIAN_POINT('Ctrl Pts',(-2.51545707599578,1.76603452650925,109.69406277828));
#28393=CARTESIAN_POINT('Ctrl Pts',(-2.46014147725528,1.84482348118488,109.689075317793));
#28394=CARTESIAN_POINT('Ctrl Pts',(-2.40106075301206,1.92109629783268,109.684087857305));
#28395=CARTESIAN_POINT('Ctrl Pts',(-2.33847557403926,1.99447593107106,109.679100396817));
#28396=CARTESIAN_POINT('Ctrl Pts',(-2.2759351762249,2.06780305946666,109.674116504974));
#28397=CARTESIAN_POINT('Ctrl Pts',(-2.20989559254838,2.13824078676674,109.66913261313));
#28398=CARTESIAN_POINT('Ctrl Pts',(-2.14065891187789,2.2054436453915,109.664148721287));
#28399=CARTESIAN_POINT('Ctrl Pts',(-2.07144744549171,2.27262203039957,109.659166644454));
#28400=CARTESIAN_POINT('Ctrl Pts',(-1.99904151011945,2.33656758198775,109.65418456762));
#28401=CARTESIAN_POINT('Ctrl Pts',(-1.92378066131403,2.3969710505457,109.649202490787));
#28402=CARTESIAN_POINT('Ctrl Pts',(-1.84852667456408,2.45736901169896,109.644220868204));
#28403=CARTESIAN_POINT('Ctrl Pts',(-1.77041863436421,2.51422525730453,109.639239245622));
#28404=CARTESIAN_POINT('Ctrl Pts',(-1.68982900327128,2.56727096148871,109.634257623039));
#28405=CARTESIAN_POINT('Ctrl Pts',(-1.60922471956359,2.62032631031647,109.62927509471));
#28406=CARTESIAN_POINT('Ctrl Pts',(-1.52613831556261,2.66956950046214,109.62429256638));
#28407=CARTESIAN_POINT('Ctrl Pts',(-1.44097012159478,2.71477574739998,109.619310038051));
#28408=CARTESIAN_POINT('Ctrl Pts',(-1.35571012886561,2.7600307200097,109.61432213929));
#28409=CARTESIAN_POINT('Ctrl Pts',(-1.26836425487647,2.80123985644017,109.609334240529));
#28410=CARTESIAN_POINT('Ctrl Pts',(-1.17935605154246,2.83822507100656,109.604346341769));
#28411=CARTESIAN_POINT('Ctrl Pts',(-1.09029526984105,2.87523213324683,109.599355496588));
#28412=CARTESIAN_POINT('Ctrl Pts',(-0.99957061620157,2.90801015632687,109.594364651407));
#28413=CARTESIAN_POINT('Ctrl Pts',(-0.90762216115675,2.93643053086177,109.589373806226));
#28414=CARTESIAN_POINT('Ctrl Pts',(-0.815525115086421,2.96489683343968,
109.584374895713));
#28415=CARTESIAN_POINT('Ctrl Pts',(-0.722200743331968,2.98899131635566,
109.5793759852));
#28416=CARTESIAN_POINT('Ctrl Pts',(-0.628100631454975,3.00863621043919,
109.574377074688));
#28417=CARTESIAN_POINT('Ctrl Pts',(-0.573469932105146,3.02004123728803,
109.571474910473));
#28418=CARTESIAN_POINT('Ctrl Pts',(-0.518577910963521,3.02994750048335,
109.568572746258));
#28419=CARTESIAN_POINT('Ctrl Pts',(-0.463513494017647,3.03834782256139,
109.565670582043));
#28420=CARTESIAN_POINT('Ctrl Pts',(-0.368642163266014,3.05282086665209,
109.560670398687));
#28421=CARTESIAN_POINT('Ctrl Pts',(-0.272925651907291,3.06287158957453,
109.555670215331));
#28422=CARTESIAN_POINT('Ctrl Pts',(-0.176811855286777,3.06840998203142,
109.550670031975));
#28423=CARTESIAN_POINT('Ctrl Pts',(-0.0808588487974082,3.07393910923315,
109.545678213497));
#28424=CARTESIAN_POINT('Ctrl Pts',(0.0154896860225316,3.07497089992223,
109.540686395018));
#28425=CARTESIAN_POINT('Ctrl Pts',(0.111777985423372,3.07146673951952,109.53569457654));
#28426=CARTESIAN_POINT('Ctrl Pts',(0.207974068326147,3.06796593509467,109.530707538788));
#28427=CARTESIAN_POINT('Ctrl Pts',(0.304109594399434,3.05993782606783,109.525720501036));
#28428=CARTESIAN_POINT('Ctrl Pts',(0.399726494775764,3.04739577005913,109.520733463284));
#28429=CARTESIAN_POINT('Ctrl Pts',(0.495277928487216,3.03486230130409,109.51574984004));
#28430=CARTESIAN_POINT('Ctrl Pts',(0.590311008371727,3.01782108468474,109.510766216797));
#28431=CARTESIAN_POINT('Ctrl Pts',(0.68437155856275,2.99633740086633,109.505782593553));
#28432=CARTESIAN_POINT('Ctrl Pts',(0.778393387336073,2.97486256112435,109.500801021892));
#28433=CARTESIAN_POINT('Ctrl Pts',(0.871443055207516,2.94894898843552,109.495819450231));
#28434=CARTESIAN_POINT('Ctrl Pts',(0.96307642652806,2.91871308056581,109.49083787857));
#28435=CARTESIAN_POINT('Ctrl Pts',(1.05472610292954,2.88847179257183,109.485855420497));
#28436=CARTESIAN_POINT('Ctrl Pts',(1.14495855950261,2.853906761974,109.480872962423));
#28437=CARTESIAN_POINT('Ctrl Pts',(1.233345300022,2.81518411847496,109.47589050435));
#28438=CARTESIAN_POINT('Ctrl Pts',(1.32173929949388,2.77645829479497,109.470907637082));
#28439=CARTESIAN_POINT('Ctrl Pts',(1.40828688260833,2.73357436304779,109.465924769813));
#28440=CARTESIAN_POINT('Ctrl Pts',(1.49258145628562,2.68674577255688,109.460941902545));
#28441=CARTESIAN_POINT('Ctrl Pts',(1.5769463622301,2.63987811002617,109.455954877757));
#28442=CARTESIAN_POINT('Ctrl Pts',(1.6590541258067,2.58905943849805,109.450967852969));
#28443=CARTESIAN_POINT('Ctrl Pts',(1.73852496201855,2.53454792940248,109.445980828181));
#28444=CARTESIAN_POINT('Ctrl Pts',(1.78403016060481,2.50333450363685,109.443125245376));
#28445=CARTESIAN_POINT('Ctrl Pts',(1.8286713227525,2.47091108800218,109.440269662572));
#28446=CARTESIAN_POINT('Ctrl Pts',(1.87238193903529,2.43733217358128,109.437414079767));
#28447=CARTESIAN_POINT('Ctrl Pts',(1.8723819390353,2.43733217358127,110.437319612009));
#28448=CARTESIAN_POINT('Ctrl Pts',(1.94890666575668,2.37854514497852,110.432337890837));
#28449=CARTESIAN_POINT('Ctrl Pts',(2.02266101654233,2.31615004673507,110.427356169666));
#28450=CARTESIAN_POINT('Ctrl Pts',(2.09329697097887,2.25044663151355,110.422374448494));
#28451=CARTESIAN_POINT('Ctrl Pts',(2.16395057773146,2.18472679664483,110.417391482363));
#28452=CARTESIAN_POINT('Ctrl Pts',(2.23148391885292,2.11569730151574,110.412408516232));
#28453=CARTESIAN_POINT('Ctrl Pts',(2.29558537922392,2.0436951868352,110.4074255501));
#28454=CARTESIAN_POINT('Ctrl Pts',(2.35975826823993,1.97161283976277,110.40243703142));
#28455=CARTESIAN_POINT('Ctrl Pts',(2.42049135228201,1.8965515907143,110.397448512739));
#28456=CARTESIAN_POINT('Ctrl Pts',(2.47751310099432,1.81888182254964,110.392459994058));
#28457=CARTESIAN_POINT('Ctrl Pts',(2.53457201502878,1.74116143121013,110.387468223988));
#28458=CARTESIAN_POINT('Ctrl Pts',(2.58791453587653,1.6608295014096,110.382476453918));
#28459=CARTESIAN_POINT('Ctrl Pts',(2.6373134392608,1.57828390129734,110.377484683848));
#28460=CARTESIAN_POINT('Ctrl Pts',(2.68678864765634,1.49561079546099,110.37248520314));
#28461=CARTESIAN_POINT('Ctrl Pts',(2.73230787459593,1.41071758103269,110.367485722432));
#28462=CARTESIAN_POINT('Ctrl Pts',(2.77369074462531,1.32402488767389,110.362486241724));
#28463=CARTESIAN_POINT('Ctrl Pts',(2.78740678543857,1.29529124693134,110.360829201471));
#28464=CARTESIAN_POINT('Ctrl Pts',(2.80066883094348,1.2663600695108,110.359172161217));
#28465=CARTESIAN_POINT('Ctrl Pts',(2.8134715159664,1.23724705651124,110.357515120964));
#28466=CARTESIAN_POINT('Ctrl Pts',(2.85209890920228,1.14940924753587,110.352515611458));
#28467=CARTESIAN_POINT('Ctrl Pts',(2.88667670388421,1.05960647784786,110.347516101952));
#28468=CARTESIAN_POINT('Ctrl Pts',(2.91700165563847,0.968247690935769,110.342516592446));
#28469=CARTESIAN_POINT('Ctrl Pts',(2.94728547178935,0.877012831634629,110.337523864743));
#28470=CARTESIAN_POINT('Ctrl Pts',(2.9733277733235,0.78422656308776,110.33253113704));
#28471=CARTESIAN_POINT('Ctrl Pts',(2.99497273314224,0.690319185402311,110.327538409336));
#28472=CARTESIAN_POINT('Ctrl Pts',(3.01659485807464,0.596510877630301,110.322550948835));
#28473=CARTESIAN_POINT('Ctrl Pts',(3.03382876544318,0.501584237411476,110.317563488333));
#28474=CARTESIAN_POINT('Ctrl Pts',(3.04656827999061,0.405985178738126,110.312576027832));
#28475=CARTESIAN_POINT('Ctrl Pts',(3.05929867911811,0.310454523422114,110.307592135975));
#28476=CARTESIAN_POINT('Ctrl Pts',(3.06754102055111,0.214252839985739,110.302608244118));
#28477=CARTESIAN_POINT('Ctrl Pts',(3.07124030137914,0.117835738146636,110.29762435226));
#28478=CARTESIAN_POINT('Ctrl Pts',(3.0749382350208,0.0214537490259393,110.292642275413));
#28479=CARTESIAN_POINT('Ctrl Pts',(3.07409637849752,-0.0751430644344541,
110.287660198566));
#28480=CARTESIAN_POINT('Ctrl Pts',(3.06871171095375,-0.171495437418373,
110.282678121719));
#28481=CARTESIAN_POINT('Ctrl Pts',(3.06332753436751,-0.267839025287296,
110.277696499122));
#28482=CARTESIAN_POINT('Ctrl Pts',(3.0534013949426,-0.363937778722953,110.272714876525));
#28483=CARTESIAN_POINT('Ctrl Pts',(3.03898233389616,-0.459334980452197,
110.267733253928));
#28484=CARTESIAN_POINT('Ctrl Pts',(3.02456065121019,-0.554749527074792,
110.262750725585));
#28485=CARTESIAN_POINT('Ctrl Pts',(3.00564449019055,-0.649461834644932,
110.257768197241));
#28486=CARTESIAN_POINT('Ctrl Pts',(2.98233427614312,-0.743023899576512,
110.252785668898));
#28487=CARTESIAN_POINT('Ctrl Pts',(2.95899893712032,-0.83668681062525,110.247797770123));
#28488=CARTESIAN_POINT('Ctrl Pts',(2.93126019609635,-0.929196577256966,
110.242809871348));
#28489=CARTESIAN_POINT('Ctrl Pts',(2.89926873314341,-1.02011914157956,110.237821972573));
#28490=CARTESIAN_POINT('Ctrl Pts',(2.8672583723941,-1.11109541510914,110.232831127378));
#28491=CARTESIAN_POINT('Ctrl Pts',(2.8309904525927,-1.20048221288414,110.227840282183));
#28492=CARTESIAN_POINT('Ctrl Pts',(2.79066349358526,-1.28786626462942,110.222849436988));
#28493=CARTESIAN_POINT('Ctrl Pts',(2.7502713651945,-1.37539153120726,110.217850526461));
#28494=CARTESIAN_POINT('Ctrl Pts',(2.70580730207173,-1.46090720000393,110.212851615934));
#28495=CARTESIAN_POINT('Ctrl Pts',(2.65751533350989,-1.54402542147461,110.207852705408));
#28496=CARTESIAN_POINT('Ctrl Pts',(2.62947898127678,-1.59228047927282,110.204950541332));
#28497=CARTESIAN_POINT('Ctrl Pts',(2.60015324980404,-1.63972802094159,110.202048377256));
#28498=CARTESIAN_POINT('Ctrl Pts',(2.56959224488743,-1.68629711053965,110.19914621318));
#28499=CARTESIAN_POINT('Ctrl Pts',(2.51694531310072,-1.76652090194077,110.194146703689));
#28500=CARTESIAN_POINT('Ctrl Pts',(2.46044537719295,-1.84441774726801,110.189147194198));
#28501=CARTESIAN_POINT('Ctrl Pts',(2.40032479908744,-1.91959451678885,110.184147684707));
#28502=CARTESIAN_POINT('Ctrl Pts',(2.34028577416437,-1.99466930949921,110.179154957019));
#28503=CARTESIAN_POINT('Ctrl Pts',(2.27663613989706,-2.06703101968213,110.174162229331));
#28504=CARTESIAN_POINT('Ctrl Pts',(2.20965198838535,-2.13631466320499,110.169169501643));
#28505=CARTESIAN_POINT('Ctrl Pts',(2.14273850346508,-2.2055252142303,110.164182041156));
#28506=CARTESIAN_POINT('Ctrl Pts',(2.07249779802678,-2.27166384008945,110.15919458067));
#28507=CARTESIAN_POINT('Ctrl Pts',(1.99924609399943,-2.33439870322703,110.154207120184));
#28508=CARTESIAN_POINT('Ctrl Pts',(1.92604680327836,-2.39708867810378,110.149223228342));
#28509=CARTESIAN_POINT('Ctrl Pts',(1.84984112933959,-2.45637944714489,110.1442393365));
#28510=CARTESIAN_POINT('Ctrl Pts',(1.77098128767597,-2.51197681691164,110.139255444659));
#28511=CARTESIAN_POINT('Ctrl Pts',(1.69215016481352,-2.56755393949334,110.134273367827));
#28512=CARTESIAN_POINT('Ctrl Pts',(1.610667153118,-2.61944008258216,110.129291290995));
#28513=CARTESIAN_POINT('Ctrl Pts',(1.52691583566181,-2.66738266486179,110.124309214163));
#28514=CARTESIAN_POINT('Ctrl Pts',(1.44317215439605,-2.71532087588257,110.119327591582));
#28515=CARTESIAN_POINT('Ctrl Pts',(1.35716095961153,-2.75931602305225,110.114345969001));
#28516=CARTESIAN_POINT('Ctrl Pts',(1.26929204279809,-2.79916058133317,110.10936434642));
#28517=CARTESIAN_POINT('Ctrl Pts',(1.18140714986676,-2.8390123840571,110.104381818092));
#28518=CARTESIAN_POINT('Ctrl Pts',(1.09166426389277,-2.87471191790758,110.099399289764));
#28519=CARTESIAN_POINT('Ctrl Pts',(1.00049384353992,-2.9060995026046,110.094416761436));
#28520=CARTESIAN_POINT('Ctrl Pts',(0.9092251549101,-2.93752091849221,110.089428862677));
#28521=CARTESIAN_POINT('Ctrl Pts',(0.816526275827664,-2.96462096350184,
110.084440963918));
#28522=CARTESIAN_POINT('Ctrl Pts',(0.722843328701962,-2.98728970341865,
110.079453065158));
#28523=CARTESIAN_POINT('Ctrl Pts',(0.629105041773077,-3.00997183407138,
110.074462219979));
#28524=CARTESIAN_POINT('Ctrl Pts',(0.534381960170196,-3.0282173645088,110.0694713748));
#28525=CARTESIAN_POINT('Ctrl Pts',(0.439128816249519,-3.04196780599981,
110.06448052962));
#28526=CARTESIAN_POINT('Ctrl Pts',(0.343721740842073,-3.05574046855162,
110.059481619109));
#28527=CARTESIAN_POINT('Ctrl Pts',(0.247783329323794,-3.06500349504237,
110.054482708597));
#28528=CARTESIAN_POINT('Ctrl Pts',(0.151771769027837,-3.0697504100702,110.049483798086));
#28529=CARTESIAN_POINT('Ctrl Pts',(0.0960313601271893,-3.07250627596647,
110.046581633856));
#28530=CARTESIAN_POINT('Ctrl Pts',(0.0402662849811449,-3.07374096692459,
110.043679469626));
#28531=CARTESIAN_POINT('Ctrl Pts',(-0.0154344978905223,-3.07346124528598,
110.040777305396));
#28532=CARTESIAN_POINT('Ctrl Pts',(-0.111389299388775,-3.07297937352541,
110.035777795905));
#28533=CARTESIAN_POINT('Ctrl Pts',(-0.207490050581665,-3.06799872221208,
110.030778286414));
#28534=CARTESIAN_POINT('Ctrl Pts',(-0.303280487470693,-3.05850015463782,
110.025778776924));
#28535=CARTESIAN_POINT('Ctrl Pts',(-0.398940985239289,-3.04901447181025,
110.020786049236));
#28536=CARTESIAN_POINT('Ctrl Pts',(-0.49429157220971,-3.03502309570359,
110.015793321548));
#28537=CARTESIAN_POINT('Ctrl Pts',(-0.588875783732631,-3.01655889406013,
110.01080059386));
#28538=CARTESIAN_POINT('Ctrl Pts',(-0.683360211295895,-2.99811417168411,
110.005813133374));
#28539=CARTESIAN_POINT('Ctrl Pts',(-0.777079442135289,-2.97520608795508,
110.000825672888));
#28540=CARTESIAN_POINT('Ctrl Pts',(-0.869582965946565,-2.94791921791211,
109.995838212402));
#28541=CARTESIAN_POINT('Ctrl Pts',(-0.962020301323166,-2.92065187226283,
109.990854320561));
#28542=CARTESIAN_POINT('Ctrl Pts',(-1.0532432391063,-2.88901209264129,109.98587042872));
#28543=CARTESIAN_POINT('Ctrl Pts',(-1.14281324783431,-2.85313514060838,
109.980886536879));
#28544=CARTESIAN_POINT('Ctrl Pts',(-1.23235063738287,-2.8172712540731,109.975904460047));
#28545=CARTESIAN_POINT('Ctrl Pts',(-1.32023588682419,-2.77717342409716,
109.970922383216));
#28546=CARTESIAN_POINT('Ctrl Pts',(-1.40604829049614,-2.7330258789102,109.965940306385));
#28547=CARTESIAN_POINT('Ctrl Pts',(-1.49185287005355,-2.68888235896243,
109.960958683804));
#28548=CARTESIAN_POINT('Ctrl Pts',(-1.57558458934891,-2.6406900588997,109.955977061223));
#28549=CARTESIAN_POINT('Ctrl Pts',(-1.65684626636518,-2.58867972133127,
109.950995438643));
#28550=CARTESIAN_POINT('Ctrl Pts',(-1.73812271818616,-2.53665992736706,
109.946012910315));
#28551=CARTESIAN_POINT('Ctrl Pts',(-1.81692786612375,-2.48082095390266,
109.941030381988));
#28552=CARTESIAN_POINT('Ctrl Pts',(-1.89289340769943,-2.42143692816642,
109.936047853661));
#28553=CARTESIAN_POINT('Ctrl Pts',(-1.96894082893254,-2.36198889520291,
109.931059954902));
#28554=CARTESIAN_POINT('Ctrl Pts',(-2.04214218703748,-2.29898845240086,
109.926072056143));
#28555=CARTESIAN_POINT('Ctrl Pts',(-2.11216237800063,-2.23274994994037,
109.921084157385));
#28556=CARTESIAN_POINT('Ctrl Pts',(-2.1822239308512,-2.16647231948774,109.916093312206));
#28557=CARTESIAN_POINT('Ctrl Pts',(-2.24910027066741,-2.09695313694679,
109.911102467027));
#28558=CARTESIAN_POINT('Ctrl Pts',(-2.31249475781148,-2.02454198402859,
109.906111621849));
#28559=CARTESIAN_POINT('Ctrl Pts',(-2.37599169204783,-1.9520138128585,109.901112711338));
#28560=CARTESIAN_POINT('Ctrl Pts',(-2.43599526512317,-1.87658468266414,
109.896113800827));
#28561=CARTESIAN_POINT('Ctrl Pts',(-2.4922505847114,-1.7986353919029,109.891114890317));
#28562=CARTESIAN_POINT('Ctrl Pts',(-2.52491013646644,-1.75338120235213,
109.888212726082));
#28563=CARTESIAN_POINT('Ctrl Pts',(-2.55630716799028,-1.70727811687191,
109.885310561847));
#28564=CARTESIAN_POINT('Ctrl Pts',(-2.58639891787753,-1.66040443495009,
109.882408397611));
#28565=CARTESIAN_POINT('Ctrl Pts',(-2.63940236178393,-1.57784138761193,
109.877296541378));
#28566=CARTESIAN_POINT('Ctrl Pts',(-2.68853322212055,-1.49260657041294,
109.872184685144));
#28567=CARTESIAN_POINT('Ctrl Pts',(-2.73351906787153,-1.40508923402848,
109.867072828911));
#28568=CARTESIAN_POINT('Ctrl Pts',(-2.77843555048245,-1.31770683958322,
109.861968854587));
#28569=CARTESIAN_POINT('Ctrl Pts',(-2.81921954317603,-1.22804928973175,
109.856864880264));
#28570=CARTESIAN_POINT('Ctrl Pts',(-2.85564221881624,-1.13653410336614,
109.851760905941));
#28571=CARTESIAN_POINT('Ctrl Pts',(-2.89200450421949,-1.04517065279952,
109.846665394209));
#28572=CARTESIAN_POINT('Ctrl Pts',(-2.92401972075752,-0.951956080133295,
109.841569882477));
#28573=CARTESIAN_POINT('Ctrl Pts',(-2.95150578637871,-0.857330649733813,
109.836474370745));
#28574=CARTESIAN_POINT('Ctrl Pts',(-2.97896501450207,-0.762797611960408,
109.83138383429));
#28575=CARTESIAN_POINT('Ctrl Pts',(-3.00190377183239,-0.666856850360775,
109.826293297835));
#28576=CARTESIAN_POINT('Ctrl Pts',(-3.02018879123147,-0.569966591406704,
109.82120276138));
#28577=CARTESIAN_POINT('Ctrl Pts',(-3.03845833192543,-0.47315835236822,
109.816116534185));
#28578=CARTESIAN_POINT('Ctrl Pts',(-3.05208189904631,-0.375402620030141,
109.81103030699));
#28579=CARTESIAN_POINT('Ctrl Pts',(-3.06097682462202,-0.277169856093556,
109.805944079796));
#28580=CARTESIAN_POINT('Ctrl Pts',(-3.06935225879234,-0.184674192052551,
109.801154904138));
#28581=CARTESIAN_POINT('Ctrl Pts',(-3.07353563445906,-0.091755982939446,
109.796365728481));
#28582=CARTESIAN_POINT('Ctrl Pts',(-3.07349977118766,0.0011859635037227,
109.791576552823));
#28583=CARTESIAN_POINT('Origin',(0.,0.,116.208423447177));
#28584=CARTESIAN_POINT('',(1.87238193903529,2.43733217358128,111.437229631665));
#28585=CARTESIAN_POINT('',(1.87238193903529,2.43733217358128,111.354256900092));
#28586=CARTESIAN_POINT('',(1.8723819390353,2.43733217358128,116.208423447177));
#28587=CARTESIAN_POINT('',(-3.07349888025591,0.00262355973274775,110.708423447212));
#28588=CARTESIAN_POINT('Ctrl Pts',(1.87238193903529,2.43733217358128,111.354256900092));
#28589=CARTESIAN_POINT('Ctrl Pts',(1.948881640316,2.37856436976194,111.349266871793));
#28590=CARTESIAN_POINT('Ctrl Pts',(2.02254958126843,2.31623943328911,111.344276843494));
#28591=CARTESIAN_POINT('Ctrl Pts',(2.09305320063531,2.25067335464529,111.339286815196));
#28592=CARTESIAN_POINT('Ctrl Pts',(2.16367582243927,2.18499660759582,111.334288364272));
#28593=CARTESIAN_POINT('Ctrl Pts',(2.23112314536882,2.11606810346765,111.329289913349));
#28594=CARTESIAN_POINT('Ctrl Pts',(2.29510062670075,2.04423955624526,111.324291462425));
#28595=CARTESIAN_POINT('Ctrl Pts',(2.34755265303044,1.98535082271439,111.32019347554));
#28596=CARTESIAN_POINT('Ctrl Pts',(2.39767308367136,1.92451353072959,111.316095488655));
#28597=CARTESIAN_POINT('Ctrl Pts',(2.44532132719983,1.86193605065848,111.31199750177));
#28598=CARTESIAN_POINT('Ctrl Pts',(2.50345178104249,1.7855920545846,111.306997992453));
#28599=CARTESIAN_POINT('Ctrl Pts',(2.55810567098051,1.70638906934886,111.301998483135));
#28600=CARTESIAN_POINT('Ctrl Pts',(2.60898960431686,1.6246770431586,111.296998973818));
#28601=CARTESIAN_POINT('Ctrl Pts',(2.65980451388741,1.54307585886654,111.292006246307));
#28602=CARTESIAN_POINT('Ctrl Pts',(2.70685940038884,1.45897276728328,111.287013518795));
#28603=CARTESIAN_POINT('Ctrl Pts',(2.7499019655331,1.37274958749117,111.282020791284));
#28604=CARTESIAN_POINT('Ctrl Pts',(2.79289912183065,1.28661737103132,111.277033330977));
#28605=CARTESIAN_POINT('Ctrl Pts',(2.83189217650519,1.19836990332672,111.27204587067));
#28606=CARTESIAN_POINT('Ctrl Pts',(2.86667344342633,1.10841581491526,111.267058410363));
#28607=CARTESIAN_POINT('Ctrl Pts',(2.90142982351349,1.01852609082005,111.262074518705));
#28608=CARTESIAN_POINT('Ctrl Pts',(2.93198024896046,0.926932581812277,111.257090627046));
#28609=CARTESIAN_POINT('Ctrl Pts',(2.9581645104515,0.834065332636013,111.252106735387));
#28610=CARTESIAN_POINT('Ctrl Pts',(2.98433923627205,0.741231903450742,111.24712465874));
#28611=CARTESIAN_POINT('Ctrl Pts',(3.0061508383937,0.647126077804854,111.242142582093));
#28612=CARTESIAN_POINT('Ctrl Pts',(3.02348878664653,0.552193631820106,111.237160505446));
#28613=CARTESIAN_POINT('Ctrl Pts',(3.04082515407159,0.45726984152198,111.232178883052));
#28614=CARTESIAN_POINT('Ctrl Pts',(3.05368859991533,0.36152001258511,111.227197260657));
#28615=CARTESIAN_POINT('Ctrl Pts',(3.06201980405686,0.26539964122729,111.222215638263));
#28616=CARTESIAN_POINT('Ctrl Pts',(3.07035252295555,0.169261793521756,111.217233110123));
#28617=CARTESIAN_POINT('Ctrl Pts',(3.07415132573822,0.0727537069176042,
111.212250581984));
#28618=CARTESIAN_POINT('Ctrl Pts',(3.07340888777848,-0.0236655556506188,
111.207268053844));
#28619=CARTESIAN_POINT('Ctrl Pts',(3.07266564958019,-0.1201887439533,111.202280155275));
#28620=CARTESIAN_POINT('Ctrl Pts',(3.06737140203435,-0.216622477408389,
111.197292256705));
#28621=CARTESIAN_POINT('Ctrl Pts',(3.0575709438332,-0.312509477339433,111.192304358135));
#28622=CARTESIAN_POINT('Ctrl Pts',(3.04776469636858,-0.408453119020665,
111.187313513147));
#28623=CARTESIAN_POINT('Ctrl Pts',(3.03344700313358,-0.503848950208386,
111.182322668158));
#28624=CARTESIAN_POINT('Ctrl Pts',(3.0147140412321,-0.598248693770405,111.177331823169));
#28625=CARTESIAN_POINT('Ctrl Pts',(2.99595080638871,-0.692800989714087,
111.172332912848));
#28626=CARTESIAN_POINT('Ctrl Pts',(2.97275816104351,-0.786353558033525,
111.167334002527));
#28627=CARTESIAN_POINT('Ctrl Pts',(2.94528248064981,-0.878472173251547,
111.162335092206));
#28628=CARTESIAN_POINT('Ctrl Pts',(2.92933120680081,-0.931952532495746,
111.159432926132));
#28629=CARTESIAN_POINT('Ctrl Pts',(2.91193725478093,-0.984949914274633,
111.156530760059));
#28630=CARTESIAN_POINT('Ctrl Pts',(2.89313660636581,-1.03738268103249,111.153628593986));
#28631=CARTESIAN_POINT('Ctrl Pts',(2.86074906560292,-1.12770767053203,111.148629084399));
#28632=CARTESIAN_POINT('Ctrl Pts',(2.82407060568943,-1.21667312579871,111.143629574812));
#28633=CARTESIAN_POINT('Ctrl Pts',(2.7832350224323,-1.30384242142457,111.138630065224));
#28634=CARTESIAN_POINT('Ctrl Pts',(2.74245483237396,-1.39089347247704,111.133637337439));
#28635=CARTESIAN_POINT('Ctrl Pts',(2.69752891095457,-1.47615281212287,111.128644609653));
#28636=CARTESIAN_POINT('Ctrl Pts',(2.6486401609382,-1.55920093248602,111.123651881868));
#28637=CARTESIAN_POINT('Ctrl Pts',(2.59980298730962,-1.64216143919449,111.118664421283));
#28638=CARTESIAN_POINT('Ctrl Pts',(2.54701151753359,-1.72291498777456,111.113676960698));
#28639=CARTESIAN_POINT('Ctrl Pts',(2.49049543277262,-1.80106489315036,111.108689500114));
#28640=CARTESIAN_POINT('Ctrl Pts',(2.43401978657781,-1.87915888046086,111.103705608173));
#28641=CARTESIAN_POINT('Ctrl Pts',(2.37382507988143,-1.95465257338061,111.098721716231));
#28642=CARTESIAN_POINT('Ctrl Pts',(2.31018480474021,-2.0271774510258,111.09373782429));
#28643=CARTESIAN_POINT('Ctrl Pts',(2.24656770580208,-2.09967591691695,111.088755747358));
#28644=CARTESIAN_POINT('Ctrl Pts',(2.17950782077992,-2.16920738609092,111.083773670426));
#28645=CARTESIAN_POINT('Ctrl Pts',(2.10931888497435,-2.2354364431785,111.078791593494));
#28646=CARTESIAN_POINT('Ctrl Pts',(2.03913634877496,-2.30165946170919,111.073809970812));
#28647=CARTESIAN_POINT('Ctrl Pts',(1.96582564840985,-2.36458036568008,111.06882834813));
#28648=CARTESIAN_POINT('Ctrl Pts',(1.88973655370966,-2.4239014021972,111.063846725449));
#28649=CARTESIAN_POINT('Ctrl Pts',(1.81363362466495,-2.48323322432898,111.05886419702));
#28650=CARTESIAN_POINT('Ctrl Pts',(1.7347516442379,-2.53896360926549,111.05388166859));
#28651=CARTESIAN_POINT('Ctrl Pts',(1.65347168301933,-2.59083647562968,111.048899140161));
#28652=CARTESIAN_POINT('Ctrl Pts',(1.57210411398258,-2.64276525329817,111.043911241301));
#28653=CARTESIAN_POINT('Ctrl Pts',(1.48833377474077,-2.69082797511479,111.038923342441));
#28654=CARTESIAN_POINT('Ctrl Pts',(1.40256861788299,-2.73481325178334,111.03393544358));
#28655=CARTESIAN_POINT('Ctrl Pts',(1.31675279836798,-2.77882451115953,111.0289445983));
#28656=CARTESIAN_POINT('Ctrl Pts',(1.22894021432322,-2.81875334785365,111.023953753019));
#28657=CARTESIAN_POINT('Ctrl Pts',(1.13955924096691,-2.85443636929025,111.018962907738));
#28658=CARTESIAN_POINT('Ctrl Pts',(1.05003382571607,-2.89017705538439,111.013963997126));
#28659=CARTESIAN_POINT('Ctrl Pts',(0.958935374812929,-2.92165808235672,
111.008965086514));
#28660=CARTESIAN_POINT('Ctrl Pts',(0.866707807624285,-2.94876581406579,
111.003966175903));
#28661=CARTESIAN_POINT('Ctrl Pts',(0.813164250758867,-2.96450345540776,
111.001064012669));
#28662=CARTESIAN_POINT('Ctrl Pts',(0.759240344083131,-2.97876803448073,
110.998161849435));
#28663=CARTESIAN_POINT('Ctrl Pts',(0.705024154617008,-2.99154528486643,
110.995259686202));
#28664=CARTESIAN_POINT('Ctrl Pts',(0.611626805219617,-3.01355644666815,
110.990260176716));
#28665=CARTESIAN_POINT('Ctrl Pts',(0.517033625005757,-3.03122821826157,
110.98526066723));
#28666=CARTESIAN_POINT('Ctrl Pts',(0.421683697314452,-3.04443510514171,
110.980261157744));
#28667=CARTESIAN_POINT('Ctrl Pts',(0.326463111192108,-3.057624076964,110.975268430061));
#28668=CARTESIAN_POINT('Ctrl Pts',(0.23048824883096,-3.06636014142969,110.970275702377));
#28669=CARTESIAN_POINT('Ctrl Pts',(0.134210571877783,-3.070568314237,110.965282974694));
#28670=CARTESIAN_POINT('Ctrl Pts',(0.0380344654444882,-3.07477204752818,
110.960295514213));
#28671=CARTESIAN_POINT('Ctrl Pts',(-0.058443384298457,-3.07445736610732,
110.955308053731));
#28672=CARTESIAN_POINT('Ctrl Pts',(-0.154765190719179,-3.06960094894135,
110.95032059325));
#28673=CARTESIAN_POINT('Ctrl Pts',(-0.25101807664028,-3.06474800665516,
110.945336701412));
#28674=CARTESIAN_POINT('Ctrl Pts',(-0.347114704050907,-3.05535981094989,
110.940352809575));
#28675=CARTESIAN_POINT('Ctrl Pts',(-0.442597057314949,-3.04146512307081,
110.935368917738));
#28676=CARTESIAN_POINT('Ctrl Pts',(-0.538044638273774,-3.02757549529249,
110.930386840911));
#28677=CARTESIAN_POINT('Ctrl Pts',(-0.632877955617285,-3.00918269928038,
110.925404764083));
#28678=CARTESIAN_POINT('Ctrl Pts',(-0.726644851861425,-2.98636727635154,
110.920422687256));
#28679=CARTESIAN_POINT('Ctrl Pts',(-0.820403198727854,-2.9635539336629,
110.915441064679));
#28680=CARTESIAN_POINT('Ctrl Pts',(-0.913094891337656,-2.93631886973509,
110.910459442102));
#28681=CARTESIAN_POINT('Ctrl Pts',(-1.00427974414338,-2.90479335676452,
110.905477819525));
#28682=CARTESIAN_POINT('Ctrl Pts',(-1.09548117596486,-2.87326211189924,
110.900495291201));
#28683=CARTESIAN_POINT('Ctrl Pts',(-1.18517480902578,-2.83743901221733,
110.895512762877));
#28684=CARTESIAN_POINT('Ctrl Pts',(-1.27293836977718,-2.79750427287413,
110.890530234554));
#28685=CARTESIAN_POINT('Ctrl Pts',(-1.36079652671805,-2.75752648976496,
110.885542335798));
#28686=CARTESIAN_POINT('Ctrl Pts',(-1.44672005794881,-2.71342840153585,
110.880554437043));
#28687=CARTESIAN_POINT('Ctrl Pts',(-1.53030954134675,-2.6654371044283,110.875566538287));
#28688=CARTESIAN_POINT('Ctrl Pts',(-1.6139484022026,-2.61741745820125,110.870575693112));
#28689=CARTESIAN_POINT('Ctrl Pts',(-1.69525010010885,-2.56550026001342,
110.865584847936));
#28690=CARTESIAN_POINT('Ctrl Pts',(-1.77384435308946,-2.50995586833965,
110.86059400276));
#28691=CARTESIAN_POINT('Ctrl Pts',(-1.8525656163727,-2.45432171552269,110.855595092252));
#28692=CARTESIAN_POINT('Ctrl Pts',(-1.92857035231037,-2.39504893459013,
110.850596181744));
#28693=CARTESIAN_POINT('Ctrl Pts',(-2.0015215512034,-2.33244801229702,110.845597271236));
#28694=CARTESIAN_POINT('Ctrl Pts',(-2.04387405236461,-2.29610446106903,
110.842695106963));
#28695=CARTESIAN_POINT('Ctrl Pts',(-2.08519804158071,-2.25863986348709,
110.839792942691));
#28696=CARTESIAN_POINT('Ctrl Pts',(-2.12543360399879,-2.22012032218812,
110.836890778418));
#28697=CARTESIAN_POINT('Ctrl Pts',(-2.1937352854616,-2.15473166395198,110.831964223703));
#28698=CARTESIAN_POINT('Ctrl Pts',(-2.25915360617813,-2.08605668722672,
110.827037668989));
#28699=CARTESIAN_POINT('Ctrl Pts',(-2.32134887028838,-2.01438369542916,
110.822111114274));
#28700=CARTESIAN_POINT('Ctrl Pts',(-2.38344339011673,-1.94282679999672,
110.817192539624));
#28701=CARTESIAN_POINT('Ctrl Pts',(-2.44232493870375,-1.86828188317021,
110.812273964974));
#28702=CARTESIAN_POINT('Ctrl Pts',(-2.49768920318606,-1.79107534578749,
110.807355390324));
#28703=CARTESIAN_POINT('Ctrl Pts',(-2.55300266298286,-1.71393965652111,
110.802441329175));
#28704=CARTESIAN_POINT('Ctrl Pts',(-2.60480498295285,-1.63414756060737,
110.797527268025));
#28705=CARTESIAN_POINT('Ctrl Pts',(-2.65283131018544,-1.55205937054606,
110.792613206876));
#28706=CARTESIAN_POINT('Ctrl Pts',(-2.70082759207679,-1.47002253497767,
110.78770221997));
#28707=CARTESIAN_POINT('Ctrl Pts',(-2.74505234385498,-1.38569284746465,
110.782791233065));
#28708=CARTESIAN_POINT('Ctrl Pts',(-2.78528406969069,-1.29945946498045,
110.777880246159));
#28709=CARTESIAN_POINT('Ctrl Pts',(-2.82550237202281,-1.21325485466784,
110.772970897827));
#28710=CARTESIAN_POINT('Ctrl Pts',(-2.86173010459517,-1.12514822177586,
110.768061549496));
#28711=CARTESIAN_POINT('Ctrl Pts',(-2.89379235729422,-1.03555204739578,
110.763152201164));
#28712=CARTESIAN_POINT('Ctrl Pts',(-2.92586678026355,-0.945921863875121,
110.758240989329));
#28713=CARTESIAN_POINT('Ctrl Pts',(-2.95377240523807,-0.854801434026095,
110.753329777495));
#28714=CARTESIAN_POINT('Ctrl Pts',(-2.97738326655227,-0.76262122580908,
110.74841856566));
#28715=CARTESIAN_POINT('Ctrl Pts',(-3.00099833095211,-0.670424608139487,
110.743506479557));
#28716=CARTESIAN_POINT('Ctrl Pts',(-3.0203170106075,-0.577168279053442,
110.738594393453));
#28717=CARTESIAN_POINT('Ctrl Pts',(-3.03526427861237,-0.483293915728025,
110.733682307349));
#28718=CARTESIAN_POINT('Ctrl Pts',(-3.05022812720535,-0.389315420185806,
110.728764772406));
#28719=CARTESIAN_POINT('Ctrl Pts',(-3.06081082419188,-0.294717971407319,
110.723847237462));
#28720=CARTESIAN_POINT('Ctrl Pts',(-3.06698918420348,-0.199948978439139,
110.718929702518));
#28721=CARTESIAN_POINT('Ctrl Pts',(-3.07138918192552,-0.132458033852455,
110.715427617416));
#28722=CARTESIAN_POINT('Ctrl Pts',(-3.07355650191939,-0.0648801894581821,
110.711925532314));
#28723=CARTESIAN_POINT('Ctrl Pts',(-3.07349888025591,0.00262355973275451,
110.708423447212));
#28724=CARTESIAN_POINT('Ctrl Pts',(-3.07349888025533,0.00262356040959872,
110.708423447177));
#28725=CARTESIAN_POINT('Ctrl Pts',(-3.07337791850908,0.144330147494426,
110.701071729185));
#28726=CARTESIAN_POINT('Ctrl Pts',(-3.06345337427643,0.285630529407084,
110.693720011193));
#28727=CARTESIAN_POINT('Ctrl Pts',(-3.04391216934768,0.425442070436255,
110.6863682932));
#28728=CARTESIAN_POINT('Ctrl Pts',(-3.0369601185254,0.475181937671709,110.683752819011));
#28729=CARTESIAN_POINT('Ctrl Pts',(-3.02879130436724,0.524733671575758,
110.681137344822));
#28730=CARTESIAN_POINT('Ctrl Pts',(-3.01941544185788,0.574049335397397,
110.678521870633));
#28731=CARTESIAN_POINT('Ctrl Pts',(-3.00149337100039,0.668316803645044,
110.673522361128));
#28732=CARTESIAN_POINT('Ctrl Pts',(-2.97912098278221,0.761909739136843,
110.668522851622));
#28733=CARTESIAN_POINT('Ctrl Pts',(-2.95236242568487,0.854376004698248,
110.663523342116));
#28734=CARTESIAN_POINT('Ctrl Pts',(-2.9256401663993,0.946716840361099,110.658530614413));
#28735=CARTESIAN_POINT('Ctrl Pts',(-2.89454368406788,1.03793362547514,110.653537886709));
#28736=CARTESIAN_POINT('Ctrl Pts',(-2.85918830111607,1.12758348194758,110.648545159006));
#28737=CARTESIAN_POINT('Ctrl Pts',(-2.82387021720086,1.21713876008429,110.643557698505));
#28738=CARTESIAN_POINT('Ctrl Pts',(-2.78430232472978,1.30512998960044,110.638570238003));
#28739=CARTESIAN_POINT('Ctrl Pts',(-2.74064970866011,1.39112954983397,110.633582777502));
#28740=CARTESIAN_POINT('Ctrl Pts',(-2.69702832705611,1.47706757537488,110.628598885645));
#28741=CARTESIAN_POINT('Ctrl Pts',(-2.64932823018674,1.56101637433474,110.623614993787));
#28742=CARTESIAN_POINT('Ctrl Pts',(-2.59776216630118,1.64256932192654,110.61863110193));
#28743=CARTESIAN_POINT('Ctrl Pts',(-2.54621488149783,1.72409256995641,110.613649025083));
#28744=CARTESIAN_POINT('Ctrl Pts',(-2.49080466135627,1.80322132956271,110.608666948236));
#28745=CARTESIAN_POINT('Ctrl Pts',(-2.4317891630379,1.87957540857807,110.603684871389));
#28746=CARTESIAN_POINT('Ctrl Pts',(-2.37277904557233,1.95592252586183,110.598703248792));
#28747=CARTESIAN_POINT('Ctrl Pts',(-2.31016457207171,2.02949511833949,110.593721626195));
#28748=CARTESIAN_POINT('Ctrl Pts',(-2.24424486111886,2.09994458339777,110.588740003598));
#28749=CARTESIAN_POINT('Ctrl Pts',(-2.17831316480023,2.17040685741097,110.583757475255));
#28750=CARTESIAN_POINT('Ctrl Pts',(-2.10907533748121,2.23774455577521,110.578774946911));
#28751=CARTESIAN_POINT('Ctrl Pts',(-2.03686790767812,2.3016453629243,110.573792418568));
#28752=CARTESIAN_POINT('Ctrl Pts',(-1.96458264890743,2.36561504572598,110.568804519793));
#28753=CARTESIAN_POINT('Ctrl Pts',(-1.88932172683329,2.42614015030467,110.563816621018));
#28754=CARTESIAN_POINT('Ctrl Pts',(-1.81145518560296,2.48294832015331,110.558828722244));
#28755=CARTESIAN_POINT('Ctrl Pts',(-1.73354264753758,2.53979004736788,110.553837877048));
#28756=CARTESIAN_POINT('Ctrl Pts',(-1.65302179180727,2.59291022635424,110.548847031853));
#28757=CARTESIAN_POINT('Ctrl Pts',(-1.57029031244102,2.64208073015453,110.543856186658));
#28758=CARTESIAN_POINT('Ctrl Pts',(-1.48742513691665,2.69133069472962,110.538857276131));
#28759=CARTESIAN_POINT('Ctrl Pts',(-1.40234259164468,2.73661803301578,110.533858365605));
#28760=CARTESIAN_POINT('Ctrl Pts',(-1.31546347572111,2.77776134576816,110.528859455078));
#28761=CARTESIAN_POINT('Ctrl Pts',(-1.26502499560561,2.80164747927776,110.525957291002));
#28762=CARTESIAN_POINT('Ctrl Pts',(-1.21398134620056,2.82413777925323,110.523055126925));
#28763=CARTESIAN_POINT('Ctrl Pts',(-1.16241729725908,2.84520443501568,110.520152962849));
#28764=CARTESIAN_POINT('Ctrl Pts',(-1.07358877298922,2.88149561038098,110.515153453358));
#28765=CARTESIAN_POINT('Ctrl Pts',(-0.982903059359573,2.91368664349634,
110.510153943867));
#28766=CARTESIAN_POINT('Ctrl Pts',(-0.890774331281627,2.94158517482152,
110.505154434376));
#28767=CARTESIAN_POINT('Ctrl Pts',(-0.798770575238357,2.9694458619661,110.500161706688));
#28768=CARTESIAN_POINT('Ctrl Pts',(-0.705328111557418,2.99302549351996,
110.495168979));
#28769=CARTESIAN_POINT('Ctrl Pts',(-0.61088121043788,3.01217967537362,110.490176251312));
#28770=CARTESIAN_POINT('Ctrl Pts',(-0.516533948418184,3.03131365004827,
110.485188790825));
#28771=CARTESIAN_POINT('Ctrl Pts',(-0.421184783409245,3.04603136940846,
110.480201330339));
#28772=CARTESIAN_POINT('Ctrl Pts',(-0.32528228108335,3.0562384867044,110.475213869853));
#28773=CARTESIAN_POINT('Ctrl Pts',(-0.229448399239483,3.06643830056934,
110.470229978011));
#28774=CARTESIAN_POINT('Ctrl Pts',(-0.133062402405853,3.07213388204652,
110.465246086169));
#28775=CARTESIAN_POINT('Ctrl Pts',(-0.0365811954306498,3.07328229522458,
110.460262194327));
#28776=CARTESIAN_POINT('Ctrl Pts',(0.0598648754787269,3.07443029017901,
110.455280117496));
#28777=CARTESIAN_POINT('Ctrl Pts',(0.156405649155184,3.07103440183982,110.450298040664));
#28778=CARTESIAN_POINT('Ctrl Pts',(0.252581941500445,3.06310375482579,110.445315963832));
#28779=CARTESIAN_POINT('Ctrl Pts',(0.348749464783802,3.05517383090404,110.440334341251));
#28780=CARTESIAN_POINT('Ctrl Pts',(0.444552135345558,3.04271000661028,110.43535271867));
#28781=CARTESIAN_POINT('Ctrl Pts',(0.539534692425912,3.0257733830657,110.430371096089));
#28782=CARTESIAN_POINT('Ctrl Pts',(0.634534519008938,3.00883368014451,110.425388567761));
#28783=CARTESIAN_POINT('Ctrl Pts',(0.728713503840477,2.98741963998045,110.420406039433));
#28784=CARTESIAN_POINT('Ctrl Pts',(0.821626455559054,2.96164349939784,110.415423511105));
#28785=CARTESIAN_POINT('Ctrl Pts',(0.914639553746905,2.93583957593433,110.410435612346));
#28786=CARTESIAN_POINT('Ctrl Pts',(1.00638347084152,2.9056642830803,110.405447713587));
#28787=CARTESIAN_POINT('Ctrl Pts',(1.09642828519429,2.87127972608485,110.400459814827));
#28788=CARTESIAN_POINT('Ctrl Pts',(1.18652629025516,2.8368748576595,110.395468969648));
#28789=CARTESIAN_POINT('Ctrl Pts',(1.27492279201485,2.79825594977819,110.390478124468));
#28790=CARTESIAN_POINT('Ctrl Pts',(1.36120991420809,2.75563238104462,110.385487279289));
#28791=CARTESIAN_POINT('Ctrl Pts',(1.4476364785706,2.7129399315472,110.380488368778));
#28792=CARTESIAN_POINT('Ctrl Pts',(1.53194647301246,2.66623011136276,110.375489458266));
#28793=CARTESIAN_POINT('Ctrl Pts',(1.61375863652375,2.61575712042326,110.370490547755));
#28794=CARTESIAN_POINT('Ctrl Pts',(1.66125545287571,2.58645455368383,110.367588383525));
#28795=CARTESIAN_POINT('Ctrl Pts',(1.70791094010491,2.55588441173041,110.364686219295));
#28796=CARTESIAN_POINT('Ctrl Pts',(1.75365561779286,2.5241026572197,110.361784055065));
#28797=CARTESIAN_POINT('Ctrl Pts',(1.79388071499675,2.49615570843531,110.359232067727));
#28798=CARTESIAN_POINT('Ctrl Pts',(1.83347357344082,2.46722195299097,110.356680080389));
#28799=CARTESIAN_POINT('Ctrl Pts',(1.8723819390353,2.43733217358127,110.35412809305));
#28800=CARTESIAN_POINT('',(-3.07349876323956,-0.0027572386409777,110.791576552868));
#28801=CARTESIAN_POINT('Ctrl Pts',(-3.07349876324033,-0.00275723777476568,
110.791576552823));
#28802=CARTESIAN_POINT('Ctrl Pts',(-3.07358427951016,0.0925679285798107,
110.786643375934));
#28803=CARTESIAN_POINT('Ctrl Pts',(-3.06923075828948,0.187999943733393,
110.781710199046));
#28804=CARTESIAN_POINT('Ctrl Pts',(-3.06043513424029,0.283088394512365,
110.776777022157));
#28805=CARTESIAN_POINT('Ctrl Pts',(-3.05164431928817,0.378124854712078,
110.771846542533));
#28806=CARTESIAN_POINT('Ctrl Pts',(-3.03841626490044,0.472817677209372,
110.766916062909));
#28807=CARTESIAN_POINT('Ctrl Pts',(-3.02079995318321,0.566718530531958,
110.761985583285));
#28808=CARTESIAN_POINT('Ctrl Pts',(-3.00318821239493,0.660595019269262,
110.757056382979));
#28809=CARTESIAN_POINT('Ctrl Pts',(-2.98119055870853,0.753679505664892,
110.752127182674));
#28810=CARTESIAN_POINT('Ctrl Pts',(-2.9549074089867,0.845532053984643,110.747197982368));
#28811=CARTESIAN_POINT('Ctrl Pts',(-2.92862352816746,0.93738715729349,110.742268644951));
#28812=CARTESIAN_POINT('Ctrl Pts',(-2.8980540394572,1.02800982286176,110.737339307534));
#28813=CARTESIAN_POINT('Ctrl Pts',(-2.8633493971494,1.11697469973324,110.732409970117));
#28814=CARTESIAN_POINT('Ctrl Pts',(-2.82861089080364,1.20602638660381,110.727475822759));
#28815=CARTESIAN_POINT('Ctrl Pts',(-2.78972933545781,1.29341663443531,110.722541675401));
#28816=CARTESIAN_POINT('Ctrl Pts',(-2.74690347158547,1.37873984775652,110.717607528043));
#28817=CARTESIAN_POINT('Ctrl Pts',(-2.70405712231737,1.46410387472712,110.712671020477));
#28818=CARTESIAN_POINT('Ctrl Pts',(-2.65726292856968,1.54739850686877,110.707734512911));
#28819=CARTESIAN_POINT('Ctrl Pts',(-2.60676464434538,1.62824455748849,110.702798005345));
#28820=CARTESIAN_POINT('Ctrl Pts',(-2.55617956998138,1.70922955619597,110.697853013526));
#28821=CARTESIAN_POINT('Ctrl Pts',(-2.50187794378262,1.78775719671831,110.692908021708));
#28822=CARTESIAN_POINT('Ctrl Pts',(-2.44414575109866,1.86347895007869,110.687963029889));
#28823=CARTESIAN_POINT('Ctrl Pts',(-2.39079118008633,1.93345899897378,110.68339299877));
#28824=CARTESIAN_POINT('Ctrl Pts',(-2.33450720666026,2.001042708641,110.678822967651));
#28825=CARTESIAN_POINT('Ctrl Pts',(-2.2755471967709,2.06598335067544,110.674252936532));
#28826=CARTESIAN_POINT('Ctrl Pts',(-2.21104629490347,2.13702692727814,110.669253427046));
#28827=CARTESIAN_POINT('Ctrl Pts',(-2.1431018958045,2.20517177216898,110.66425391756));
#28828=CARTESIAN_POINT('Ctrl Pts',(-2.07200476361226,2.27006575005398,110.659254408074));
#28829=CARTESIAN_POINT('Ctrl Pts',(-2.00100407422677,2.33487169967151,110.654261680391));
#28830=CARTESIAN_POINT('Ctrl Pts',(-1.92685947277257,2.39643525303404,110.649268952708));
#28831=CARTESIAN_POINT('Ctrl Pts',(-1.84990053545108,2.45443888881712,110.644276225025));
#28832=CARTESIAN_POINT('Ctrl Pts',(-1.77302278786648,2.51238133222811,110.639288764543));
#28833=CARTESIAN_POINT('Ctrl Pts',(-1.69333695539624,2.56677106121078,110.634301304062));
#28834=CARTESIAN_POINT('Ctrl Pts',(-1.61120709089405,2.61732954750691,110.62931384358));
#28835=CARTESIAN_POINT('Ctrl Pts',(-1.52913599222579,2.6678518580267,110.624329951743));
#28836=CARTESIAN_POINT('Ctrl Pts',(-1.44462471072116,2.7145481460659,110.619346059906));
#28837=CARTESIAN_POINT('Ctrl Pts',(-1.35806698952089,2.75718267475582,110.614362168069));
#28838=CARTESIAN_POINT('Ctrl Pts',(-1.27154079049631,2.7998016770076,110.609380091241));
#28839=CARTESIAN_POINT('Ctrl Pts',(-1.18297002591487,2.83836166514092,110.604398014414));
#28840=CARTESIAN_POINT('Ctrl Pts',(-1.09277294158465,2.87267289264553,110.599415937587));
#28841=CARTESIAN_POINT('Ctrl Pts',(-1.00258408114756,2.9069809917578,110.59443431501));
#28842=CARTESIAN_POINT('Ctrl Pts',(-0.910769606120397,2.93704094454205,
110.589452692433));
#28843=CARTESIAN_POINT('Ctrl Pts',(-0.817766632290743,2.96271159330635,
110.584471069856));
#28844=CARTESIAN_POINT('Ctrl Pts',(-0.724746748878659,2.98838690944777,
110.579488541532));
#28845=CARTESIAN_POINT('Ctrl Pts',(-0.630538360653306,3.00967121987548,
110.574506013208));
#28846=CARTESIAN_POINT('Ctrl Pts',(-0.535591545412797,3.02647384698469,
110.569523484885));
#28847=CARTESIAN_POINT('Ctrl Pts',(-0.440542391492857,3.0432945848506,110.564535586129));
#28848=CARTESIAN_POINT('Ctrl Pts',(-0.344753654548596,3.05562391894161,
110.559547687374));
#28849=CARTESIAN_POINT('Ctrl Pts',(-0.248683135866333,3.06342275044364,
110.554559788619));
#28850=CARTESIAN_POINT('Ctrl Pts',(-0.152555867006806,3.07122618882275,
110.549568943443));
#28851=CARTESIAN_POINT('Ctrl Pts',(-0.0561469234809696,3.07449378093882,
110.544578098267));
#28852=CARTESIAN_POINT('Ctrl Pts',(0.0400854023518479,3.07323858665713,
110.539587253091));
#28853=CARTESIAN_POINT('Ctrl Pts',(0.136473242059387,3.07198136394969,110.534588342584));
#28854=CARTESIAN_POINT('Ctrl Pts',(0.232683456282823,3.06618678688432,110.529589432076));
#28855=CARTESIAN_POINT('Ctrl Pts',(0.328262442087564,3.05591983191881,110.524590521568));
#28856=CARTESIAN_POINT('Ctrl Pts',(0.383751716687541,3.04995925513941,110.521688357295));
#28857=CARTESIAN_POINT('Ctrl Pts',(0.439028399776211,3.04249223002058,110.518786193021));
#28858=CARTESIAN_POINT('Ctrl Pts',(0.494005672129351,3.03353929361464,110.515884028748));
#28859=CARTESIAN_POINT('Ctrl Pts',(0.588714582648808,3.01811614116157,110.5108844934));
#28860=CARTESIAN_POINT('Ctrl Pts',(0.682866871070267,2.99822634453998,110.505884958052));
#28861=CARTESIAN_POINT('Ctrl Pts',(0.776008855003659,2.97392207479549,110.500885422704));
#28862=CARTESIAN_POINT('Ctrl Pts',(0.869028892685815,2.94964962544455,110.495892433004));
#28863=CARTESIAN_POINT('Ctrl Pts',(0.961040833031793,2.92097429707105,110.490899443303));
#28864=CARTESIAN_POINT('Ctrl Pts',(1.05159883344927,2.88799967858172,110.485906453603));
#28865=CARTESIAN_POINT('Ctrl Pts',(1.14204898499438,2.85506433078527,110.480919410238));
#28866=CARTESIAN_POINT('Ctrl Pts',(1.23104823087104,2.81784002774614,110.475932366874));
#28867=CARTESIAN_POINT('Ctrl Pts',(1.31816484313995,2.77648045127457,110.47094532351));
#28868=CARTESIAN_POINT('Ctrl Pts',(1.40522191994573,2.73514913992345,110.465961688289));
#28869=CARTESIAN_POINT('Ctrl Pts',(1.4903985248001,2.68968835917862,110.460978053068));
#28870=CARTESIAN_POINT('Ctrl Pts',(1.57328261187453,2.64029999681348,110.455994417848));
#28871=CARTESIAN_POINT('Ctrl Pts',(1.65613361834081,2.59093134627868,110.45101277169));
#28872=CARTESIAN_POINT('Ctrl Pts',(1.73669354957927,2.53763845506773,110.446031125533));
#28873=CARTESIAN_POINT('Ctrl Pts',(1.8145756300531,2.48066876725157,110.441049479375));
#28874=CARTESIAN_POINT('Ctrl Pts',(1.83401296871451,2.46645061708428,110.439806190253));
#28875=CARTESIAN_POINT('Ctrl Pts',(1.85328364809906,2.45200366374706,110.438562901131));
#28876=CARTESIAN_POINT('Ctrl Pts',(1.8723819390353,2.43733217358127,110.437319612009));
#28877=CARTESIAN_POINT('Ctrl Pts',(1.87238193903529,2.43733217358128,111.437229631665));
#28878=CARTESIAN_POINT('Ctrl Pts',(1.94871667497837,2.3786910977156,111.432241834346));
#28879=CARTESIAN_POINT('Ctrl Pts',(2.02237837223609,2.31639560571599,111.427254037028));
#28880=CARTESIAN_POINT('Ctrl Pts',(2.09300115674764,2.25072175265026,111.42226623971));
#28881=CARTESIAN_POINT('Ctrl Pts',(2.16357129200264,2.18509685941473,111.417282160793));
#28882=CARTESIAN_POINT('Ctrl Pts',(2.23110669796282,2.11609891015331,111.412298081876));
#28883=CARTESIAN_POINT('Ctrl Pts',(2.29527476119916,2.04404403587647,111.407314002958));
#28884=CARTESIAN_POINT('Ctrl Pts',(2.35941815820086,1.97201685952826,111.402331839923));
#28885=CARTESIAN_POINT('Ctrl Pts',(2.42019649266593,1.89693542031554,111.397349676888));
#28886=CARTESIAN_POINT('Ctrl Pts',(2.47731487587539,1.8191517956912,111.392367513854));
#28887=CARTESIAN_POINT('Ctrl Pts',(2.53442689601226,1.74137683627798,111.387385905839));
#28888=CARTESIAN_POINT('Ctrl Pts',(2.58787951574812,1.66090064377156,111.382404297824));
#28889=CARTESIAN_POINT('Ctrl Pts',(2.63741958716114,1.57810651454797,111.37742268981));
#28890=CARTESIAN_POINT('Ctrl Pts',(2.68696766394427,1.49529900630356,111.372440276798));
#28891=CARTESIAN_POINT('Ctrl Pts',(2.73260171149074,1.41017319421669,111.367457863786));
#28892=CARTESIAN_POINT('Ctrl Pts',(2.77411373158308,1.32313841084076,111.362475450775));
#28893=CARTESIAN_POINT('Ctrl Pts',(2.81567003196019,1.23601078869223,111.357487723093));
#28894=CARTESIAN_POINT('Ctrl Pts',(2.85309533663416,1.14697052651153,111.352499995412));
#28895=CARTESIAN_POINT('Ctrl Pts',(2.88622925913025,1.05644825417076,111.347512267731));
#28896=CARTESIAN_POINT('Ctrl Pts',(2.91938215337648,0.965874150781834,111.342521684187));
#28897=CARTESIAN_POINT('Ctrl Pts',(2.94823864118371,0.873816766246551,111.337531100644));
#28898=CARTESIAN_POINT('Ctrl Pts',(2.9726884541713,0.780721207881932,111.3325405171));
#28899=CARTESIAN_POINT('Ctrl Pts',(2.99717831341183,0.687473168666888,111.327541759499));
#28900=CARTESIAN_POINT('Ctrl Pts',(3.01724699218182,0.593183989036835,111.322543001898));
#28901=CARTESIAN_POINT('Ctrl Pts',(3.03283549421489,0.498308253022458,111.317544244298));
#28902=CARTESIAN_POINT('Ctrl Pts',(3.04303880920497,0.436208186100302,111.314272352088));
#28903=CARTESIAN_POINT('Ctrl Pts',(3.05132377438297,0.373856959073547,111.311000459879));
#28904=CARTESIAN_POINT('Ctrl Pts',(3.05768593427511,0.31138236516561,111.307728567669));
#28905=CARTESIAN_POINT('Ctrl Pts',(3.06740742905065,0.21592006170639,111.302729057509));
#28906=CARTESIAN_POINT('Ctrl Pts',(3.07267115116372,0.119834385611258,111.297729547349));
#28907=CARTESIAN_POINT('Ctrl Pts',(3.07340956853436,0.0235769811771108,
111.292730037189));
#28908=CARTESIAN_POINT('Ctrl Pts',(3.0741469842478,-0.0725498508641107,
111.287737308824));
#28909=CARTESIAN_POINT('Ctrl Pts',(3.07037129182113,-0.168847513080869,
111.282744580459));
#28910=CARTESIAN_POINT('Ctrl Pts',(3.06206664760734,-0.264858633256908,
111.277751852094));
#28911=CARTESIAN_POINT('Ctrl Pts',(3.05377076457157,-0.360768464263453,
111.272764390924));
#28912=CARTESIAN_POINT('Ctrl Pts',(3.04095546559796,-0.45639191916809,111.267776929754));
#28913=CARTESIAN_POINT('Ctrl Pts',(3.0236569543179,-0.551272049540874,111.262789468585));
#28914=CARTESIAN_POINT('Ctrl Pts',(3.00637082050063,-0.646084291107248,
111.257805576052));
#28915=CARTESIAN_POINT('Ctrl Pts',(2.98460792991186,-0.740153834858849,
111.25282168352));
#28916=CARTESIAN_POINT('Ctrl Pts',(2.95845615891374,-0.833030255023996,
111.247837790988));
#28917=CARTESIAN_POINT('Ctrl Pts',(2.93231391171984,-0.925872851979168,
111.242855713461));
#28918=CARTESIAN_POINT('Ctrl Pts',(2.90178607865338,-1.01752276656253,111.237873635935));
#28919=CARTESIAN_POINT('Ctrl Pts',(2.86701112026954,-1.10754209231559,111.232891558408));
#28920=CARTESIAN_POINT('Ctrl Pts',(2.8322393325373,-1.19755321044073,111.227909935129));
#28921=CARTESIAN_POINT('Ctrl Pts',(2.79322134773867,-1.28593362591614,111.22292831185));
#28922=CARTESIAN_POINT('Ctrl Pts',(2.75014437794742,-1.37226387784718,111.217946688571));
#28923=CARTESIAN_POINT('Ctrl Pts',(2.70705957598402,-1.4586098261793,111.212964159542));
#28924=CARTESIAN_POINT('Ctrl Pts',(2.6599145193837,-1.54290447791132,111.207981630514));
#28925=CARTESIAN_POINT('Ctrl Pts',(2.60894262908064,-1.62475247596851,111.202999101486));
#28926=CARTESIAN_POINT('Ctrl Pts',(2.55791579860506,-1.70668869408397,111.198011202027));
#28927=CARTESIAN_POINT('Ctrl Pts',(2.50305413215539,-1.78617262050403,111.193023302568));
#28928=CARTESIAN_POINT('Ctrl Pts',(2.4446345749057,-1.86283763253152,111.188035403109));
#28929=CARTESIAN_POINT('Ctrl Pts',(2.38618050841788,-1.93954793163889,111.183044557229));
#28930=CARTESIAN_POINT('Ctrl Pts',(2.32416464838364,-2.0134356646547,111.178053711348));
#28931=CARTESIAN_POINT('Ctrl Pts',(2.25890306088313,-2.08416870994956,111.173062865468));
#28932=CARTESIAN_POINT('Ctrl Pts',(2.19353600909908,-2.15501606153439,111.168063954262));
#28933=CARTESIAN_POINT('Ctrl Pts',(2.12491306871472,-2.22269823768194,111.163065043056));
#28934=CARTESIAN_POINT('Ctrl Pts',(2.05338578367992,-2.28692130896128,111.15806613185));
#28935=CARTESIAN_POINT('Ctrl Pts',(2.01186005429569,-2.32420651944946,111.155163974528));
#28936=CARTESIAN_POINT('Ctrl Pts',(1.96935602978709,-2.36032661270555,111.152261817207));
#28937=CARTESIAN_POINT('Ctrl Pts',(1.92594701958487,-2.39523074624391,111.149359659885));
#28938=CARTESIAN_POINT('Ctrl Pts',(1.85116686987237,-2.45535965310967,111.144360150382));
#28939=CARTESIAN_POINT('Ctrl Pts',(1.77343679923049,-2.51208881208536,111.13936064088));
#28940=CARTESIAN_POINT('Ctrl Pts',(1.69309887531852,-2.56511567933985,111.134361131377));
#28941=CARTESIAN_POINT('Ctrl Pts',(1.61286992925858,-2.6180706160065,111.129368403676));
#28942=CARTESIAN_POINT('Ctrl Pts',(1.53004052376622,-2.66733300236767,111.124375675974));
#28943=CARTESIAN_POINT('Ctrl Pts',(1.44498567289287,-2.71264053186823,111.119382948272));
#28944=CARTESIAN_POINT('Ctrl Pts',(1.36002055271011,-2.75790026308486,111.114395487771));
#28945=CARTESIAN_POINT('Ctrl Pts',(1.27283503977061,-2.79921322638924,111.109408027269));
#28946=CARTESIAN_POINT('Ctrl Pts',(1.18383212988815,-2.83636100280703,111.104420566767));
#28947=CARTESIAN_POINT('Ctrl Pts',(1.09489290361739,-2.87348219914364,111.099436674907));
#28948=CARTESIAN_POINT('Ctrl Pts',(1.00413926944769,-2.90644396466975,111.094452783047));
#28949=CARTESIAN_POINT('Ctrl Pts',(0.911996885344304,-2.93507477436645,
111.089468891187));
#28950=CARTESIAN_POINT('Ctrl Pts',(0.819888057182536,-2.96369515744149,
111.084486814336));
#28951=CARTESIAN_POINT('Ctrl Pts',(0.726391902716913,-2.98798758834278,
111.079504737484));
#28952=CARTESIAN_POINT('Ctrl Pts',(0.631951119459168,-3.00782978783945,
111.074522660632));
#28953=CARTESIAN_POINT('Ctrl Pts',(0.537518946992066,-3.02767017819159,
111.069541038029));
#28954=CARTESIAN_POINT('Ctrl Pts',(0.442142746592162,-3.04306105378232,
111.064559415426));
#28955=CARTESIAN_POINT('Ctrl Pts',(0.346276286620338,-3.05393107049331,
111.059577792823));
#28956=CARTESIAN_POINT('Ctrl Pts',(0.250392396404009,-3.0648030635686,111.054595264472));
#28957=CARTESIAN_POINT('Ctrl Pts',(0.154018505754517,-3.07115251590384,
111.049612736121));
#28958=CARTESIAN_POINT('Ctrl Pts',(0.0576133234244592,-3.07295996637834,
111.044630207769));
#28959=CARTESIAN_POINT('Ctrl Pts',(-0.0388957695325551,-3.07476936501899,
111.039642308984));
#28960=CARTESIAN_POINT('Ctrl Pts',(-0.135435781891717,-3.07202697992187,
111.034654410199));
#28961=CARTESIAN_POINT('Ctrl Pts',(-0.23154841023164,-3.0647655022398,111.029666511414));
#28962=CARTESIAN_POINT('Ctrl Pts',(-0.327717813648208,-3.05749973510109,
111.024675666207));
#28963=CARTESIAN_POINT('Ctrl Pts',(-0.423458894885145,-3.04570961360995,
111.019684821));
#28964=CARTESIAN_POINT('Ctrl Pts',(-0.518320990312167,-3.02947942739373,
111.014693975793));
#28965=CARTESIAN_POINT('Ctrl Pts',(-0.613336385319549,-3.01322301278011,
111.009695065253));
#28966=CARTESIAN_POINT('Ctrl Pts',(-0.707469529745186,-2.99251230029474,
111.004696154712));
#28967=CARTESIAN_POINT('Ctrl Pts',(-0.80028247929883,-2.96748213193059,
110.999697244171));
#28968=CARTESIAN_POINT('Ctrl Pts',(-0.854165900677711,-2.95295063481046,
110.996795080148));
#28969=CARTESIAN_POINT('Ctrl Pts',(-0.90760466305668,-2.93696419463733,
110.993892916124));
#28970=CARTESIAN_POINT('Ctrl Pts',(-0.960516206135646,-2.91955662177509,
110.990990752101));
#28971=CARTESIAN_POINT('Ctrl Pts',(-1.05166603449257,-2.88956888779168,
110.985991242784));
#28972=CARTESIAN_POINT('Ctrl Pts',(-1.14157026989393,-2.85525578517736,
110.980991733467));
#28973=CARTESIAN_POINT('Ctrl Pts',(-1.22978890165704,-2.8167395171299,110.97599222415));
#28974=CARTESIAN_POINT('Ctrl Pts',(-1.31788786534854,-2.77827549618071,
110.970999496639));
#28975=CARTESIAN_POINT('Ctrl Pts',(-1.4043053708423,-2.73561981542936,110.966006769128));
#28976=CARTESIAN_POINT('Ctrl Pts',(-1.48861722045163,-2.6889442205027,110.961014041617));
#28977=CARTESIAN_POINT('Ctrl Pts',(-1.57284012313476,-2.64231786717987,
110.95602658131));
#28978=CARTESIAN_POINT('Ctrl Pts',(-1.65496140397517,-2.59168024183188,
110.951039121004));
#28979=CARTESIAN_POINT('Ctrl Pts',(-1.73457844313087,-2.53725045563612,
110.946051660697));
#28980=CARTESIAN_POINT('Ctrl Pts',(-1.81413851437789,-2.48285961526303,
110.941067769039));
#28981=CARTESIAN_POINT('Ctrl Pts',(-1.89119754470857,-2.42468225514321,
110.93608387738));
#28982=CARTESIAN_POINT('Ctrl Pts',(-1.96537991012113,-2.36298202678147,
110.931099985722));
#28983=CARTESIAN_POINT('Ctrl Pts',(-2.03953526012232,-2.30130426814069,
110.926117909075));
#28984=CARTESIAN_POINT('Ctrl Pts',(-2.11081568955522,-2.23610647073804,
110.921135832429));
#28985=CARTESIAN_POINT('Ctrl Pts',(-2.17887760419358,-2.16769339066752,
110.916153755782));
#28986=CARTESIAN_POINT('Ctrl Pts',(-2.24693331312855,-2.09928654831872,
110.911172133388));
#28987=CARTESIAN_POINT('Ctrl Pts',(-2.31177078124945,-2.0276653174803,110.906190510994));
#28988=CARTESIAN_POINT('Ctrl Pts',(-2.37308311076532,-1.95317147209363,
110.9012088886));
#28989=CARTESIAN_POINT('Ctrl Pts',(-2.43440658792414,-1.87866408243623,
110.896226360461));
#28990=CARTESIAN_POINT('Ctrl Pts',(-2.49220337466263,-1.80128337990646,
110.891243832322));
#28991=CARTESIAN_POINT('Ctrl Pts',(-2.54620740244167,-1.72140353019019,
110.886261304183));
#28992=CARTESIAN_POINT('Ctrl Pts',(-2.60026963859217,-1.64143758178544,
110.881273405613));
#28993=CARTESIAN_POINT('Ctrl Pts',(-2.65053070813879,-1.55896747270389,
110.876285507044));
#28994=CARTESIAN_POINT('Ctrl Pts',(-2.69676850814867,-1.47439542303197,
110.871297608475));
#28995=CARTESIAN_POINT('Ctrl Pts',(-2.74303362145348,-1.38977341550444,
110.866306763487));
#28996=CARTESIAN_POINT('Ctrl Pts',(-2.78527054091283,-1.30304738953272,
110.861315918498));
#28997=CARTESIAN_POINT('Ctrl Pts',(-2.82330460349125,-1.21464124987797,
110.85632507351));
#28998=CARTESIAN_POINT('Ctrl Pts',(-2.86140013008018,-1.12609224365762,
110.851326163189));
#28999=CARTESIAN_POINT('Ctrl Pts',(-2.89527908362788,-1.03585811296161,
110.846327252868));
#29000=CARTESIAN_POINT('Ctrl Pts',(-2.92481612909701,-0.944379616983535,
110.841328342548));
#29001=CARTESIAN_POINT('Ctrl Pts',(-2.94196414854108,-0.891270885123915,
110.838426176471));
#29002=CARTESIAN_POINT('Ctrl Pts',(-2.95764967560813,-0.83774298313627,
110.835524010394));
#29003=CARTESIAN_POINT('Ctrl Pts',(-2.97185612004942,-0.783883570260808,
110.832621844317));
#29004=CARTESIAN_POINT('Ctrl Pts',(-3.00334933232157,-0.664486635330965,
110.826188247741));
#29005=CARTESIAN_POINT('Ctrl Pts',(-3.02766111559864,-0.543122440475141,
110.819754651165));
#29006=CARTESIAN_POINT('Ctrl Pts',(-3.04459242176316,-0.420546353381311,
110.813321054589));
#29007=CARTESIAN_POINT('Ctrl Pts',(-3.06118864013233,-0.300396171908,110.807014785442));
#29008=CARTESIAN_POINT('Ctrl Pts',(-3.07069363673407,-0.179081372834902,
110.800708516296));
#29009=CARTESIAN_POINT('Ctrl Pts',(-3.07296516881628,-0.0573351658404085,
110.79440224715));
#29010=CARTESIAN_POINT('Ctrl Pts',(-3.07330444259114,-0.0391512733276938,
110.793460349056));
#29011=CARTESIAN_POINT('Ctrl Pts',(-3.07348243549809,-0.0209578007778193,
110.792518450962));
#29012=CARTESIAN_POINT('Ctrl Pts',(-3.07349876323956,-0.00275723864097975,
110.791576552868));
#29013=CARTESIAN_POINT('Origin',(0.,0.,116.208423447177));
#29014=CARTESIAN_POINT('',(1.87238193903529,2.43733217358128,112.437403601774));
#29015=CARTESIAN_POINT('',(1.86967294057238,2.43383856956498,112.354102866614));
#29016=CARTESIAN_POINT('',(1.8723819390353,2.43733217358128,116.208423447177));
#29017=CARTESIAN_POINT('',(-3.07300208187459,-5.30343035903902E-5,111.708423450995));
#29018=CARTESIAN_POINT('Ctrl Pts',(1.8696729405724,2.43383856956497,112.354102866614));
#29019=CARTESIAN_POINT('Ctrl Pts',(2.33883235148557,2.07028612302645,112.323472227234));
#29020=CARTESIAN_POINT('Ctrl Pts',(3.34734616429362,0.724855016743962,112.240051951927));
#29021=CARTESIAN_POINT('Ctrl Pts',(2.87385982532852,-2.21711305274817,112.103842040691));
#29022=CARTESIAN_POINT('Ctrl Pts',(-0.295019362129256,-3.61768143627294,
111.945473132907));
#29023=CARTESIAN_POINT('Ctrl Pts',(-2.70868458642244,-2.0401170948013,111.813666947708));
#29024=CARTESIAN_POINT('Ctrl Pts',(-3.06863383704806,-0.508468182011378,
111.734650398436));
#29025=CARTESIAN_POINT('Ctrl Pts',(-3.06855559257655,-5.3618658338984E-5,
111.708423485093));
#29026=CARTESIAN_POINT('Ctrl Pts',(-3.07349999954357,-5.29688675722701E-5,
111.708423447177));
#29027=CARTESIAN_POINT('Ctrl Pts',(-3.0735017428754,0.101103250511966,111.703213628981));
#29028=CARTESIAN_POINT('Ctrl Pts',(-3.06850524053228,0.202167062758812,
111.698003810785));
#29029=CARTESIAN_POINT('Ctrl Pts',(-3.05856358047855,0.302640172763362,
111.69279399259));
#29030=CARTESIAN_POINT('Ctrl Pts',(-3.04837689147292,0.405589611741622,
111.687455769652));
#29031=CARTESIAN_POINT('Ctrl Pts',(-3.03299816639765,0.507918428276897,
111.682117546715));
#29032=CARTESIAN_POINT('Ctrl Pts',(-3.01253985928769,0.609102492363057,
111.676779323777));
#29033=CARTESIAN_POINT('Ctrl Pts',(-2.99249659337028,0.708233817950399,
111.671549398286));
#29034=CARTESIAN_POINT('Ctrl Pts',(-2.96757807806514,0.806266060873926,
111.666319472794));
#29035=CARTESIAN_POINT('Ctrl Pts',(-2.93794030454541,0.902723111993713,
111.661089547303));
#29036=CARTESIAN_POINT('Ctrl Pts',(-2.90738195523853,1.00217620550186,111.655697175642));
#29037=CARTESIAN_POINT('Ctrl Pts',(-2.87180656578605,1.09995424282145,111.650304803981));
#29038=CARTESIAN_POINT('Ctrl Pts',(-2.83143769168113,1.19555963804716,111.644912432321));
#29039=CARTESIAN_POINT('Ctrl Pts',(-2.79106881757621,1.29116503327286,111.63952006066));
#29040=CARTESIAN_POINT('Ctrl Pts',(-2.74590671329826,1.38459743088285,111.634127688999));
#29041=CARTESIAN_POINT('Ctrl Pts',(-2.69622482898178,1.47538941353873,111.628735317339));
#29042=CARTESIAN_POINT('Ctrl Pts',(-2.65016252078614,1.55956674184112,111.62373580718));
#29043=CARTESIAN_POINT('Ctrl Pts',(-2.60007344932545,1.64173272528624,111.618736297021));
#29044=CARTESIAN_POINT('Ctrl Pts',(-2.54615779135673,1.72147690995652,111.613736786863));
#29045=CARTESIAN_POINT('Ctrl Pts',(-2.4923152695435,1.80111292228299,111.608744058499));
#29046=CARTESIAN_POINT('Ctrl Pts',(-2.43465672122309,1.87833330431815,111.603751330136));
#29047=CARTESIAN_POINT('Ctrl Pts',(-2.373428164222,1.95275216022869,111.598758601772));
#29048=CARTESIAN_POINT('Ctrl Pts',(-2.31226420171481,2.02709250623193,111.593771140604));
#29049=CARTESIAN_POINT('Ctrl Pts',(-2.24753799504432,2.09863686436192,111.588783679436));
#29050=CARTESIAN_POINT('Ctrl Pts',(-2.17953821425042,2.16702916976724,111.583796218267));
#29051=CARTESIAN_POINT('Ctrl Pts',(-2.11158708878564,2.2353725389835,111.578812325737));
#29052=CARTESIAN_POINT('Ctrl Pts',(-2.04036735421783,2.30056802863682,111.573828433206));
#29053=CARTESIAN_POINT('Ctrl Pts',(-1.96620656948055,2.36229421879061,111.568844540675));
#29054=CARTESIAN_POINT('Ctrl Pts',(-1.89207279219901,2.42399792984908,111.56386246315));
#29055=CARTESIAN_POINT('Ctrl Pts',(-1.81500042985993,2.48223457117628,111.558880385625));
#29056=CARTESIAN_POINT('Ctrl Pts',(-1.73535163647026,2.53672169301246,111.5538983081));
#29057=CARTESIAN_POINT('Ctrl Pts',(-1.655710105162,2.59120384691506,111.548916684823));
#29058=CARTESIAN_POINT('Ctrl Pts',(-1.57349297224867,2.64193691332774,111.543935061545));
#29059=CARTESIAN_POINT('Ctrl Pts',(-1.48909211962564,2.68868125839952,111.538953438267));
#29060=CARTESIAN_POINT('Ctrl Pts',(-1.40467592140137,2.73543410243851,111.533970909241));
#29061=CARTESIAN_POINT('Ctrl Pts',(-1.31807559896087,2.77819657220395,111.528988380214));
#29062=CARTESIAN_POINT('Ctrl Pts',(-1.22970746160734,2.81677507246625,111.524005851187));
#29063=CARTESIAN_POINT('Ctrl Pts',(-1.14124407644792,2.85539515465632,111.519017951729));
#29064=CARTESIAN_POINT('Ctrl Pts',(-1.05100947529692,2.88982208822087,111.514030052272));
#29065=CARTESIAN_POINT('Ctrl Pts',(-0.959439559524308,2.91991061192287,
111.509042152814));
#29066=CARTESIAN_POINT('Ctrl Pts',(-0.867815552139671,2.95001690933075,
111.504051306936));
#29067=CARTESIAN_POINT('Ctrl Pts',(-0.774855082346382,2.97577957682628,
111.499060461057));
#29068=CARTESIAN_POINT('Ctrl Pts',(-0.681006748292446,2.99710394527453,
111.494069615179));
#29069=CARTESIAN_POINT('Ctrl Pts',(-0.587006753089678,3.01846277441139,
111.489070703974));
#29070=CARTESIAN_POINT('Ctrl Pts',(-0.492116460493753,3.03536890586542,
111.48407179277));
#29071=CARTESIAN_POINT('Ctrl Pts',(-0.396792072387789,3.04777924090479,
111.479072881565));
#29072=CARTESIAN_POINT('Ctrl Pts',(-0.341450746844712,3.05498415881886,
111.476170724228));
#29073=CARTESIAN_POINT('Ctrl Pts',(-0.285963177142949,3.06067475437294,
111.473268566891));
#29074=CARTESIAN_POINT('Ctrl Pts',(-0.230418577022753,3.06485065368001,
111.470366409554));
#29075=CARTESIAN_POINT('Ctrl Pts',(-0.13475653099004,3.07204262321219,111.46536815035));
#29076=CARTESIAN_POINT('Ctrl Pts',(-0.0385894607515949,3.07476413519502,
111.460369891147));
#29077=CARTESIAN_POINT('Ctrl Pts',(0.057629702772162,3.07295965924683,111.455371631943));
#29078=CARTESIAN_POINT('Ctrl Pts',(0.153728586124074,3.07115743901018,111.450379620886));
#29079=CARTESIAN_POINT('Ctrl Pts',(0.249878998755944,3.06484047776547,111.44538760983));
#29080=CARTESIAN_POINT('Ctrl Pts',(0.345623507471124,3.05400501654522,111.440395598773));
#29081=CARTESIAN_POINT('Ctrl Pts',(0.441274476905546,3.04318014121926,111.435408464749));
#29082=CARTESIAN_POINT('Ctrl Pts',(0.536519896763965,3.02784558640366,111.430421330726));
#29083=CARTESIAN_POINT('Ctrl Pts',(0.630904023771938,3.00804959446954,111.425434196702));
#29084=CARTESIAN_POINT('Ctrl Pts',(0.725221712157909,2.98826753727707,111.420450573208));
#29085=CARTESIAN_POINT('Ctrl Pts',(0.818678884568398,2.96403037526767,111.415466949714));
#29086=CARTESIAN_POINT('Ctrl Pts',(0.910827663943631,2.93543782366362,111.410483326221));
#29087=CARTESIAN_POINT('Ctrl Pts',(1.00295458034917,2.90685205585087,111.405500885128));
#29088=CARTESIAN_POINT('Ctrl Pts',(1.09377329924995,2.87391307357728,111.400518444035));
#29089=CARTESIAN_POINT('Ctrl Pts',(1.18284962564052,2.83677087779787,111.395536002943));
#29090=CARTESIAN_POINT('Ctrl Pts',(1.27191077845996,2.79963500894921,111.390554410576));
#29091=CARTESIAN_POINT('Ctrl Pts',(1.35922972560432,2.75829752370882,111.38557281821));
#29092=CARTESIAN_POINT('Ctrl Pts',(1.44439210090478,2.71295663600506,111.380591225844));
#29093=CARTESIAN_POINT('Ctrl Pts',(1.52959967204653,2.66759168580237,111.375606989736));
#29094=CARTESIAN_POINT('Ctrl Pts',(1.61264799791362,2.6182192970358,111.370622753629));
#29095=CARTESIAN_POINT('Ctrl Pts',(1.69314762423507,2.56508350206131,111.365638517522));
#29096=CARTESIAN_POINT('Ctrl Pts',(1.75442187170347,2.52463790001969,111.361844645045));
#29097=CARTESIAN_POINT('Ctrl Pts',(1.81421992195117,2.48201279262311,111.358050772568));
#29098=CARTESIAN_POINT('Ctrl Pts',(1.87238193903529,2.43733217358128,111.354256900092));
#29099=CARTESIAN_POINT('',(-3.07349983534499,0.00100604885424971,111.791576552851));
#29100=CARTESIAN_POINT('Ctrl Pts',(-3.07349983534482,0.00100604938365495,
111.791576552823));
#29101=CARTESIAN_POINT('Ctrl Pts',(-3.07348152082622,0.0569572490138065,
111.788662798889));
#29102=CARTESIAN_POINT('Ctrl Pts',(-3.07193546894597,0.112881401490518,
111.785749044955));
#29103=CARTESIAN_POINT('Ctrl Pts',(-3.06886550242914,0.168721006399079,
111.782835291022));
#29104=CARTESIAN_POINT('Ctrl Pts',(-3.06359795374749,0.264532421803207,
111.777835776985));
#29105=CARTESIAN_POINT('Ctrl Pts',(-3.05382993681823,0.360265200941909,
111.772836262949));
#29106=CARTESIAN_POINT('Ctrl Pts',(-3.03956509812897,0.455462692474593,
111.767836748913));
#29107=CARTESIAN_POINT('Ctrl Pts',(-3.02531960945124,0.550531050226053,
111.762844016632));
#29108=CARTESIAN_POINT('Ctrl Pts',(-3.00658948658028,0.645065133062805,
111.757851284352));
#29109=CARTESIAN_POINT('Ctrl Pts',(-2.98343032572477,0.738610683341211,
111.752858552071));
#29110=CARTESIAN_POINT('Ctrl Pts',(-2.96029559699084,0.83205754626771,111.747871086952));
#29111=CARTESIAN_POINT('Ctrl Pts',(-2.93274122381603,0.924517525962698,
111.742883621833));
#29112=CARTESIAN_POINT('Ctrl Pts',(-2.90087414832287,1.01554489097826,111.737896156715));
#29113=CARTESIAN_POINT('Ctrl Pts',(-2.86902987418579,1.10650712459,111.7329122602));
#29114=CARTESIAN_POINT('Ctrl Pts',(-2.83287917678328,1.19603836816774,111.727928363685));
#29115=CARTESIAN_POINT('Ctrl Pts',(-2.79257902413718,1.28370738252493,111.72294446717));
#29116=CARTESIAN_POINT('Ctrl Pts',(-2.75229354760534,1.3713444704405,111.717962385641));
#29117=CARTESIAN_POINT('Ctrl Pts',(-2.70786180139085,1.45712027815022,111.712980304113));
#29118=CARTESIAN_POINT('Ctrl Pts',(-2.65948877004993,1.54062381260913,111.707998222584));
#29119=CARTESIAN_POINT('Ctrl Pts',(-2.6111201490396,1.62411973377235,111.703016595289));
#29120=CARTESIAN_POINT('Ctrl Pts',(-2.5588111775301,1.70534341383878,111.698034967993));
#29121=CARTESIAN_POINT('Ctrl Pts',(-2.50281212316432,1.78390967432258,111.693053340698));
#29122=CARTESIAN_POINT('Ctrl Pts',(-2.44680288705992,1.86249021971062,111.688070807643));
#29123=CARTESIAN_POINT('Ctrl Pts',(-2.3871024904373,1.93841202850577,111.683088274589));
#29124=CARTESIAN_POINT('Ctrl Pts',(-2.32400309100997,2.01132092988069,111.678105741535));
#29125=CARTESIAN_POINT('Ctrl Pts',(-2.26083567993026,2.08430841607417,111.673117838061));
#29126=CARTESIAN_POINT('Ctrl Pts',(-2.19426223971617,2.15427617912469,111.668129934586));
#29127=CARTESIAN_POINT('Ctrl Pts',(-2.12461344499306,2.22090521169966,111.663142031111));
#29128=CARTESIAN_POINT('Ctrl Pts',(-2.05492350779719,2.28757360293359,111.658151181216));
#29129=CARTESIAN_POINT('Ctrl Pts',(-1.98215492981803,2.35089904862615,111.65316033132));
#29130=CARTESIAN_POINT('Ctrl Pts',(-1.90667165472996,2.4106027153078,111.648169481424));
#29131=CARTESIAN_POINT('Ctrl Pts',(-1.83106639756289,2.47040286398995,111.643170566242));
#29132=CARTESIAN_POINT('Ctrl Pts',(-1.75273803992456,2.5265692911926,111.63817165106));
#29133=CARTESIAN_POINT('Ctrl Pts',(-1.67207962099826,2.57886641589717,111.633172735877));
#29134=CARTESIAN_POINT('Ctrl Pts',(-1.6252534188489,2.6092274837912,111.63027061833));
#29135=CARTESIAN_POINT('Ctrl Pts',(-1.57764237847426,2.63828530138454,111.627368500784));
#29136=CARTESIAN_POINT('Ctrl Pts',(-1.52932683085211,2.6660010679735,111.624466383237));
#29137=CARTESIAN_POINT('Ctrl Pts',(-1.44609310154743,2.71374732621273,111.619466873179));
#29138=CARTESIAN_POINT('Ctrl Pts',(-1.36047504679114,2.75767582035157,111.614467363121));
#29139=CARTESIAN_POINT('Ctrl Pts',(-1.272857686705,2.79754098439969,111.609467853063));
#29140=CARTESIAN_POINT('Ctrl Pts',(-1.18535917861251,2.83735207178744,111.604475124786));
#29141=CARTESIAN_POINT('Ctrl Pts',(-1.09586715131362,2.87311060331083,111.599482396509));
#29142=CARTESIAN_POINT('Ctrl Pts',(-1.00479290128081,2.90461589122137,111.594489668232));
#29143=CARTESIAN_POINT('Ctrl Pts',(-0.913814731890411,2.93608794198418,
111.589502207136));
#29144=CARTESIAN_POINT('Ctrl Pts',(-0.821258070667402,2.96331552636819,
111.584514746039));
#29145=CARTESIAN_POINT('Ctrl Pts',(-0.727555017792677,2.98614566725816,
111.579527284943));
#29146=CARTESIAN_POINT('Ctrl Pts',(-0.633919011088274,3.00895947278373,
111.574543392462));
#29147=CARTESIAN_POINT('Ctrl Pts',(-0.539138668639977,3.02738198619175,
111.569559499982));
#29148=CARTESIAN_POINT('Ctrl Pts',(-0.443661171355982,3.04131008202568,
111.564575607501));
#29149=CARTESIAN_POINT('Ctrl Pts',(-0.348218444266958,3.05523310564237,
111.559593530012));
#29150=CARTESIAN_POINT('Ctrl Pts',(-0.252079500703078,3.06466490040868,
111.554611452524));
#29151=CARTESIAN_POINT('Ctrl Pts',(-0.15570068197844,3.06955363980359,111.549629375035));
#29152=CARTESIAN_POINT('Ctrl Pts',(-0.0593306504513404,3.07444193347485,
111.54464775178));
#29153=CARTESIAN_POINT('Ctrl Pts',(0.0372787743465924,3.07478797323944,
111.539666128525));
#29154=CARTESIAN_POINT('Ctrl Pts',(0.133668249681294,3.07059197045572,111.53468450527));
#29155=CARTESIAN_POINT('Ctrl Pts',(0.230075250633477,3.06639520475116,111.529701976252));
#29156=CARTESIAN_POINT('Ctrl Pts',(0.326261784158633,3.05765477550851,111.524719447234));
#29157=CARTESIAN_POINT('Ctrl Pts',(0.421771709378268,3.04442291332333,111.519736918216));
#29158=CARTESIAN_POINT('Ctrl Pts',(0.517384580606425,3.03117678908745,111.514749018746));
#29159=CARTESIAN_POINT('Ctrl Pts',(0.612318952045057,3.01342962739635,111.509761119276));
#29160=CARTESIAN_POINT('Ctrl Pts',(0.706127207081683,2.99128511135582,111.504773219806));
#29161=CARTESIAN_POINT('Ctrl Pts',(0.799990876175341,2.96912751419067,111.499782373903));
#29162=CARTESIAN_POINT('Ctrl Pts',(0.892726682516278,2.94256751125802,111.494791528));
#29163=CARTESIAN_POINT('Ctrl Pts',(0.983902593640346,2.91175856420614,111.489800682096));
#29164=CARTESIAN_POINT('Ctrl Pts',(1.0752258475601,2.88089982904318,111.484801770848));
#29165=CARTESIAN_POINT('Ctrl Pts',(1.16498376420778,2.84577859889926,111.4798028596));
#29166=CARTESIAN_POINT('Ctrl Pts',(1.25276474985378,2.80659628937327,111.474803948352));
#29167=CARTESIAN_POINT('Ctrl Pts',(1.30372669833892,2.78384868834216,111.471901790719));
#29168=CARTESIAN_POINT('Ctrl Pts',(1.35402277901538,2.75973317641541,111.468999633086));
#29169=CARTESIAN_POINT('Ctrl Pts',(1.40357670663329,2.73429601151676,111.466097475453));
#29170=CARTESIAN_POINT('Ctrl Pts',(1.48892153014178,2.6904865608195,111.46109920099));
#29171=CARTESIAN_POINT('Ctrl Pts',(1.57236313612921,2.6426005861688,111.456100926526));
#29172=CARTESIAN_POINT('Ctrl Pts',(1.65348622624554,2.59082719408615,111.451102652063));
#29173=CARTESIAN_POINT('Ctrl Pts',(1.7285402802135,2.54292710845203,111.44647831193));
#29174=CARTESIAN_POINT('Ctrl Pts',(1.80160966012451,2.49170011663527,111.441853971797));
#29175=CARTESIAN_POINT('Ctrl Pts',(1.87238193903529,2.43733217358128,111.437229631665));
#29176=CARTESIAN_POINT('Ctrl Pts',(1.87238193903529,2.43733217358128,112.437403601774));
#29177=CARTESIAN_POINT('Ctrl Pts',(1.94879948025963,2.37862748590479,112.432404200454));
#29178=CARTESIAN_POINT('Ctrl Pts',(2.02235522355243,2.31640107103305,112.427404799134));
#29179=CARTESIAN_POINT('Ctrl Pts',(2.09272617106382,2.25097743723578,112.422405397814));
#29180=CARTESIAN_POINT('Ctrl Pts',(2.12132119668281,2.22439273785799,112.420373905928));
#29181=CARTESIAN_POINT('Ctrl Pts',(2.14939080333889,2.19728052007338,112.418342414043));
#29182=CARTESIAN_POINT('Ctrl Pts',(2.17691522061888,2.16966411507354,112.416310922158));
#29183=CARTESIAN_POINT('Ctrl Pts',(2.24465163213634,2.10170132571918,112.411311507677));
#29184=CARTESIAN_POINT('Ctrl Pts',(2.30932133936017,2.03044400536883,112.406312093196));
#29185=CARTESIAN_POINT('Ctrl Pts',(2.37058714894232,1.95620009694037,112.401312678715));
#29186=CARTESIAN_POINT('Ctrl Pts',(2.4317698329323,1.88205692281862,112.396320047451));
#29187=CARTESIAN_POINT('Ctrl Pts',(2.48955752105744,1.80493554979578,112.391327416187));
#29188=CARTESIAN_POINT('Ctrl Pts',(2.54364952514628,1.72518095955848,112.386334784923));
#29189=CARTESIAN_POINT('Ctrl Pts',(2.59768444864421,1.64551053035782,112.381347422133));
#29190=CARTESIAN_POINT('Ctrl Pts',(2.64803119571126,1.56321276920054,112.376360059344));
#29191=CARTESIAN_POINT('Ctrl Pts',(2.69442974111918,1.47866514808879,112.371372696554));
#29192=CARTESIAN_POINT('Ctrl Pts',(2.74079507273524,1.39417804928576,112.366388903903));
#29193=CARTESIAN_POINT('Ctrl Pts',(2.7832176105889,1.30744467592563,112.361405111252));
#29194=CARTESIAN_POINT('Ctrl Pts',(2.82148154763242,1.21887002029328,112.356421318601));
#29195=CARTESIAN_POINT('Ctrl Pts',(2.85973154280678,1.13032763777123,112.351439341847));
#29196=CARTESIAN_POINT('Ctrl Pts',(2.89382577385429,1.03994570853644,112.346457365094));
#29197=CARTESIAN_POINT('Ctrl Pts',(2.92359558836734,0.94815140440702,112.34147538834));
#29198=CARTESIAN_POINT('Ctrl Pts',(2.95336268392932,0.856365484079305,112.336493866603));
#29199=CARTESIAN_POINT('Ctrl Pts',(2.97880601296027,0.763167862951526,112.331512344865));
#29200=CARTESIAN_POINT('Ctrl Pts',(2.99980639222127,0.669002136908707,112.326530823128));
#29201=CARTESIAN_POINT('Ctrl Pts',(3.02081058708148,0.574819301714405,112.321548396289));
#29202=CARTESIAN_POINT('Ctrl Pts',(3.03737013346229,0.479668440734097,112.316565969449));
#29203=CARTESIAN_POINT('Ctrl Pts',(3.04941691172385,0.384003578749662,112.311583542609));
#29204=CARTESIAN_POINT('Ctrl Pts',(3.0614766740101,0.288235609120851,112.306595745707));
#29205=CARTESIAN_POINT('Ctrl Pts',(3.06901390298465,0.191952968761404,112.301607948805));
#29206=CARTESIAN_POINT('Ctrl Pts',(3.07201237877847,0.0956148243308455,
112.296620151903));
#29207=CARTESIAN_POINT('Ctrl Pts',(3.07501262563339,-0.00078022258996073,
112.29162940894));
#29208=CARTESIAN_POINT('Ctrl Pts',(3.07346878836156,-0.0972304001388508,
112.286638665976));
#29209=CARTESIAN_POINT('Ctrl Pts',(3.06741676537897,-0.193278652395989,
112.281647923013));
#29210=CARTESIAN_POINT('Ctrl Pts',(3.06135496143944,-0.289482132718584,
112.276649114277));
#29211=CARTESIAN_POINT('Ctrl Pts',(3.05077047165617,-0.385281954668675,
112.271650305541));
#29212=CARTESIAN_POINT('Ctrl Pts',(3.0357508125885,-0.480228335136801,112.266651496805));
#29213=CARTESIAN_POINT('Ctrl Pts',(3.02702783719739,-0.535370395057574,
112.263748335995));
#29214=CARTESIAN_POINT('Ctrl Pts',(3.01680985790913,-0.59022480529076,112.260845175184));
#29215=CARTESIAN_POINT('Ctrl Pts',(3.00512174396439,-0.644705788676058,
112.257942014374));
#29216=CARTESIAN_POINT('Ctrl Pts',(2.98499361965295,-0.738527598710917,
112.252942475358));
#29217=CARTESIAN_POINT('Ctrl Pts',(2.96043216917071,-0.831570661220707,
112.247942936343));
#29218=CARTESIAN_POINT('Ctrl Pts',(2.93151213234959,-0.923384463745818,
112.242943397327));
#29219=CARTESIAN_POINT('Ctrl Pts',(2.90263132364309,-1.01507372692849,112.237950639855));
#29220=CARTESIAN_POINT('Ctrl Pts',(2.86940380932578,-1.10553662889735,112.232957882383));
#29221=CARTESIAN_POINT('Ctrl Pts',(2.83195527184254,-1.19433311445478,112.227965124911));
#29222=CARTESIAN_POINT('Ctrl Pts',(2.79454623976421,-1.28303592636426,112.222977634424));
#29223=CARTESIAN_POINT('Ctrl Pts',(2.75292520621421,-1.37007541424261,112.217990143938));
#29224=CARTESIAN_POINT('Ctrl Pts',(2.70726724450543,-1.4550279436588,112.213002653451));
#29225=CARTESIAN_POINT('Ctrl Pts',(2.66164195014025,-1.53991969126688,112.208018731413));
#29226=CARTESIAN_POINT('Ctrl Pts',(2.61198567671238,-1.62272706323516,112.203034809374));
#29227=CARTESIAN_POINT('Ctrl Pts',(2.55852065513925,-1.70304853343227,112.198050887336));
#29228=CARTESIAN_POINT('Ctrl Pts',(2.50507510290357,-1.78334075449113,112.193068780197));
#29229=CARTESIAN_POINT('Ctrl Pts',(2.44782380124132,-1.86114850736622,112.188086673059));
#29230=CARTESIAN_POINT('Ctrl Pts',(2.38703325753857,-1.93609774479616,112.18310456592));
#29231=CARTESIAN_POINT('Ctrl Pts',(2.32624825561316,-2.01104014971631,112.178122912959));
#29232=CARTESIAN_POINT('Ctrl Pts',(2.26192492977835,-2.08312421648798,112.173141259999));
#29233=CARTESIAN_POINT('Ctrl Pts',(2.19437049641909,-2.15200845129508,112.168159607038));
#29234=CARTESIAN_POINT('Ctrl Pts',(2.12680378007173,-2.22090521087952,112.163177048296));
#29235=CARTESIAN_POINT('Ctrl Pts',(2.05600509681178,-2.28660066966237,112.158194489553));
#29236=CARTESIAN_POINT('Ctrl Pts',(1.9823182115159,-2.34879048837745,112.153211930811));
#29237=CARTESIAN_POINT('Ctrl Pts',(1.90855190506639,-2.4110473364849,112.14822400177));
#29238=CARTESIAN_POINT('Ctrl Pts',(1.83189151785293,-2.46979071762057,112.143236072729));
#29239=CARTESIAN_POINT('Ctrl Pts',(1.75271338391871,-2.52475702669232,112.138248143688));
#29240=CARTESIAN_POINT('Ctrl Pts',(1.67348847913685,-2.5797558045877,112.133257268257));
#29241=CARTESIAN_POINT('Ctrl Pts',(1.59174323809057,-2.63097283491827,112.128266392826));
#29242=CARTESIAN_POINT('Ctrl Pts',(1.50788059978875,-2.67818937843849,112.123275517395));
#29243=CARTESIAN_POINT('Ctrl Pts',(1.42388244400905,-2.72548222133374,112.11827657698));
#29244=CARTESIAN_POINT('Ctrl Pts',(1.33776045074766,-2.7687614721309,112.113277636565));
#29245=CARTESIAN_POINT('Ctrl Pts',(1.24993956183347,-2.80785564831306,112.108278696149));
#29246=CARTESIAN_POINT('Ctrl Pts',(1.19895991747353,-2.83054964769012,112.105376832963));
#29247=CARTESIAN_POINT('Ctrl Pts',(1.1474081292581,-2.85183429548936,112.102474969776));
#29248=CARTESIAN_POINT('Ctrl Pts',(1.09536956853821,-2.87168378452789,112.09957310659));
#29249=CARTESIAN_POINT('Ctrl Pts',(1.00571417110824,-2.90588176779091,112.094573589046));
#29250=CARTESIAN_POINT('Ctrl Pts',(0.914298255469063,-2.93593716116456,
112.089574071502));
#29251=CARTESIAN_POINT('Ctrl Pts',(0.82154039614416,-2.96166737286673,112.084574553959));
#29252=CARTESIAN_POINT('Ctrl Pts',(0.728908357998077,-2.98736268288411,
112.079581817999));
#29253=CARTESIAN_POINT('Ctrl Pts',(0.634938413216042,-3.00874435494215,
112.074589082039));
#29254=CARTESIAN_POINT('Ctrl Pts',(0.540068100907363,-3.02567822089235,
112.069596346079));
#29255=CARTESIAN_POINT('Ctrl Pts',(0.445297870295764,-3.04259422277105,
112.064608877114));
#29256=CARTESIAN_POINT('Ctrl Pts',(0.349629590187939,-3.05507166949399,
112.059621408149));
#29257=CARTESIAN_POINT('Ctrl Pts',(0.253513917243686,-3.06302676184257,
112.054633939184));
#29258=CARTESIAN_POINT('Ctrl Pts',(0.157467011910874,-3.07097616258349,
112.04965003859));
#29259=CARTESIAN_POINT('Ctrl Pts',(0.0609737862857786,-3.07440960505889,
112.044666137996));
#29260=CARTESIAN_POINT('Ctrl Pts',(-0.0355079720195087,-3.07329488235722,
112.039682237402));
#29261=CARTESIAN_POINT('Ctrl Pts',(-0.131954597342464,-3.072180565572,112.034700151651));
#29262=CARTESIAN_POINT('Ctrl Pts',(-0.228389325159465,-3.06652137931458,
112.0297180659));
#29263=CARTESIAN_POINT('Ctrl Pts',(-0.324353310408222,-3.05633721634692,
112.024735980149));
#29264=CARTESIAN_POINT('Ctrl Pts',(-0.420308548972106,-3.04615398161983,
112.019754348493));
#29265=CARTESIAN_POINT('Ctrl Pts',(-0.515792693782929,-3.0314466366791,
112.014772716837));
#29266=CARTESIAN_POINT('Ctrl Pts',(-0.610352041216524,-3.0122869444631,
112.009791085181));
#29267=CARTESIAN_POINT('Ctrl Pts',(-0.70492858393743,-2.99312376812393,
112.004808547633));
#29268=CARTESIAN_POINT('Ctrl Pts',(-0.79857956508617,-2.96950672376021,
111.999826010084));
#29269=CARTESIAN_POINT('Ctrl Pts',(-0.890862547100991,-2.94155845975781,
111.994843472536));
#29270=CARTESIAN_POINT('Ctrl Pts',(-0.983244999487806,-2.91358007076209,
111.989855564389));
#29271=CARTESIAN_POINT('Ctrl Pts',(-1.07425608813524,-2.88126126923715,
111.984867656242));
#29272=CARTESIAN_POINT('Ctrl Pts',(-1.16346981067153,-2.84477420011782,
111.979879748094));
#29273=CARTESIAN_POINT('Ctrl Pts',(-1.25273623481969,-2.80826557683282,
111.974888893419));
#29274=CARTESIAN_POINT('Ctrl Pts',(-1.34020278087729,-2.76758396806884,
111.969898038743));
#29275=CARTESIAN_POINT('Ctrl Pts',(-1.4254665945932,-2.72294826203123,111.964907184067));
#29276=CARTESIAN_POINT('Ctrl Pts',(-1.51086819786687,-2.67824042299924,
111.95990826398));
#29277=CARTESIAN_POINT('Ctrl Pts',(-1.59405958224704,-2.62956594886001,
111.954909343894));
#29278=CARTESIAN_POINT('Ctrl Pts',(-1.67466555268891,-2.57718791255841,
111.949910423808));
#29279=CARTESIAN_POINT('Ctrl Pts',(-1.72146057395033,-2.54678034710228,
111.947008348807));
#29280=CARTESIAN_POINT('Ctrl Pts',(-1.76738482178594,-2.51512536555158,
111.944106273806));
#29281=CARTESIAN_POINT('Ctrl Pts',(-1.81237015387301,-2.48228053921194,
111.941204198806));
#29282=CARTESIAN_POINT('Ctrl Pts',(-1.88923164428324,-2.42616219601858,
111.93624574236));
#29283=CARTESIAN_POINT('Ctrl Pts',(-1.96363015846744,-2.36636383511589,
111.931287285915));
#29284=CARTESIAN_POINT('Ctrl Pts',(-2.03518809297881,-2.30313084217924,
111.926328829469));
#29285=CARTESIAN_POINT('Ctrl Pts',(-2.10664864570303,-2.23998390178032,
111.92137712089));
#29286=CARTESIAN_POINT('Ctrl Pts',(-2.17527596659793,-2.17341190847224,
111.91642541231));
#29287=CARTESIAN_POINT('Ctrl Pts',(-2.24072242206252,-2.10370275401879,
111.911473703731));
#29288=CARTESIAN_POINT('Ctrl Pts',(-2.30675050290536,-2.03337409140347,
111.906477989111));
#29289=CARTESIAN_POINT('Ctrl Pts',(-2.36954051726184,-1.95985248829929,
111.901482274491));
#29290=CARTESIAN_POINT('Ctrl Pts',(-2.42877049203524,-1.88347448801912,
111.896486559871));
#29291=CARTESIAN_POINT('Ctrl Pts',(-2.48737632744141,-1.8079013254406,111.89154348789));
#29292=CARTESIAN_POINT('Ctrl Pts',(-2.54249651377506,-1.72953203929604,
111.886600415908));
#29293=CARTESIAN_POINT('Ctrl Pts',(-2.59385799705819,-1.64872767341888,
111.881657343927));
#29294=CARTESIAN_POINT('Ctrl Pts',(-2.6452024680113,-1.5679500721609,111.876715909226));
#29295=CARTESIAN_POINT('Ctrl Pts',(-2.69279046934162,-1.48473937024501,
111.871774474526));
#29296=CARTESIAN_POINT('Ctrl Pts',(-2.7363920694606,-1.39948586709303,111.866833039825));
#29297=CARTESIAN_POINT('Ctrl Pts',(-2.77999162848551,-1.31423635485925,
111.861891836445));
#29298=CARTESIAN_POINT('Ctrl Pts',(-2.81960495457762,-1.22694462992712,
111.856950633065));
#29299=CARTESIAN_POINT('Ctrl Pts',(-2.85504846778913,-1.13802482247749,
111.852009429685));
#29300=CARTESIAN_POINT('Ctrl Pts',(-2.89117248629991,-1.04739778019993,
111.846973356615));
#29301=CARTESIAN_POINT('Ctrl Pts',(-2.92296471426377,-0.95507992912274,
111.841937283546));
#29302=CARTESIAN_POINT('Ctrl Pts',(-2.95028314976414,-0.861528633428869,
111.836901210476));
#29303=CARTESIAN_POINT('Ctrl Pts',(-2.97712196335533,-0.769619790907143,
111.831953554292));
#29304=CARTESIAN_POINT('Ctrl Pts',(-2.99964275917986,-0.676520919820833,
111.827005898108));
#29305=CARTESIAN_POINT('Ctrl Pts',(-3.01776236287641,-0.582677072834153,
111.822058241924));
#29306=CARTESIAN_POINT('Ctrl Pts',(-3.03636767501656,-0.486317676963264,
111.816977960412));
#29307=CARTESIAN_POINT('Ctrl Pts',(-3.05033240432285,-0.389173298906863,
111.811897678899));
#29308=CARTESIAN_POINT('Ctrl Pts',(-3.05962341637771,-0.291730697653163,
111.806817397387));
#29309=CARTESIAN_POINT('Ctrl Pts',(-3.06891442843256,-0.194288096399463,
111.801737115875));
#29310=CARTESIAN_POINT('Ctrl Pts',(-3.07353176764381,-0.0965477774265246,
111.796656834363));
#29311=CARTESIAN_POINT('Ctrl Pts',(-3.07349983534499,0.0010060488542432,
111.791576552851));
#29312=CARTESIAN_POINT('Origin',(0.,0.,116.208423447177));
#29313=CARTESIAN_POINT('',(1.8723819390353,2.43733217358127,113.437353936953));
#29314=CARTESIAN_POINT('',(1.8746157427793,2.44019679077305,113.354075550313));
#29315=CARTESIAN_POINT('',(1.8723819390353,2.43733217358128,116.208423447177));
#29316=CARTESIAN_POINT('',(-3.07304940657614,-0.00348278968395837,113.791576743866));
#29317=CARTESIAN_POINT('Ctrl Pts',(-3.07349803031876,-0.00347960151198421,
113.791576552823));
#29318=CARTESIAN_POINT('Ctrl Pts',(-3.07360613510913,0.0920083039628076,
113.786645986316));
#29319=CARTESIAN_POINT('Ctrl Pts',(-3.06926002918478,0.187573875915372,
113.78171541981));
#29320=CARTESIAN_POINT('Ctrl Pts',(-3.0604649665282,0.282765695680308,113.776784853303));
#29321=CARTESIAN_POINT('Ctrl Pts',(-3.05167259930464,0.37792834189809,113.771855797873));
#29322=CARTESIAN_POINT('Ctrl Pts',(-3.0384340242833,0.472717016989944,113.766926742443));
#29323=CARTESIAN_POINT('Ctrl Pts',(-3.02080650617518,0.566683599771268,
113.761997687013));
#29324=CARTESIAN_POINT('Ctrl Pts',(-3.00317934056945,0.660648303476645,
113.757068730151));
#29325=CARTESIAN_POINT('Ctrl Pts',(-2.98116348973558,0.753790506665149,
113.752139773288));
#29326=CARTESIAN_POINT('Ctrl Pts',(-2.95486745376389,0.845671674284358,
113.747210816426));
#29327=CARTESIAN_POINT('Ctrl Pts',(-2.9285644100671,0.937577327646052,113.742280546028));
#29328=CARTESIAN_POINT('Ctrl Pts',(-2.89797904042123,1.02822084712495,113.73735027563));
#29329=CARTESIAN_POINT('Ctrl Pts',(-2.86326952617376,1.11717942627168,113.732420005232));
#29330=CARTESIAN_POINT('Ctrl Pts',(-2.82851938726505,1.20624212419447,113.727483964354));
#29331=CARTESIAN_POINT('Ctrl Pts',(-2.78963563639662,1.29361552880427,113.722547923476));
#29332=CARTESIAN_POINT('Ctrl Pts',(-2.74682422301602,1.37889772566801,113.717611882598));
#29333=CARTESIAN_POINT('Ctrl Pts',(-2.70398333184197,1.46423864357798,113.71267244301));
#29334=CARTESIAN_POINT('Ctrl Pts',(-2.65720961820313,1.54748509953168,113.707733003422));
#29335=CARTESIAN_POINT('Ctrl Pts',(-2.60675337106642,1.628262605489,113.702793563833));
#29336=CARTESIAN_POINT('Ctrl Pts',(-2.55621556095394,1.70917068900878,113.697846139597));
#29337=CARTESIAN_POINT('Ctrl Pts',(-2.50198359661781,1.78760149362166,113.69289871536));
#29338=CARTESIAN_POINT('Ctrl Pts',(-2.44434893228502,1.86321242676112,113.687951291123));
#29339=CARTESIAN_POINT('Ctrl Pts',(-2.42614046142172,1.88710012505789,113.686388255559));
#29340=CARTESIAN_POINT('Ctrl Pts',(-2.40759264321255,1.91070664089894,113.684825219995));
#29341=CARTESIAN_POINT('Ctrl Pts',(-2.38871541829762,1.93402194930337,113.683262184432));
#29342=CARTESIAN_POINT('Ctrl Pts',(-2.3282774956313,2.00866898098517,113.678257920142));
#29343=CARTESIAN_POINT('Ctrl Pts',(-2.26423183045799,2.08061038074523,113.673253655852));
#29344=CARTESIAN_POINT('Ctrl Pts',(-2.19684950773242,2.14947772502434,113.668249391562));
#29345=CARTESIAN_POINT('Ctrl Pts',(-2.12955880479925,2.21825143032619,113.663251931574));
#29346=CARTESIAN_POINT('Ctrl Pts',(-2.05894076516932,2.28395907721264,113.658254471586));
#29347=CARTESIAN_POINT('Ctrl Pts',(-1.98530715722022,2.34626463586062,113.653257011598));
#29348=CARTESIAN_POINT('Ctrl Pts',(-1.91175158892653,2.4085041607441,113.648264848105));
#29349=CARTESIAN_POINT('Ctrl Pts',(-1.8351871386764,2.46734848414005,113.643272684612));
#29350=CARTESIAN_POINT('Ctrl Pts',(-1.75596218297494,2.52249857521504,113.638280521119));
#29351=CARTESIAN_POINT('Ctrl Pts',(-1.67679488852393,2.57760852712951,113.633291991007));
#29352=CARTESIAN_POINT('Ctrl Pts',(-1.59497129682453,2.6290293427901,113.628303460894));
#29353=CARTESIAN_POINT('Ctrl Pts',(-1.51087183006416,2.67650304747044,113.623314930782));
#29354=CARTESIAN_POINT('Ctrl Pts',(-1.42680367119149,2.72395907901359,113.61832825776));
#29355=CARTESIAN_POINT('Ctrl Pts',(-1.34046170176576,2.7674707042323,113.613341584738));
#29356=CARTESIAN_POINT('Ctrl Pts',(-1.25225340771642,2.8068244784565,113.608354911716));
#29357=CARTESIAN_POINT('Ctrl Pts',(-1.16405400161499,2.84617428735863,113.603368741156));
#29358=CARTESIAN_POINT('Ctrl Pts',(-1.07398904484235,2.88136689997652,113.598382570596));
#29359=CARTESIAN_POINT('Ctrl Pts',(-0.982487622527084,2.91223630936452,
113.593396400036));
#29360=CARTESIAN_POINT('Ctrl Pts',(-0.890970576799521,2.94311098955048,
113.588409378112));
#29361=CARTESIAN_POINT('Ctrl Pts',(-0.798016993449633,2.96966086056145,
113.583422356188));
#29362=CARTESIAN_POINT('Ctrl Pts',(-0.704071778567027,2.99176957345071,
113.578435334264));
#29363=CARTESIAN_POINT('Ctrl Pts',(-0.610027500913148,3.01390159939931,
113.573443053656));
#29364=CARTESIAN_POINT('Ctrl Pts',(-0.514989931181838,3.03158301716507,
113.568450773048));
#29365=CARTESIAN_POINT('Ctrl Pts',(-0.419414628834668,3.04474853134368,
113.56345849244));
#29366=CARTESIAN_POINT('Ctrl Pts',(-0.323784005594781,3.05792166598468,
113.5584633222));
#29367=CARTESIAN_POINT('Ctrl Pts',(-0.227615465991627,3.06657365253343,
113.55346815196));
#29368=CARTESIAN_POINT('Ctrl Pts',(-0.131368064689393,3.0706912383989,113.54847298172));
#29369=CARTESIAN_POINT('Ctrl Pts',(-0.0349678284998302,3.07481536273464,
113.543469879461));
#29370=CARTESIAN_POINT('Ctrl Pts',(0.0615110817052908,3.07439071040301,
113.538466777202));
#29371=CARTESIAN_POINT('Ctrl Pts',(0.157611306929676,3.06945612868598,113.533463674942));
#29372=CARTESIAN_POINT('Ctrl Pts',(0.212485074158239,3.06663845486806,113.53060687551));
#29373=CARTESIAN_POINT('Ctrl Pts',(0.2672354795067,3.06235128439908,113.527750076079));
#29374=CARTESIAN_POINT('Ctrl Pts',(0.321778771217115,3.05660934245677,113.524893276647));
#29375=CARTESIAN_POINT('Ctrl Pts',(0.417380576494212,3.04654504310359,113.519885966409));
#29376=CARTESIAN_POINT('Ctrl Pts',(0.512671443783229,3.03197421992204,113.514878656172));
#29377=CARTESIAN_POINT('Ctrl Pts',(0.607194239830824,3.01292505799867,113.509871345934));
#29378=CARTESIAN_POINT('Ctrl Pts',(0.701597580057766,2.99389996998514,113.504870363824));
#29379=CARTESIAN_POINT('Ctrl Pts',(0.795234352760283,2.97040787511575,113.499869381714));
#29380=CARTESIAN_POINT('Ctrl Pts',(0.887652546274494,2.94252870964625,113.494868399605));
#29381=CARTESIAN_POINT('Ctrl Pts',(0.979969062029866,2.91468021661207,113.489872919536));
#29382=CARTESIAN_POINT('Ctrl Pts',(1.07106924864573,2.88245437851228,113.484877439466));
#29383=CARTESIAN_POINT('Ctrl Pts',(1.1605124657483,2.8459819161131,113.479881959397));
#29384=CARTESIAN_POINT('Ctrl Pts',(1.24989707729888,2.80953335143206,113.474889752498));
#29385=CARTESIAN_POINT('Ctrl Pts',(1.33762647348917,2.76884385735648,113.469897545599));
#29386=CARTESIAN_POINT('Ctrl Pts',(1.42327710334293,2.72409334221494,113.4649053387));
#29387=CARTESIAN_POINT('Ctrl Pts',(1.50890863332699,2.67935280632294,113.459914245051));
#29388=CARTESIAN_POINT('Ctrl Pts',(1.59246192734598,2.63055324429409,113.454923151401));
#29389=CARTESIAN_POINT('Ctrl Pts',(1.67353604504419,2.57792151857613,113.449932057751));
#29390=CARTESIAN_POINT('Ctrl Pts',(1.74164136207261,2.53370888367436,113.445739350819));
#29391=CARTESIAN_POINT('Ctrl Pts',(1.80799749284803,2.48679292230585,113.441546643886));
#29392=CARTESIAN_POINT('Ctrl Pts',(1.8723819390353,2.43733217358127,113.437353936953));
#29393=CARTESIAN_POINT('',(-0.793799282533091,-2.96922295374563,114.));
#29394=CARTESIAN_POINT('Ctrl Pts',(-0.793799282533038,-2.96922295374565,
114.));
#29395=CARTESIAN_POINT('Ctrl Pts',(-1.77865212890027,-2.7059299996545,113.947210364072));
#29396=CARTESIAN_POINT('Ctrl Pts',(-2.87774335179386,-1.66670642438129,
113.877736327106));
#29397=CARTESIAN_POINT('Ctrl Pts',(-3.07274765096662,-0.326293812111691,
113.808262290142));
#29398=CARTESIAN_POINT('Ctrl Pts',(-3.07036006322683,-0.00350190166640733,
113.791577889105));
#29399=CARTESIAN_POINT('',(0.794173972183063,-2.96912275797195,113.999999974814));
#29400=CARTESIAN_POINT('Origin',(0.,0.,114.));
#29401=CARTESIAN_POINT('',(-3.07349930869882,0.00206141404370558,113.708423447177));
#29402=CARTESIAN_POINT('Ctrl Pts',(0.794173972183063,-2.96912275797195,
113.999999974814));
#29403=CARTESIAN_POINT('Ctrl Pts',(0.701819794355633,-2.99382543624822,
113.995019289507));
#29404=CARTESIAN_POINT('Ctrl Pts',(0.608144005864226,-3.01425987787217,
113.990038604201));
#29405=CARTESIAN_POINT('Ctrl Pts',(0.513578555021576,-3.03028700254975,
113.985057918894));
#29406=CARTESIAN_POINT('Ctrl Pts',(0.419141384954323,-3.04629238596811,
113.980083990031));
#29407=CARTESIAN_POINT('Ctrl Pts',(0.32381738326219,-3.05790225921004,113.975110061168));
#29408=CARTESIAN_POINT('Ctrl Pts',(0.228052546930729,-3.06502761583618,
113.970136132306));
#29409=CARTESIAN_POINT('Ctrl Pts',(0.128387450814283,-3.07244317023184,
113.964959627889));
#29410=CARTESIAN_POINT('Ctrl Pts',(0.0282453099355113,-3.07500098941394,
113.959783123473));
#29411=CARTESIAN_POINT('Ctrl Pts',(-0.0718603908461009,-3.07265981426963,
113.954606619057));
#29412=CARTESIAN_POINT('Ctrl Pts',(-0.167878281058049,-3.07041424087852,
113.949641496903));
#29413=CARTESIAN_POINT('Ctrl Pts',(-0.263862157958898,-3.0636619461203,
113.944676374749));
#29414=CARTESIAN_POINT('Ctrl Pts',(-0.35935623066889,-3.05241958935521,
113.939711252594));
#29415=CARTESIAN_POINT('Ctrl Pts',(-0.454818200664135,-3.0411810119888,
113.93474779959));
#29416=CARTESIAN_POINT('Ctrl Pts',(-0.549790254354859,-3.02545542312751,
113.929784346585));
#29417=CARTESIAN_POINT('Ctrl Pts',(-0.643821149403549,-3.00531139444496,
113.924820893581));
#29418=CARTESIAN_POINT('Ctrl Pts',(-0.737846617600058,-2.98516852834483,
113.919857727034));
#29419=CARTESIAN_POINT('Ctrl Pts',(-0.830930602409861,-2.96060782271577,
113.914894560488));
#29420=CARTESIAN_POINT('Ctrl Pts',(-0.922632597200634,-2.93174885359964,
113.909931393942));
#29421=CARTESIAN_POINT('Ctrl Pts',(-1.01435483510214,-2.902883513899,113.904967131782));
#29422=CARTESIAN_POINT('Ctrl Pts',(-1.10469405510182,-2.86971815972228,
113.900002869622));
#29423=CARTESIAN_POINT('Ctrl Pts',(-1.1932265144058,-2.83242170859478,113.895038607463));
#29424=CARTESIAN_POINT('Ctrl Pts',(-1.28185417451937,-2.79508515181146,
113.890069007128));
#29425=CARTESIAN_POINT('Ctrl Pts',(-1.36867078859752,-2.7536088056063,113.885099406793));
#29426=CARTESIAN_POINT('Ctrl Pts',(-1.45327446783635,-2.70820892309567,
113.880129806458));
#29427=CARTESIAN_POINT('Ctrl Pts',(-1.53793198498444,-2.66278015017769,
113.875157043697));
#29428=CARTESIAN_POINT('Ctrl Pts',(-1.62037338541075,-2.6134230987979,113.870184280936));
#29429=CARTESIAN_POINT('Ctrl Pts',(-1.70022497884624,-2.56039787363357,
113.865211518175));
#29430=CARTESIAN_POINT('Ctrl Pts',(-1.78019708483401,-2.50729262244916,
113.860231250487));
#29431=CARTESIAN_POINT('Ctrl Pts',(-1.85757122926894,-2.4505084124833,113.8552509828));
#29432=CARTESIAN_POINT('Ctrl Pts',(-1.93200631417581,-2.39034596909836,
113.850270715113));
#29433=CARTESIAN_POINT('Ctrl Pts',(-1.95378108694139,-2.37274642534332,
113.848813818847));
#29434=CARTESIAN_POINT('Ctrl Pts',(-1.97530458760304,-2.35485802645277,
113.847356922582));
#29435=CARTESIAN_POINT('Ctrl Pts',(-1.99656889110003,-2.33668887811185,
113.845900026317));
#29436=CARTESIAN_POINT('Ctrl Pts',(-2.06860404074852,-2.27513890447132,
113.84096463116));
#29437=CARTESIAN_POINT('Ctrl Pts',(-2.13792989564559,-2.21013527188959,
113.836029236003));
#29438=CARTESIAN_POINT('Ctrl Pts',(-2.20419088223709,-2.1419488333438,113.831093840846));
#29439=CARTESIAN_POINT('Ctrl Pts',(-2.27281305813786,-2.07133259261707,
113.825982574443));
#29440=CARTESIAN_POINT('Ctrl Pts',(-2.33814741676195,-1.99730269472254,
113.820871308041));
#29441=CARTESIAN_POINT('Ctrl Pts',(-2.39983504643822,-1.92020675967117,
113.815760041638));
#29442=CARTESIAN_POINT('Ctrl Pts',(-2.45925381887982,-1.845946395883,113.810836766471));
#29443=CARTESIAN_POINT('Ctrl Pts',(-2.51528907345824,-1.76884194831064,
113.805913491304));
#29444=CARTESIAN_POINT('Ctrl Pts',(-2.56765762979606,-1.68924141144777,
113.800990216137));
#29445=CARTESIAN_POINT('Ctrl Pts',(-2.61999590973637,-1.60968689490063,
113.796069787317));
#29446=CARTESIAN_POINT('Ctrl Pts',(-2.66867145318846,-1.52763953052981,
113.791149358496));
#29447=CARTESIAN_POINT('Ctrl Pts',(-2.71344297688252,-1.44347825103358,
113.786228929675));
#29448=CARTESIAN_POINT('Ctrl Pts',(-2.7582015959496,-1.35934122958862,113.781309919084));
#29449=CARTESIAN_POINT('Ctrl Pts',(-2.79905821921307,-1.273091901828,113.776390908493));
#29450=CARTESIAN_POINT('Ctrl Pts',(-2.8358169452503,-1.18513480373806,113.771471897902));
#29451=CARTESIAN_POINT('Ctrl Pts',(-2.8725757322411,-1.09717755979707,113.766552879154));
#29452=CARTESIAN_POINT('Ctrl Pts',(-2.9052364368862,-1.00751295730005,113.761633860406));
#29453=CARTESIAN_POINT('Ctrl Pts',(-2.93365132713148,-0.916565404550987,
113.756714841659));
#29454=CARTESIAN_POINT('Ctrl Pts',(-2.96208830210682,-0.825547165195897,
113.751791999732));
#29455=CARTESIAN_POINT('Ctrl Pts',(-2.98627274234399,-0.733244416947654,
113.746869157806));
#29456=CARTESIAN_POINT('Ctrl Pts',(-3.00610700087766,-0.64009604691351,
113.741946315879));
#29457=CARTESIAN_POINT('Ctrl Pts',(-3.02595053053168,-0.54690413657019,
113.737021172871));
#29458=CARTESIAN_POINT('Ctrl Pts',(-3.04143975801272,-0.452866262744185,
113.732096029862));
#29459=CARTESIAN_POINT('Ctrl Pts',(-3.05252863509209,-0.358428768296877,
113.727170886853));
#29460=CARTESIAN_POINT('Ctrl Pts',(-3.06363167096095,-0.263870691702751,
113.722239455195));
#29461=CARTESIAN_POINT('Ctrl Pts',(-3.07032311601581,-0.168912425696858,
113.717308023536));
#29462=CARTESIAN_POINT('Ctrl Pts',(-3.07260897912071,-0.0740021042050705,
113.712376591878));
#29463=CARTESIAN_POINT('Ctrl Pts',(-3.07321977859683,-0.0486413664947478,
113.711058876978));
#29464=CARTESIAN_POINT('Ctrl Pts',(-3.07351630803801,-0.0232840314320732,
113.709741162077));
#29465=CARTESIAN_POINT('Ctrl Pts',(-3.07349930869882,0.00206141404370563,
113.708423447177));
#29466=CARTESIAN_POINT('Ctrl Pts',(-3.07651118397331,0.00206343412614721,
113.708423447177));
#29467=CARTESIAN_POINT('Ctrl Pts',(-3.0775723946044,0.136145886725428,113.701459337629));
#29468=CARTESIAN_POINT('Ctrl Pts',(-3.00879601357565,1.28554760232957,113.641705592153));
#29469=CARTESIAN_POINT('Ctrl Pts',(-1.56068784542394,3.27732114239516,113.529162210748));
#29470=CARTESIAN_POINT('Ctrl Pts',(0.867539436947584,3.14804109327096,113.418010354676));
#29471=CARTESIAN_POINT('Ctrl Pts',(1.79005390196206,2.5061803198351,113.359648134531));
#29472=CARTESIAN_POINT('Ctrl Pts',(1.8746157427793,2.44019679077305,113.354075550313));
#29473=CARTESIAN_POINT('Origin',(0.,0.,104.));
#29474=CARTESIAN_POINT('',(-2.36143112101026,0.872610629504498,95.3311773795575));
#29475=CARTESIAN_POINT('',(-2.3614311210294,0.872610629452704,95.0532830566435));
#29476=CARTESIAN_POINT('',(-2.36143112101026,0.872610629504505,104.));
#29477=CARTESIAN_POINT('',(-1.91346599666497,1.63598720337506,95.));
#29478=CARTESIAN_POINT('Ctrl Pts',(-2.36143112104854,0.872610629400893,
95.0532830566435));
#29479=CARTESIAN_POINT('Ctrl Pts',(-2.31579433560925,0.996111446111038,
95.0453131407852));
#29480=CARTESIAN_POINT('Ctrl Pts',(-2.26053801495448,1.11584628337841,95.0375896339826));
#29481=CARTESIAN_POINT('Ctrl Pts',(-2.13200539566163,1.34520787555974,95.0221295983418));
#29482=CARTESIAN_POINT('Ctrl Pts',(-2.05899555128104,1.45449729498176,95.0144128937844));
#29483=CARTESIAN_POINT('Ctrl Pts',(-1.96578302134751,1.57285764443762,95.0051301889263));
#29484=CARTESIAN_POINT('Ctrl Pts',(-1.95358099596075,1.58798781731369,95.0039247102501));
#29485=CARTESIAN_POINT('Ctrl Pts',(-1.93616947814021,1.60907319677807,95.0022158593805));
#29486=CARTESIAN_POINT('Ctrl Pts',(-1.93110497507636,1.61514778668851,95.0017201146326));
#29487=CARTESIAN_POINT('Ctrl Pts',(-1.92184895461832,1.62614410096873,95.0008162608354));
#29488=CARTESIAN_POINT('Ctrl Pts',(-1.91766692397879,1.6310737593378,95.0004086818932));
#29489=CARTESIAN_POINT('Ctrl Pts',(-1.91346599666497,1.63598720337506,95.));
#29490=CARTESIAN_POINT('',(-2.36143112101026,0.872610629504506,95.));
#29491=CARTESIAN_POINT('Origin',(0.,0.,95.));
#29492=CARTESIAN_POINT('',(-2.36143112101026,0.872610629504505,94.));
#29493=CARTESIAN_POINT('',(-2.36143112101026,0.872610629504505,104.));
#29494=CARTESIAN_POINT('Origin',(0.,0.,94.));
#29495=CARTESIAN_POINT('',(1.91365527685913,1.63576579355029,95.0000017045188));
#29496=CARTESIAN_POINT('Origin',(0.,0.,95.));
#29497=CARTESIAN_POINT('Ctrl Pts',(1.91365527685913,1.63576579355029,95.0000017045188));
#29498=CARTESIAN_POINT('Ctrl Pts',(1.86017230240225,1.69833463848829,95.0052371659376));
#29499=CARTESIAN_POINT('Ctrl Pts',(1.80351517637209,1.75839729036196,95.0104726273563));
#29500=CARTESIAN_POINT('Ctrl Pts',(1.74394864222121,1.81561267435948,95.0157080887751));
#29501=CARTESIAN_POINT('Ctrl Pts',(1.68446655011802,1.87274694932065,95.0209361283573));
#29502=CARTESIAN_POINT('Ctrl Pts',(1.62208357330082,1.92704165258672,95.0261641679395));
#29503=CARTESIAN_POINT('Ctrl Pts',(1.55710418779672,1.97818927262937,95.0313922075217));
#29504=CARTESIAN_POINT('Ctrl Pts',(1.49219891201617,2.0292785582333,95.0366142844656));
#29505=CARTESIAN_POINT('Ctrl Pts',(1.424703476094,2.07722760724393,95.0418363614096));
#29506=CARTESIAN_POINT('Ctrl Pts',(1.35495753679941,2.12176726420936,95.0470584383535));
#29507=CARTESIAN_POINT('Ctrl Pts',(1.2852548997391,2.16627926842998,95.052277273136));
#29508=CARTESIAN_POINT('Ctrl Pts',(1.21330492382474,2.20738583238343,95.0574961079185));
#29509=CARTESIAN_POINT('Ctrl Pts',(1.13947758010576,2.24486015030699,95.0627149427009));
#29510=CARTESIAN_POINT('Ctrl Pts',(1.06567335706128,2.28232273231452,95.0679321430892));
#29511=CARTESIAN_POINT('Ctrl Pts',(0.989993348399747,2.3161551167964,95.0731493434775));
#29512=CARTESIAN_POINT('Ctrl Pts',(0.912832280854548,2.34617635249993,95.0783665438658));
#29513=CARTESIAN_POINT('Ctrl Pts',(0.835671637012119,2.37619742335244,95.0835837156057));
#29514=CARTESIAN_POINT('Ctrl Pts',(0.75703038467285,2.40240721980204,95.0888008873455));
#29515=CARTESIAN_POINT('Ctrl Pts',(0.677322039911264,2.42467340156369,95.0940180590854));
#29516=CARTESIAN_POINT('Ctrl Pts',(0.597536860009014,2.44696104688996,95.0992402599364));
#29517=CARTESIAN_POINT('Ctrl Pts',(0.516682982388146,2.46529735964048,95.1044624607874));
#29518=CARTESIAN_POINT('Ctrl Pts',(0.435187289079247,2.47960042616222,95.1096846616385));
#29519=CARTESIAN_POINT('Ctrl Pts',(0.353652247998477,2.49391039849426,95.1149093838738));
#29520=CARTESIAN_POINT('Ctrl Pts',(0.271475236215456,2.50418318862084,95.1201341061092));
#29521=CARTESIAN_POINT('Ctrl Pts',(0.18908902819608,2.51038873272963,95.1253588283446));
#29522=CARTESIAN_POINT('Ctrl Pts',(0.106561009261774,2.51660495840646,95.1305925438649));
#29523=CARTESIAN_POINT('Ctrl Pts',(0.023823540639689,2.5187399408743,95.1358262593852));
#29524=CARTESIAN_POINT('Ctrl Pts',(-0.0586900854461119,2.51681579061129,
95.1410599749055));
#29525=CARTESIAN_POINT('Ctrl Pts',(-0.12721868487804,2.5152177597299,95.1454066411647));
#29526=CARTESIAN_POINT('Ctrl Pts',(-0.195592795310752,2.51082090606575,
95.1497533074239));
#29527=CARTESIAN_POINT('Ctrl Pts',(-0.263568565194451,2.50366488601037,
95.1540999736831));
#29528=CARTESIAN_POINT('Ctrl Pts',(-0.345886810085939,2.4949989891419,95.1593637601499));
#29529=CARTESIAN_POINT('Ctrl Pts',(-0.427923601593685,2.4822535690543,95.1646275466167));
#29530=CARTESIAN_POINT('Ctrl Pts',(-0.509243989845148,2.46545671404034,
95.1698913330835));
#29531=CARTESIAN_POINT('Ctrl Pts',(-0.59045192433296,2.4486830865294,95.175147840532));
#29532=CARTESIAN_POINT('Ctrl Pts',(-0.670944976960685,2.42786924586806,
95.1804043479804));
#29533=CARTESIAN_POINT('Ctrl Pts',(-0.750293725218741,2.40309499934925,
95.1856608554289));
#29534=CARTESIAN_POINT('Ctrl Pts',(-0.830052467389669,2.37819274463257,
95.1909445231805));
#29535=CARTESIAN_POINT('Ctrl Pts',(-0.908654577485922,2.34928908694531,
95.1962281909321));
#29536=CARTESIAN_POINT('Ctrl Pts',(-0.985674728067885,2.31651712284807,
95.2015118586837));
#29537=CARTESIAN_POINT('Ctrl Pts',(-1.06216749166448,2.28396956116006,95.2067593471032));
#29538=CARTESIAN_POINT('Ctrl Pts',(-1.13709946505231,2.24760668753531,95.2120068355227));
#29539=CARTESIAN_POINT('Ctrl Pts',(-1.21007126184921,2.207608160713,95.2172543239422));
#29540=CARTESIAN_POINT('Ctrl Pts',(-1.28302066508639,2.16762190862475,95.2225002020142));
#29541=CARTESIAN_POINT('Ctrl Pts',(-1.35401068378094,2.12400244024195,95.2277460800863));
#29542=CARTESIAN_POINT('Ctrl Pts',(-1.42266586687652,2.07697570549693,95.2329919581583));
#29543=CARTESIAN_POINT('Ctrl Pts',(-1.49132049147426,2.02994935330614,95.2382377935561));
#29544=CARTESIAN_POINT('Ctrl Pts',(-1.55763993968314,1.97951605058171,95.2434836289539));
#29545=CARTESIAN_POINT('Ctrl Pts',(-1.62127827210285,1.92594470699633,95.2487294643516));
#29546=CARTESIAN_POINT('Ctrl Pts',(-1.68571462823238,1.8717015795863,95.2540410824446));
#29547=CARTESIAN_POINT('Ctrl Pts',(-1.74740177712543,1.81424145821353,95.2593527005376));
#29548=CARTESIAN_POINT('Ctrl Pts',(-1.80601705811497,1.75388387181071,95.2646643186305));
#29549=CARTESIAN_POINT('Ctrl Pts',(-1.86399106750709,1.69418661843362,95.2699178257708));
#29550=CARTESIAN_POINT('Ctrl Pts',(-1.91895983457342,1.63165537912202,95.2751713329111));
#29551=CARTESIAN_POINT('Ctrl Pts',(-1.97065124961128,1.56663330183087,95.2804248400514));
#29552=CARTESIAN_POINT('Ctrl Pts',(-2.02320033095449,1.50053237528099,95.2857655136207));
#29553=CARTESIAN_POINT('Ctrl Pts',(-2.07236202720979,1.43185760662661,95.2911061871901));
#29554=CARTESIAN_POINT('Ctrl Pts',(-2.11789688966922,1.36099927065721,95.2964468607594));
#29555=CARTESIAN_POINT('Ctrl Pts',(-2.16343175212864,1.29014093468782,95.3017875343287));
#29556=CARTESIAN_POINT('Ctrl Pts',(-2.20533959179403,1.2170994902856,95.307128207898));
#29557=CARTESIAN_POINT('Ctrl Pts',(-2.24343108861944,1.14228858027024,95.3124688814673));
#29558=CARTESIAN_POINT('Ctrl Pts',(-2.28325410804496,1.06407699576786,95.3180523256746));
#29559=CARTESIAN_POINT('Ctrl Pts',(-2.31903886419149,0.983671855279027,
95.3236357698818));
#29560=CARTESIAN_POINT('Ctrl Pts',(-2.3505537867259,0.901500496787727,95.3292192140891));
#29561=CARTESIAN_POINT('Ctrl Pts',(-2.35423797822459,0.891894411922428,
95.3298719359119));
#29562=CARTESIAN_POINT('Ctrl Pts',(-2.35786386636583,0.882264220521029,
95.3305246577347));
#29563=CARTESIAN_POINT('Ctrl Pts',(-2.36143112101026,0.872610629504497,
95.3311773795575));
#29564=CARTESIAN_POINT('Origin',(0.,0.,104.));
#29565=CARTESIAN_POINT('',(-2.35791364508473,0.871329681353405,96.3311375631035));
#29566=CARTESIAN_POINT('',(-2.36143112101026,0.872610629504502,96.0561753867426));
#29567=CARTESIAN_POINT('',(-2.36143112101026,0.872610629504505,104.));
#29568=CARTESIAN_POINT('',(-2.51749766382103,-0.00342967281893025,95.1125851160815));
#29569=CARTESIAN_POINT('Ctrl Pts',(-2.36143112101026,0.872610629504502,
96.0561753867426));
#29570=CARTESIAN_POINT('Ctrl Pts',(-2.33265141387007,0.950493357260157,
96.0509366716251));
#29571=CARTESIAN_POINT('Ctrl Pts',(-2.29999690568281,1.02699878203394,96.0456979565076));
#29572=CARTESIAN_POINT('Ctrl Pts',(-2.26362920233033,1.10172096483518,96.0404592413902));
#29573=CARTESIAN_POINT('Ctrl Pts',(-2.22727000798159,1.17642566478007,96.0352217519824));
#29574=CARTESIAN_POINT('Ctrl Pts',(-2.18719954614185,1.24934753707113,96.0299842625746));
#29575=CARTESIAN_POINT('Ctrl Pts',(-2.14362668723944,1.32010260046516,96.0247467731668));
#29576=CARTESIAN_POINT('Ctrl Pts',(-2.10005089320364,1.39086243002679,96.0195089309538));
#29577=CARTESIAN_POINT('Ctrl Pts',(-2.05297247670035,1.45945476887936,96.0142710887409));
#29578=CARTESIAN_POINT('Ctrl Pts',(-2.00264446347711,1.5255233209966,96.0090332465279));
#29579=CARTESIAN_POINT('Ctrl Pts',(-1.95226457423269,1.59165997382732,96.0037900053652));
#29580=CARTESIAN_POINT('Ctrl Pts',(-1.89862867988026,1.65526727771402,95.9985467642025));
#29581=CARTESIAN_POINT('Ctrl Pts',(-1.84203073908618,1.71602127208891,95.9933035230399));
#29582=CARTESIAN_POINT('Ctrl Pts',(-1.78540246993703,1.77680782186576,95.9880574722541));
#29583=CARTESIAN_POINT('Ctrl Pts',(-1.72580932439884,1.83473769565866,95.9828114214684));
#29584=CARTESIAN_POINT('Ctrl Pts',(-1.66358109354304,1.88952485964227,95.9775653706826));
#29585=CARTESIAN_POINT('Ctrl Pts',(-1.60124600512162,1.94440610348145,95.9723103114419));
#29586=CARTESIAN_POINT('Ctrl Pts',(-1.5362671547045,1.99613357105326,95.9670552522011));
#29587=CARTESIAN_POINT('Ctrl Pts',(-1.46900605360172,2.04446263465036,95.9618001929604));
#29588=CARTESIAN_POINT('Ctrl Pts',(-1.41957195745204,2.07998247505607,95.9579379442086));
#29589=CARTESIAN_POINT('Ctrl Pts',(-1.36890572652446,2.11366750477514,95.9540756954568));
#29590=CARTESIAN_POINT('Ctrl Pts',(-1.31715930479627,2.1454364627713,95.950213446705));
#29591=CARTESIAN_POINT('Ctrl Pts',(-1.24673646073771,2.18867153681405,95.9449572273863));
#29592=CARTESIAN_POINT('Ctrl Pts',(-1.17405304514657,2.22851509199812,95.9397010080676));
#29593=CARTESIAN_POINT('Ctrl Pts',(-1.09946919902374,2.26472376470026,95.9344447887488));
#29594=CARTESIAN_POINT('Ctrl Pts',(-1.02499086952048,2.30088121160832,95.9291960056046));
#29595=CARTESIAN_POINT('Ctrl Pts',(-0.948617861385659,2.33341379073347,
95.9239472224604));
#29596=CARTESIAN_POINT('Ctrl Pts',(-0.870737623933377,2.36212240162674,
95.9186984393161));
#29597=CARTESIAN_POINT('Ctrl Pts',(-0.792311415316317,2.39103227119924,
95.913412860133));
#29598=CARTESIAN_POINT('Ctrl Pts',(-0.712357162115909,2.41606409095858,
95.9081272809498));
#29599=CARTESIAN_POINT('Ctrl Pts',(-0.631294033309228,2.43706259532006,
95.9028417017667));
#29600=CARTESIAN_POINT('Ctrl Pts',(-0.550938551744799,2.4578777915127,95.8976022634813));
#29601=CARTESIAN_POINT('Ctrl Pts',(-0.469493933549941,2.47472969831333,
95.8923628251958));
#29602=CARTESIAN_POINT('Ctrl Pts',(-0.387384999349596,2.48751665567869,
95.8871233869104));
#29603=CARTESIAN_POINT('Ctrl Pts',(-0.305302936472543,2.50029942832934,
95.8818856633061));
#29604=CARTESIAN_POINT('Ctrl Pts',(-0.222557444742411,2.50901982274132,
95.8766479397017));
#29605=CARTESIAN_POINT('Ctrl Pts',(-0.139582707846034,2.51362744209844,
95.8714102160974));
#29606=CARTESIAN_POINT('Ctrl Pts',(-0.056610124402918,2.51823494187347,
95.8661726284284));
#29607=CARTESIAN_POINT('Ctrl Pts',(0.026591231815042,2.51872985428838,95.8609350407593));
#29608=CARTESIAN_POINT('Ctrl Pts',(0.109584284531156,2.51511382139731,95.8556974530903));
#29609=CARTESIAN_POINT('Ctrl Pts',(0.193900268125644,2.51144014800006,95.8503763769095));
#29610=CARTESIAN_POINT('Ctrl Pts',(0.278000758163298,2.50352332510973,95.8450553007287));
#29611=CARTESIAN_POINT('Ctrl Pts',(0.361431683604489,2.49141995418011,95.8397342245479));
#29612=CARTESIAN_POINT('Ctrl Pts',(0.443671569616648,2.47948936800537,95.8344891107456));
#29613=CARTESIAN_POINT('Ctrl Pts',(0.525260437824858,2.4634911463882,95.8292439969433));
#29614=CARTESIAN_POINT('Ctrl Pts',(0.605774396105066,2.44353097607203,95.823998883141));
#29615=CARTESIAN_POINT('Ctrl Pts',(0.688037419897433,2.42313719590408,95.818639825771));
#29616=CARTESIAN_POINT('Ctrl Pts',(0.769177794999873,2.39860745724191,95.813280768401));
#29617=CARTESIAN_POINT('Ctrl Pts',(0.848762379063284,2.37010731273646,95.8079217110309));
#29618=CARTESIAN_POINT('Ctrl Pts',(0.928346963126706,2.341607168231,95.8025626536609));
#29619=CARTESIAN_POINT('Ctrl Pts',(1.00637531423859,2.30913687376708,95.7972035962909));
#29620=CARTESIAN_POINT('Ctrl Pts',(1.08244033181905,2.27291204802374,95.7918445389208));
#29621=CARTESIAN_POINT('Ctrl Pts',(1.15694499484728,2.23743031777356,95.7865954142088));
#29622=CARTESIAN_POINT('Ctrl Pts',(1.22984274428871,2.19821491727435,95.7813462894968));
#29623=CARTESIAN_POINT('Ctrl Pts',(1.30073401346762,2.15543435905815,95.7760971647847));
#29624=CARTESIAN_POINT('Ctrl Pts',(1.37152445649355,2.11271464612172,95.7708555057177));
#29625=CARTESIAN_POINT('Ctrl Pts',(1.44031369453238,2.06644008345905,95.7656138466507));
#29626=CARTESIAN_POINT('Ctrl Pts',(1.50672433125253,2.01682622940391,95.7603721875837));
#29627=CARTESIAN_POINT('Ctrl Pts',(1.57371394436528,1.9667798354476,95.7550848310651));
#29628=CARTESIAN_POINT('Ctrl Pts',(1.63828284277624,1.91333583623313,95.7497974745464));
#29629=CARTESIAN_POINT('Ctrl Pts',(1.70007126986955,1.85676167758927,95.7445101180278));
#29630=CARTESIAN_POINT('Ctrl Pts',(1.76121623418599,1.80077668049124,95.7392778238771));
#29631=CARTESIAN_POINT('Ctrl Pts',(1.81963802047758,1.74172673474641,95.7340455297265));
#29632=CARTESIAN_POINT('Ctrl Pts',(1.87502056171392,1.67991194505844,95.7288132355758));
#29633=CARTESIAN_POINT('Ctrl Pts',(1.9303850390111,1.61811731729469,95.7235826480251));
#29634=CARTESIAN_POINT('Ctrl Pts',(1.98271193141133,1.55355998075114,95.7183520604744));
#29635=CARTESIAN_POINT('Ctrl Pts',(2.03172305193611,1.48657582727267,95.7131214729237));
#29636=CARTESIAN_POINT('Ctrl Pts',(2.08073306299572,1.41959319011508,95.7078910037779));
#29637=CARTESIAN_POINT('Ctrl Pts',(2.12642717908222,1.35018421921784,95.702660534632));
#29638=CARTESIAN_POINT('Ctrl Pts',(2.16856928100672,1.27871557567507,95.6974300654862));
#29639=CARTESIAN_POINT('Ctrl Pts',(2.21150957016828,1.20589328918329,95.6921005292904));
#29640=CARTESIAN_POINT('Ctrl Pts',(2.25076163563882,1.130932923186,95.6867709930946));
#29641=CARTESIAN_POINT('Ctrl Pts',(2.28612453916548,1.05424894660863,95.6814414568988));
#29642=CARTESIAN_POINT('Ctrl Pts',(2.32088080922383,0.978880446477947,95.676203346313));
#29643=CARTESIAN_POINT('Ctrl Pts',(2.35188018984607,0.90184746780268,95.6709652357273));
#29644=CARTESIAN_POINT('Ctrl Pts',(2.378981170246,0.823562287635228,95.6657271251415));
#29645=CARTESIAN_POINT('Ctrl Pts',(2.40679167852567,0.743227531508555,95.6603518761407));
#29646=CARTESIAN_POINT('Ctrl Pts',(2.43049665313458,0.66157458996074,95.6549766271399));
#29647=CARTESIAN_POINT('Ctrl Pts',(2.44999868103596,0.579061924945903,95.6496013781391));
#29648=CARTESIAN_POINT('Ctrl Pts',(2.46950070893734,0.496549259931055,95.6442261291383));
#29649=CARTESIAN_POINT('Ctrl Pts',(2.48479976500474,0.413177394251107,95.6388508801375));
#29650=CARTESIAN_POINT('Ctrl Pts',(2.4958556042303,0.329410158969318,95.6334756311367));
#29651=CARTESIAN_POINT('Ctrl Pts',(2.50668406766696,0.247365691251163,95.6282109301873));
#29652=CARTESIAN_POINT('Ctrl Pts',(2.51348245591912,0.164637609670783,95.6229462292378));
#29653=CARTESIAN_POINT('Ctrl Pts',(2.51617541011446,0.0816551010979545,
95.6176815282883));
#29654=CARTESIAN_POINT('Ctrl Pts',(2.51886454077522,-0.00120958649902303,
95.6124243023141));
#29655=CARTESIAN_POINT('Ctrl Pts',(2.51745980182278,-0.0843275278565643,
95.60716707634));
#29656=CARTESIAN_POINT('Ctrl Pts',(2.51193738922762,-0.167262675454818,
95.6019098503658));
#29657=CARTESIAN_POINT('Ctrl Pts',(2.50638741549332,-0.250611734021007,
95.5966263867403));
#29658=CARTESIAN_POINT('Ctrl Pts',(2.49667848808217,-0.333775703050781,
95.5913429231147));
#29659=CARTESIAN_POINT('Ctrl Pts',(2.48283953433707,-0.41631009684233,95.5860594594891));
#29660=CARTESIAN_POINT('Ctrl Pts',(2.46909418980429,-0.498286212910473,
95.5808117341771));
#29661=CARTESIAN_POINT('Ctrl Pts',(2.45127459572428,-0.579640785447499,
95.5755640088651));
#29662=CARTESIAN_POINT('Ctrl Pts',(2.42946105419747,-0.659943358279883,
95.5703162835531));
#29663=CARTESIAN_POINT('Ctrl Pts',(2.40765495986179,-0.740218515636984,
95.5650703498261));
#29664=CARTESIAN_POINT('Ctrl Pts',(2.38185774685792,-0.819441943492977,
95.5598244160991));
#29665=CARTESIAN_POINT('Ctrl Pts',(2.35220035334611,-0.897195490246381,
95.5545784823721));
#29666=CARTESIAN_POINT('Ctrl Pts',(2.32254422495082,-0.974945720211436,
95.5493327724246));
#29667=CARTESIAN_POINT('Ctrl Pts',(2.28902840815539,-1.05122576465178,95.5440870624771));
#29668=CARTESIAN_POINT('Ctrl Pts',(2.25183256125782,-1.12563598292657,95.5388413525296));
#29669=CARTESIAN_POINT('Ctrl Pts',(2.21417220748495,-1.2009754462882,95.5335301334315));
#29670=CARTESIAN_POINT('Ctrl Pts',(2.17273947002901,-1.27439761774384,95.5282189143334));
#29671=CARTESIAN_POINT('Ctrl Pts',(2.12776869285796,-1.34551352267212,95.5229076952353));
#29672=CARTESIAN_POINT('Ctrl Pts',(2.08329138828702,-1.4158490597099,95.5176547571202));
#29673=CARTESIAN_POINT('Ctrl Pts',(2.03535362741242,-1.48392835009897,95.512401819005));
#29674=CARTESIAN_POINT('Ctrl Pts',(1.98422465432488,-1.54940594137537,95.5071488808899));
#29675=CARTESIAN_POINT('Ctrl Pts',(1.93224477263797,-1.6159732366321,95.5018085213003));
#29676=CARTESIAN_POINT('Ctrl Pts',(1.87696681445754,-1.67985107003741,95.4964681617107));
#29677=CARTESIAN_POINT('Ctrl Pts',(1.81871363381257,-1.74071449933189,95.4911278021212));
#29678=CARTESIAN_POINT('Ctrl Pts',(1.76046045316761,-1.80157792862636,95.4857874425316));
#29679=CARTESIAN_POINT('Ctrl Pts',(1.69923245075008,-1.85942666068594,95.480447082942));
#29680=CARTESIAN_POINT('Ctrl Pts',(1.63538709547285,-1.91397891784651,95.4751067233524));
#29681=CARTESIAN_POINT('Ctrl Pts',(1.57250694959504,-1.96770645798353,95.4698470989275));
#29682=CARTESIAN_POINT('Ctrl Pts',(1.50686280030885,-2.01842901296663,95.4645874745026));
#29683=CARTESIAN_POINT('Ctrl Pts',(1.4387734646105,-2.06585022872731,95.4593278500777));
#29684=CARTESIAN_POINT('Ctrl Pts',(1.37077917835537,-2.1132052467478,95.454075567836));
#29685=CARTESIAN_POINT('Ctrl Pts',(1.30034686084804,-2.15726781899979,95.4488232855942));
#29686=CARTESIAN_POINT('Ctrl Pts',(1.22782911905335,-2.1977811320522,95.4435710033524));
#29687=CARTESIAN_POINT('Ctrl Pts',(1.15486356538724,-2.23854462308984,95.4382862871948));
#29688=CARTESIAN_POINT('Ctrl Pts',(1.07978709863394,-2.27571455706946,95.4330015710371));
#29689=CARTESIAN_POINT('Ctrl Pts',(1.0029894234992,-2.30907307514265,95.4277168548794));
#29690=CARTESIAN_POINT('Ctrl Pts',(0.9267959794547,-2.34216913405014,95.4224737179727));
#29691=CARTESIAN_POINT('Ctrl Pts',(0.848908745038345,-2.37151335508,95.417230581066));
#29692=CARTESIAN_POINT('Ctrl Pts',(0.769732253879452,-2.39693940418561,
95.4119874441592));
#29693=CARTESIAN_POINT('Ctrl Pts',(0.690580662639252,-2.4223574571481,95.406745956147));
#29694=CARTESIAN_POINT('Ctrl Pts',(0.610141058004238,-2.44385964492363,
95.4015044681348));
#29695=CARTESIAN_POINT('Ctrl Pts',(0.528835141361276,-2.46132883688088,
95.3962629801226));
#29696=CARTESIAN_POINT('Ctrl Pts',(0.447530402502071,-2.47879777578237,
95.3910215680377));
#29697=CARTESIAN_POINT('Ctrl Pts',(0.365359826960715,-2.49223373940727,
95.3857801559528));
#29698=CARTESIAN_POINT('Ctrl Pts',(0.282756021243529,-2.50157056315638,
95.3805387438679));
#29699=CARTESIAN_POINT('Ctrl Pts',(0.198964996349559,-2.51104157995034,
95.3752219998429));
#29700=CARTESIAN_POINT('Ctrl Pts',(0.114728671082748,-2.51629461967136,
95.3699052558179));
#29701=CARTESIAN_POINT('Ctrl Pts',(0.0305028474469036,-2.51731520201536,
95.364588511793));
#29702=CARTESIAN_POINT('Ctrl Pts',(-0.0526504958620326,-2.51832278888554,
95.3593394679474));
#29703=CARTESIAN_POINT('Ctrl Pts',(-0.135793139660068,-2.51520516872692,
95.3540904241019));
#29704=CARTESIAN_POINT('Ctrl Pts',(-0.218489369668261,-2.50800092610469,
95.3488413802563));
#29705=CARTESIAN_POINT('Ctrl Pts',(-0.302785476655478,-2.50065730709346,
95.3434907861416));
#29706=CARTESIAN_POINT('Ctrl Pts',(-0.386617216445367,-2.48906734892347,
95.338140192027));
#29707=CARTESIAN_POINT('Ctrl Pts',(-0.469533550827451,-2.47332660492855,
95.3327895979123));
#29708=CARTESIAN_POINT('Ctrl Pts',(-0.552449885209547,-2.45758586093362,
95.3274390037977));
#29709=CARTESIAN_POINT('Ctrl Pts',(-0.634450344179456,-2.4376945126903,
95.322088409683));
#29710=CARTESIAN_POINT('Ctrl Pts',(-0.715101646661369,-2.4138011278774,
95.3167378155684));
#29711=CARTESIAN_POINT('Ctrl Pts',(-0.793553864869304,-2.39055923368122,
95.3115331137953));
#29712=CARTESIAN_POINT('Ctrl Pts',(-0.871032543613655,-2.3634408582058,
95.3063284120223));
#29713=CARTESIAN_POINT('Ctrl Pts',(-0.947121846064168,-2.33254506038104,
95.3011237102492));
#29714=CARTESIAN_POINT('Ctrl Pts',(-1.02310194916727,-2.30169360257323,
95.2959264779893));
#29715=CARTESIAN_POINT('Ctrl Pts',(-1.09769620193994,-2.2670756598159,95.2907292457293));
#29716=CARTESIAN_POINT('Ctrl Pts',(-1.17050286371611,-2.22884034781148,
95.2855320134693));
#29717=CARTESIAN_POINT('Ctrl Pts',(-1.24472763665675,-2.18986029732424,
95.2802335507324));
#29718=CARTESIAN_POINT('Ctrl Pts',(-1.31709396224004,-2.14712059290674,
95.2749350879955));
#29719=CARTESIAN_POINT('Ctrl Pts',(-1.38719665267716,-2.10083119188603,
95.2696366252586));
#29720=CARTESIAN_POINT('Ctrl Pts',(-1.45583983912076,-2.05550551372996,
95.2644484739445));
#29721=CARTESIAN_POINT('Ctrl Pts',(-1.52231232778246,-2.0067767973796,95.2592603226305));
#29722=CARTESIAN_POINT('Ctrl Pts',(-1.5862594930535,-1.95488799441238,95.2540721713164));
#29723=CARTESIAN_POINT('Ctrl Pts',(-1.65018796402017,-1.90301436060977,
95.2488855367056));
#29724=CARTESIAN_POINT('Ctrl Pts',(-1.71159221114548,-1.84798277033845,
95.2436989020949));
#29725=CARTESIAN_POINT('Ctrl Pts',(-1.77014939416049,-1.79007747663425,
95.2385122674842));
#29726=CARTESIAN_POINT('Ctrl Pts',(-1.8287079575656,-1.73217081790718,95.233325510607));
#29727=CARTESIAN_POINT('Ctrl Pts',(-1.8844189893606,-1.67139065339286,95.2281387537298));
#29728=CARTESIAN_POINT('Ctrl Pts',(-1.93699644193566,-1.60805815626444,
95.2229519968526));
#29729=CARTESIAN_POINT('Ctrl Pts',(-1.9915522781266,-1.54234258486113,95.2175700727636));
#29730=CARTESIAN_POINT('Ctrl Pts',(-2.04273367412091,-1.47387920327015,
95.2121881486745));
#29731=CARTESIAN_POINT('Ctrl Pts',(-2.09026826242715,-1.40306266470524,
95.2068062245855));
#29732=CARTESIAN_POINT('Ctrl Pts',(-2.13615558916376,-1.33470019940844,
95.2016108054613));
#29733=CARTESIAN_POINT('Ctrl Pts',(-2.1786445252822,-1.2641454407714,95.1964153863372));
#29734=CARTESIAN_POINT('Ctrl Pts',(-2.21753644921349,-1.19177948732542,
95.191219967213));
#29735=CARTESIAN_POINT('Ctrl Pts',(-2.2564599203922,-1.11935483411846,95.1860203338162));
#29736=CARTESIAN_POINT('Ctrl Pts',(-2.29178037823891,-1.04511648975722,
95.1808207004193));
#29737=CARTESIAN_POINT('Ctrl Pts',(-2.32334730809328,-0.969465592981872,
95.1756210670225));
#29738=CARTESIAN_POINT('Ctrl Pts',(-2.3549680583398,-0.893685714359086,
95.1704125684522));
#29739=CARTESIAN_POINT('Ctrl Pts',(-2.38282236627793,-0.816488923342303,
95.1652040698819));
#29740=CARTESIAN_POINT('Ctrl Pts',(-2.40680970688121,-0.738290786115048,
95.1599955713116));
#29741=CARTESIAN_POINT('Ctrl Pts',(-2.40930686491077,-0.730150112686395,
95.1594533501358));
#29742=CARTESIAN_POINT('Ctrl Pts',(-2.41176216078532,-0.721998594537591,
95.15891112896));
#29743=CARTESIAN_POINT('Ctrl Pts',(-2.41417551320215,-0.713836705034951,
95.1583689077841));
#29744=CARTESIAN_POINT('Ctrl Pts',(-2.44522521635681,-0.608827488614062,
95.1513928000114));
#29745=CARTESIAN_POINT('Ctrl Pts',(-2.46942455892676,-0.501773885157136,
95.1444166922386));
#29746=CARTESIAN_POINT('Ctrl Pts',(-2.48656498776096,-0.393447342907944,
95.1374405844659));
#29747=CARTESIAN_POINT('Ctrl Pts',(-2.50328860943498,-0.287754998372505,
95.1306341160702));
#29748=CARTESIAN_POINT('Ctrl Pts',(-2.51329252836617,-0.180850497788633,
95.1238276476745));
#29749=CARTESIAN_POINT('Ctrl Pts',(-2.51642765153617,-0.0734719305866939,
95.1170211792788));
#29750=CARTESIAN_POINT('Ctrl Pts',(-2.51710874897196,-0.050144213360273,
95.1155424915463));
#29751=CARTESIAN_POINT('Ctrl Pts',(-2.51746583350749,-0.0267942163812354,
95.1140638038139));
#29752=CARTESIAN_POINT('Ctrl Pts',(-2.51749766382103,-0.00342967281893025,
95.1125851160815));
#29753=CARTESIAN_POINT('Ctrl Pts',(-2.51749757130744,-0.00349692166510488,
95.1115697988903));
#29754=CARTESIAN_POINT('Ctrl Pts',(-2.51766860658887,0.119634491284325,
95.1030512768662));
#29755=CARTESIAN_POINT('Ctrl Pts',(-2.50880598011611,0.242625205407994,
95.0946581244734));
#29756=CARTESIAN_POINT('Ctrl Pts',(-2.48347800210713,0.415721636410033,
95.0830838099193));
#29757=CARTESIAN_POINT('Ctrl Pts',(-2.47440185369426,0.466715694875851,
95.0797022152716));
#29758=CARTESIAN_POINT('Ctrl Pts',(-2.46015542500379,0.534554887518458,
95.0752365418874));
#29759=CARTESIAN_POINT('Ctrl Pts',(-2.45637290771386,0.551675452432403,
95.0741123445084));
#29760=CARTESIAN_POINT('Ctrl Pts',(-2.44948335309491,0.581382464738478,
95.0721661139171));
#29761=CARTESIAN_POINT('Ctrl Pts',(-2.4464574163654,0.593986857357515,95.0713417440849));
#29762=CARTESIAN_POINT('Ctrl Pts',(-2.44017548710644,0.619291300554413,
95.0696893113859));
#29763=CARTESIAN_POINT('Ctrl Pts',(-2.43691736707658,0.631990410057167,
95.0688613392206));
#29764=CARTESIAN_POINT('Ctrl Pts',(-2.43050098128503,0.656211816588521,
95.0672843425808));
#29765=CARTESIAN_POINT('Ctrl Pts',(-2.42735961356931,0.667738183509839,
95.0665348553807));
#29766=CARTESIAN_POINT('Ctrl Pts',(-2.41897310744704,0.697668660180833,
95.0645908614003));
#29767=CARTESIAN_POINT('Ctrl Pts',(-2.41359990664641,0.716036292656748,
95.0634000524792));
#29768=CARTESIAN_POINT('Ctrl Pts',(-2.39410128500123,0.779975268331027,
95.0592603824716));
#29769=CARTESIAN_POINT('Ctrl Pts',(-2.37888995878851,0.825206231053676,
95.0563421777975));
#29770=CARTESIAN_POINT('Ctrl Pts',(-2.36207867090852,0.870856748450194,
95.053396239938));
#29771=CARTESIAN_POINT('Ctrl Pts',(-2.36175513843305,0.871733783864357,
95.0533396423838));
#29772=CARTESIAN_POINT('Ctrl Pts',(-2.36143112104854,0.872610629400897,
95.0532830566435));
#29773=CARTESIAN_POINT('',(-2.51439859764413,0.000444055452618797,95.387416697508));
#29774=CARTESIAN_POINT('Ctrl Pts',(-2.36143112101026,0.872610629504497,
95.3311773795575));
#29775=CARTESIAN_POINT('Ctrl Pts',(-2.39184210810317,0.790313383844522,
95.336741858942));
#29776=CARTESIAN_POINT('Ctrl Pts',(-2.4179880049747,0.706313645512247,95.3423063383265));
#29777=CARTESIAN_POINT('Ctrl Pts',(-2.43969002558945,0.62106266112154,95.347870817711));
#29778=CARTESIAN_POINT('Ctrl Pts',(-2.46134996455353,0.535976984017515,
95.3534245072026));
#29779=CARTESIAN_POINT('Ctrl Pts',(-2.47858308353986,0.449645249570044,
95.3589781966942));
#29780=CARTESIAN_POINT('Ctrl Pts',(-2.49125949193803,0.362536058659951,
95.3645318861859));
#29781=CARTESIAN_POINT('Ctrl Pts',(-2.50390335952531,0.275650480276184,
95.3700713191504));
#29782=CARTESIAN_POINT('Ctrl Pts',(-2.51201376412536,0.187991789932431,
95.375610752115));
#29783=CARTESIAN_POINT('Ctrl Pts',(-2.51551154229381,0.100039645074327,
95.3811501850796));
#29784=CARTESIAN_POINT('Ctrl Pts',(-2.51683050222496,0.066874204231872,
95.3832390225557));
#29785=CARTESIAN_POINT('Ctrl Pts',(-2.51749409347004,0.0336671575514469,
95.3853278600319));
#29786=CARTESIAN_POINT('Ctrl Pts',(-2.51749996074042,0.000444603168957273,
95.387416697508));
#29787=CARTESIAN_POINT('Ctrl Pts',(-2.51343655732594,0.000443885551454637,
95.387416697508));
#29788=CARTESIAN_POINT('Ctrl Pts',(-2.51289686506427,-0.441107800258806,
95.4152237280892));
#29789=CARTESIAN_POINT('Ctrl Pts',(-2.19219217530483,-1.7217534319749,95.4958203945983));
#29790=CARTESIAN_POINT('Ctrl Pts',(-0.1532262480843,-2.96902544840633,95.6292066970356));
#29791=CARTESIAN_POINT('Ctrl Pts',(2.40697591309465,-1.74517565678557,95.7875756048197));
#29792=CARTESIAN_POINT('Ctrl Pts',(2.77431937328859,1.06887020238785,95.945944512604));
#29793=CARTESIAN_POINT('Ctrl Pts',(0.613923595831106,2.90898477565689,96.1043134203881));
#29794=CARTESIAN_POINT('Ctrl Pts',(-1.59108002946992,2.25210786338312,96.232711103888));
#29795=CARTESIAN_POINT('Ctrl Pts',(-2.23357827729263,1.21153303328952,96.3083191514598));
#29796=CARTESIAN_POINT('Ctrl Pts',(-2.35791364508473,0.871329681353405,
96.3311375631035));
#29797=CARTESIAN_POINT('Origin',(0.,0.,104.));
#29798=CARTESIAN_POINT('',(-2.36143105416444,0.872610810400505,97.3312318328322));
#29799=CARTESIAN_POINT('',(-2.36143112101025,0.872610629504517,97.0562333997462));
#29800=CARTESIAN_POINT('',(-2.36143112101026,0.872610629504505,104.));
#29801=CARTESIAN_POINT('',(-2.51749996796861,0.000401594395392813,96.1125833025275));
#29802=CARTESIAN_POINT('Ctrl Pts',(-2.36143112101025,0.872610629504516,
97.0562333997462));
#29803=CARTESIAN_POINT('Ctrl Pts',(-2.33278461148586,0.950132902110356,
97.0509794704497));
#29804=CARTESIAN_POINT('Ctrl Pts',(-2.3002655010888,1.02638145292235,97.0457255411532));
#29805=CARTESIAN_POINT('Ctrl Pts',(-2.26400778685995,1.10094277373418,97.0404716118567));
#29806=CARTESIAN_POINT('Ctrl Pts',(-2.22779951602781,1.17540241783961,97.0352248471628));
#29807=CARTESIAN_POINT('Ctrl Pts',(-2.18786296857266,1.24817899050201,97.0299780824688));
#29808=CARTESIAN_POINT('Ctrl Pts',(-2.14438090452949,1.31887709294281,97.0247313177748));
#29809=CARTESIAN_POINT('Ctrl Pts',(-2.10094555076451,1.38949924848218,97.0194901893781));
#29810=CARTESIAN_POINT('Ctrl Pts',(-2.05397249102578,1.45804698034267,97.0142490609813));
#29811=CARTESIAN_POINT('Ctrl Pts',(-2.00369062619877,1.52414898368998,97.0090079325846));
#29812=CARTESIAN_POINT('Ctrl Pts',(-1.95343813060393,1.59021237738965,97.0037698654888));
#29813=CARTESIAN_POINT('Ctrl Pts',(-1.89988094561557,1.65383251233682,96.9985317983929));
#29814=CARTESIAN_POINT('Ctrl Pts',(-1.84329090933107,1.71466756940738,96.9932937312971));
#29815=CARTESIAN_POINT('Ctrl Pts',(-1.78671685664124,1.77548544389673,96.9880571436691));
#29816=CARTESIAN_POINT('Ctrl Pts',(-1.72711196820619,1.83351946532465,96.9828205560411));
#29817=CARTESIAN_POINT('Ctrl Pts',(-1.66478702169368,1.8884624492958,96.9775839684132));
#29818=CARTESIAN_POINT('Ctrl Pts',(-1.60246087887709,1.94340648787701,96.9723472802709));
#29819=CARTESIAN_POINT('Ctrl Pts',(-1.537414921354,1.99525906708839,96.9671105921285));
#29820=CARTESIAN_POINT('Ctrl Pts',(-1.46999424040511,2.04375223135678,96.9618739039862));
#29821=CARTESIAN_POINT('Ctrl Pts',(-1.40250584265483,2.09229410177774,96.9566319561556));
#29822=CARTESIAN_POINT('Ctrl Pts',(-1.33263833275752,2.13746954757229,96.9513900083249));
#29823=CARTESIAN_POINT('Ctrl Pts',(-1.26076671530658,2.17905335858833,96.9461480604942));
#29824=CARTESIAN_POINT('Ctrl Pts',(-1.18885965972192,2.22065767356277,96.9409035279875));
#29825=CARTESIAN_POINT('Ctrl Pts',(-1.11494693892174,2.25866661476735,96.9356589954808));
#29826=CARTESIAN_POINT('Ctrl Pts',(-1.03942695786404,2.29290162223884,96.9304144629741));
#29827=CARTESIAN_POINT('Ctrl Pts',(-0.963772929437472,2.32719739657774,
96.9251606214636));
#29828=CARTESIAN_POINT('Ctrl Pts',(-0.886506370644806,2.35770568296987,
96.9199067799532));
#29829=CARTESIAN_POINT('Ctrl Pts',(-0.808044271200453,2.38429668996543,
96.9146529384428));
#29830=CARTESIAN_POINT('Ctrl Pts',(-0.737225908558111,2.40829721492937,
96.9099109234319));
#29831=CARTESIAN_POINT('Ctrl Pts',(-0.665434042401576,2.42910711943873,
96.905168908421));
#29832=CARTESIAN_POINT('Ctrl Pts',(-0.592982192526457,2.44666678755946,
96.9004268934101));
#29833=CARTESIAN_POINT('Ctrl Pts',(-0.512688307529111,2.46612707704975,
96.8951716127155));
#29834=CARTESIAN_POINT('Ctrl Pts',(-0.431287177478855,2.48166652730587,
96.8899163320209));
#29835=CARTESIAN_POINT('Ctrl Pts',(-0.349196172064143,2.4931643113553,96.8846610513262));
#29836=CARTESIAN_POINT('Ctrl Pts',(-0.26722154874824,2.50464579476092,96.8794132211506));
#29837=CARTESIAN_POINT('Ctrl Pts',(-0.184559445904595,2.51209692985521,
96.874165390975));
#29838=CARTESIAN_POINT('Ctrl Pts',(-0.101639614812427,2.5154474032865,96.8689175607994));
#29839=CARTESIAN_POINT('Ctrl Pts',(-0.0181195837250174,2.51882212850546,
96.8636317451671));
#29840=CARTESIAN_POINT('Ctrl Pts',(0.0656614618329577,2.51803646644374,
96.8583459295349));
#29841=CARTESIAN_POINT('Ctrl Pts',(0.149256758489685,2.51307156086832,96.8530601139027));
#29842=CARTESIAN_POINT('Ctrl Pts',(0.232103088575756,2.50815113803837,96.8478216561885));
#29843=CARTESIAN_POINT('Ctrl Pts',(0.314766515769923,2.49912608718189,96.8425831984743));
#29844=CARTESIAN_POINT('Ctrl Pts',(0.396811685536492,2.48603031683479,96.8373447407601));
#29845=CARTESIAN_POINT('Ctrl Pts',(0.478829872982636,2.47293885331371,96.8321080058255));
#29846=CARTESIAN_POINT('Ctrl Pts',(0.560229751533338,2.45577940179306,96.8268712708909));
#29847=CARTESIAN_POINT('Ctrl Pts',(0.640582822350771,2.43463752901928,96.8216345359563));
#29848=CARTESIAN_POINT('Ctrl Pts',(0.720933704526701,2.41349623210378,96.8163979436589));
#29849=CARTESIAN_POINT('Ctrl Pts',(0.800237389695353,2.38837284801125,96.8111613513615));
#29850=CARTESIAN_POINT('Ctrl Pts',(0.878078632796223,2.359403349287,96.8059247590641));
#29851=CARTESIAN_POINT('Ctrl Pts',(0.957192885521912,2.32996008563771,96.8006025279442));
#29852=CARTESIAN_POINT('Ctrl Pts',(1.03479596623164,2.29654393433539,96.7952802968244));
#29853=CARTESIAN_POINT('Ctrl Pts',(1.11047287007365,2.25934863507835,96.7899580657046));
#29854=CARTESIAN_POINT('Ctrl Pts',(1.18503900163065,2.22269928188212,96.784713953357));
#29855=CARTESIAN_POINT('Ctrl Pts',(1.25773474598859,2.18238126500678,96.7794698410095));
#29856=CARTESIAN_POINT('Ctrl Pts',(1.32818942411985,2.13862551739574,96.774225728662));
#29857=CARTESIAN_POINT('Ctrl Pts',(1.40021839145288,2.09389206038616,96.768864438156));
#29858=CARTESIAN_POINT('Ctrl Pts',(1.4699045123945,2.04556568193834,96.76350314765));
#29859=CARTESIAN_POINT('Ctrl Pts',(1.5368860919091,1.99393765963141,96.758141857144));
#29860=CARTESIAN_POINT('Ctrl Pts',(1.60386767142369,1.94230963732448,96.752780566638));
#29861=CARTESIAN_POINT('Ctrl Pts',(1.66814436666828,1.88738035199303,96.747419276132));
#29862=CARTESIAN_POINT('Ctrl Pts',(1.7293947723073,1.82948079287982,96.7420579856259));
#29863=CARTESIAN_POINT('Ctrl Pts',(1.78943248688574,1.77272758172979,96.7368028428099));
#29864=CARTESIAN_POINT('Ctrl Pts',(1.84678445224079,1.71291103807284,96.7315476999939));
#29865=CARTESIAN_POINT('Ctrl Pts',(1.90112208808839,1.65031544141792,96.7262925571779));
#29866=CARTESIAN_POINT('Ctrl Pts',(1.95538268272115,1.58780859431448,96.7210448652305));
#29867=CARTESIAN_POINT('Ctrl Pts',(2.00663713686189,1.52253086616357,96.7157971732831));
#29868=CARTESIAN_POINT('Ctrl Pts',(2.05459249820959,1.45480442544724,96.7105494813357));
#29869=CARTESIAN_POINT('Ctrl Pts',(2.1028965633686,1.38658551699965,96.7052636311901));
#29870=CARTESIAN_POINT('Ctrl Pts',(2.14785300996875,1.3158824595113,96.6999777810446));
#29871=CARTESIAN_POINT('Ctrl Pts',(2.18920275961304,1.24305974406005,96.694691930899));
#29872=CARTESIAN_POINT('Ctrl Pts',(2.23018069123416,1.17089185235826,96.6894536112553));
#29873=CARTESIAN_POINT('Ctrl Pts',(2.26761629636635,1.09664267832251,96.6842152916115));
#29874=CARTESIAN_POINT('Ctrl Pts',(2.30130099255538,1.02069583699729,96.6789769719678));
#29875=CARTESIAN_POINT('Ctrl Pts',(2.33497461285341,0.944773967811713,96.67374037474));
#29876=CARTESIAN_POINT('Ctrl Pts',(2.36489958674497,0.86715596145425,96.6685037775122));
#29877=CARTESIAN_POINT('Ctrl Pts',(2.39091439469562,0.78824780826671,96.6632671802844));
#29878=CARTESIAN_POINT('Ctrl Pts',(2.41692849676088,0.709341796171769,96.6580307251464));
#29879=CARTESIAN_POINT('Ctrl Pts',(2.4390325003349,0.629146145411388,96.6527942700083));
#29880=CARTESIAN_POINT('Ctrl Pts',(2.45711438189941,0.548083172760395,96.6475578148703));
#29881=CARTESIAN_POINT('Ctrl Pts',(2.47549301954925,0.465689811435834,96.6422354201179));
#29882=CARTESIAN_POINT('Ctrl Pts',(2.48971620069626,0.382400879284435,96.6369130253655));
#29883=CARTESIAN_POINT('Ctrl Pts',(2.49972047828995,0.298670019281929,96.6315906306132));
#29884=CARTESIAN_POINT('Ctrl Pts',(2.50957735913563,0.216172797226468,96.6263466526851));
#29885=CARTESIAN_POINT('Ctrl Pts',(2.51533885485511,0.133247053970913,96.621102674757));
#29886=CARTESIAN_POINT('Ctrl Pts',(2.51699686113291,0.0503294252607898,
96.6158586968289));
#29887=CARTESIAN_POINT('Ctrl Pts',(2.51869205738044,-0.0344480903165743,
96.6104970936644));
#29888=CARTESIAN_POINT('Ctrl Pts',(2.51609746535214,-0.119216610928426,
96.6051354904999));
#29889=CARTESIAN_POINT('Ctrl Pts',(2.50926050336597,-0.203514068917991,
96.5997738873354));
#29890=CARTESIAN_POINT('Ctrl Pts',(2.5024235413798,-0.287811526907556,96.5944122841709));
#29891=CARTESIAN_POINT('Ctrl Pts',(2.49134434230851,-0.371637427127336,
96.5890506810063));
#29892=CARTESIAN_POINT('Ctrl Pts',(2.47612558791285,-0.45454188243027,96.5836890778418));
#29893=CARTESIAN_POINT('Ctrl Pts',(2.46120841128382,-0.535803487088283,
96.5784337212377));
#29894=CARTESIAN_POINT('Ctrl Pts',(2.44225918150389,-0.616480033833178,
96.5731783646336));
#29895=CARTESIAN_POINT('Ctrl Pts',(2.41933747240763,-0.696141109692764,
96.5679230080295));
#29896=CARTESIAN_POINT('Ctrl Pts',(2.39644826324253,-0.775689236754743,
96.5626751028212));
#29897=CARTESIAN_POINT('Ctrl Pts',(2.36959788897822,-0.85422431309093,96.5574271976129));
#29898=CARTESIAN_POINT('Ctrl Pts',(2.33889710181438,-0.931325183340554,
96.5521792924046));
#29899=CARTESIAN_POINT('Ctrl Pts',(2.30797464513566,-1.00898274656396,96.5468934956401));
#29900=CARTESIAN_POINT('Ctrl Pts',(2.27314602487704,-1.08518483970174,96.5416076988757));
#29901=CARTESIAN_POINT('Ctrl Pts',(2.23457590956298,-1.15951574133375,96.5363219021112));
#29902=CARTESIAN_POINT('Ctrl Pts',(2.19635069606593,-1.23318196092313,96.5310833720166));
#29903=CARTESIAN_POINT('Ctrl Pts',(2.15445085106199,-1.30500990341387,96.5258448419221));
#29904=CARTESIAN_POINT('Ctrl Pts',(2.10908459973996,-1.37461572853643,96.5206063118275));
#29905=CARTESIAN_POINT('Ctrl Pts',(2.06373327781223,-1.44419864736237,96.5153695056594));
#29906=CARTESIAN_POINT('Ctrl Pts',(2.01491806688972,-1.51156051491705,96.5101326994913));
#29907=CARTESIAN_POINT('Ctrl Pts',(1.96289158387131,-1.57634478461001,96.5048958933232));
#29908=CARTESIAN_POINT('Ctrl Pts',(1.91086653019555,-1.64112727446096,96.4996592310278));
#29909=CARTESIAN_POINT('Ctrl Pts',(1.85563066954816,-1.70333194814043,96.4944225687324));
#29910=CARTESIAN_POINT('Ctrl Pts',(1.79747726185939,-1.76263488649762,96.489185906437));
#29911=CARTESIAN_POINT('Ctrl Pts',(1.73837456763181,-1.82290587614074,96.4838637617387));
#29912=CARTESIAN_POINT('Ctrl Pts',(1.67625855285653,-1.88017918278022,96.4785416170404));
#29913=CARTESIAN_POINT('Ctrl Pts',(1.61147511189883,-1.93415465093427,96.4732194723421));
#29914=CARTESIAN_POINT('Ctrl Pts',(1.54764070768506,-1.98733941236153,96.4679752937228));
#29915=CARTESIAN_POINT('Ctrl Pts',(1.48121692313514,-2.03732208599083,96.4627311151035));
#29916=CARTESIAN_POINT('Ctrl Pts',(1.41256560716746,-2.08385811787838,96.4574869364842));
#29917=CARTESIAN_POINT('Ctrl Pts',(1.34238331533709,-2.13143193819811,96.4521258087464));
#29918=CARTESIAN_POINT('Ctrl Pts',(1.26987338288143,-2.17540327598279,96.4467646810087));
#29919=CARTESIAN_POINT('Ctrl Pts',(1.19544906565652,-2.2155603763881,96.4414035532709));
#29920=CARTESIAN_POINT('Ctrl Pts',(1.12102474843161,-2.2557174767934,96.4360424255331));
#29921=CARTESIAN_POINT('Ctrl Pts',(1.04468653373815,-2.29206018174533,96.4306812977953));
#29922=CARTESIAN_POINT('Ctrl Pts',(0.966867543843202,-2.32442969406747,
96.4253201700575));
#29923=CARTESIAN_POINT('Ctrl Pts',(0.890582723867995,-2.35616105454278,
96.4200647347853));
#29924=CARTESIAN_POINT('Ctrl Pts',(0.8125933817548,-2.38419164490845,96.4148092995131));
#29925=CARTESIAN_POINT('Ctrl Pts',(0.733293001241794,-2.40833710770104,
96.4095538642409));
#29926=CARTESIAN_POINT('Ctrl Pts',(0.654105018669554,-2.43244834745107,
96.4043058778624));
#29927=CARTESIAN_POINT('Ctrl Pts',(0.573610126382135,-2.45268526421946,
96.3990578914839));
#29928=CARTESIAN_POINT('Ctrl Pts',(0.492221904547019,-2.46891146999728,
96.3938099051053));
#29929=CARTESIAN_POINT('Ctrl Pts',(0.410247611457908,-2.48525451961997,
96.3885241283207));
#29930=CARTESIAN_POINT('Ctrl Pts',(0.327367506731554,-2.49752867233272,
96.383238351536));
#29931=CARTESIAN_POINT('Ctrl Pts',(0.244019939406591,-2.50564572898325,
96.3779525747513));
#29932=CARTESIAN_POINT('Ctrl Pts',(0.161416005165548,-2.51369036466143,
96.3727139580533));
#29933=CARTESIAN_POINT('Ctrl Pts',(0.0783533841716873,-2.51765174293905,
96.3674753413552));
#29934=CARTESIAN_POINT('Ctrl Pts',(-0.00473257817738232,-2.51749555167508,
96.3622367246571));
#29935=CARTESIAN_POINT('Ctrl Pts',(-0.0877912275859617,-2.51733941175603,
96.3569998300553));
#29936=CARTESIAN_POINT('Ctrl Pts',(-0.170872742092727,-2.51306839143966,
96.3517629354535));
#29937=CARTESIAN_POINT('Ctrl Pts',(-0.253540502778757,-2.50470027417468,
96.3465260408517));
#29938=CARTESIAN_POINT('Ctrl Pts',(-0.336206019147242,-2.49633238409272,
96.3412892884245));
#29939=CARTESIAN_POINT('Ctrl Pts',(-0.418457345096286,-2.48386766571071,
96.3360525359972));
#29940=CARTESIAN_POINT('Ctrl Pts',(-0.499863102816892,-2.46737575744804,
96.33081578357));
#29941=CARTESIAN_POINT('Ctrl Pts',(-0.582594716538996,-2.45061524538928,
96.3254937401286));
#29942=CARTESIAN_POINT('Ctrl Pts',(-0.664452486780437,-2.42969526837323,
96.3201716966873));
#29943=CARTESIAN_POINT('Ctrl Pts',(-0.744996360411872,-2.40474253777261,
96.3148496532459));
#29944=CARTESIAN_POINT('Ctrl Pts',(-0.82436323944698,-2.38015444358388,
96.3096053812859));
#29945=CARTESIAN_POINT('Ctrl Pts',(-0.902453950006558,-2.35165089785812,
96.304361109326));
#29946=CARTESIAN_POINT('Ctrl Pts',(-0.978866343377746,-2.31940227899394,
96.299116837366));
#29947=CARTESIAN_POINT('Ctrl Pts',(-1.05697850701551,-2.28643629948883,
96.2937559081839));
#29948=CARTESIAN_POINT('Ctrl Pts',(-1.1333363289692,-2.24955685305805,96.2883949790018));
#29949=CARTESIAN_POINT('Ctrl Pts',(-1.20753724918357,-2.20899525618191,
96.2830340498197));
#29950=CARTESIAN_POINT('Ctrl Pts',(-1.28173816939795,-2.16843365930577,
96.2776731206376));
#29951=CARTESIAN_POINT('Ctrl Pts',(-1.35378179009948,-2.1241902345683,96.2723121914555));
#29952=CARTESIAN_POINT('Ctrl Pts',(-1.42329914826855,-2.07654178492464,
96.2669512622735));
#29953=CARTESIAN_POINT('Ctrl Pts',(-1.49115044797179,-2.0300352817675,96.2617188135412));
#29954=CARTESIAN_POINT('Ctrl Pts',(-1.55685069166608,-1.98011000497322,
96.2564863648089));
#29955=CARTESIAN_POINT('Ctrl Pts',(-1.62003283028502,-1.92699244388729,
96.2512539160767));
#29956=CARTESIAN_POINT('Ctrl Pts',(-1.68312519141424,-1.87395035921604,
96.2460289022955));
#29957=CARTESIAN_POINT('Ctrl Pts',(-1.74370619932942,-1.81772529526381,
96.2408038885144));
#29958=CARTESIAN_POINT('Ctrl Pts',(-1.80143792018448,-1.75858683883436,
96.2355788747332));
#29959=CARTESIAN_POINT('Ctrl Pts',(-1.85910373811189,-1.69951589117404,
96.2303598255016));
#29960=CARTESIAN_POINT('Ctrl Pts',(-1.91392640870733,-1.63753849161027,
96.2251407762699));
#29961=CARTESIAN_POINT('Ctrl Pts',(-1.96560237125858,-1.57296330793272,
96.2199217270382));
#29962=CARTESIAN_POINT('Ctrl Pts',(-2.01724621436462,-1.50842826127385,
96.2147059217319));
#29963=CARTESIAN_POINT('Ctrl Pts',(-2.06574694108255,-1.4412989981258,96.2094901164256));
#29964=CARTESIAN_POINT('Ctrl Pts',(-2.11083986172856,-1.3719188489622,96.2042743111193));
#29965=CARTESIAN_POINT('Ctrl Pts',(-2.15591867107367,-1.30256041150293,
96.1990601380381));
#29966=CARTESIAN_POINT('Ctrl Pts',(-2.19759153829349,-1.230952877166,96.1938459649569));
#29967=CARTESIAN_POINT('Ctrl Pts',(-2.23563672808269,-1.15746907952124,
96.1886317918757));
#29968=CARTESIAN_POINT('Ctrl Pts',(-2.27368175334582,-1.08398559965646,
96.1834176413432));
#29969=CARTESIAN_POINT('Ctrl Pts',(-2.308098919539,-1.00862628711035,96.1782034908107));
#29970=CARTESIAN_POINT('Ctrl Pts',(-2.33871282661468,-0.931787832410345,
96.1729893402781));
#29971=CARTESIAN_POINT('Ctrl Pts',(-2.36935658379212,-0.85487445634579,
96.1677701056861));
#29972=CARTESIAN_POINT('Ctrl Pts',(-2.39618950242494,-0.776479491398637,
96.1625508710941));
#29973=CARTESIAN_POINT('Ctrl Pts',(-2.41908490056256,-0.697018288045754,
96.1573316365021));
#29974=CARTESIAN_POINT('Ctrl Pts',(-2.44199140476928,-0.61751853975865,
96.1521098701708));
#29975=CARTESIAN_POINT('Ctrl Pts',(-2.4609564779823,-0.536951977037695,
96.1468881038394));
#29976=CARTESIAN_POINT('Ctrl Pts',(-2.47590437245768,-0.455745310941257,
96.1416663375081));
#29977=CARTESIAN_POINT('Ctrl Pts',(-2.49087835027489,-0.374396943200185,
96.136435459451));
#29978=CARTESIAN_POINT('Ctrl Pts',(-2.50182108451074,-0.292406703397515,
96.1312045813938));
#29979=CARTESIAN_POINT('Ctrl Pts',(-2.508708654222,-0.21020736959398,96.1259737033366));
#29980=CARTESIAN_POINT('Ctrl Pts',(-2.51458576306344,-0.140067327212032,
96.1215102364002));
#29981=CARTESIAN_POINT('Ctrl Pts',(-2.51751116265911,-0.0697752639189464,
96.1170467694638));
#29982=CARTESIAN_POINT('Ctrl Pts',(-2.51749996796861,0.000401594395409275,
96.1125833025275));
#29983=CARTESIAN_POINT('Ctrl Pts',(-2.51749996796852,0.000401594953133782,
96.112583302492));
#29984=CARTESIAN_POINT('Ctrl Pts',(-2.5174966230771,0.0213698964335877,
96.1112496531577));
#29985=CARTESIAN_POINT('Ctrl Pts',(-2.51723131533456,0.0423358846343242,
96.1099160038235));
#29986=CARTESIAN_POINT('Ctrl Pts',(-2.51670418679687,0.0632952301448918,
96.1085823544893));
#29987=CARTESIAN_POINT('Ctrl Pts',(-2.51462701145563,0.145886538621763,
96.1033270451808));
#29988=CARTESIAN_POINT('Ctrl Pts',(-2.50847607316376,0.228527745844191,
96.0980717358723));
#29989=CARTESIAN_POINT('Ctrl Pts',(-2.49824322749019,0.310784533558853,
96.0928164265637));
#29990=CARTESIAN_POINT('Ctrl Pts',(-2.48802311238251,0.392938986547741,
96.0875676553252));
#29991=CARTESIAN_POINT('Ctrl Pts',(-2.47373122398474,0.474709515524631,
96.0823188840867));
#29992=CARTESIAN_POINT('Ctrl Pts',(-2.45541140221161,0.555662753735768,
96.0770701128482));
#29993=CARTESIAN_POINT('Ctrl Pts',(-2.43711230709236,0.636524403187498,
96.071827279957));
#29994=CARTESIAN_POINT('Ctrl Pts',(-2.41479443687441,0.716570152071475,
96.0665844470658));
#29995=CARTESIAN_POINT('Ctrl Pts',(-2.38855310451469,0.79537432502768,96.0613416141747));
#29996=CARTESIAN_POINT('Ctrl Pts',(-2.3799338018142,0.821258567925877,96.059619538364));
#29997=CARTESIAN_POINT('Ctrl Pts',(-2.37089161588231,0.847008939293941,
96.0578974625533));
#29998=CARTESIAN_POINT('Ctrl Pts',(-2.36143112101026,0.872610629504502,
96.0561753867426));
#29999=CARTESIAN_POINT('',(-2.51804717241927,-0.00223002504931176,96.387416372278));
#30000=CARTESIAN_POINT('Ctrl Pts',(-2.35791364508473,0.871329681353405,
96.3311375631035));
#30001=CARTESIAN_POINT('Ctrl Pts',(-2.46013294861404,0.591639756348386,
96.3498971661617));
#30002=CARTESIAN_POINT('Ctrl Pts',(-2.51533068634196,0.294269068221567,
96.3686567692199));
#30003=CARTESIAN_POINT('Ctrl Pts',(-2.51804717241927,-0.00223002504931176,
96.387416372278));
#30004=CARTESIAN_POINT('Ctrl Pts',(-2.51749899202554,-0.00225280944616036,
96.3871012985794));
#30005=CARTESIAN_POINT('Ctrl Pts',(-2.51736869845421,-0.147854975242588,
96.3954712422479));
#30006=CARTESIAN_POINT('Ctrl Pts',(-2.50460703660455,-0.293157170744765,
96.4038561557088));
#30007=CARTESIAN_POINT('Ctrl Pts',(-2.47713855551654,-0.449172301708327,
96.4136292598055));
#30008=CARTESIAN_POINT('Ctrl Pts',(-2.47481501998665,-0.461802751706162,
96.4144261123344));
#30009=CARTESIAN_POINT('Ctrl Pts',(-2.47085734709265,-0.482428025777387,
96.4157374330634));
#30010=CARTESIAN_POINT('Ctrl Pts',(-2.46928076369863,-0.490433823824153,
96.416248919652));
#30011=CARTESIAN_POINT('Ctrl Pts',(-2.46615177369721,-0.505925014025159,
96.4172437220335));
#30012=CARTESIAN_POINT('Ctrl Pts',(-2.46460413363991,-0.513411288839801,
96.4177267738757));
#30013=CARTESIAN_POINT('Ctrl Pts',(-2.46167272031015,-0.527272435975308,
96.4186256324734));
#30014=CARTESIAN_POINT('Ctrl Pts',(-2.46029824341979,-0.533649092358558,
96.419040915781));
#30015=CARTESIAN_POINT('Ctrl Pts',(-2.45709173712559,-0.54824942296337,
96.4199958092197));
#30016=CARTESIAN_POINT('Ctrl Pts',(-2.45524320293902,-0.556469265974654,
96.4205363306388));
#30017=CARTESIAN_POINT('Ctrl Pts',(-2.45026371327949,-0.578103569240206,
96.421966400759));
#30018=CARTESIAN_POINT('Ctrl Pts',(-2.44706390474626,-0.591501671672988,
96.4228595971909));
#30019=CARTESIAN_POINT('Ctrl Pts',(-2.41553413935428,-0.718885549531426,
96.4314195309139));
#30020=CARTESIAN_POINT('Ctrl Pts',(-2.37937258034627,-0.830771642697027,
96.4394499975993));
#30021=CARTESIAN_POINT('Ctrl Pts',(-2.29695512651911,-1.03561035858076,
96.4546748422432));
#30022=CARTESIAN_POINT('Ctrl Pts',(-2.25249859383891,-1.1290451952626,96.4618406556468));
#30023=CARTESIAN_POINT('Ctrl Pts',(-2.14168670374415,-1.32917466175404,
96.4774656388834));
#30024=CARTESIAN_POINT('Ctrl Pts',(-2.07283412553353,-1.43418762657598,
96.4858491771246));
#30025=CARTESIAN_POINT('Ctrl Pts',(-1.9813782849684,-1.55324077978427,96.4955397713327));
#30026=CARTESIAN_POINT('Ctrl Pts',(-1.96603707706141,-1.57261410104507,
96.4971235943012));
#30027=CARTESIAN_POINT('Ctrl Pts',(-1.94151940078541,-1.60265607756257,
96.499591283578));
#30028=CARTESIAN_POINT('Ctrl Pts',(-1.93253482708415,-1.61347861521284,
96.5004827052764));
#30029=CARTESIAN_POINT('Ctrl Pts',(-1.91670809061988,-1.63222114394683,
96.502030979773));
#30030=CARTESIAN_POINT('Ctrl Pts',(-1.90990643789813,-1.64017473800895,
96.5026894474174));
#30031=CARTESIAN_POINT('Ctrl Pts',(-1.89445073822101,-1.65802153426466,
96.5041703630596));
#30032=CARTESIAN_POINT('Ctrl Pts',(-1.88576836702892,-1.667889889638,96.5049916242427));
#30033=CARTESIAN_POINT('Ctrl Pts',(-1.86207567245965,-1.69439740997439,
96.5072045071578));
#30034=CARTESIAN_POINT('Ctrl Pts',(-1.84691960726537,-1.71090514263882,
96.508590032471));
#30035=CARTESIAN_POINT('Ctrl Pts',(-1.77181792987299,-1.79054351030284,
96.5153149543631));
#30036=CARTESIAN_POINT('Ctrl Pts',(-1.70884243550823,-1.8507416645472,96.5205228595494));
#30037=CARTESIAN_POINT('Ctrl Pts',(-1.49171958293045,-2.03773668503772,
96.5373633179015));
#30038=CARTESIAN_POINT('Ctrl Pts',(-1.32564751779107,-2.14947629899044,
96.5484980300191));
#30039=CARTESIAN_POINT('Ctrl Pts',(-1.08760705431638,-2.27146291121257,
96.5642849552167));
#30040=CARTESIAN_POINT('Ctrl Pts',(-1.02584674250349,-2.3000151272654,96.5683732811711));
#30041=CARTESIAN_POINT('Ctrl Pts',(-0.950853998876421,-2.33106329685779,
96.5734154553201));
#30042=CARTESIAN_POINT('Ctrl Pts',(-0.938656422552669,-2.3360016104919,
96.5742379770537));
#30043=CARTESIAN_POINT('Ctrl Pts',(-0.919218732074385,-2.3436943422727,
96.5755533950753));
#30044=CARTESIAN_POINT('Ctrl Pts',(-0.912003462970394,-2.34651143767192,
96.5760426940437));
#30045=CARTESIAN_POINT('Ctrl Pts',(-0.898696808362354,-2.35163618075541,
96.5769471450763));
#30046=CARTESIAN_POINT('Ctrl Pts',(-0.892609352845022,-2.35395352974292,
96.5773617178837));
#30047=CARTESIAN_POINT('Ctrl Pts',(-0.878752856314007,-2.35916688923337,
96.578307206302));
#30048=CARTESIAN_POINT('Ctrl Pts',(-0.870978499856468,-2.36204814554349,
96.5788389624841));
#30049=CARTESIAN_POINT('Ctrl Pts',(-0.850673276283677,-2.36945959514692,
96.5802308780278));
#30050=CARTESIAN_POINT('Ctrl Pts',(-0.83812060822937,-2.37392873187347,
96.5810943882574));
#30051=CARTESIAN_POINT('Ctrl Pts',(-0.746297215186853,-2.40580164232354,
96.587430035659));
#30052=CARTESIAN_POINT('Ctrl Pts',(-0.665743868903635,-2.42932567990088,
96.5930896452486));
#30053=CARTESIAN_POINT('Ctrl Pts',(-0.43442119867569,-2.48450947825652,
96.6093611230807));
#30054=CARTESIAN_POINT('Ctrl Pts',(-0.281693688112623,-2.50642412335036,
96.6201050150125));
#30055=CARTESIAN_POINT('Ctrl Pts',(-0.01462777033248,-2.52001211653579,
96.6382770469461));
#30056=CARTESIAN_POINT('Ctrl Pts',(0.0989383796333694,-2.51811288601598,
96.6458196306118));
#30057=CARTESIAN_POINT('Ctrl Pts',(0.235061587411381,-2.50660881794183,
96.6546166001066));
#30058=CARTESIAN_POINT('Ctrl Pts',(0.258092168782863,-2.50434227031001,
96.6560968632599));
#30059=CARTESIAN_POINT('Ctrl Pts',(0.294307558461799,-2.50027323518626,
96.6584124611988));
#30060=CARTESIAN_POINT('Ctrl Pts',(0.307514469074636,-2.49868326362219,
96.6592543664414));
#30061=CARTESIAN_POINT('Ctrl Pts',(0.332221808824444,-2.49550990096949,
96.6608248342909));
#30062=CARTESIAN_POINT('Ctrl Pts',(0.343725037358974,-2.4939515035475,96.6615541563901));
#30063=CARTESIAN_POINT('Ctrl Pts',(0.369460172429428,-2.49028360094326,
96.6631818328872));
#30064=CARTESIAN_POINT('Ctrl Pts',(0.383685676705576,-2.48813153736058,
96.6640788303803));
#30065=CARTESIAN_POINT('Ctrl Pts',(0.419846857765702,-2.48234349406893,
96.6663525193734));
#30066=CARTESIAN_POINT('Ctrl Pts',(0.441754523847646,-2.47853860077018,
96.6677239055907));
#30067=CARTESIAN_POINT('Ctrl Pts',(0.617903764149041,-2.44553544627036,
96.6787079687245));
#30068=CARTESIAN_POINT('Ctrl Pts',(0.769163806993482,-2.40225825460969,
96.6878460610998));
#30069=CARTESIAN_POINT('Ctrl Pts',(1.02082027151597,-2.30402544269776,96.70339569076));
#30070=CARTESIAN_POINT('Ctrl Pts',(1.1233190824176,-2.25582789362918,96.7098465679069));
#30071=CARTESIAN_POINT('Ctrl Pts',(1.29194759528697,-2.16218365981552,96.7211585768009));
#30072=CARTESIAN_POINT('Ctrl Pts',(1.35978451204018,-2.12017692513694,96.7259224771952));
#30073=CARTESIAN_POINT('Ctrl Pts',(1.4370440739107,-2.067100994749,96.7317426504604));
#30074=CARTESIAN_POINT('Ctrl Pts',(1.44851515365224,-2.05907892555464,96.7326174912785));
#30075=CARTESIAN_POINT('Ctrl Pts',(1.46614712528584,-2.04652811157846,96.733979819267));
#30076=CARTESIAN_POINT('Ctrl Pts',(1.47235549102788,-2.04206611274972,96.7344629280109));
#30077=CARTESIAN_POINT('Ctrl Pts',(1.48382314310826,-2.03374474421842,96.7353618487868));
#30078=CARTESIAN_POINT('Ctrl Pts',(1.48908784809098,-2.02989314547075,96.7357771369691));
#30079=CARTESIAN_POINT('Ctrl Pts',(1.50111750270568,-2.02102040285675,96.7367320025181));
#30080=CARTESIAN_POINT('Ctrl Pts',(1.50787223600282,-2.015985749133,96.7372724907548));
#30081=CARTESIAN_POINT('Ctrl Pts',(1.52560355928216,-2.00263070611328,96.7387024428408));
#30082=CARTESIAN_POINT('Ctrl Pts',(1.53653718614361,-1.99425410138389,96.7395955537004));
#30083=CARTESIAN_POINT('Ctrl Pts',(1.63758129532717,-1.91551672049043,96.7479514150837));
#30084=CARTESIAN_POINT('Ctrl Pts',(1.72286006376316,-1.83919116019482,96.7557591018763));
#30085=CARTESIAN_POINT('Ctrl Pts',(1.95750172031732,-1.59850081971393,96.778926717251));
#30086=CARTESIAN_POINT('Ctrl Pts',(2.09071643795581,-1.41984541168163,96.7942838728304));
#30087=CARTESIAN_POINT('Ctrl Pts',(2.21433353769386,-1.19814506270149,96.8107629793089));
#30088=CARTESIAN_POINT('Ctrl Pts',(2.22934366403865,-1.16997931080664,96.81281624481));
#30089=CARTESIAN_POINT('Ctrl Pts',(2.25065184014371,-1.1280956946248,96.8158120644517));
#30090=CARTESIAN_POINT('Ctrl Pts',(2.25736813462483,-1.1145953178947,96.8167690924862));
#30091=CARTESIAN_POINT('Ctrl Pts',(2.2690701561936,-1.09053346879776,96.8184598488054));
#30092=CARTESIAN_POINT('Ctrl Pts',(2.27410439477052,-1.07999621730903,96.8191952360079));
#30093=CARTESIAN_POINT('Ctrl Pts',(2.28453611738341,-1.05776502355943,96.8207363543664));
#30094=CARTESIAN_POINT('Ctrl Pts',(2.28991756455601,-1.0460638957742,96.8215415194635));
#30095=CARTESIAN_POINT('Ctrl Pts',(2.30391723192259,-1.01499797115693,96.8236637521622));
#30096=CARTESIAN_POINT('Ctrl Pts',(2.31238121449784,-0.995564490250916,
96.8249755693114));
#30097=CARTESIAN_POINT('Ctrl Pts',(2.3487777427595,-0.909028118383248,96.8307505985041));
#30098=CARTESIAN_POINT('Ctrl Pts',(2.37404354144121,-0.840837505874827,
96.835124562483));
#30099=CARTESIAN_POINT('Ctrl Pts',(2.45519220682739,-0.588831965276025,
96.8507971199932));
#30100=CARTESIAN_POINT('Ctrl Pts',(2.49294487011241,-0.399894162543879,
96.8615700915236));
#30101=CARTESIAN_POINT('Ctrl Pts',(2.51396283906021,-0.146992712775582,
96.876373814445));
#30102=CARTESIAN_POINT('Ctrl Pts',(2.51681064548625,-0.0853181810766132,
96.8800188223732));
#30103=CARTESIAN_POINT('Ctrl Pts',(2.51772190102843,0.0118611696635401,
96.8859005307417));
#30104=CARTESIAN_POINT('Ctrl Pts',(2.51730489349256,0.0473290425222484,
96.8880762732822));
#30105=CARTESIAN_POINT('Ctrl Pts',(2.51577740093312,0.0937612139800365,
96.8909763876195));
#30106=CARTESIAN_POINT('Ctrl Pts',(2.51534400302675,0.104745559996041,96.8916662618259));
#30107=CARTESIAN_POINT('Ctrl Pts',(2.51451751233488,0.122705933496783,96.8928009975015));
#30108=CARTESIAN_POINT('Ctrl Pts',(2.51416728639153,0.129683920177109,96.8932435293651));
#30109=CARTESIAN_POINT('Ctrl Pts',(2.51342584239047,0.143322362638641,96.8941118645075));
#30110=CARTESIAN_POINT('Ctrl Pts',(2.51303718676604,0.149982863058114,96.8945375250866));
#30111=CARTESIAN_POINT('Ctrl Pts',(2.51210863132155,0.164877429387833,96.8954928725087));
#30112=CARTESIAN_POINT('Ctrl Pts',(2.51155471380607,0.173110534955513,96.8960233169788));
#30113=CARTESIAN_POINT('Ctrl Pts',(2.50949076308395,0.201689339334537,96.8978724783795));
#30114=CARTESIAN_POINT('Ctrl Pts',(2.50777393767597,0.222018681227759,96.8992017402161));
#30115=CARTESIAN_POINT('Ctrl Pts',(2.49020576267543,0.403686569900397,96.9111914343765));
#30116=CARTESIAN_POINT('Ctrl Pts',(2.45905275197633,0.563150936138783,96.9224745232812));
#30117=CARTESIAN_POINT('Ctrl Pts',(2.38459567424872,0.81318520545695,96.9404746501786));
#30118=CARTESIAN_POINT('Ctrl Pts',(2.35084830705162,0.906135567231456,96.947245222874));
#30119=CARTESIAN_POINT('Ctrl Pts',(2.27835607887696,1.0742440202384,96.9595309643992));
#30120=CARTESIAN_POINT('Ctrl Pts',(2.24112323784498,1.14990257913459,96.965077506078));
#30121=CARTESIAN_POINT('Ctrl Pts',(2.18976502278141,1.24225318390907,96.9718695864845));
#30122=CARTESIAN_POINT('Ctrl Pts',(2.17913040673448,1.26081503183629,96.9732360717253));
#30123=CARTESIAN_POINT('Ctrl Pts',(2.16169416597186,1.2903687671375,96.9754144456115));
#30124=CARTESIAN_POINT('Ctrl Pts',(2.15504242208814,1.30144742172417,96.9762316600626));
#30125=CARTESIAN_POINT('Ctrl Pts',(2.1422225507075,1.32243144865635,96.9777809161396));
#30126=CARTESIAN_POINT('Ctrl Pts',(2.13607030080289,1.3323460776185,96.9785135074402));
#30127=CARTESIAN_POINT('Ctrl Pts',(2.12185325763241,1.35490587443932,96.9801820060662));
#30128=CARTESIAN_POINT('Ctrl Pts',(2.11374390273684,1.36752254259395,96.9811162505746));
#30129=CARTESIAN_POINT('Ctrl Pts',(2.08826416861913,1.40639614452347,96.9839989631298));
#30130=CARTESIAN_POINT('Ctrl Pts',(2.07051326833901,1.43240088442351,96.9859333128201));
#30131=CARTESIAN_POINT('Ctrl Pts',(1.93668811609335,1.62076434748675,97.0000068083844));
#30132=CARTESIAN_POINT('Ctrl Pts',(1.80216266846783,1.76914002491917,97.0113636465397));
#30133=CARTESIAN_POINT('Ctrl Pts',(1.55142643676616,1.98707519675985,97.0304880479226));
#30134=CARTESIAN_POINT('Ctrl Pts',(1.44463392168879,2.06601439443902,97.0381736802327));
#30135=CARTESIAN_POINT('Ctrl Pts',(1.3166970266823,2.14579738148926,97.0474774836565));
#30136=CARTESIAN_POINT('Ctrl Pts',(1.30115101569777,2.15525948613846,97.0486096512545));
#30137=CARTESIAN_POINT('Ctrl Pts',(1.2782032725643,2.16888790631447,97.0502853260724));
#30138=CARTESIAN_POINT('Ctrl Pts',(1.27088046722993,2.17318687397538,97.0508207053334));
#30139=CARTESIAN_POINT('Ctrl Pts',(1.25793946092228,2.18069631845741,97.0517682489921));
#30140=CARTESIAN_POINT('Ctrl Pts',(1.25233043839155,2.1839222954403,97.0521794156654));
#30141=CARTESIAN_POINT('Ctrl Pts',(1.24012711544488,2.1908784502098,97.0530750669781));
#30142=CARTESIAN_POINT('Ctrl Pts',(1.23352850387399,2.19460043574964,97.0535600315285));
#30143=CARTESIAN_POINT('Ctrl Pts',(1.21529119896742,2.20477905923512,97.0549019992571));
#30144=CARTESIAN_POINT('Ctrl Pts',(1.20361814052377,2.21117316189203,97.0557627523496));
#30145=CARTESIAN_POINT('Ctrl Pts',(1.14072903020723,2.24497613901738,97.0604075348055));
#30146=CARTESIAN_POINT('Ctrl Pts',(1.08863044425069,2.27069663241653,97.0642813579726));
#30147=CARTESIAN_POINT('Ctrl Pts',(0.825971085596482,2.38925142704281,97.0837788145354));
#30148=CARTESIAN_POINT('Ctrl Pts',(0.604250468243455,2.45472146883869,97.1000067331764));
#30149=CARTESIAN_POINT('Ctrl Pts',(0.330128578060306,2.49620490956519,97.1184837667602));
#30150=CARTESIAN_POINT('Ctrl Pts',(0.28337676540084,2.50194362445227,97.1215870442982));
#30151=CARTESIAN_POINT('Ctrl Pts',(0.202070612964586,2.50961528626762,97.1269005838679));
#30152=CARTESIAN_POINT('Ctrl Pts',(0.167587734951365,2.51215365027907,97.1291283529388));
#30153=CARTESIAN_POINT('Ctrl Pts',(0.117520123271069,2.51480367010516,97.1323271682915));
#30154=CARTESIAN_POINT('Ctrl Pts',(0.101970614308654,2.51548215857317,97.1333156406632));
#30155=CARTESIAN_POINT('Ctrl Pts',(0.0746774914852433,2.51641957276513,
97.1350421807336));
#30156=CARTESIAN_POINT('Ctrl Pts',(0.0629366247317871,2.51674058709904,
97.135782152265));
#30157=CARTESIAN_POINT('Ctrl Pts',(0.0385431276468122,2.51723673548667,
97.137314027442));
#30158=CARTESIAN_POINT('Ctrl Pts',(0.0258905370800573,2.51739866619819,
97.1381055008062));
#30159=CARTESIAN_POINT('Ctrl Pts',(-0.00692212389810397,2.51757119835855,
97.1401503682554));
#30160=CARTESIAN_POINT('Ctrl Pts',(-0.0270823072891021,2.51743505176332,
97.1413991943718));
#30161=CARTESIAN_POINT('Ctrl Pts',(-0.110287950182441,2.51587348052676,
97.1465245885052));
#30162=CARTESIAN_POINT('Ctrl Pts',(-0.173273414679198,2.51232165581684,
97.1503354272722));
#30163=CARTESIAN_POINT('Ctrl Pts',(-0.273033299736258,2.50292588396244,
97.1562998760702));
#30164=CARTESIAN_POINT('Ctrl Pts',(-0.309922823053082,2.49862625490241,
97.1584900008439));
#30165=CARTESIAN_POINT('Ctrl Pts',(-0.516659148436956,2.46988106653034,
97.1707136866586));
#30166=CARTESIAN_POINT('Ctrl Pts',(-0.683743833263817,2.42893812048489,
97.180367943746));
#30167=CARTESIAN_POINT('Ctrl Pts',(-0.900286280017697,2.35174212152534,
97.1938078005655));
#30168=CARTESIAN_POINT('Ctrl Pts',(-0.954510960348861,2.33026057545199,
97.1972595329997));
#30169=CARTESIAN_POINT('Ctrl Pts',(-1.02899490947952,2.29771708372573,97.2021852815925));
#30170=CARTESIAN_POINT('Ctrl Pts',(-1.04992477460914,2.2882290557155,97.2035902919113));
#30171=CARTESIAN_POINT('Ctrl Pts',(-1.08628043958002,2.27114434030453,97.2060725163512));
#30172=CARTESIAN_POINT('Ctrl Pts',(-1.10176402719163,2.26367351857929,97.2071431115649));
#30173=CARTESIAN_POINT('Ctrl Pts',(-1.12460623442567,2.25236230123277,97.2087443010268));
#30174=CARTESIAN_POINT('Ctrl Pts',(-1.13202469839731,2.24864296768326,97.2092677616357));
#30175=CARTESIAN_POINT('Ctrl Pts',(-1.14467824957472,2.242220477007,97.2101667505426));
#30176=CARTESIAN_POINT('Ctrl Pts',(-1.14992244278479,2.23953551818768,97.2105411499245));
#30177=CARTESIAN_POINT('Ctrl Pts',(-1.16180804725903,2.23339748836304,97.2113938921814));
#30178=CARTESIAN_POINT('Ctrl Pts',(-1.16844338071537,2.22993325960517,97.211872914691));
#30179=CARTESIAN_POINT('Ctrl Pts',(-1.18648273432046,2.22041250789946,97.2131831199835));
#30180=CARTESIAN_POINT('Ctrl Pts',(-1.19785558250237,2.21429785051938,97.2140177773428));
#30181=CARTESIAN_POINT('Ctrl Pts',(-1.25515630304325,2.18291927117981,97.2182650961704));
#30182=CARTESIAN_POINT('Ctrl Pts',(-1.30033095319087,2.15631454840361,97.2217507745425));
#30183=CARTESIAN_POINT('Ctrl Pts',(-1.5439540730968,2.00239747028653,97.2411852899693));
#30184=CARTESIAN_POINT('Ctrl Pts',(-1.72460488253679,1.84909555864324,97.2578426910313));
#30185=CARTESIAN_POINT('Ctrl Pts',(-1.92889053692023,1.61935656662453,97.2783386397707));
#30186=CARTESIAN_POINT('Ctrl Pts',(-1.97417430087555,1.56383243602918,97.2830302668108));
#30187=CARTESIAN_POINT('Ctrl Pts',(-2.02920284415557,1.49015291552007,97.2889341807666));
#30188=CARTESIAN_POINT('Ctrl Pts',(-2.04117542662496,1.47371055901491,97.2902322560841));
#30189=CARTESIAN_POINT('Ctrl Pts',(-2.06029392013924,1.44677444787349,97.2923279748971));
#30190=CARTESIAN_POINT('Ctrl Pts',(-2.06756183816379,1.43636882287495,97.293130246396));
#30191=CARTESIAN_POINT('Ctrl Pts',(-2.08139554654044,1.41624025365992,97.2946683272234));
#30192=CARTESIAN_POINT('Ctrl Pts',(-2.0879726579124,1.40652552928541,97.2954045501611));
#30193=CARTESIAN_POINT('Ctrl Pts',(-2.1029205020329,1.38411088902672,97.2970894735906));
#30194=CARTESIAN_POINT('Ctrl Pts',(-2.11124458202282,1.37138029803988,97.2980364205715));
#30195=CARTESIAN_POINT('Ctrl Pts',(-2.13687201109165,1.33140007140476,97.3009798983876));
#30196=CARTESIAN_POINT('Ctrl Pts',(-2.15376742209557,1.30389193499914,97.3029615083089));
#30197=CARTESIAN_POINT('Ctrl Pts',(-2.24575106326858,1.14746075079896,97.3140030727608));
#30198=CARTESIAN_POINT('Ctrl Pts',(-2.30975897673764,1.01244410929445,97.3226562753726));
#30199=CARTESIAN_POINT('Ctrl Pts',(-2.36143105416443,0.872610810400539,
97.3312318328322));
#30200=CARTESIAN_POINT('Origin',(0.,0.,104.));
#30201=CARTESIAN_POINT('',(-2.36143112099219,0.872610629553384,98.3289997116198));
#30202=CARTESIAN_POINT('',(-2.36143112101026,0.872610629504505,98.0563225720173));
#30203=CARTESIAN_POINT('',(-2.36143112101026,0.872610629504505,104.));
#30204=CARTESIAN_POINT('',(-2.51749930506837,0.00187055614564606,97.1125833024347));
#30205=CARTESIAN_POINT('Ctrl Pts',(-2.36143112101026,0.872610629504505,
98.0563225720173));
#30206=CARTESIAN_POINT('Ctrl Pts',(-2.33256999240762,0.950713697431207,
98.0510687730156));
#30207=CARTESIAN_POINT('Ctrl Pts',(-2.29985371519826,1.02731921157481,98.0458149740139));
#30208=CARTESIAN_POINT('Ctrl Pts',(-2.2634766993883,1.10203424689356,98.0405611750122));
#30209=CARTESIAN_POINT('Ctrl Pts',(-2.22702982976517,1.17689275550175,98.0352972872804));
#30210=CARTESIAN_POINT('Ctrl Pts',(-2.18690839552841,1.24985312765648,98.0300333995486));
#30211=CARTESIAN_POINT('Ctrl Pts',(-2.14335225325123,1.3205481318312,98.0247695118168));
#30212=CARTESIAN_POINT('Ctrl Pts',(-2.09988271562105,1.39110256993278,98.019516090511));
#30213=CARTESIAN_POINT('Ctrl Pts',(-2.05299243786544,1.45940031406957,98.0142626692052));
#30214=CARTESIAN_POINT('Ctrl Pts',(-2.0029596359888,1.52510948675812,98.0090092478994));
#30215=CARTESIAN_POINT('Ctrl Pts',(-1.95290942326789,1.59084152548915,98.0037539984629));
#30216=CARTESIAN_POINT('Ctrl Pts',(-1.89952761528302,1.65422856294524,97.9984987490264));
#30217=CARTESIAN_POINT('Ctrl Pts',(-1.84306196639629,1.71491365322673,97.9932434995899));
#30218=CARTESIAN_POINT('Ctrl Pts',(-1.78667637299258,1.77551270581432,97.9879957009051));
#30219=CARTESIAN_POINT('Ctrl Pts',(-1.72721593482255,1.83341708522346,97.9827479022204));
#30220=CARTESIAN_POINT('Ctrl Pts',(-1.66496986728393,1.88830124477969,97.9775001035356));
#30221=CARTESIAN_POINT('Ctrl Pts',(-1.60227277373286,1.94358308702674,97.9722142800598));
#30222=CARTESIAN_POINT('Ctrl Pts',(-1.53674979902648,1.99580037955735,97.9669284565839));
#30223=CARTESIAN_POINT('Ctrl Pts',(-1.46873581608155,2.04465678111493,97.9616426331081));
#30224=CARTESIAN_POINT('Ctrl Pts',(-1.4013317094487,2.09307509096382,97.9564042072171));
#30225=CARTESIAN_POINT('Ctrl Pts',(-1.33148147068404,2.13819226799277,97.9511657813261));
#30226=CARTESIAN_POINT('Ctrl Pts',(-1.25954438060733,2.17976012516986,97.9459273554351));
#30227=CARTESIAN_POINT('Ctrl Pts',(-1.18763094946768,2.22131431135586,97.940690652377));
#30228=CARTESIAN_POINT('Ctrl Pts',(-1.11363242931061,2.25932126536479,97.935453949319));
#30229=CARTESIAN_POINT('Ctrl Pts',(-1.03793535235416,2.29357721787025,97.9302172462609));
#30230=CARTESIAN_POINT('Ctrl Pts',(-0.962240337375317,2.32783223724844,
97.9249806858499));
#30231=CARTESIAN_POINT('Ctrl Pts',(-0.884847278394691,2.3583362689779,97.9197441254389));
#30232=CARTESIAN_POINT('Ctrl Pts',(-0.806164203337558,2.38493302364178,
97.9145075650279));
#30233=CARTESIAN_POINT('Ctrl Pts',(-0.726193299139214,2.41196509524889,
97.9091852962852));
#30234=CARTESIAN_POINT('Ctrl Pts',(-0.644890231355187,2.43496066281516,
97.9038630275425));
#30235=CARTESIAN_POINT('Ctrl Pts',(-0.562699283145033,2.45380842095467,
97.8985407587997));
#30236=CARTESIAN_POINT('Ctrl Pts',(-0.481715779428683,2.47237929189089,
97.8932966780355));
#30237=CARTESIAN_POINT('Ctrl Pts',(-0.399870780873901,2.486923391632,97.8880525972712));
#30238=CARTESIAN_POINT('Ctrl Pts',(-0.317597601026388,2.49738623641244,
97.8828085165069));
#30239=CARTESIAN_POINT('Ctrl Pts',(-0.233484411298407,2.50808307892834,
97.877447153775));
#30240=CARTESIAN_POINT('Ctrl Pts',(-0.14892416749316,2.5145138732317,97.872085791043));
#30241=CARTESIAN_POINT('Ctrl Pts',(-0.0643812861428095,2.51667663794827,
97.8667244283111));
#30242=CARTESIAN_POINT('Ctrl Pts',(0.0201615952075295,2.51883940266483,
97.8613630655791));
#30243=CARTESIAN_POINT('Ctrl Pts',(0.104686607816869,2.51673421722273,97.8560017028472));
#30244=CARTESIAN_POINT('Ctrl Pts',(0.188735567811208,2.51041533126353,97.8506403401152));
#30245=CARTESIAN_POINT('Ctrl Pts',(0.271121022824545,2.50422150929404,97.8453850899825));
#30246=CARTESIAN_POINT('Ctrl Pts',(0.353353400731598,2.49395643019617,97.8401298398498));
#30247=CARTESIAN_POINT('Ctrl Pts',(0.434998407716047,2.47963356875255,97.8348745897171));
#30248=CARTESIAN_POINT('Ctrl Pts',(0.516527660694896,2.46533101386097,97.8296267903309));
#30249=CARTESIAN_POINT('Ctrl Pts',(0.597470746163032,2.44698218284478,97.8243789909448));
#30250=CARTESIAN_POINT('Ctrl Pts',(0.677397134217739,2.42465242303997,97.8191311915586));
#30251=CARTESIAN_POINT('Ctrl Pts',(0.757902643912019,2.40216086877123,97.8138453682574));
#30252=CARTESIAN_POINT('Ctrl Pts',(0.837376188129912,2.37563048869662,97.8085595449563));
#30253=CARTESIAN_POINT('Ctrl Pts',(0.915386876163325,2.34518082819811,97.8032737216551));
#30254=CARTESIAN_POINT('Ctrl Pts',(0.992698061192939,2.31500420245316,97.7980352950553));
#30255=CARTESIAN_POINT('Ctrl Pts',(1.0685720813671,2.28097847213127,97.7927968684554));
#30256=CARTESIAN_POINT('Ctrl Pts',(1.14260514823941,2.24326987346971,97.7875584418555));
#30257=CARTESIAN_POINT('Ctrl Pts',(1.21661386686244,2.20557367654157,97.7823217380873));
#30258=CARTESIAN_POINT('Ctrl Pts',(1.28878242382462,2.16419722610919,97.7770850343192));
#30259=CARTESIAN_POINT('Ctrl Pts',(1.35872945084618,2.11935379995961,97.771848330551));
#30260=CARTESIAN_POINT('Ctrl Pts',(1.42867457252424,2.07451159533629,97.7666117694297));
#30261=CARTESIAN_POINT('Ctrl Pts',(1.49639789668942,2.0262028526693,97.7613752083083));
#30262=CARTESIAN_POINT('Ctrl Pts',(1.56154617747477,1.97468473068841,97.756138647187));
#30263=CARTESIAN_POINT('Ctrl Pts',(1.6277607400155,1.92232341172859,97.7508163792823));
#30264=CARTESIAN_POINT('Ctrl Pts',(1.69131481339937,1.86664700454359,97.7454941113776));
#30265=CARTESIAN_POINT('Ctrl Pts',(1.75187314508481,1.80796756982272,97.740171843473));
#30266=CARTESIAN_POINT('Ctrl Pts',(1.81154184846608,1.75015016159015,97.7349277620051));
#30267=CARTESIAN_POINT('Ctrl Pts',(1.86830196868316,1.68941775557057,97.7296836805371));
#30268=CARTESIAN_POINT('Ctrl Pts',(1.92187188685686,1.62610414811268,97.7244395990692));
#30269=CARTESIAN_POINT('Ctrl Pts',(1.97663985307147,1.56137458285676,97.7190782379462));
#30270=CARTESIAN_POINT('Ctrl Pts',(2.02807289226775,1.49394737715799,97.7137168768231));
#30271=CARTESIAN_POINT('Ctrl Pts',(2.07591649040969,1.42421100081594,97.7083555157001));
#30272=CARTESIAN_POINT('Ctrl Pts',(2.12376008855163,1.35447462447388,97.702994154577));
#30273=CARTESIAN_POINT('Ctrl Pts',(2.16801403661508,1.282429545401,97.697632793454));
#30274=CARTESIAN_POINT('Ctrl Pts',(2.20847437999406,1.20848962052218,97.692271432331));
#30275=CARTESIAN_POINT('Ctrl Pts',(2.24813392220464,1.1360131330067,97.6870161845993));
#30276=CARTESIAN_POINT('Ctrl Pts',(2.28429518581942,1.06144844418236,97.6817609368676));
#30277=CARTESIAN_POINT('Ctrl Pts',(2.31673302142714,0.985167172326145,97.6765056891359));
#30278=CARTESIAN_POINT('Ctrl Pts',(2.34912486754154,0.908994050011247,97.6712578921535));
#30279=CARTESIAN_POINT('Ctrl Pts',(2.37780359217612,0.83110959983421,97.6660100951711));
#30280=CARTESIAN_POINT('Ctrl Pts',(2.40258960547228,0.751910525047065,97.6607622981887));
#30281=CARTESIAN_POINT('Ctrl Pts',(2.42755522475012,0.672137552900731,97.655476474287));
#30282=CARTESIAN_POINT('Ctrl Pts',(2.44857125192748,0.59103123923539,97.6501906503852));
#30283=CARTESIAN_POINT('Ctrl Pts',(2.46550336138273,0.509018098902654,97.6449048264835));
#30284=CARTESIAN_POINT('Ctrl Pts',(2.4822836351284,0.427740396962234,97.6396664022767));
#30285=CARTESIAN_POINT('Ctrl Pts',(2.49505284639742,0.345572527047932,97.6344279780699));
#30286=CARTESIAN_POINT('Ctrl Pts',(2.50373058960798,0.262943691046724,97.6291895538631));
#30287=CARTESIAN_POINT('Ctrl Pts',(2.51240547886663,0.180342030166865,97.6239528524787));
#30288=CARTESIAN_POINT('Ctrl Pts',(2.51699152436522,0.0972801628280084,
97.6187161510943));
#30289=CARTESIAN_POINT('Ctrl Pts',(2.51745998530524,0.0141940969049517,
97.61347944971));
#30290=CARTESIAN_POINT('Ctrl Pts',(2.51792843348557,-0.068889705965877,
97.60824289096));
#30291=CARTESIAN_POINT('Ctrl Pts',(2.5142795185248,-0.151997244690935,97.60300633221));
#30292=CARTESIAN_POINT('Ctrl Pts',(2.50653661791235,-0.234692209211345,
97.59776977346));
#30293=CARTESIAN_POINT('Ctrl Pts',(2.49866698150394,-0.318740724897604,
97.5924475027172));
#30294=CARTESIAN_POINT('Ctrl Pts',(2.48656816229883,-0.402362547682886,
97.5871252319745));
#30295=CARTESIAN_POINT('Ctrl Pts',(2.47031938587987,-0.485106567411868,
97.5818029612317));
#30296=CARTESIAN_POINT('Ctrl Pts',(2.4543093266835,-0.566634961910552,97.5765588820805));
#30297=CARTESIAN_POINT('Ctrl Pts',(2.43427061054853,-0.647310735018868,
97.5713148029294));
#30298=CARTESIAN_POINT('Ctrl Pts',(2.41032989547979,-0.726715931404013,
97.5660707237782));
#30299=CARTESIAN_POINT('Ctrl Pts',(2.38585373007903,-0.807897078868578,
97.5607093572396));
#30300=CARTESIAN_POINT('Ctrl Pts',(2.3572990901666,-0.887749646995334,97.5553479907011));
#30301=CARTESIAN_POINT('Ctrl Pts',(2.32485325153221,-0.965848646962927,
97.5499866241625));
#30302=CARTESIAN_POINT('Ctrl Pts',(2.29240741289782,-1.04394764693051,97.5446252576239));
#30303=CARTESIAN_POINT('Ctrl Pts',(2.25607065422207,-1.12029264865219,97.5392638910854));
#30304=CARTESIAN_POINT('Ctrl Pts',(2.21607907323478,-1.19448725031742,97.5339025245468));
#30305=CARTESIAN_POINT('Ctrl Pts',(2.17687903689243,-1.26721333440516,97.5286472743675));
#30306=CARTESIAN_POINT('Ctrl Pts',(2.13402278743501,-1.33814201184334,97.5233920241881));
#30307=CARTESIAN_POINT('Ctrl Pts',(2.08769945270457,-1.40688210066694,97.5181367740087));
#30308=CARTESIAN_POINT('Ctrl Pts',(2.04144179405224,-1.47552473149299,97.5128889745931));
#30309=CARTESIAN_POINT('Ctrl Pts',(1.99172706954891,-1.54198455757053,97.5076411751774));
#30310=CARTESIAN_POINT('Ctrl Pts',(1.93879025308253,-1.60589495439526,97.5023933757618));
#30311=CARTESIAN_POINT('Ctrl Pts',(1.88546987337671,-1.67026842551265,97.4971075524702));
#30312=CARTESIAN_POINT('Ctrl Pts',(1.8288807370468,-1.73205494964748,97.4918217291785));
#30313=CARTESIAN_POINT('Ctrl Pts',(1.76930746740127,-1.7909096392052,97.4865359058869));
#30314=CARTESIAN_POINT('Ctrl Pts',(1.71026837691022,-1.84923659294294,97.4812974792991));
#30315=CARTESIAN_POINT('Ctrl Pts',(1.64829878907119,-1.90468374936841,97.4760590527113));
#30316=CARTESIAN_POINT('Ctrl Pts',(1.58371493837924,-1.95694998504163,97.4708206261234));
#30317=CARTESIAN_POINT('Ctrl Pts',(1.5191523284362,-2.00919903106177,97.4655839223828));
#30318=CARTESIAN_POINT('Ctrl Pts',(1.4519775216383,-2.05826894402127,97.4603472186421));
#30319=CARTESIAN_POINT('Ctrl Pts',(1.38254059026732,-2.10389823096634,97.4551105149015));
#30320=CARTESIAN_POINT('Ctrl Pts',(1.31310555054775,-2.14952627484517,97.4498739538229));
#30321=CARTESIAN_POINT('Ctrl Pts',(1.241408894964,-2.19171362653536,97.4446373927444));
#30322=CARTESIAN_POINT('Ctrl Pts',(1.16782932516116,-2.23024234496918,97.4394008316658));
#30323=CARTESIAN_POINT('Ctrl Pts',(1.09304547804947,-2.26940166319413,97.4340785637572));
#30324=CARTESIAN_POINT('Ctrl Pts',(1.01631695483261,-2.30478126619033,97.4287562958486));
#30325=CARTESIAN_POINT('Ctrl Pts',(0.938065276735081,-2.33620200038095,
97.42343402794));
#30326=CARTESIAN_POINT('Ctrl Pts',(0.860963151144127,-2.36716114978992,
97.4181899465517));
#30327=CARTESIAN_POINT('Ctrl Pts',(0.782382787729207,-2.39427687881259,
97.4129458651633));
#30328=CARTESIAN_POINT('Ctrl Pts',(0.702743723592735,-2.41742787047536,
97.407701783775));
#30329=CARTESIAN_POINT('Ctrl Pts',(0.621323594049227,-2.44109661596705,
97.4023404226063));
#30330=CARTESIAN_POINT('Ctrl Pts',(0.538797336628929,-2.46062102983402,
97.3969790614375));
#30331=CARTESIAN_POINT('Ctrl Pts',(0.455623389616077,-2.47592681168785,
97.3916177002688));
#30332=CARTESIAN_POINT('Ctrl Pts',(0.372449442603224,-2.49123259354168,
97.3862563391001));
#30333=CARTESIAN_POINT('Ctrl Pts',(0.288628318475212,-2.50231974297535,
97.3808949779313));
#30334=CARTESIAN_POINT('Ctrl Pts',(0.204621058188024,-2.50917047498691,
97.3755336167626));
#30335=CARTESIAN_POINT('Ctrl Pts',(0.122276388344548,-2.51588562393652,
97.3702783624686));
#30336=CARTESIAN_POINT('Ctrl Pts',(0.0394487396834575,-2.5185553615653,
97.3650231081747));
#30337=CARTESIAN_POINT('Ctrl Pts',(-0.0434307957414703,-2.51712534768955,
97.3597678538807));
#30338=CARTESIAN_POINT('Ctrl Pts',(-0.126192827362948,-2.51569736123914,
97.3545200503086));
#30339=CARTESIAN_POINT('Ctrl Pts',(-0.20900614212781,-2.51018117647843,
97.3492722467364));
#30340=CARTESIAN_POINT('Ctrl Pts',(-0.291435285714752,-2.50057427888882,
97.3440244431643));
#30341=CARTESIAN_POINT('Ctrl Pts',(-0.37446160251036,-2.49089778234903,
97.3387386209066));
#30342=CARTESIAN_POINT('Ctrl Pts',(-0.457097685928118,-2.4770710125533,
97.3334527986488));
#30343=CARTESIAN_POINT('Ctrl Pts',(-0.538899284068818,-2.45914493505977,
97.3281669763911));
#30344=CARTESIAN_POINT('Ctrl Pts',(-0.619967468262847,-2.44137957857343,
97.3229285455762));
#30345=CARTESIAN_POINT('Ctrl Pts',(-0.700215611826423,-2.41958822747458,
97.3176901147613));
#30346=CARTESIAN_POINT('Ctrl Pts',(-0.779218959865339,-2.3938721901109,
97.3124516839464));
#30347=CARTESIAN_POINT('Ctrl Pts',(-0.858196325055373,-2.36816461031174,
97.3072149759618));
#30348=CARTESIAN_POINT('Ctrl Pts',(-0.935929269381141,-2.33853505047875,
97.3019782679771));
#30349=CARTESIAN_POINT('Ctrl Pts',(-1.01200785669301,-2.30513477870419,
97.2967415599924));
#30350=CARTESIAN_POINT('Ctrl Pts',(-1.08808437157927,-2.27173541677274,
97.2915049946588));
#30351=CARTESIAN_POINT('Ctrl Pts',(-1.16250619697185,-2.23456573355622,
97.2862684293251));
#30352=CARTESIAN_POINT('Ctrl Pts',(-1.23488434042773,-2.19382472311859,
97.2810318639915));
#30353=CARTESIAN_POINT('Ctrl Pts',(-1.3084469686825,-2.15241697676801,97.2757096010737));
#30354=CARTESIAN_POINT('Ctrl Pts',(-1.37989798599608,-2.10732018730508,
97.270387338156));
#30355=CARTESIAN_POINT('Ctrl Pts',(-1.44885762334226,-2.05879038206492,
97.2650650752382));
#30356=CARTESIAN_POINT('Ctrl Pts',(-1.51680433109064,-2.01097341810402,
97.2598209896115));
#30357=CARTESIAN_POINT('Ctrl Pts',(-1.58233203236523,-1.95982395866017,
97.2545769039847));
#30358=CARTESIAN_POINT('Ctrl Pts',(-1.64511054929148,-1.90562785732417,
97.249332818358));
#30359=CARTESIAN_POINT('Ctrl Pts',(-1.70929289180417,-1.85021984660473,
97.2439714667947));
#30360=CARTESIAN_POINT('Ctrl Pts',(-1.7706012442335,-1.79162764845339,97.2386101152315));
#30361=CARTESIAN_POINT('Ctrl Pts',(-1.82872368836751,-1.73019534203613,
97.2332487636682));
#30362=CARTESIAN_POINT('Ctrl Pts',(-1.88684613250151,-1.66876303561888,
97.2278874121049));
#30363=CARTESIAN_POINT('Ctrl Pts',(-1.94178238898331,-1.60449105056951,
97.2225260605417));
#30364=CARTESIAN_POINT('Ctrl Pts',(-1.9932665267309,-1.53775641875237,97.2171647089784));
#30365=CARTESIAN_POINT('Ctrl Pts',(-2.04375879578633,-1.47230746432789,
97.2119066466416));
#30366=CARTESIAN_POINT('Ctrl Pts',(-2.09112029805458,-1.40424435744742,
97.2066485843049));
#30367=CARTESIAN_POINT('Ctrl Pts',(-2.13506935929913,-1.33389845227514,
97.2013905219681));
#30368=CARTESIAN_POINT('Ctrl Pts',(-2.1789570760028,-1.26365073662348,97.1961397988875));
#30369=CARTESIAN_POINT('Ctrl Pts',(-2.21944156720512,-1.19112693546319,
97.1908890758069));
#30370=CARTESIAN_POINT('Ctrl Pts',(-2.25628201011796,-1.11669053045957,
97.1856383527263));
#30371=CARTESIAN_POINT('Ctrl Pts',(-2.29308207556009,-1.04233570845343,
97.1803933844874));
#30372=CARTESIAN_POINT('Ctrl Pts',(-2.32624582231096,-0.966072856005633,
97.1751484162485));
#30373=CARTESIAN_POINT('Ctrl Pts',(-2.35557701969086,-0.888292268515459,
97.1699034480096));
#30374=CARTESIAN_POINT('Ctrl Pts',(-2.38488563777284,-0.810571556898563,
97.1646625173727));
#30375=CARTESIAN_POINT('Ctrl Pts',(-2.41036740587786,-0.73133586059678,
97.1594215867358));
#30376=CARTESIAN_POINT('Ctrl Pts',(-2.431873704451,-0.650996571112148,97.1541806560988));
#30377=CARTESIAN_POINT('Ctrl Pts',(-2.45337004841148,-0.570694468245425,
97.1489421513296));
#30378=CARTESIAN_POINT('Ctrl Pts',(-2.4708944621029,-0.489290231623965,
97.1437036465604));
#30379=CARTESIAN_POINT('Ctrl Pts',(-2.48434821360103,-0.407210269489083,
97.1384651417911));
#30380=CARTESIAN_POINT('Ctrl Pts',(-2.497803310619,-0.325122098475233,97.1332261131151));
#30381=CARTESIAN_POINT('Ctrl Pts',(-2.50718685030444,-0.242358519957874,
97.127987084439));
#30382=CARTESIAN_POINT('Ctrl Pts',(-2.51245144076967,-0.159354974112484,
97.1227480557629));
#30383=CARTESIAN_POINT('Ctrl Pts',(-2.51585622350457,-0.105673867918983,
97.1193598046726));
#30384=CARTESIAN_POINT('Ctrl Pts',(-2.51753925219785,-0.0518925558902497,
97.1159715535823));
#30385=CARTESIAN_POINT('Ctrl Pts',(-2.51749930506904,0.0018705552357781,
97.112583302492));
#30386=CARTESIAN_POINT('Ctrl Pts',(-2.51749930506837,0.00187055614564556,
97.1125833024347));
#30387=CARTESIAN_POINT('Ctrl Pts',(-2.51742786227618,0.0980222702224651,
97.1065236428793));
#30388=CARTESIAN_POINT('Ctrl Pts',(-2.51184391378265,0.193950035127749,
97.100463983324));
#30389=CARTESIAN_POINT('Ctrl Pts',(-2.5008479055551,0.28907784986171,97.0944043237686));
#30390=CARTESIAN_POINT('Ctrl Pts',(-2.48974553226095,0.385125841821851,
97.0882860487522));
#30391=CARTESIAN_POINT('Ctrl Pts',(-2.47312598902194,0.480358183904104,
97.0821677737357));
#30392=CARTESIAN_POINT('Ctrl Pts',(-2.45114231090937,0.574201725589434,
97.0760494987193));
#30393=CARTESIAN_POINT('Ctrl Pts',(-2.43047745948084,0.662415482929026,
97.070298266211));
#30394=CARTESIAN_POINT('Ctrl Pts',(-2.40507329585502,0.749402171584247,
97.0645470337027));
#30395=CARTESIAN_POINT('Ctrl Pts',(-2.37509517890798,0.834703025709186,
97.0587958011944));
#30396=CARTESIAN_POINT('Ctrl Pts',(-2.37064303349584,0.84737132662399,97.0579416673783));
#30397=CARTESIAN_POINT('Ctrl Pts',(-2.36608819785996,0.860007796311788,
97.0570875335623));
#30398=CARTESIAN_POINT('Ctrl Pts',(-2.36143112101025,0.872610629504516,
97.0562333997462));
#30399=CARTESIAN_POINT('Ctrl Pts',(-2.36143105416443,0.872610810400539,
97.3312318328322));
#30400=CARTESIAN_POINT('Ctrl Pts',(-2.37281360699947,0.841807715343776,
97.3331208944054));
#30401=CARTESIAN_POINT('Ctrl Pts',(-2.38359750920899,0.810770938666179,
97.3350072777569));
#30402=CARTESIAN_POINT('Ctrl Pts',(-2.43975997246009,0.638304921164849,
97.3454324317484));
#30403=CARTESIAN_POINT('Ctrl Pts',(-2.47315310182676,0.493318849580991,
97.3539746313534));
#30404=CARTESIAN_POINT('Ctrl Pts',(-2.4960546078397,0.328394506053,97.364251471772));
#30405=CARTESIAN_POINT('Ctrl Pts',(-2.49834319432965,0.310504101672879,
97.3653736840554));
#30406=CARTESIAN_POINT('Ctrl Pts',(-2.50142261429291,0.284187858038864,
97.3670373345829));
#30407=CARTESIAN_POINT('Ctrl Pts',(-2.50236355938732,0.275779705033789,
97.3675708097129));
#30408=CARTESIAN_POINT('Ctrl Pts',(-2.50395522976449,0.260877467930617,
97.3685199899254));
#30409=CARTESIAN_POINT('Ctrl Pts',(-2.5046231096316,0.254385383389946,97.3689347384058));
#30410=CARTESIAN_POINT('Ctrl Pts',(-2.5060161268914,0.240307085286784,97.3698368928681));
#30411=CARTESIAN_POINT('Ctrl Pts',(-2.5067320546669,0.23272027399879,97.3703247764144));
#30412=CARTESIAN_POINT('Ctrl Pts',(-2.50862130915018,0.211678508054357,
97.3716824300492));
#30413=CARTESIAN_POINT('Ctrl Pts',(-2.50972080149989,0.198217413372497,
97.3725560894118));
#30414=CARTESIAN_POINT('Ctrl Pts',(-2.51520391391042,0.123702507622724,
97.3774182431325));
#30415=CARTESIAN_POINT('Ctrl Pts',(-2.51746761848308,0.0625181454298513,
97.381506471314));
#30416=CARTESIAN_POINT('Ctrl Pts',(-2.51756609999443,-0.125612640580314,
97.3942560028986));
#30417=CARTESIAN_POINT('Ctrl Pts',(-2.50803295207504,-0.252362804816378,
97.4030866037753));
#30418=CARTESIAN_POINT('Ctrl Pts',(-2.46462296398122,-0.538313904815139,
97.4230024390044));
#30419=CARTESIAN_POINT('Ctrl Pts',(-2.42479939024921,-0.696069878556848,
97.43396711388));
#30420=CARTESIAN_POINT('Ctrl Pts',(-2.36255428111609,-0.869849386733493,
97.4458725758867));
#30421=CARTESIAN_POINT('Ctrl Pts',(-2.3547789886642,-0.890683250745074,
97.447297645885));
#30422=CARTESIAN_POINT('Ctrl Pts',(-2.34151978796341,-0.924823405229062,
97.4496297518918));
#30423=CARTESIAN_POINT('Ctrl Pts',(-2.33619613767803,-0.938190209165906,
97.4505420374371));
#30424=CARTESIAN_POINT('Ctrl Pts',(-2.32637072677582,-0.962257885902154,
97.4521834466888));
#30425=CARTESIAN_POINT('Ctrl Pts',(-2.32190901852356,-0.972974570252401,
97.4529138842239));
#30426=CARTESIAN_POINT('Ctrl Pts',(-2.31217600757012,-0.995904257287378,
97.4544759803793));
#30427=CARTESIAN_POINT('Ctrl Pts',(-2.30688169462198,-1.00810715574672,
97.4553068381418));
#30428=CARTESIAN_POINT('Ctrl Pts',(-2.29211353583333,-1.04142074762595,
97.4575741538986));
#30429=CARTESIAN_POINT('Ctrl Pts',(-2.28244482868597,-1.06244401903929,
97.4590039806668));
#30430=CARTESIAN_POINT('Ctrl Pts',(-2.22368670639655,-1.18569999899059,
97.4673861007413));
#30431=CARTESIAN_POINT('Ctrl Pts',(-2.16802172990752,-1.28466082291107,
97.4741048865652));
#30432=CARTESIAN_POINT('Ctrl Pts',(-2.00862344146145,-1.5279820934026,97.4910267562332));
#30433=CARTESIAN_POINT('Ctrl Pts',(-1.89596563923792,-1.66571423925124,
97.5009880948812));
#30434=CARTESIAN_POINT('Ctrl Pts',(-1.72548688834964,-1.83422429670881,
97.5151821352445));
#30435=CARTESIAN_POINT('Ctrl Pts',(-1.67959545783295,-1.87633725813853,
97.5189354148818));
#30436=CARTESIAN_POINT('Ctrl Pts',(-1.62185931615923,-1.92550328180932,
97.5236461257159));
#30437=CARTESIAN_POINT('Ctrl Pts',(-1.6114532467947,-1.93422050036199,97.524494741165));
#30438=CARTESIAN_POINT('Ctrl Pts',(-1.59508430424113,-1.9477090706605,97.5258299005359));
#30439=CARTESIAN_POINT('Ctrl Pts',(-1.58916917786768,-1.95253831768638,
97.5263124320269));
#30440=CARTESIAN_POINT('Ctrl Pts',(-1.57815940811866,-1.96144378031291,
97.5272108591022));
#30441=CARTESIAN_POINT('Ctrl Pts',(-1.57307080034118,-1.96552717471724,
97.5276262361295));
#30442=CARTESIAN_POINT('Ctrl Pts',(-1.56136463829118,-1.97484630301446,
97.5285820694113));
#30443=CARTESIAN_POINT('Ctrl Pts',(-1.55473661388178,-1.98006856214416,
97.5291234435864));
#30444=CARTESIAN_POINT('Ctrl Pts',(-1.53395297274917,-1.99627542486301,
97.5308212762787));
#30445=CARTESIAN_POINT('Ctrl Pts',(-1.51970661315254,-2.00714201324545,
97.5319854075817));
#30446=CARTESIAN_POINT('Ctrl Pts',(-1.38684868636179,-2.10625573571253,
97.5428356343875));
#30447=CARTESIAN_POINT('Ctrl Pts',(-1.26080637835686,-2.18403785035919,
97.5530668564912));
#30448=CARTESIAN_POINT('Ctrl Pts',(-0.965154630837059,-2.33232762971752,
97.5759159329082));
#30449=CARTESIAN_POINT('Ctrl Pts',(-0.793143586764814,-2.39629326884446,
97.5884284569396));
#30450=CARTESIAN_POINT('Ctrl Pts',(-0.584032937634819,-2.44903611769644,
97.6024378858756));
#30451=CARTESIAN_POINT('Ctrl Pts',(-0.552219357105514,-2.45640516265882,
97.6045396653788));
#30452=CARTESIAN_POINT('Ctrl Pts',(-0.505542694743742,-2.46626426174268,
97.607581697783));
#30453=CARTESIAN_POINT('Ctrl Pts',(-0.49078737478013,-2.46924291914619,
97.6085373118365));
#30454=CARTESIAN_POINT('Ctrl Pts',(-0.464508867927245,-2.47430290094711,
97.6102287752873));
#30455=CARTESIAN_POINT('Ctrl Pts',(-0.452996317369128,-2.47643648776811,
97.6109662560458));
#30456=CARTESIAN_POINT('Ctrl Pts',(-0.42890120789017,-2.48072831406022,
97.6125025311236));
#30457=CARTESIAN_POINT('Ctrl Pts',(-0.416316248486393,-2.4828713227058,
97.6133008263237));
#30458=CARTESIAN_POINT('Ctrl Pts',(-0.383306797932391,-2.48823424366376,
97.6153842761601));
#30459=CARTESIAN_POINT('Ctrl Pts',(-0.362857724829885,-2.49129846940272,
97.6166645270829));
#30460=CARTESIAN_POINT('Ctrl Pts',(-0.267674308370134,-2.50436453327672,
97.6225781716718));
#30461=CARTESIAN_POINT('Ctrl Pts',(-0.192548483506289,-2.51125823788772,
97.6271141508825));
#30462=CARTESIAN_POINT('Ctrl Pts',(0.0329049403354752,-2.52176727470881,
97.6404646416206));
#30463=CARTESIAN_POINT('Ctrl Pts',(0.183355378832519,-2.51530830826447,
97.6490107494887));
#30464=CARTESIAN_POINT('Ctrl Pts',(0.373159109006744,-2.49003104900377,
97.6600477066965));
#30465=CARTESIAN_POINT('Ctrl Pts',(0.41384196790483,-2.4835935711914,97.6624301333511));
#30466=CARTESIAN_POINT('Ctrl Pts',(0.541589500905969,-2.46015333929717,
97.6700105540017));
#30467=CARTESIAN_POINT('Ctrl Pts',(0.627915115593771,-2.43954765955099,
97.6752791662137));
#30468=CARTESIAN_POINT('Ctrl Pts',(0.725915818944569,-2.41060881689443,
97.6816141425477));
#30469=CARTESIAN_POINT('Ctrl Pts',(0.73883693893511,-2.4066799960731,97.6824566408256));
#30470=CARTESIAN_POINT('Ctrl Pts',(0.759689854632868,-2.40015566475958,
97.683829012624));
#30471=CARTESIAN_POINT('Ctrl Pts',(0.767641641638585,-2.39762428158098,
97.6843553392976));
#30472=CARTESIAN_POINT('Ctrl Pts',(0.781780759349992,-2.3930456677565,97.6852968055591));
#30473=CARTESIAN_POINT('Ctrl Pts',(0.787972913074359,-2.39101388752923,
97.685711048318));
#30474=CARTESIAN_POINT('Ctrl Pts',(0.801467635600247,-2.38652786011651,
97.6866180953795));
#30475=CARTESIAN_POINT('Ctrl Pts',(0.80876674422791,-2.38406416601737,97.6871114238652));
#30476=CARTESIAN_POINT('Ctrl Pts',(0.829554481414299,-2.37694115740719,
97.6885239521368));
#30477=CARTESIAN_POINT('Ctrl Pts',(0.843014704381204,-2.3722006848545,97.6894476566685));
#30478=CARTESIAN_POINT('Ctrl Pts',(0.938476132205947,-2.33766565653956,
97.6960598512106));
#30479=CARTESIAN_POINT('Ctrl Pts',(1.01891205295563,-2.30374329211678,97.701951990921));
#30480=CARTESIAN_POINT('Ctrl Pts',(1.25530101938894,-2.18924675681002,97.7199373960713));
#30481=CARTESIAN_POINT('Ctrl Pts',(1.4047781191554,-2.09647082363536,97.7321929472169));
#30482=CARTESIAN_POINT('Ctrl Pts',(1.61480439854475,-1.93348986294657,97.7500969924981));
#30483=CARTESIAN_POINT('Ctrl Pts',(1.6831840653497,-1.87426544511501,97.7560645103172));
#30484=CARTESIAN_POINT('Ctrl Pts',(1.76434277940056,-1.79594037453304,97.7633239603216));
#30485=CARTESIAN_POINT('Ctrl Pts',(1.78024138223736,-1.78018199797686,97.7647553930719));
#30486=CARTESIAN_POINT('Ctrl Pts',(1.80522386420587,-1.7547504113409,97.7670203718386));
#30487=CARTESIAN_POINT('Ctrl Pts',(1.81444480277616,-1.74521410566861,97.7678598736036));
#30488=CARTESIAN_POINT('Ctrl Pts',(1.83151923951415,-1.72727409646956,97.7694211815081));
#30489=CARTESIAN_POINT('Ctrl Pts',(1.83939131515179,-1.71888863101991,97.7701437749559));
#30490=CARTESIAN_POINT('Ctrl Pts',(1.85697936031183,-1.69989436070961,97.7717646610353));
#30491=CARTESIAN_POINT('Ctrl Pts',(1.86666247374198,-1.68925557713864,97.7726615524833));
#30492=CARTESIAN_POINT('Ctrl Pts',(1.89514449671421,-1.65741856707189,97.7753137545754));
#30493=CARTESIAN_POINT('Ctrl Pts',(1.91367771442445,-1.63598492486266,97.7770580744112));
#30494=CARTESIAN_POINT('Ctrl Pts',(1.95519658948156,-1.58629717841548,97.781012928919));
#30495=CARTESIAN_POINT('Ctrl Pts',(1.97793909233074,-1.55784773918961,97.7832139894324));
#30496=CARTESIAN_POINT('Ctrl Pts',(2.05340073033681,-1.45913217464225,97.7906550455423));
#30497=CARTESIAN_POINT('Ctrl Pts',(2.10305847857833,-1.38660305518453,97.7957907029949));
#30498=CARTESIAN_POINT('Ctrl Pts',(2.21176121903907,-1.20851578406784,97.8078604249669));
#30499=CARTESIAN_POINT('Ctrl Pts',(2.26719228766116,-1.10101592713616,97.8147271602574));
#30500=CARTESIAN_POINT('Ctrl Pts',(2.35277925420826,-0.900898334255344,
97.8273884471995));
#30501=CARTESIAN_POINT('Ctrl Pts',(2.38569165680028,-0.809727726736834,
97.8331180783741));
#30502=CARTESIAN_POINT('Ctrl Pts',(2.41713426828811,-0.703883902727919,
97.8399625019929));
#30503=CARTESIAN_POINT('Ctrl Pts',(2.42089544100432,-0.690837075177546,
97.84080946823));
#30504=CARTESIAN_POINT('Ctrl Pts',(2.42680329825976,-0.669702922670512,
97.8421876990666));
#30505=CARTESIAN_POINT('Ctrl Pts',(2.42901558002388,-0.661634007846177,
97.8427153674314));
#30506=CARTESIAN_POINT('Ctrl Pts',(2.43287986613074,-0.64725906828058,97.8436582710199));
#30507=CARTESIAN_POINT('Ctrl Pts',(2.43454765282329,-0.640957462791354,
97.8440725981799));
#30508=CARTESIAN_POINT('Ctrl Pts',(2.43812898014234,-0.627210032828775,
97.844978679935));
#30509=CARTESIAN_POINT('Ctrl Pts',(2.44003286808013,-0.619762009187752,
97.8454709496951));
#30510=CARTESIAN_POINT('Ctrl Pts',(2.44535500699364,-0.598537073706251,
97.8468774756022));
#30511=CARTESIAN_POINT('Ctrl Pts',(2.44869082809743,-0.584740066337355,
97.8477961784328));
#30512=CARTESIAN_POINT('Ctrl Pts',(2.47119225778582,-0.488103299000273,
97.8542581964196));
#30513=CARTESIAN_POINT('Ctrl Pts',(2.48626500098483,-0.404375197363053,
97.8599950908284));
#30514=CARTESIAN_POINT('Ctrl Pts',(2.51843418994899,-0.153390808775393,
97.8773090953986));
#30515=CARTESIAN_POINT('Ctrl Pts',(2.52305792026864,0.0150097981747123,
97.8890468033371));
#30516=CARTESIAN_POINT('Ctrl Pts',(2.50367702977971,0.281486739478573,97.9071101364023));
#30517=CARTESIAN_POINT('Ctrl Pts',(2.49065193401831,0.379856090177702,97.9136746690665));
#30518=CARTESIAN_POINT('Ctrl Pts',(2.46751176654368,0.499717209907458,97.9215361462574));
#30519=CARTESIAN_POINT('Ctrl Pts',(2.46285971084279,0.52216253155518,97.9230025477102));
#30520=CARTESIAN_POINT('Ctrl Pts',(2.45500600072512,0.557611869986909,97.9253100364121));
#30521=CARTESIAN_POINT('Ctrl Pts',(2.45200611315563,0.570658824034685,97.9261574654601));
#30522=CARTESIAN_POINT('Ctrl Pts',(2.44621270862469,0.594965715610145,97.9277330328811));
#30523=CARTESIAN_POINT('Ctrl Pts',(2.44344516872562,0.606231418903919,97.9284619759452));
#30524=CARTESIAN_POINT('Ctrl Pts',(2.43709915709077,0.631314225543083,97.9300822381141));
#30525=CARTESIAN_POINT('Ctrl Pts',(2.43348083657293,0.645120906622737,97.9309722576839));
#30526=CARTESIAN_POINT('Ctrl Pts',(2.42247660915201,0.685700083069867,97.9335832009061));
#30527=CARTESIAN_POINT('Ctrl Pts',(2.41476474117469,0.712382526551963,97.9352936517657));
#30528=CARTESIAN_POINT('Ctrl Pts',(2.35655958860768,0.901949523238102,97.9474117363831));
#30529=CARTESIAN_POINT('Ctrl Pts',(2.29007199876082,1.05946486753853,97.9572603741884));
#30530=CARTESIAN_POINT('Ctrl Pts',(2.1295535704852,1.35262596591857,97.9764676837467));
#30531=CARTESIAN_POINT('Ctrl Pts',(2.03714445278447,1.48816101619655,97.9857982361846));
#30532=CARTESIAN_POINT('Ctrl Pts',(1.91922667862163,1.62935212838372,97.9971107436977));
#30533=CARTESIAN_POINT('Ctrl Pts',(1.9060093580292,1.64479411141045,97.9983718362741));
#30534=CARTESIAN_POINT('Ctrl Pts',(1.88717425850953,1.66626751902552,98.0001621293693));
#30535=CARTESIAN_POINT('Ctrl Pts',(1.88171123466018,1.67243443872519,98.0006806102809));
#30536=CARTESIAN_POINT('Ctrl Pts',(1.87177189059984,1.68354409123085,98.0016227541463));
#30537=CARTESIAN_POINT('Ctrl Pts',(1.86730596417978,1.68849612148886,98.0020456548498));
#30538=CARTESIAN_POINT('Ctrl Pts',(1.85811715520747,1.69860406692417,98.0029150677586));
#30539=CARTESIAN_POINT('Ctrl Pts',(1.85339239879728,1.70375812598781,98.003361713218));
#30540=CARTESIAN_POINT('Ctrl Pts',(1.84116827032712,1.71698194887245,98.0045161294051));
#30541=CARTESIAN_POINT('Ctrl Pts',(1.83363738124604,1.72502218997871,98.0052262073246));
#30542=CARTESIAN_POINT('Ctrl Pts',(1.80149276094251,1.75889258294977,98.0082513718593));
#30543=CARTESIAN_POINT('Ctrl Pts',(1.77638541763499,1.78424601136328,98.010600178534));
#30544=CARTESIAN_POINT('Ctrl Pts',(1.70600382410769,1.85235918542044,98.0171255345371));
#30545=CARTESIAN_POINT('Ctrl Pts',(1.65966977088861,1.89398491661036,98.021356958145));
#30546=CARTESIAN_POINT('Ctrl Pts',(1.45949304357544,2.06083033133244,98.0392252916538));
#30547=CARTESIAN_POINT('Ctrl Pts',(1.29264373078522,2.16938535835508,98.0530775030175));
#30548=CARTESIAN_POINT('Ctrl Pts',(1.05487407908419,2.28681219353953,98.0707212031858));
#30549=CARTESIAN_POINT('Ctrl Pts',(0.993816664272778,2.31400067528736,98.0750932092784));
#30550=CARTESIAN_POINT('Ctrl Pts',(0.912634475287457,2.34634348291541,98.0807050057469));
#30551=CARTESIAN_POINT('Ctrl Pts',(0.893430985698294,2.35372269822172,98.0820182144541));
#30552=CARTESIAN_POINT('Ctrl Pts',(0.862188682874349,2.36529053315015,98.0841322197037));
#30553=CARTESIAN_POINT('Ctrl Pts',(0.850205041001811,2.36962444894422,98.0849377954015));
#30554=CARTESIAN_POINT('Ctrl Pts',(0.82714203928663,2.37776776459769,98.0864782088236));
#30555=CARTESIAN_POINT('Ctrl Pts',(0.816068012450916,2.38159117020877,98.0872134910557));
#30556=CARTESIAN_POINT('Ctrl Pts',(0.790415201640926,2.39024809314571,98.0889068928647));
#30557=CARTESIAN_POINT('Ctrl Pts',(0.775817973468088,2.39502580910364,98.0898631673919));
#30558=CARTESIAN_POINT('Ctrl Pts',(0.729311286397423,2.4097777775398,98.0928873979151));
#30559=CARTESIAN_POINT('Ctrl Pts',(0.697245641753475,2.41925041389897,98.0949391141746));
#30560=CARTESIAN_POINT('Ctrl Pts',(0.621526012239214,2.43998839888775,98.0997129787148));
#30561=CARTESIAN_POINT('Ctrl Pts',(0.577738804714182,2.45072564443698,98.1024188331686));
#30562=CARTESIAN_POINT('Ctrl Pts',(0.412167792175033,2.48664135144035,98.1124820576477));
#30563=CARTESIAN_POINT('Ctrl Pts',(0.288858932063695,2.50396302351564,98.1196283491873));
#30564=CARTESIAN_POINT('Ctrl Pts',(0.00999197980473201,2.52225415536473,
98.1356859488692));
#30565=CARTESIAN_POINT('Ctrl Pts',(-0.145374015523826,2.51807852617538,
98.1445612025003));
#30566=CARTESIAN_POINT('Ctrl Pts',(-0.320034961545601,2.49716201287453,
98.1553717404444));
#30567=CARTESIAN_POINT('Ctrl Pts',(-0.340693341883785,2.49442748484183,
98.1566640006003));
#30568=CARTESIAN_POINT('Ctrl Pts',(-0.369554961381498,2.49024189827448,
98.1584914767358));
#30569=CARTESIAN_POINT('Ctrl Pts',(-0.37778919061541,2.48900600727672,98.1590153791614));
#30570=CARTESIAN_POINT('Ctrl Pts',(-0.392032409704921,2.48679590962537,
98.1599262092788));
#30571=CARTESIAN_POINT('Ctrl Pts',(-0.398044337151493,2.48584070490485,
98.1603120853364));
#30572=CARTESIAN_POINT('Ctrl Pts',(-0.410779453852282,2.4837699040808,98.1611326209815));
#30573=CARTESIAN_POINT('Ctrl Pts',(-0.417501659141065,2.48264879867973,
98.1615675953625));
#30574=CARTESIAN_POINT('Ctrl Pts',(-0.434271712197452,2.47978191339147,
98.1626572341668));
#30575=CARTESIAN_POINT('Ctrl Pts',(-0.444313569685101,2.47800236104002,
98.1633137434831));
#30576=CARTESIAN_POINT('Ctrl Pts',(-0.482813842093714,2.47093805198034,
98.1658455797619));
#30577=CARTESIAN_POINT('Ctrl Pts',(-0.511189933465595,2.46522387326448,
98.1677427031991));
#30578=CARTESIAN_POINT('Ctrl Pts',(-0.584482348915421,2.44914499920631,
98.1727128230025));
#30579=CARTESIAN_POINT('Ctrl Pts',(-0.629222723096888,2.43803386323016,
98.1758154574126));
#30580=CARTESIAN_POINT('Ctrl Pts',(-0.880760921333106,2.3681803775212,98.1935628479852));
#30581=CARTESIAN_POINT('Ctrl Pts',(-1.07970973780586,2.28435230278158,98.2086755042068));
#30582=CARTESIAN_POINT('Ctrl Pts',(-1.32909493024918,2.1393249064049,98.2279415870915));
#30583=CARTESIAN_POINT('Ctrl Pts',(-1.39096536804762,2.09962413853786,98.2327625031926));
#30584=CARTESIAN_POINT('Ctrl Pts',(-1.46840891681978,2.04500232739952,98.2388531113517));
#30585=CARTESIAN_POINT('Ctrl Pts',(-1.4856462269452,2.03251435416267,98.2402126481037));
#30586=CARTESIAN_POINT('Ctrl Pts',(-1.51307201845986,2.01210975986223,98.2423826259386));
#30587=CARTESIAN_POINT('Ctrl Pts',(-1.52336133202795,2.00433103077238,98.2431983202902));
#30588=CARTESIAN_POINT('Ctrl Pts',(-1.54245930445251,1.98966092816235,98.2447154926867));
#30589=CARTESIAN_POINT('Ctrl Pts',(-1.55128266346323,1.9827893028434,98.2454177155535));
#30590=CARTESIAN_POINT('Ctrl Pts',(-1.56020685970427,1.97574311081126,98.2461293512056));
#30591=CARTESIAN_POINT('Ctrl Pts',(-1.56035365021658,1.97562718427395,98.246141056998));
#30592=CARTESIAN_POINT('Ctrl Pts',(-1.56063564896794,1.97540442716535,98.2461635456943));
#30593=CARTESIAN_POINT('Ctrl Pts',(-1.56077085916982,1.97529759906207,98.2461743286966));
#30594=CARTESIAN_POINT('Ctrl Pts',(-1.56103095389672,1.97509205768155,98.2461950718576));
#30595=CARTESIAN_POINT('Ctrl Pts',(-1.56115584001412,1.97499334645215,98.2462050320954));
#30596=CARTESIAN_POINT('Ctrl Pts',(-1.5613963655788,1.97480319558456,98.2462242156443));
#30597=CARTESIAN_POINT('Ctrl Pts',(-1.56151200635576,1.97471175763465,98.2462334390217));
#30598=CARTESIAN_POINT('Ctrl Pts',(-1.56173497338694,1.97453542425206,98.2462512230814));
#30599=CARTESIAN_POINT('Ctrl Pts',(-1.56184230074504,1.97445053023103,98.2462597838186));
#30600=CARTESIAN_POINT('Ctrl Pts',(-1.57332625660252,1.96536540422798,98.2471757991006));
#30601=CARTESIAN_POINT('Ctrl Pts',(-1.58462507082855,1.9562668735716,98.2480793652999));
#30602=CARTESIAN_POINT('Ctrl Pts',(-1.60839911360544,1.93678135824142,98.2499859344445));
#30603=CARTESIAN_POINT('Ctrl Pts',(-1.62085383291634,1.92637031992174,98.2509879338353));
#30604=CARTESIAN_POINT('Ctrl Pts',(-1.65367260613589,1.89839310099913,98.2536376247734));
#30605=CARTESIAN_POINT('Ctrl Pts',(-1.67385768124324,1.88061957821771,98.2552770552511));
#30606=CARTESIAN_POINT('Ctrl Pts',(-1.73513503392139,1.82489481040161,98.2602896863143));
#30607=CARTESIAN_POINT('Ctrl Pts',(-1.77525158559537,1.78589391181513,98.2636217760274));
#30608=CARTESIAN_POINT('Ctrl Pts',(-1.88291529018487,1.674008331585,98.2727640849382));
#30609=CARTESIAN_POINT('Ctrl Pts',(-1.94749849400705,1.59841324201354,98.2784799864133));
#30610=CARTESIAN_POINT('Ctrl Pts',(-2.10473141360437,1.39064773189292,98.2934522043514));
#30611=CARTESIAN_POINT('Ctrl Pts',(-2.18942968502766,1.2530678219741,98.3026522644494));
#30612=CARTESIAN_POINT('Ctrl Pts',(-2.26939443951164,1.08998799169555,98.3138197982368));
#30613=CARTESIAN_POINT('Ctrl Pts',(-2.27817843654644,1.07150729995071,98.315089157258));
#30614=CARTESIAN_POINT('Ctrl Pts',(-2.29019145720924,1.04541743011927,98.3168893207269));
#30615=CARTESIAN_POINT('Ctrl Pts',(-2.29361002473671,1.03789573840632,98.3174092495864));
#30616=CARTESIAN_POINT('Ctrl Pts',(-2.29972322432121,1.02426749049372,98.3183532289286));
#30617=CARTESIAN_POINT('Ctrl Pts',(-2.30243074466243,1.01816671774747,98.3187765072962));
#30618=CARTESIAN_POINT('Ctrl Pts',(-2.3079211188865,1.00566153320459,98.3196456999727));
#30619=CARTESIAN_POINT('Ctrl Pts',(-2.31070163110441,0.999256213157136,
98.3200917410988));
#30620=CARTESIAN_POINT('Ctrl Pts',(-2.3177835515073,0.98275434443663,98.3212428388734));
#30621=CARTESIAN_POINT('Ctrl Pts',(-2.32204559785041,0.972641210403324,
98.3219501782195));
#30622=CARTESIAN_POINT('Ctrl Pts',(-2.33854544639524,0.932763185612064,
98.324745857215));
#30623=CARTESIAN_POINT('Ctrl Pts',(-2.35027748300159,0.902794249797349,
98.3268610144102));
#30624=CARTESIAN_POINT('Ctrl Pts',(-2.36143112099219,0.872610629553384,
98.3289997116198));
#30625=CARTESIAN_POINT('Origin',(0.,0.,104.));
#30626=CARTESIAN_POINT('',(-2.36143108732087,0.87261072067364,99.3329358985331));
#30627=CARTESIAN_POINT('',(-2.36143112101025,0.872610629504521,99.0561732563161));
#30628=CARTESIAN_POINT('',(-2.36143112101026,0.872610629504505,104.));
#30629=CARTESIAN_POINT('',(-2.51749934288707,-0.00181894562271404,98.1125833025509));
#30630=CARTESIAN_POINT('Ctrl Pts',(-2.36143112101025,0.87261062950452,99.0561732563161));
#30631=CARTESIAN_POINT('Ctrl Pts',(-2.33278640704966,0.950128043012731,
99.050962759861));
#30632=CARTESIAN_POINT('Ctrl Pts',(-2.30030652899971,1.02627179950822,99.0457522634059));
#30633=CARTESIAN_POINT('Ctrl Pts',(-2.26415467450212,1.10064065885747,99.0405417669508));
#30634=CARTESIAN_POINT('Ctrl Pts',(-2.22800672982909,1.1750014752115,99.0353318340111));
#30635=CARTESIAN_POINT('Ctrl Pts',(-2.18818780234614,1.24758735633662,99.0301219010714));
#30636=CARTESIAN_POINT('Ctrl Pts',(-2.14490811357667,1.3180195121139,99.0249119681317));
#30637=CARTESIAN_POINT('Ctrl Pts',(-2.09943389879839,1.39202297817794,99.0194378620045));
#30638=CARTESIAN_POINT('Ctrl Pts',(-2.05013895512243,1.46364803471633,99.0139637558772));
#30639=CARTESIAN_POINT('Ctrl Pts',(-1.99731898245969,1.53248919484158,99.0084896497499));
#30640=CARTESIAN_POINT('Ctrl Pts',(-1.94698099158007,1.59809554629982,99.0032727688918));
#30641=CARTESIAN_POINT('Ctrl Pts',(-1.89344213718278,1.66117339722202,98.9980558880337));
#30642=CARTESIAN_POINT('Ctrl Pts',(-1.83699876145007,1.72140692470749,98.9928390071756));
#30643=CARTESIAN_POINT('Ctrl Pts',(-1.78051668615308,1.78168175041863,98.9876185494404));
#30644=CARTESIAN_POINT('Ctrl Pts',(-1.72112646326178,1.83910804989151,98.9823980917053));
#30645=CARTESIAN_POINT('Ctrl Pts',(-1.65915940431223,1.89340865136987,98.9771776339701));
#30646=CARTESIAN_POINT('Ctrl Pts',(-1.5970964362197,1.94779329627775,98.9719490963029));
#30647=CARTESIAN_POINT('Ctrl Pts',(-1.53244904350619,1.99904230777826,98.9667205586356));
#30648=CARTESIAN_POINT('Ctrl Pts',(-1.46557888184648,2.04692080723354,98.9614920209684));
#30649=CARTESIAN_POINT('Ctrl Pts',(-1.45590439728475,2.05384766059119,98.960735578847));
#30650=CARTESIAN_POINT('Ctrl Pts',(-1.44618343088935,2.06070404354763,98.9599791367257));
#30651=CARTESIAN_POINT('Ctrl Pts',(-1.43641711982849,2.06748932472785,98.9592226946043));
#30652=CARTESIAN_POINT('Ctrl Pts',(-1.36856738097082,2.11462887960022,98.9539674451989));
#30653=CARTESIAN_POINT('Ctrl Pts',(-1.29826938246395,2.15851196666169,98.9487121957935));
#30654=CARTESIAN_POINT('Ctrl Pts',(-1.22586870214749,2.19887520680352,98.943456946388));
#30655=CARTESIAN_POINT('Ctrl Pts',(-1.15357066954887,2.23918122103992,98.9382091477325));
#30656=CARTESIAN_POINT('Ctrl Pts',(-1.07917627618452,2.27597707782582,98.9329613490769));
#30657=CARTESIAN_POINT('Ctrl Pts',(-1.00306088599235,2.30904203274697,98.9277135504213));
#30658=CARTESIAN_POINT('Ctrl Pts',(-0.926393974143907,2.34234657178713,
98.922427726938));
#30659=CARTESIAN_POINT('Ctrl Pts',(-0.847981409199212,2.37186564323599,
98.9171419034546));
#30660=CARTESIAN_POINT('Ctrl Pts',(-0.768233009155977,2.39742034145937,
98.9118560799712));
#30661=CARTESIAN_POINT('Ctrl Pts',(-0.689199707548472,2.42274589245578,
98.9066176541046));
#30662=CARTESIAN_POINT('Ctrl Pts',(-0.608854879083993,2.44417773859863,
98.901379228238));
#30663=CARTESIAN_POINT('Ctrl Pts',(-0.527616746100529,2.46159030288029,
98.8961408023714));
#30664=CARTESIAN_POINT('Ctrl Pts',(-0.446405330987264,2.47899714045929,
98.8909040993359));
#30665=CARTESIAN_POINT('Ctrl Pts',(-0.364301645661412,2.49238722486515,
98.8856673963005));
#30666=CARTESIAN_POINT('Ctrl Pts',(-0.281736172190727,2.50168562758779,
98.880430693265));
#30667=CARTESIAN_POINT('Ctrl Pts',(-0.199172947762835,2.51098377702652,
98.8751941328747));
#30668=CARTESIAN_POINT('Ctrl Pts',(-0.116148418837698,2.51619041577051,
98.8699575724844));
#30669=CARTESIAN_POINT('Ctrl Pts',(-0.033098908478487,2.51728240613912,
98.8647210120941));
#30670=CARTESIAN_POINT('Ctrl Pts',(0.0513098985704013,2.51839226944745,
98.8593987433213));
#30671=CARTESIAN_POINT('Ctrl Pts',(0.135744020678939,2.51525155817116,98.8540764745485));
#30672=CARTESIAN_POINT('Ctrl Pts',(0.21974648244285,2.50789109282161,98.8487542057757));
#30673=CARTESIAN_POINT('Ctrl Pts',(0.302514886547704,2.50063875809643,98.8435101250274));
#30674=CARTESIAN_POINT('Ctrl Pts',(0.384863773673149,2.48928995356123,98.8382660442791));
#30675=CARTESIAN_POINT('Ctrl Pts',(0.466364092043617,2.47392618799598,98.8330219635309));
#30676=CARTESIAN_POINT('Ctrl Pts',(0.549687136607523,2.45821881717267,98.8276606007458));
#30677=CARTESIAN_POINT('Ctrl Pts',(0.632122700779561,2.43831485202597,98.8222992379607));
#30678=CARTESIAN_POINT('Ctrl Pts',(0.713228296358643,2.41435532746805,98.8169378751756));
#30679=CARTESIAN_POINT('Ctrl Pts',(0.794333891937714,2.39039580291013,98.8115765123905));
#30680=CARTESIAN_POINT('Ctrl Pts',(0.874109061651032,2.36238095031963,98.8062151496054));
#30681=CARTESIAN_POINT('Ctrl Pts',(0.952134552090648,2.3305033886942,98.8008537868203));
#30682=CARTESIAN_POINT('Ctrl Pts',(1.0286157435233,2.29925675532677,98.7955985373986));
#30683=CARTESIAN_POINT('Ctrl Pts',(1.10369839365188,2.26418355164877,98.790343287977));
#30684=CARTESIAN_POINT('Ctrl Pts',(1.17697343171605,2.22543024852152,98.7850880385553));
#30685=CARTESIAN_POINT('Ctrl Pts',(1.25014458242303,2.18673188877404,98.7798402398835));
#30686=CARTESIAN_POINT('Ctrl Pts',(1.32151280701535,2.14436400706664,98.7745924412116));
#30687=CARTESIAN_POINT('Ctrl Pts',(1.39068857929799,2.09852127113598,98.7693446425397));
#30688=CARTESIAN_POINT('Ctrl Pts',(1.46036558944912,2.05234636522027,98.7640588190604));
#30689=CARTESIAN_POINT('Ctrl Pts',(1.52781780214095,2.00264621522567,98.7587729955811));
#30690=CARTESIAN_POINT('Ctrl Pts',(1.59267202666219,1.94966716787449,98.7534871721018));
#30691=CARTESIAN_POINT('Ctrl Pts',(1.65694470804885,1.89716317980421,98.7482487462188));
#30692=CARTESIAN_POINT('Ctrl Pts',(1.7186654426701,1.84143915942296,98.7430103203358));
#30693=CARTESIAN_POINT('Ctrl Pts',(1.77750119569472,1.7827775378055,98.7377718944529));
#30694=CARTESIAN_POINT('Ctrl Pts',(1.83631759861892,1.72413520901953,98.732535191401));
#30695=CARTESIAN_POINT('Ctrl Pts',(1.89225057786082,1.66255752331376,98.7272984883492));
#30696=CARTESIAN_POINT('Ctrl Pts',(1.94500290732925,1.59836477078317,98.7220617852973));
#30697=CARTESIAN_POINT('Ctrl Pts',(1.99775379985013,1.53417376683165,98.7168252248907));
#30698=CARTESIAN_POINT('Ctrl Pts',(2.04732392269868,1.46736819483014,98.7115886644841));
#30699=CARTESIAN_POINT('Ctrl Pts',(2.09345631139287,1.39830144185341,98.7063521040775));
#30700=CARTESIAN_POINT('Ctrl Pts',(2.14034376265922,1.32810425272046,98.701029835324));
#30701=CARTESIAN_POINT('Ctrl Pts',(2.18367964760589,1.25557159756422,98.6957075665706));
#30702=CARTESIAN_POINT('Ctrl Pts',(2.22324101727091,1.18110356409767,98.6903852978171));
#30703=CARTESIAN_POINT('Ctrl Pts',(2.26222120171519,1.10772952006664,98.6851412170528));
#30704=CARTESIAN_POINT('Ctrl Pts',(2.29753689219085,1.03247703424813,98.6798971362884));
#30705=CARTESIAN_POINT('Ctrl Pts',(2.32902285972319,0.955750369545749,98.6746530555241));
#30706=CARTESIAN_POINT('Ctrl Pts',(2.36121299961584,0.877307740532357,98.6692916927761));
#30707=CARTESIAN_POINT('Ctrl Pts',(2.38939987853756,0.7973246809162,98.6639303300281));
#30708=CARTESIAN_POINT('Ctrl Pts',(2.41346088209449,0.716249133053366,98.6585689672801));
#30709=CARTESIAN_POINT('Ctrl Pts',(2.43752188565141,0.635173585190543,98.6532076045321));
#30710=CARTESIAN_POINT('Ctrl Pts',(2.45745695895928,0.553006058612372,98.6478462417841));
#30711=CARTESIAN_POINT('Ctrl Pts',(2.47319940617432,0.470203091545531,98.6424848790361));
#30712=CARTESIAN_POINT('Ctrl Pts',(2.48863027513713,0.389038980458705,98.6372296296523));
#30713=CARTESIAN_POINT('Ctrl Pts',(2.50009000850579,0.306964572849086,98.6319743802685));
#30714=CARTESIAN_POINT('Ctrl Pts',(2.50747874569295,0.224402740397944,98.6267191308847));
#30715=CARTESIAN_POINT('Ctrl Pts',(2.51485700732933,0.141957961869083,98.6214713322506));
#30716=CARTESIAN_POINT('Ctrl Pts',(2.5181756963732,0.0590275868908074,98.6162235336166));
#30717=CARTESIAN_POINT('Ctrl Pts',(2.51738602047343,-0.023955665821825,
98.6109757349825));
#30718=CARTESIAN_POINT('Ctrl Pts',(2.51659062268654,-0.107540204206683,
98.6056899114938));
#30719=CARTESIAN_POINT('Ctrl Pts',(2.51162698289234,-0.191177924300599,
98.600404088005));
#30720=CARTESIAN_POINT('Ctrl Pts',(2.50249855055409,-0.274421672749577,
98.5951182645162));
#30721=CARTESIAN_POINT('Ctrl Pts',(2.49345197228857,-0.356918979795724,
98.5898798386708));
#30722=CARTESIAN_POINT('Ctrl Pts',(2.48031504441379,-0.439028885213252,
98.5846414128253));
#30723=CARTESIAN_POINT('Ctrl Pts',(2.46314334660122,-0.520318271920331,
98.5794029869799));
#30724=CARTESIAN_POINT('Ctrl Pts',(2.44597729627376,-0.601580923903414,
98.5741662839654));
#30725=CARTESIAN_POINT('Ctrl Pts',(2.42477920673235,-0.682023142020918,
98.5689295809509));
#30726=CARTESIAN_POINT('Ctrl Pts',(2.39965590962701,-0.76122123288318,98.5636928779364));
#30727=CARTESIAN_POINT('Ctrl Pts',(2.37453329686682,-0.840417166431858,
98.5584563175669));
#30728=CARTESIAN_POINT('Ctrl Pts',(2.34548582963169,-0.91836860059621,98.5532197571974));
#30729=CARTESIAN_POINT('Ctrl Pts',(2.31267002155887,-0.994667593411446,
98.5479831968278));
#30730=CARTESIAN_POINT('Ctrl Pts',(2.2793171068472,-1.07221539580916,98.5426609280298));
#30731=CARTESIAN_POINT('Ctrl Pts',(2.24207156535357,-1.14805571987408,98.5373386592318));
#30732=CARTESIAN_POINT('Ctrl Pts',(2.20114760266341,-1.22178372934375,98.5320163904338));
#30733=CARTESIAN_POINT('Ctrl Pts',(2.16082484328938,-1.29442861975869,98.5267723097056));
#30734=CARTESIAN_POINT('Ctrl Pts',(2.11693132202151,-1.36502248149198,98.5215282289774));
#30735=CARTESIAN_POINT('Ctrl Pts',(2.06971617229043,-1.43320662019105,98.5162841482492));
#30736=CARTESIAN_POINT('Ctrl Pts',(2.02144507158909,-1.50291567425786,98.5109227854163));
#30737=CARTESIAN_POINT('Ctrl Pts',(1.96970228778801,-1.57010551367019,98.5055614225834));
#30738=CARTESIAN_POINT('Ctrl Pts',(1.91479679390173,-1.63442940748863,98.5002000597505));
#30739=CARTESIAN_POINT('Ctrl Pts',(1.85989130001545,-1.69875330130708,98.4948386969176));
#30740=CARTESIAN_POINT('Ctrl Pts',(1.80182349355314,-1.76021092607999,98.4894773340847));
#30741=CARTESIAN_POINT('Ctrl Pts',(1.74094000262391,-1.8184977748856,98.4841159712518));
#30742=CARTESIAN_POINT('Ctrl Pts',(1.6812615329398,-1.87563099583494,98.47886072185));
#30743=CARTESIAN_POINT('Ctrl Pts',(1.6186574225678,-1.92992887123232,98.4736054724482));
#30744=CARTESIAN_POINT('Ctrl Pts',(1.55342800376033,-1.98107740563896,98.4683502230463));
#30745=CARTESIAN_POINT('Ctrl Pts',(1.48829106545379,-2.03215342304069,98.4631024243945));
#30746=CARTESIAN_POINT('Ctrl Pts',(1.42053657194417,-2.08008868599946,98.4578546257428));
#30747=CARTESIAN_POINT('Ctrl Pts',(1.35050091928083,-2.12460667348609,98.452606827091));
#30748=CARTESIAN_POINT('Ctrl Pts',(1.27995779784039,-2.16944723223193,98.4473210036067));
#30749=CARTESIAN_POINT('Ctrl Pts',(1.2071006621332,-2.21082045661513,98.4420351801224));
#30750=CARTESIAN_POINT('Ctrl Pts',(1.13230645900514,-2.2484857866785,98.4367493566381));
#30751=CARTESIAN_POINT('Ctrl Pts',(1.05818293044283,-2.28581337427217,98.4315109307758));
#30752=CARTESIAN_POINT('Ctrl Pts',(0.982157354137152,-2.3194990867312,98.4262725049135));
#30753=CARTESIAN_POINT('Ctrl Pts',(0.904623285795088,-2.34935373258207,
98.4210340790513));
#30754=CARTESIAN_POINT('Ctrl Pts',(0.827114717120905,-2.37919855973556,
98.4157973760203));
#30755=CARTESIAN_POINT('Ctrl Pts',(0.748099071990192,-2.40521465698546,
98.4105606729893));
#30756=CARTESIAN_POINT('Ctrl Pts',(0.667989905809573,-2.42726095336627,
98.4053239699583));
#30757=CARTESIAN_POINT('Ctrl Pts',(0.587882921765202,-2.44930664921626,
98.4000874095727));
#30758=CARTESIAN_POINT('Ctrl Pts',(0.506682921049927,-2.46738263775978,
98.3948508491871));
#30759=CARTESIAN_POINT('Ctrl Pts',(0.42481729633244,-2.48139809678673,98.3896142888014));
#30760=CARTESIAN_POINT('Ctrl Pts',(0.341611751791082,-2.49564295113626,
98.3842920200236));
#30761=CARTESIAN_POINT('Ctrl Pts',(0.257719080177702,-2.50569306096329,
98.3789697512458));
#30762=CARTESIAN_POINT('Ctrl Pts',(0.173595479584124,-2.51150768652377,
98.373647482468));
#30763=CARTESIAN_POINT('Ctrl Pts',(0.0907077164253666,-2.51723689096714,
98.3684034017248));
#30764=CARTESIAN_POINT('Ctrl Pts',(0.00759623340742896,-2.51885428209207,
98.3631593209815));
#30765=CARTESIAN_POINT('Ctrl Pts',(-0.075302458326526,-2.51637353939553,
98.3579152402383));
#30766=CARTESIAN_POINT('Ctrl Pts',(-0.160055150626523,-2.51383731574667,
98.3525538774432));
#30767=CARTESIAN_POINT('Ctrl Pts',(-0.244584908401927,-2.50701748080513,
98.3471925146481));
#30768=CARTESIAN_POINT('Ctrl Pts',(-0.328432675586283,-2.49598442054578,
98.341831151853));
#30769=CARTESIAN_POINT('Ctrl Pts',(-0.412280442770639,-2.48495136028642,
98.3364697890579));
#30770=CARTESIAN_POINT('Ctrl Pts',(-0.495445731630717,-2.4697052320331,
98.3311084262627));
#30771=CARTESIAN_POINT('Ctrl Pts',(-0.57748440190406,-2.45037099549385,
98.3257470634676));
#30772=CARTESIAN_POINT('Ctrl Pts',(-0.657899344579412,-2.43141942646188,
98.3204918139567));
#30773=CARTESIAN_POINT('Ctrl Pts',(-0.737528890838629,-2.40847014411869,
98.3152365644458));
#30774=CARTESIAN_POINT('Ctrl Pts',(-0.81594614735313,-2.38160410954877,
98.3099813149348));
#30775=CARTESIAN_POINT('Ctrl Pts',(-0.894252226019699,-2.35477616491005,
98.3047335161734));
#30776=CARTESIAN_POINT('Ctrl Pts',(-0.97134899601205,-2.32404264635472,
98.2994857174119));
#30777=CARTESIAN_POINT('Ctrl Pts',(-1.04682136225834,-2.28953516800236,
98.2942379186504));
#30778=CARTESIAN_POINT('Ctrl Pts',(-1.12284058898346,-2.25477765407972,
98.2889520951935));
#30779=CARTESIAN_POINT('Ctrl Pts',(-1.19721131105349,-2.21619136730165,
98.2836662717365));
#30780=CARTESIAN_POINT('Ctrl Pts',(-1.2695265193546,-2.1739615145295,98.2783804482796));
#30781=CARTESIAN_POINT('Ctrl Pts',(-1.34119328395092,-2.13211033289482,
98.2731420223069));
#30782=CARTESIAN_POINT('Ctrl Pts',(-1.41084084453737,-2.0866809035605,98.2679035963341));
#30783=CARTESIAN_POINT('Ctrl Pts',(-1.47809623673638,-2.03790033243673,
98.2626651703614));
#30784=CARTESIAN_POINT('Ctrl Pts',(-1.54532950975434,-1.98913580443232,
98.25742846722));
#30785=CARTESIAN_POINT('Ctrl Pts',(-1.61017180367999,-1.93702259423835,
98.2521917640785));
#30786=CARTESIAN_POINT('Ctrl Pts',(-1.67227962837945,-1.88183078264415,
98.2469550609371));
#30787=CARTESIAN_POINT('Ctrl Pts',(-1.73438576128929,-1.82664047445043,
98.2417185004411));
#30788=CARTESIAN_POINT('Ctrl Pts',(-1.79375722884276,-1.76837203886615,
98.2364819399451));
#30789=CARTESIAN_POINT('Ctrl Pts',(-1.85008515545565,-1.70733452128241,
98.2312453794491));
#30790=CARTESIAN_POINT('Ctrl Pts',(-1.90733501593176,-1.64529798673193,
98.225923110802));
#30791=CARTESIAN_POINT('Ctrl Pts',(-1.96144046461852,-1.58040126026179,
98.2206008421549));
#30792=CARTESIAN_POINT('Ctrl Pts',(-2.01211895159742,-1.51300481645714,
98.2152785735077));
#30793=CARTESIAN_POINT('Ctrl Pts',(-2.06205293667055,-1.44659847286751,
98.2100344926556));
#30794=CARTESIAN_POINT('Ctrl Pts',(-2.10865976894878,-1.37776579151508,
98.2047904118035));
#30795=CARTESIAN_POINT('Ctrl Pts',(-2.15171326350379,-1.30688036241344,
98.1995463309513));
#30796=CARTESIAN_POINT('Ctrl Pts',(-2.1957296316017,-1.23440961010017,98.1941849684067));
#30797=CARTESIAN_POINT('Ctrl Pts',(-2.23603156289674,-1.15979363489705,
98.1888236058621));
#30798=CARTESIAN_POINT('Ctrl Pts',(-2.27242816283364,-1.08345581117115,
98.1834622433175));
#30799=CARTESIAN_POINT('Ctrl Pts',(-2.30882476277054,-1.00711798744524,
98.1781008807728));
#30800=CARTESIAN_POINT('Ctrl Pts',(-2.34131589776423,-0.929058809958435,
98.1727395182282));
#30801=CARTESIAN_POINT('Ctrl Pts',(-2.36976457020348,-0.849718854567983,
98.1673781556836));
#30802=CARTESIAN_POINT('Ctrl Pts',(-2.40208841952505,-0.759571492904689,
98.1612864874196));
#30803=CARTESIAN_POINT('Ctrl Pts',(-2.42929323988043,-0.667497660029118,
98.1551948191556));
#30804=CARTESIAN_POINT('Ctrl Pts',(-2.45117917966575,-0.574044318126351,
98.1491031508916));
#30805=CARTESIAN_POINT('Ctrl Pts',(-2.47304705906853,-0.48066809436979,
98.1430165095015));
#30806=CARTESIAN_POINT('Ctrl Pts',(-2.48960468697981,-0.385914765713439,
98.1369298681114));
#30807=CARTESIAN_POINT('Ctrl Pts',(-2.50070035454831,-0.290351488306736,
98.1308432267212));
#30808=CARTESIAN_POINT('Ctrl Pts',(-2.51179602211682,-0.194788210900033,
98.1247565853311));
#30809=CARTESIAN_POINT('Ctrl Pts',(-2.51742955013952,-0.0984151241393797,
98.118669943941));
#30810=CARTESIAN_POINT('Ctrl Pts',(-2.51749934288707,-0.00181894562268696,
98.1125833025509));
#30811=CARTESIAN_POINT('Ctrl Pts',(-2.51749934288774,-0.00181894468837515,
98.112583302492));
#30812=CARTESIAN_POINT('Ctrl Pts',(-2.51755948791397,0.0814244133741985,
98.107338038379));
#30813=CARTESIAN_POINT('Ctrl Pts',(-2.51348653839861,0.164706576949697,
98.102092774266));
#30814=CARTESIAN_POINT('Ctrl Pts',(-2.50529558036044,0.247588984057089,
98.096847510153));
#30815=CARTESIAN_POINT('Ctrl Pts',(-2.49710604242185,0.330457021505943,
98.0916031554326));
#30816=CARTESIAN_POINT('Ctrl Pts',(-2.48479996557399,0.412924984202785,
98.0863588007123));
#30817=CARTESIAN_POINT('Ctrl Pts',(-2.4684443260827,0.494559257349544,98.081114445992));
#30818=CARTESIAN_POINT('Ctrl Pts',(-2.45208034729026,0.576235153618919,
98.0758674173161));
#30819=CARTESIAN_POINT('Ctrl Pts',(-2.43166277620762,0.657076061900327,
98.0706203886402));
#30820=CARTESIAN_POINT('Ctrl Pts',(-2.40730958369761,0.736659228027211,
98.0653733599643));
#30821=CARTESIAN_POINT('Ctrl Pts',(-2.39330701863621,0.782417847190807,
98.0623564306486));
#30822=CARTESIAN_POINT('Ctrl Pts',(-2.37800426835301,0.827760905486719,
98.0593395013329));
#30823=CARTESIAN_POINT('Ctrl Pts',(-2.36143112101026,0.872610629504505,
98.0563225720173));
#30824=CARTESIAN_POINT('',(-2.51749969980483,0.00122942367908718,98.3894800759037));
#30825=CARTESIAN_POINT('Ctrl Pts',(-2.36143112099219,0.872610629553384,
98.3289997116198));
#30826=CARTESIAN_POINT('Ctrl Pts',(-2.36251252634525,0.86968416479508,98.3292070698479));
#30827=CARTESIAN_POINT('Ctrl Pts',(-2.36358849455286,0.866755681947571,
98.3294146496157));
#30828=CARTESIAN_POINT('Ctrl Pts',(-2.38569176180474,0.806249585917351,
98.3337050233089));
#30829=CARTESIAN_POINT('Ctrl Pts',(-2.4046133940344,0.747928505123625,98.3378683249366));
#30830=CARTESIAN_POINT('Ctrl Pts',(-2.48503075249899,0.465305249999661,
98.3580083728554));
#30831=CARTESIAN_POINT('Ctrl Pts',(-2.51738610202588,0.233844411718779,
98.3742563990415));
#30832=CARTESIAN_POINT('Ctrl Pts',(-2.51749969980483,0.00122942367908718,
98.3894800759037));
#30833=CARTESIAN_POINT('Ctrl Pts',(-2.51749970102175,0.00122692926385033,
98.3894802391527));
#30834=CARTESIAN_POINT('Ctrl Pts',(-2.51751699362345,-0.0342552463685801,
98.3918023979318));
#30835=CARTESIAN_POINT('Ctrl Pts',(-2.51678414767873,-0.0697355527763528,
98.3941023709484));
#30836=CARTESIAN_POINT('Ctrl Pts',(-2.51468428064402,-0.119947354296721,
98.3973271767744));
#30837=CARTESIAN_POINT('Ctrl Pts',(-2.51393727670791,-0.134698860759586,
98.3982709040074));
#30838=CARTESIAN_POINT('Ctrl Pts',(-2.51238467930962,-0.160807584097307,
98.3999348979899));
#30839=CARTESIAN_POINT('Ctrl Pts',(-2.51163178999321,-0.172167402147022,
98.4006567785607));
#30840=CARTESIAN_POINT('Ctrl Pts',(-2.50998576638091,-0.194687001615117,
98.4020837535092));
#30841=CARTESIAN_POINT('Ctrl Pts',(-2.50909519904191,-0.205846701982753,
98.4027889107625));
#30842=CARTESIAN_POINT('Ctrl Pts',(-2.50703690369869,-0.229636872795596,
98.4042880715654));
#30843=CARTESIAN_POINT('Ctrl Pts',(-2.50584809806961,-0.242265244382523,
98.4050813985938));
#30844=CARTESIAN_POINT('Ctrl Pts',(-2.5025086037242,-0.27508004554831,98.4071367631431));
#30845=CARTESIAN_POINT('Ctrl Pts',(-2.50020907757556,-0.295250654440163,
98.4083941422339));
#30846=CARTESIAN_POINT('Ctrl Pts',(-2.48960195094086,-0.37925114101235,
98.4136078207328));
#30847=CARTESIAN_POINT('Ctrl Pts',(-2.47909158077049,-0.44278128912095,
98.4174954056116));
#30848=CARTESIAN_POINT('Ctrl Pts',(-2.42391125053333,-0.711804189701246,
98.4338297233657));
#30849=CARTESIAN_POINT('Ctrl Pts',(-2.35603586036114,-0.911647589929297,
98.4455667959131));
#30850=CARTESIAN_POINT('Ctrl Pts',(-2.23948847655878,-1.15137727999021,
98.4611714800706));
#30851=CARTESIAN_POINT('Ctrl Pts',(-2.21317205832378,-1.20118563047322,
98.4645102083124));
#30852=CARTESIAN_POINT('Ctrl Pts',(-2.17405848863169,-1.26955907691938,
98.4692874520271));
#30853=CARTESIAN_POINT('Ctrl Pts',(-2.162647579165,-1.28890105826086,98.4706613819721));
#30854=CARTESIAN_POINT('Ctrl Pts',(-2.14220510259818,-1.32251606415087,
98.4730935572093));
#30855=CARTESIAN_POINT('Ctrl Pts',(-2.13328564759608,-1.33685592028066,
98.4741455453322));
#30856=CARTESIAN_POINT('Ctrl Pts',(-2.11980100133727,-1.35805664463297,
98.4757241647799));
#30857=CARTESIAN_POINT('Ctrl Pts',(-2.11534508855464,-1.36498691828661,
98.4762439509061));
#30858=CARTESIAN_POINT('Ctrl Pts',(-2.10764829526881,-1.3768295272819,98.4771388537794));
#30859=CARTESIAN_POINT('Ctrl Pts',(-2.10442409021737,-1.38175255789982,
98.4775128710844));
#30860=CARTESIAN_POINT('Ctrl Pts',(-2.09703725211919,-1.3929456746197,98.4783678683661));
#30861=CARTESIAN_POINT('Ctrl Pts',(-2.09286382753363,-1.39920830654091,
98.4788495506993));
#30862=CARTESIAN_POINT('Ctrl Pts',(-2.0813546906116,-1.41631220020541,98.4801739478363));
#30863=CARTESIAN_POINT('Ctrl Pts',(-2.07396252345917,-1.42711493246564,
98.4810202591172));
#30864=CARTESIAN_POINT('Ctrl Pts',(-2.0351665779363,-1.48287233928722,98.4854376591868));
#30865=CARTESIAN_POINT('Ctrl Pts',(-2.00238659106204,-1.52684653211508,
98.4890887172663));
#30866=CARTESIAN_POINT('Ctrl Pts',(-1.95146611126933,-1.59069372807524,
98.4946041354914));
#30867=CARTESIAN_POINT('Ctrl Pts',(-1.93439815217987,-1.61140629071393,
98.4964288023875));
#30868=CARTESIAN_POINT('Ctrl Pts',(-1.82945276958812,-1.73469068796356,
98.5074885870588));
#30869=CARTESIAN_POINT('Ctrl Pts',(-1.73376798993656,-1.83032752193577,
98.5169002565777));
#30870=CARTESIAN_POINT('Ctrl Pts',(-1.56194742099078,-1.97643930116815,
98.532338102714));
#30871=CARTESIAN_POINT('Ctrl Pts',(-1.48990865438214,-2.03129687856708,
98.5384488730024));
#30872=CARTESIAN_POINT('Ctrl Pts',(-1.38436608735715,-2.10302510487333,
98.5468759228934));
#30873=CARTESIAN_POINT('Ctrl Pts',(-1.35320715832976,-2.12320858021311,
98.5493039478005));
#30874=CARTESIAN_POINT('Ctrl Pts',(-1.30438961140577,-2.15331916827592,
98.5530173911187));
#30875=CARTESIAN_POINT('Ctrl Pts',(-1.28703947715253,-2.16373406914773,
98.5543200160027));
#30876=CARTESIAN_POINT('Ctrl Pts',(-1.25790319702832,-2.18074945458449,
98.5564794816089));
#30877=CARTESIAN_POINT('Ctrl Pts',(-1.24618636264018,-2.18746615926823,
98.5573404502793));
#30878=CARTESIAN_POINT('Ctrl Pts',(-1.22326125242602,-2.2003640534734,98.5590107797653));
#30879=CARTESIAN_POINT('Ctrl Pts',(-1.21205878877034,-2.20655468137506,
98.5598204589114));
#30880=CARTESIAN_POINT('Ctrl Pts',(-1.19109946262436,-2.21792929830086,
98.561323388808));
#30881=CARTESIAN_POINT('Ctrl Pts',(-1.18135479006627,-2.22313498653789,
98.562017393489));
#30882=CARTESIAN_POINT('Ctrl Pts',(-1.15884198390379,-2.23497169761749,
98.5636099864298));
#30883=CARTESIAN_POINT('Ctrl Pts',(-1.14605056677791,-2.24155779420834,
98.5645069851632));
#30884=CARTESIAN_POINT('Ctrl Pts',(-1.11334886549381,-2.25804227448824,
98.5667806794855));
#30885=CARTESIAN_POINT('Ctrl Pts',(-1.09336236924063,-2.2677873329584,98.5681520697682));
#30886=CARTESIAN_POINT('Ctrl Pts',(-0.927130462668619,-2.34613047095334,
98.5794152305849));
#30887=CARTESIAN_POINT('Ctrl Pts',(-0.774716962842792,-2.40077531994733,
98.5888014870537));
#30888=CARTESIAN_POINT('Ctrl Pts',(-0.498314926994687,-2.47078073313339,
98.6052044919033));
#30889=CARTESIAN_POINT('Ctrl Pts',(-0.376465446982886,-2.49225711870617,
98.6122472279382));
#30890=CARTESIAN_POINT('Ctrl Pts',(-0.209544896812296,-2.50915375730239,
98.6221647301031));
#30891=CARTESIAN_POINT('Ctrl Pts',(-0.165442618148325,-2.51244700340151,
98.6248111354426));
#30892=CARTESIAN_POINT('Ctrl Pts',(-0.0932156440727912,-2.51593054004382,
98.6292202654478));
#30893=CARTESIAN_POINT('Ctrl Pts',(-0.0651328580131158,-2.5168140966657,
98.6309531204751));
#30894=CARTESIAN_POINT('Ctrl Pts',(-0.026960124412928,-2.51737583188876,
98.6333408143243));
#30895=CARTESIAN_POINT('Ctrl Pts',(-0.0168771009210558,-2.51746362091817,
98.6339745602995));
#30896=CARTESIAN_POINT('Ctrl Pts',(-2.87216088621246E-6,-2.51750915987809,
98.635040669953));
#30897=CARTESIAN_POINT('Ctrl Pts',(0.00678825361368961,-2.51750000750709,
98.6354712274952));
#30898=CARTESIAN_POINT('Ctrl Pts',(0.0196863967509814,-2.5174304349512,
98.6362919498681));
#30899=CARTESIAN_POINT('Ctrl Pts',(0.0257933834337942,-2.51737526969945,
98.6366818083085));
#30900=CARTESIAN_POINT('Ctrl Pts',(0.0419340648825511,-2.51717072965315,
98.637715433853));
#30901=CARTESIAN_POINT('Ctrl Pts',(0.0519670494144753,-2.51698358471215,
98.6383612360471));
#30902=CARTESIAN_POINT('Ctrl Pts',(0.0876723555727046,-2.51610400377987,
98.6406706409705));
#30903=CARTESIAN_POINT('Ctrl Pts',(0.113333938011973,-2.51507874590665,
98.6423508974433));
#30904=CARTESIAN_POINT('Ctrl Pts',(0.310297827850211,-2.50418909695351,
98.6553826259731));
#30905=CARTESIAN_POINT('Ctrl Pts',(0.480193025962468,-2.47722750799108,
98.6673744499423));
#30906=CARTESIAN_POINT('Ctrl Pts',(0.796505995138727,-2.39324641363297,
98.6899025226779));
#30907=CARTESIAN_POINT('Ctrl Pts',(0.942987044736867,-2.33941031592157,
98.7004236803611));
#30908=CARTESIAN_POINT('Ctrl Pts',(1.1083308856421,-2.26056655500363,98.7122689446717));
#30909=CARTESIAN_POINT('Ctrl Pts',(1.13289370070507,-2.24835728070326,98.7140287624617));
#30910=CARTESIAN_POINT('Ctrl Pts',(1.16986600128615,-2.22921993154496,98.716678807802));
#30911=CARTESIAN_POINT('Ctrl Pts',(1.18242382800012,-2.22258450201499,98.7175791186557));
#30912=CARTESIAN_POINT('Ctrl Pts',(1.20513188855768,-2.21033885569095,98.7192077433897));
#30913=CARTESIAN_POINT('Ctrl Pts',(1.21530071682184,-2.20476413721329,98.7199372787107));
#30914=CARTESIAN_POINT('Ctrl Pts',(1.23717239769552,-2.19257642566458,98.7215070698305));
#30915=CARTESIAN_POINT('Ctrl Pts',(1.24886158098583,-2.18593954323024,98.7223464504472));
#30916=CARTESIAN_POINT('Ctrl Pts',(1.28054623452729,-2.16761252027556,98.7246232107151));
#30917=CARTESIAN_POINT('Ctrl Pts',(1.30043473743483,-2.15573937326398,98.7260540112355));
#30918=CARTESIAN_POINT('Ctrl Pts',(1.40829909415721,-2.0893098388904,98.7338280696146));
#30919=CARTESIAN_POINT('Ctrl Pts',(1.49301494487951,-2.02963838208085,98.7399803227214));
#30920=CARTESIAN_POINT('Ctrl Pts',(1.70345095965785,-1.86108686495952,98.7557145617346));
#30921=CARTESIAN_POINT('Ctrl Pts',(1.82247939099285,-1.74469330797658,98.7650668714782));
#30922=CARTESIAN_POINT('Ctrl Pts',(1.96492130134873,-1.57479712484879,98.7780521717106));
#30923=CARTESIAN_POINT('Ctrl Pts',(1.99924124099459,-1.53099163609463,98.7813520089986));
#30924=CARTESIAN_POINT('Ctrl Pts',(2.04522878744721,-1.46810818330624,98.7860780605237));
#30925=CARTESIAN_POINT('Ctrl Pts',(2.05813818263662,-1.44995502741673,98.7874411795667));
#30926=CARTESIAN_POINT('Ctrl Pts',(2.08034765104763,-1.41782986132642,98.7898559206268));
#30927=CARTESIAN_POINT('Ctrl Pts',(2.08975221065323,-1.40393145412892,98.7909014088085));
#30928=CARTESIAN_POINT('Ctrl Pts',(2.10355427283277,-1.38308828804054,98.7924721369203));
#30929=CARTESIAN_POINT('Ctrl Pts',(2.10805806111619,-1.37621400869465,98.7929906310838));
#30930=CARTESIAN_POINT('Ctrl Pts',(2.11572780997627,-1.36438143183146,98.793884104961));
#30931=CARTESIAN_POINT('Ctrl Pts',(2.11891016971707,-1.35943390757987,98.7942579955972));
#30932=CARTESIAN_POINT('Ctrl Pts',(2.12613225931577,-1.3481189588307,98.795113823292));
#30933=CARTESIAN_POINT('Ctrl Pts',(2.13016066271556,-1.34174463246024,98.7955964709219));
#30934=CARTESIAN_POINT('Ctrl Pts',(2.14113780895645,-1.32420095658078,98.7969260292657));
#30935=CARTESIAN_POINT('Ctrl Pts',(2.14802762637555,-1.31299527380286,98.7977765812414));
#30936=CARTESIAN_POINT('Ctrl Pts',(2.18366325818061,-1.25400583669762,98.8022589023628));
#30937=CARTESIAN_POINT('Ctrl Pts',(2.21090124289708,-1.20533419886879,98.8059733849085));
#30938=CARTESIAN_POINT('Ctrl Pts',(2.33440870036381,-0.966345106520117,
98.8241512694426));
#30939=CARTESIAN_POINT('Ctrl Pts',(2.40785316135883,-0.765209203929734,
98.8391750234135));
#30940=CARTESIAN_POINT('Ctrl Pts',(2.46790762697627,-0.500605938009424,
98.8574141232757));
#30941=CARTESIAN_POINT('Ctrl Pts',(2.47879254550975,-0.443579430810109,
98.8612661773974));
#30942=CARTESIAN_POINT('Ctrl Pts',(2.49390609296479,-0.346231944753901,
98.8677051805415));
#30943=CARTESIAN_POINT('Ctrl Pts',(2.4991500068134,-0.306094288218767,98.8703212997873));
#30944=CARTESIAN_POINT('Ctrl Pts',(2.50517238454175,-0.249382565083663,
98.8739652399694));
#30945=CARTESIAN_POINT('Ctrl Pts',(2.50675824026645,-0.232902310541583,
98.8750179675019));
#30946=CARTESIAN_POINT('Ctrl Pts',(2.50920534040131,-0.204540182300264,
98.8768193674926));
#30947=CARTESIAN_POINT('Ctrl Pts',(2.51014502032862,-0.192665802059044,
98.8775704576663));
#30948=CARTESIAN_POINT('Ctrl Pts',(2.51178056805739,-0.169948982264116,
98.8790015967649));
#30949=CARTESIAN_POINT('Ctrl Pts',(2.51249059156029,-0.159107862402842,
98.8796820696292));
#30950=CARTESIAN_POINT('Ctrl Pts',(2.51399123933149,-0.133671036346462,
98.881272975351));
#30951=CARTESIAN_POINT('Ctrl Pts',(2.5147249762436,-0.119072269529612,98.8821816282468));
#30952=CARTESIAN_POINT('Ctrl Pts',(2.51651852755542,-0.0758878556344527,
98.8848570935973));
#30953=CARTESIAN_POINT('Ctrl Pts',(2.51721836844828,-0.0472890303797434,
98.8866128267951));
#30954=CARTESIAN_POINT('Ctrl Pts',(2.51888958382193,0.177890982017307,98.9003251482861));
#30955=CARTESIAN_POINT('Ctrl Pts',(2.497321116647,0.373959927687693,98.9115238248948));
#30956=CARTESIAN_POINT('Ctrl Pts',(2.42226595916285,0.699529847463623,98.930750766372));
#30957=CARTESIAN_POINT('Ctrl Pts',(2.38045389933403,0.830748659818356,98.9387105772089));
#30958=CARTESIAN_POINT('Ctrl Pts',(2.32179454098603,0.973321748433057,98.948243862286));
#30959=CARTESIAN_POINT('Ctrl Pts',(2.31528735363616,0.988700941661192,98.9492843270587));
#30960=CARTESIAN_POINT('Ctrl Pts',(2.30535672658936,1.01153541133451,98.9508489540232));
#30961=CARTESIAN_POINT('Ctrl Pts',(2.30204891225037,1.01904088551106,98.9513664468257));
#30962=CARTESIAN_POINT('Ctrl Pts',(2.29630646334231,1.03189992925071,98.9522588160658));
#30963=CARTESIAN_POINT('Ctrl Pts',(2.2938896599225,1.03726132899413,98.9526326114611));
#30964=CARTESIAN_POINT('Ctrl Pts',(2.28832631590083,1.0494884269284,98.9534890970397));
#30965=CARTESIAN_POINT('Ctrl Pts',(2.28516771340179,1.05634833476745,98.9539725042462));
#30966=CARTESIAN_POINT('Ctrl Pts',(2.27640145300119,1.07516373420176,98.9553061277819));
#30967=CARTESIAN_POINT('Ctrl Pts',(2.27073061108246,1.08708928088393,98.9561600208168));
#30968=CARTESIAN_POINT('Ctrl Pts',(2.24029753181949,1.14981159478994,98.9606946003531));
#30969=CARTESIAN_POINT('Ctrl Pts',(2.21392576400893,1.19980472671081,98.9644602448049));
#30970=CARTESIAN_POINT('Ctrl Pts',(2.09744788662719,1.40367692515224,98.9803326742536));
#30971=CARTESIAN_POINT('Ctrl Pts',(1.99280345357862,1.54865568462149,98.9928370597096));
#30972=CARTESIAN_POINT('Ctrl Pts',(1.8211376922936,1.73996021357985,99.010336023566));
#30973=CARTESIAN_POINT('Ctrl Pts',(1.76583564903728,1.79605969141301,99.015622626624));
#30974=CARTESIAN_POINT('Ctrl Pts',(1.68308597709842,1.87247885525332,99.0230366522767));
#30975=CARTESIAN_POINT('Ctrl Pts',(1.65771833506833,1.89497376499894,99.0252483089887));
#30976=CARTESIAN_POINT('Ctrl Pts',(1.61150845941753,1.93431231005251,99.0291702459706));
#30977=CARTESIAN_POINT('Ctrl Pts',(1.59083746903626,1.95134821730251,99.0308880534518));
#30978=CARTESIAN_POINT('Ctrl Pts',(1.55889778375257,1.97682623079763,99.0334881386531));
#30979=CARTESIAN_POINT('Ctrl Pts',(1.54782414292937,1.98550867099786,99.0343799301567));
#30980=CARTESIAN_POINT('Ctrl Pts',(1.52838868740956,2.00048588854729,99.0359285845265));
#30981=CARTESIAN_POINT('Ctrl Pts',(1.52005942234716,2.00682214656534,99.0365870652251));
#30982=CARTESIAN_POINT('Ctrl Pts',(1.50118464189965,2.02099568069085,99.0380676724236));
#30983=CARTESIAN_POINT('Ctrl Pts',(1.49061674424518,2.02880275103887,99.0388886146387));
#30984=CARTESIAN_POINT('Ctrl Pts',(1.46187875495682,2.04968726858238,99.0410998056959));
#30985=CARTESIAN_POINT('Ctrl Pts',(1.44359429530408,2.06260586480312,99.042483973662));
#30986=CARTESIAN_POINT('Ctrl Pts',(1.35365026743666,2.12437239083864,99.0491872593423));
#30987=CARTESIAN_POINT('Ctrl Pts',(1.27966762159844,2.16974196526879,99.0543759556894));
#30988=CARTESIAN_POINT('Ctrl Pts',(1.04654538881708,2.29662247419423,99.0699767135842));
#30989=CARTESIAN_POINT('Ctrl Pts',(0.880967243998219,2.3650847480179,99.0800184088173));
#30990=CARTESIAN_POINT('Ctrl Pts',(0.624982175647708,2.44028085453877,99.0956015921277));
#30991=CARTESIAN_POINT('Ctrl Pts',(0.539186741567531,2.46065998944262,99.100842112574));
#30992=CARTESIAN_POINT('Ctrl Pts',(0.438442990266717,2.47906806768612,99.1071980010465));
#30993=CARTESIAN_POINT('Ctrl Pts',(0.424354630710516,2.48151845956877,99.1080913909655));
#30994=CARTESIAN_POINT('Ctrl Pts',(0.402639616267851,2.48510503466635,99.1094764810659));
#30995=CARTESIAN_POINT('Ctrl Pts',(0.395027076194549,2.48632646674423,99.1099635680923));
#30996=CARTESIAN_POINT('Ctrl Pts',(0.380970151714646,2.48851571424831,99.1108660033671));
#30997=CARTESIAN_POINT('Ctrl Pts',(0.374527501603449,2.48949349546782,99.1112807919467));
#30998=CARTESIAN_POINT('Ctrl Pts',(0.359833889308503,2.49166517109962,99.1122294573842));
#30999=CARTESIAN_POINT('Ctrl Pts',(0.351580783123815,2.49284309593926,99.1127641989881));
#31000=CARTESIAN_POINT('Ctrl Pts',(0.329970364214883,2.49581799344352,99.114169085439));
#31001=CARTESIAN_POINT('Ctrl Pts',(0.316604403689426,2.4975487043405,99.1150426808899));
#31002=CARTESIAN_POINT('Ctrl Pts',(0.215821389323318,2.50977674799173,99.121661819589));
#31003=CARTESIAN_POINT('Ctrl Pts',(0.1279298592638,2.51578792258693,99.1276135051862));
#31004=CARTESIAN_POINT('Ctrl Pts',(-0.00828600142811408,2.51794786567276,
99.1369474368046));
#31005=CARTESIAN_POINT('Ctrl Pts',(-0.0564975498331805,2.51732754540024,
99.1402726909946));
#31006=CARTESIAN_POINT('Ctrl Pts',(-0.227141696781966,2.51022718001341,
99.1520691875792));
#31007=CARTESIAN_POINT('Ctrl Pts',(-0.349095860765041,2.49619110546966,
99.1605386739852));
#31008=CARTESIAN_POINT('Ctrl Pts',(-0.56195856385726,2.45578017283049,99.1751458661343));
#31009=CARTESIAN_POINT('Ctrl Pts',(-0.653321333576555,2.43306978720321,
99.1813588140841));
#31010=CARTESIAN_POINT('Ctrl Pts',(-0.764296576239692,2.39877972270679,
99.1888300983966));
#31011=CARTESIAN_POINT('Ctrl Pts',(-0.785298568465696,2.39198654334872,
99.1902408465567));
#31012=CARTESIAN_POINT('Ctrl Pts',(-0.818590861470113,2.3807322570265,99.1924726533573));
#31013=CARTESIAN_POINT('Ctrl Pts',(-0.830940059036212,2.37645023236023,
99.1932995094898));
#31014=CARTESIAN_POINT('Ctrl Pts',(-0.854222109443938,2.36817362158646,
99.1948566996009));
#31015=CARTESIAN_POINT('Ctrl Pts',(-0.865161655149543,2.36419902546531,
99.195587666996));
#31016=CARTESIAN_POINT('Ctrl Pts',(-0.889889440708315,2.35502021590934,
99.1972385291194));
#31017=CARTESIAN_POINT('Ctrl Pts',(-0.903660415365992,2.34977047864266,
99.1981568915802));
#31018=CARTESIAN_POINT('Ctrl Pts',(-0.945434112719405,2.33342405666579,
99.2009402451735));
#31019=CARTESIAN_POINT('Ctrl Pts',(-0.973285116314992,2.32194523850266,
99.2027925150356));
#31020=CARTESIAN_POINT('Ctrl Pts',(-1.19530910431112,2.22574082244616,99.2175478919344));
#31021=CARTESIAN_POINT('Ctrl Pts',(-1.37828220071341,2.11731727543549,99.2295483855258));
#31022=CARTESIAN_POINT('Ctrl Pts',(-1.64278533664376,1.91160762569995,99.2488711704504));
#31023=CARTESIAN_POINT('Ctrl Pts',(-1.73434933352431,1.82893741228284,99.2560474614189));
#31024=CARTESIAN_POINT('Ctrl Pts',(-1.83173235238424,1.72710074748358,99.2647478964081));
#31025=CARTESIAN_POINT('Ctrl Pts',(-1.84384609874572,1.71416216439873,99.2658510502251));
#31026=CARTESIAN_POINT('Ctrl Pts',(-1.8614987313224,1.69490392265879,99.2674916646551));
#31027=CARTESIAN_POINT('Ctrl Pts',(-1.86714450740241,1.68868239093063,99.268021473472));
#31028=CARTESIAN_POINT('Ctrl Pts',(-1.87711721794238,1.67758151214792,99.26896668032));
#31029=CARTESIAN_POINT('Ctrl Pts',(-1.88145647247008,1.67271346038088,99.2693811523807));
#31030=CARTESIAN_POINT('Ctrl Pts',(-1.89085309742834,1.6620889041754,99.2702857399228));
#31031=CARTESIAN_POINT('Ctrl Pts',(-1.89590304035709,1.65632624180449,99.2707763564439));
#31032=CARTESIAN_POINT('Ctrl Pts',(-1.90990248676862,1.6402030896841,99.2721487480768));
#31033=CARTESIAN_POINT('Ctrl Pts',(-1.91879374491143,1.6297926951168,99.2730345454454));
#31034=CARTESIAN_POINT('Ctrl Pts',(-1.96895578313804,1.57008066906743,99.2781108995259));
#31035=CARTESIAN_POINT('Ctrl Pts',(-2.00840742653807,1.51928874754185,99.282411487989));
#31036=CARTESIAN_POINT('Ctrl Pts',(-2.06229364670572,1.44414183428322,99.2886878372842));
#31037=CARTESIAN_POINT('Ctrl Pts',(-2.07833276406017,1.4209621988587,99.2906126766852));
#31038=CARTESIAN_POINT('Ctrl Pts',(-2.17748209749237,1.27240131684512,99.3028590059017));
#31039=CARTESIAN_POINT('Ctrl Pts',(-2.2496092496616,1.14004211783502,99.3133447890744));
#31040=CARTESIAN_POINT('Ctrl Pts',(-2.32799801044045,0.959371796268697,
99.3267118840795));
#31041=CARTESIAN_POINT('Ctrl Pts',(-2.34531855308029,0.916213942992361,
99.3298409628682));
#31042=CARTESIAN_POINT('Ctrl Pts',(-2.36143108732087,0.87261072067364,99.3329358985331));
#31043=CARTESIAN_POINT('Origin',(0.,0.,104.));
#31044=CARTESIAN_POINT('',(-2.36143107613328,0.872610750949147,100.332008666168));
#31045=CARTESIAN_POINT('',(-2.36143112101026,0.8726106295045,100.056192078358));
#31046=CARTESIAN_POINT('',(-2.36143112101026,0.872610629504505,104.));
#31047=CARTESIAN_POINT('',(-2.51749995409241,-0.000480775099579418,99.1125833024489));
#31048=CARTESIAN_POINT('Ctrl Pts',(-2.36143112101026,0.8726106295045,100.056192078358));
#31049=CARTESIAN_POINT('Ctrl Pts',(-2.33275321512777,0.950217865935678,
100.050942487041));
#31050=CARTESIAN_POINT('Ctrl Pts',(-2.30020045113898,1.0265317094225,100.045692895725));
#31051=CARTESIAN_POINT('Ctrl Pts',(-2.26391198059064,1.10113977048245,100.040443304408));
#31052=CARTESIAN_POINT('Ctrl Pts',(-2.22617849102928,1.17871874944353,100.034984672612));
#31053=CARTESIAN_POINT('Ctrl Pts',(-2.18440565730927,1.25445275645764,100.029526040816));
#31054=CARTESIAN_POINT('Ctrl Pts',(-2.13880631067855,1.32789826997462,100.02406740902));
#31055=CARTESIAN_POINT('Ctrl Pts',(-2.09504128200363,1.39838930203143,100.018828360773));
#31056=CARTESIAN_POINT('Ctrl Pts',(-2.04775194893672,1.46677198470564,100.013589312525));
#31057=CARTESIAN_POINT('Ctrl Pts',(-1.99717363357701,1.53267861188991,100.008350264277));
#31058=CARTESIAN_POINT('Ctrl Pts',(-1.94661547449549,1.59855897421539,100.003113303875));
#31059=CARTESIAN_POINT('Ctrl Pts',(-1.89277121654677,1.66196487490729,99.9978763434726));
#31060=CARTESIAN_POINT('Ctrl Pts',(-1.83591852413709,1.7225589751095,99.9926393830704));
#31061=CARTESIAN_POINT('Ctrl Pts',(-1.77907133909669,1.78314720550904,99.987402929977));
#31062=CARTESIAN_POINT('Ctrl Pts',(-1.71921661485095,1.84092384063048,99.9821664768837));
#31063=CARTESIAN_POINT('Ctrl Pts',(-1.65667024491431,1.89558696704096,99.9769300237903));
#31064=CARTESIAN_POINT('Ctrl Pts',(-1.59411106748309,1.95026128671008,99.971692498439));
#31065=CARTESIAN_POINT('Ctrl Pts',(-1.52885949824838,2.00182052920588,99.9664549730876));
#31066=CARTESIAN_POINT('Ctrl Pts',(-1.46126493165182,2.05000269500423,99.9612174477363));
#31067=CARTESIAN_POINT('Ctrl Pts',(-1.39359507066367,2.09823853149006,99.9559740882432));
#31068=CARTESIAN_POINT('Ctrl Pts',(-1.32357738102401,2.14308951729394,99.95073072875));
#31069=CARTESIAN_POINT('Ctrl Pts',(-1.25159019006132,2.1843370266839,99.9454873692569));
#31070=CARTESIAN_POINT('Ctrl Pts',(-1.17955552358119,2.22561173878625,99.9402405517708));
#31071=CARTESIAN_POINT('Ctrl Pts',(-1.10554918158347,2.26327803598502,99.9349937342846));
#31072=CARTESIAN_POINT('Ctrl Pts',(-1.02997188865551,2.29716437343508,99.9297469167985));
#31073=CARTESIAN_POINT('Ctrl Pts',(-0.954274422211247,2.33110459268176,
99.9244917564824));
#31074=CARTESIAN_POINT('Ctrl Pts',(-0.877001449681806,2.36125269283684,
99.9192365961662));
#31075=CARTESIAN_POINT('Ctrl Pts',(-0.798570787510214,2.38748632401011,
99.9139814358501));
#31076=CARTESIAN_POINT('Ctrl Pts',(-0.775958698366631,2.39504965689837,
99.9124663376698));
#31077=CARTESIAN_POINT('Ctrl Pts',(-0.753250453814723,2.40228793947742,
99.9109512394895));
#31078=CARTESIAN_POINT('Ctrl Pts',(-0.73045621841153,2.40919902934231,99.9094361413093));
#31079=CARTESIAN_POINT('Ctrl Pts',(-0.651392436504516,2.43317074377591,
99.904180891902));
#31080=CARTESIAN_POINT('Ctrl Pts',(-0.571001358178255,2.45329059604218,
99.8989256424948));
#31081=CARTESIAN_POINT('Ctrl Pts',(-0.489692843022924,2.46941433734643,
99.8936703930876));
#31082=CARTESIAN_POINT('Ctrl Pts',(-0.408499604871022,2.48551521884839,
99.8884225944301));
#31083=CARTESIAN_POINT('Ctrl Pts',(-0.326391962325043,2.49763115387418,
99.8831747957727));
#31084=CARTESIAN_POINT('Ctrl Pts',(-0.243794995103415,2.50566762567634,
99.8779269971153));
#31085=CARTESIAN_POINT('Ctrl Pts',(-0.16059954164588,2.51376232864511,99.8726411736324));
#31086=CARTESIAN_POINT('Ctrl Pts',(-0.0769080959350252,2.51771806298665,
99.8673553501494));
#31087=CARTESIAN_POINT('Ctrl Pts',(0.00683435582160804,2.51749072323624,
99.8620695266665));
#31088=CARTESIAN_POINT('Ctrl Pts',(0.0898258947923132,2.51726542202568,
99.856831100798));
#31089=CARTESIAN_POINT('Ctrl Pts',(0.172867058815803,2.5129317662099,99.8515926749295));
#31090=CARTESIAN_POINT('Ctrl Pts',(0.255521276622755,2.5044989772793,99.846354249061));
#31091=CARTESIAN_POINT('Ctrl Pts',(0.338148310833058,2.49606896175264,99.8411175460235));
#31092=CARTESIAN_POINT('Ctrl Pts',(0.420388192896793,2.48354253738092,99.8358808429861));
#31093=CARTESIAN_POINT('Ctrl Pts',(0.501808273409439,2.46698088900945,99.8306441399487));
#31094=CARTESIAN_POINT('Ctrl Pts',(0.583226136079772,2.450419691769,99.8254075795564));
#31095=CARTESIAN_POINT('Ctrl Pts',(0.663823789642993,2.4298235820575,99.8201710191642));
#31096=CARTESIAN_POINT('Ctrl Pts',(0.743178965335783,2.40530481966058,99.8149344587719));
#31097=CARTESIAN_POINT('Ctrl Pts',(0.823832971350214,2.38038475121435,99.8096121900014));
#31098=CARTESIAN_POINT('Ctrl Pts',(0.903202986832025,2.35141259769608,99.8042899212308));
#31099=CARTESIAN_POINT('Ctrl Pts',(0.980863698094443,2.31855831407375,99.7989676524603));
#31100=CARTESIAN_POINT('Ctrl Pts',(1.05738351671678,2.28618668390347,99.79372357171));
#31101=CARTESIAN_POINT('Ctrl Pts',(1.13224352481678,2.25004648789801,99.7884794909598));
#31102=CARTESIAN_POINT('Ctrl Pts',(1.2050605760744,2.21034731614541,99.7832354102096));
#31103=CARTESIAN_POINT('Ctrl Pts',(1.27950615519606,2.16976028631203,99.7778740474289));
#31104=CARTESIAN_POINT('Ctrl Pts',(1.35181585816839,2.12545343680915,99.7725126846481));
#31105=CARTESIAN_POINT('Ctrl Pts',(1.42161207296085,2.07769713000041,99.7671513218674));
#31106=CARTESIAN_POINT('Ctrl Pts',(1.49140828775331,2.02994082319168,99.7617899590867));
#31107=CARTESIAN_POINT('Ctrl Pts',(1.55869065048926,1.97873541994863,99.756428596306));
#31108=CARTESIAN_POINT('Ctrl Pts',(1.62311953089869,1.92439321304541,99.7510672335253));
#31109=CARTESIAN_POINT('Ctrl Pts',(1.68627321951298,1.87112656008526,99.7458119841178));
#31110=CARTESIAN_POINT('Ctrl Pts',(1.74691864446473,1.81464942875828,99.7405567347102));
#31111=CARTESIAN_POINT('Ctrl Pts',(1.80471166228413,1.75522706964531,99.7353014853027));
#31112=CARTESIAN_POINT('Ctrl Pts',(1.86242274273326,1.69588895793843,99.7300536866449));
#31113=CARTESIAN_POINT('Ctrl Pts',(1.91728912972066,1.63361424055039,99.7248058879872));
#31114=CARTESIAN_POINT('Ctrl Pts',(1.96900010801149,1.56870801127895,99.7195580893294));
#31115=CARTESIAN_POINT('Ctrl Pts',(2.02108577691702,1.5033314804246,99.7142722658466));
#31116=CARTESIAN_POINT('Ctrl Pts',(2.06996975462605,1.43528544716466,99.7089864423638));
#31117=CARTESIAN_POINT('Ctrl Pts',(2.11537277237975,1.36491914920789,99.7037006188809));
#31118=CARTESIAN_POINT('Ctrl Pts',(2.16036866440994,1.29518382098363,99.6984621930121));
#31119=CARTESIAN_POINT('Ctrl Pts',(2.20194551872949,1.22317006756963,99.6932237671432));
#31120=CARTESIAN_POINT('Ctrl Pts',(2.23987337834433,1.14924910223343,99.6879853412744));
#31121=CARTESIAN_POINT('Ctrl Pts',(2.27778876411735,1.07535244827252,99.6827486382366));
#31122=CARTESIAN_POINT('Ctrl Pts',(2.31205732816317,0.999550238354843,99.6775119351988));
#31123=CARTESIAN_POINT('Ctrl Pts',(2.34249483521434,0.922238687647695,99.6722752321611));
#31124=CARTESIAN_POINT('Ctrl Pts',(2.37293151316303,0.844929242868551,99.6670386717685));
#31125=CARTESIAN_POINT('Ctrl Pts',(2.39953717353041,0.766110968767055,99.6618021113759));
#31126=CARTESIAN_POINT('Ctrl Pts',(2.42217607407124,0.686199181139743,99.6565655509833));
#31127=CARTESIAN_POINT('Ctrl Pts',(2.44518551238695,0.604979452964636,99.6512432822131));
#31128=CARTESIAN_POINT('Ctrl Pts',(2.46409702235611,0.52263056209984,99.645921013443));
#31129=CARTESIAN_POINT('Ctrl Pts',(2.478821598194,0.43960179063209,99.6405987446728));
#31130=CARTESIAN_POINT('Ctrl Pts',(2.49332985924698,0.357792772523543,99.6353546639222));
#31131=CARTESIAN_POINT('Ctrl Pts',(2.50377338992084,0.275324189124085,99.6301105831716));
#31132=CARTESIAN_POINT('Ctrl Pts',(2.51011938815238,0.192631532261719,99.624866502421));
#31133=CARTESIAN_POINT('Ctrl Pts',(2.51660731241188,0.108089483089288,99.619505139641));
#31134=CARTESIAN_POINT('Ctrl Pts',(2.51881219952784,0.0233137287272409,
99.6141437768611));
#31135=CARTESIAN_POINT('Ctrl Pts',(2.51675523590554,-0.0612317935557103,
99.6087824140811));
#31136=CARTESIAN_POINT('Ctrl Pts',(2.51469827228324,-0.145777315838661,
99.6034210513011));
#31137=CARTESIAN_POINT('Ctrl Pts',(2.50837956250575,-0.230092104348521,
99.5980596885211));
#31138=CARTESIAN_POINT('Ctrl Pts',(2.49787614311196,-0.313721251546827,
99.5926983257411));
#31139=CARTESIAN_POINT('Ctrl Pts',(2.48758060990405,-0.395695190685063,
99.5874430763341));
#31140=CARTESIAN_POINT('Ctrl Pts',(2.47322652414446,-0.477313167572697,
99.5821878269271));
#31141=CARTESIAN_POINT('Ctrl Pts',(2.45484900652466,-0.558142101229502,
99.57693257752));
#31142=CARTESIAN_POINT('Ctrl Pts',(2.43649754404998,-0.638856437820514,
99.5716847788628));
#31143=CARTESIAN_POINT('Ctrl Pts',(2.41413408159011,-0.71878350702968,99.5664369802056));
#31144=CARTESIAN_POINT('Ctrl Pts',(2.38784536007417,-0.797496574520719,
99.5611891815484));
#31145=CARTESIAN_POINT('Ctrl Pts',(2.36136615410554,-0.876779986049647,
99.5559033580654));
#31146=CARTESIAN_POINT('Ctrl Pts',(2.33090462434359,-0.954831258455381,
99.5506175345824));
#31147=CARTESIAN_POINT('Ctrl Pts',(2.29660166037244,-1.03122600024173,99.5453317110994));
#31148=CARTESIAN_POINT('Ctrl Pts',(2.26260628871365,-1.10693571564675,99.5400932852311));
#31149=CARTESIAN_POINT('Ctrl Pts',(2.22483829116516,-1.18101806074897,99.5348548593628));
#31150=CARTESIAN_POINT('Ctrl Pts',(2.18348383810752,-1.2530780417529,99.5296164334945));
#31151=CARTESIAN_POINT('Ctrl Pts',(2.14214298584121,-1.32511432342837,99.5243797304572));
#31152=CARTESIAN_POINT('Ctrl Pts',(2.09721825015777,-1.39512916208937,99.51914302742));
#31153=CARTESIAN_POINT('Ctrl Pts',(2.0489416661038,-1.4627523026486,99.5139063243828));
#31154=CARTESIAN_POINT('Ctrl Pts',(2.00066639707982,-1.53037360118732,99.5086697639907));
#31155=CARTESIAN_POINT('Ctrl Pts',(1.94903973015863,-1.59560295621481,99.5034332035986));
#31156=CARTESIAN_POINT('Ctrl Pts',(1.89433612394891,-1.6581003888493,99.4981966432066));
#31157=CARTESIAN_POINT('Ctrl Pts',(1.83873716715634,-1.72162073599736,99.4928743744358));
#31158=CARTESIAN_POINT('Ctrl Pts',(1.77995995392479,-1.7823185468515,99.4875521056649));
#31159=CARTESIAN_POINT('Ctrl Pts',(1.71833287926423,-1.83987455171256,99.4822298368941));
#31160=CARTESIAN_POINT('Ctrl Pts',(1.65761115140187,-1.89658501676819,99.4769857561441));
#31161=CARTESIAN_POINT('Ctrl Pts',(1.59412313646232,-1.95024511869322,99.471741675394));
#31162=CARTESIAN_POINT('Ctrl Pts',(1.52821626249666,-2.00059023916462,99.4664975946439));
#31163=CARTESIAN_POINT('Ctrl Pts',(1.46083540435537,-2.05206131063975,99.4611362318628));
#31164=CARTESIAN_POINT('Ctrl Pts',(1.39092660984415,-2.10006704475547,99.4557748690816));
#31165=CARTESIAN_POINT('Ctrl Pts',(1.31889056093659,-2.14437262113476,99.4504135063004));
#31166=CARTESIAN_POINT('Ctrl Pts',(1.24685451202902,-2.18867819751406,99.4450521435193));
#31167=CARTESIAN_POINT('Ctrl Pts',(1.17269168648258,-2.22928343073232,99.4396907807381));
#31168=CARTESIAN_POINT('Ctrl Pts',(1.0968255998952,-2.26600526332455,99.4343294179569));
#31169=CARTESIAN_POINT('Ctrl Pts',(1.02246107303578,-2.30200028862464,99.42907416855));
#31170=CARTESIAN_POINT('Ctrl Pts',(0.946185439293675,-2.33439722715269,
99.4238189191431));
#31171=CARTESIAN_POINT('Ctrl Pts',(0.868381085169217,-2.36298974625798,
99.4185636697362));
#31172=CARTESIAN_POINT('Ctrl Pts',(0.790687039943935,-2.3915417276666,99.4133158710791));
#31173=CARTESIAN_POINT('Ctrl Pts',(0.711469008870073,-2.41629984548479,
99.408068072422));
#31174=CARTESIAN_POINT('Ctrl Pts',(0.631132159650954,-2.43710452115914,
99.4028202737649));
#31175=CARTESIAN_POINT('Ctrl Pts',(0.550213200693043,-2.45805994464649,
99.3975344502819));
#31176=CARTESIAN_POINT('Ctrl Pts',(0.468159568119976,-2.4750041855899,99.3922486267989));
#31177=CARTESIAN_POINT('Ctrl Pts',(0.385403945798672,-2.48782436047298,
99.3869628033159));
#31178=CARTESIAN_POINT('Ctrl Pts',(0.303390387438331,-2.50052957773159,
99.3817243774477));
#31179=CARTESIAN_POINT('Ctrl Pts',(0.220687842678183,-2.50918432119756,
99.3764859515795));
#31180=CARTESIAN_POINT('Ctrl Pts',(0.137728990020848,-2.51372969416122,
99.3712475257113));
#31181=CARTESIAN_POINT('Ctrl Pts',(0.0547974211495223,-2.51827357222735,
99.3660108226742));
#31182=CARTESIAN_POINT('Ctrl Pts',(-0.0283898278374614,-2.51871073872765,
99.3607741196371));
#31183=CARTESIAN_POINT('Ctrl Pts',(-0.111395857986024,-2.51503423690883,
99.3555374166));
#31184=CARTESIAN_POINT('Ctrl Pts',(-0.194399627091786,-2.51135783523607,
99.3503008562081));
#31185=CARTESIAN_POINT('Ctrl Pts',(-0.277221726250651,-2.50356800948417,
99.3450642958162));
#31186=CARTESIAN_POINT('Ctrl Pts',(-0.359427554381548,-2.49170987138377,
99.3398277354243));
#31187=CARTESIAN_POINT('Ctrl Pts',(-0.442978870342003,-2.47965764752499,
99.3345054666533));
#31188=CARTESIAN_POINT('Ctrl Pts',(-0.525893071314123,-2.46340279239329,
99.3291831978823));
#31189=CARTESIAN_POINT('Ctrl Pts',(-0.607723561161488,-2.44304693430339,
99.3238609291114));
#31190=CARTESIAN_POINT('Ctrl Pts',(-0.688351901260997,-2.42299011865741,
99.3186168483614));
#31191=CARTESIAN_POINT('Ctrl Pts',(-0.76792772961714,-2.39895218778448,
99.3133727676115));
#31192=CARTESIAN_POINT('Ctrl Pts',(-0.846039928677307,-2.37108048979441,
99.3081286868616));
#31193=CARTESIAN_POINT('Ctrl Pts',(-0.925899079745084,-2.34258545102857,
99.3027673240801));
#31194=CARTESIAN_POINT('Ctrl Pts',(-1.00422787147293,-2.31008329040283,
99.2974059612987));
#31195=CARTESIAN_POINT('Ctrl Pts',(-1.08061118641412,-2.27378224854463,
99.2920445985172));
#31196=CARTESIAN_POINT('Ctrl Pts',(-1.15699450135531,-2.23748120668643,
99.2866832357357));
#31197=CARTESIAN_POINT('Ctrl Pts',(-1.23143192386132,-2.19738158338034,
99.2813218729542));
#31198=CARTESIAN_POINT('Ctrl Pts',(-1.30353932301423,-2.15373895432005,
99.2759605101728));
#31199=CARTESIAN_POINT('Ctrl Pts',(-1.374219555307,-2.11096011059407,99.2707052607635));
#31200=CARTESIAN_POINT('Ctrl Pts',(-1.44292224529696,-2.06461926119626,
99.2654500113543));
#31201=CARTESIAN_POINT('Ctrl Pts',(-1.50926613182133,-2.01492481083962,
99.260194761945));
#31202=CARTESIAN_POINT('Ctrl Pts',(-1.57551595778619,-1.96530081592432,
99.2549469632856));
#31203=CARTESIAN_POINT('Ctrl Pts',(-1.63941325671187,-1.91233293847999,
99.2496991646262));
#31204=CARTESIAN_POINT('Ctrl Pts',(-1.70060358115018,-1.85627414725821,
99.2444513659668));
#31205=CARTESIAN_POINT('Ctrl Pts',(-1.76223728221295,-1.79980916179165,
99.2391655424843));
#31206=CARTESIAN_POINT('Ctrl Pts',(-1.82112420912457,-1.7402085262543,99.2338797190019));
#31207=CARTESIAN_POINT('Ctrl Pts',(-1.87693410065596,-1.67777371292877,
99.2285938955195));
#31208=CARTESIAN_POINT('Ctrl Pts',(-1.93224354876778,-1.61589874823624,
99.223355469649));
#31209=CARTESIAN_POINT('Ctrl Pts',(-1.98453061042904,-1.55124058028577,
99.2181170437784));
#31210=CARTESIAN_POINT('Ctrl Pts',(-2.03351031104773,-1.48413007006211,
99.2128786179079));
#31211=CARTESIAN_POINT('Ctrl Pts',(-2.08247390305797,-1.41704163136847,
99.2076419148685));
#31212=CARTESIAN_POINT('Ctrl Pts',(-2.12813202252442,-1.34750282464206,
99.2024052118291));
#31213=CARTESIAN_POINT('Ctrl Pts',(-2.17024096385839,-1.27587632974007,
99.1971685087896));
#31214=CARTESIAN_POINT('Ctrl Pts',(-2.21234875816577,-1.20425178590814,
99.1919319483954));
#31215=CARTESIAN_POINT('Ctrl Pts',(-2.25090733360058,-1.13054006526377,
99.1866953880011));
#31216=CARTESIAN_POINT('Ctrl Pts',(-2.28571791029733,-1.05513026899337,
99.1814588276069));
#31217=CARTESIAN_POINT('Ctrl Pts',(-2.32109824227236,-0.978486217690824,
99.1761365588387));
#31218=CARTESIAN_POINT('Ctrl Pts',(-2.35260656131234,-0.900088444370652,
99.1708142900705));
#31219=CARTESIAN_POINT('Ctrl Pts',(-2.38008496250032,-0.820366882120347,
99.1654920213023));
#31220=CARTESIAN_POINT('Ctrl Pts',(-2.40715968590261,-0.741816487853945,
99.1602479405501));
#31221=CARTESIAN_POINT('Ctrl Pts',(-2.43032203890123,-0.661981407916923,
99.1550038597979));
#31222=CARTESIAN_POINT('Ctrl Pts',(-2.44947178236045,-0.581286708449395,
99.1497597790457));
#31223=CARTESIAN_POINT('Ctrl Pts',(-2.46904980310552,-0.498787300373405,
99.1443984162695));
#31224=CARTESIAN_POINT('Ctrl Pts',(-2.48443347442554,-0.415389862155177,
99.1390370534934));
#31225=CARTESIAN_POINT('Ctrl Pts',(-2.49557145561039,-0.331555968039523,
99.1336756907172));
#31226=CARTESIAN_POINT('Ctrl Pts',(-2.50670943679524,-0.247722073923868,
99.128314327941));
#31227=CARTESIAN_POINT('Ctrl Pts',(-2.5136017530014,-0.163452235771735,
99.1229529651648));
#31228=CARTESIAN_POINT('Ctrl Pts',(-2.51625363847077,-0.079207808217358,
99.1175916023886));
#31229=CARTESIAN_POINT('Ctrl Pts',(-2.51707938858173,-0.0529755873299053,
99.1159221690898));
#31230=CARTESIAN_POINT('Ctrl Pts',(-2.51749494111227,-0.0267303864513461,
99.1142527357909));
#31231=CARTESIAN_POINT('Ctrl Pts',(-2.51749995409228,-0.00048077577683593,
99.112583302492));
#31232=CARTESIAN_POINT('Ctrl Pts',(-2.51749995409241,-0.000480775099579418,
99.1125833024489));
#31233=CARTESIAN_POINT('Ctrl Pts',(-2.51751564872535,0.0817015960768791,
99.1073566349482));
#31234=CARTESIAN_POINT('Ctrl Pts',(-2.51350287458033,0.16404280022504,99.1021299674474));
#31235=CARTESIAN_POINT('Ctrl Pts',(-2.50544101952395,0.246112875906163,
99.0969032999467));
#31236=CARTESIAN_POINT('Ctrl Pts',(-2.49738907342895,0.328082077879528,
99.0916830566307));
#31237=CARTESIAN_POINT('Ctrl Pts',(-2.48529796461774,0.409780352380315,
99.0864628133147));
#31238=CARTESIAN_POINT('Ctrl Pts',(-2.46919906308424,0.490777176388562,
99.0812425699987));
#31239=CARTESIAN_POINT('Ctrl Pts',(-2.45311733396175,0.571687602529829,
99.0760278950232));
#31240=CARTESIAN_POINT('Ctrl Pts',(-2.43303639485911,0.651897609163979,
99.0708132200476));
#31241=CARTESIAN_POINT('Ctrl Pts',(-2.40903928512245,0.730982881288401,
99.065598545072));
#31242=CARTESIAN_POINT('Ctrl Pts',(-2.39458138892031,0.77863056336517,99.0624567821534));
#31243=CARTESIAN_POINT('Ctrl Pts',(-2.37870296850341,0.825870105370799,
99.0593150192347));
#31244=CARTESIAN_POINT('Ctrl Pts',(-2.36143112101025,0.87261062950452,99.0561732563161));
#31245=CARTESIAN_POINT('Ctrl Pts',(-2.36143108732087,0.87261072067364,99.3329358985331));
#31246=CARTESIAN_POINT('Ctrl Pts',(-2.38350361458074,0.812878756795239,
99.3371756444856));
#31247=CARTESIAN_POINT('Ctrl Pts',(-2.40330917650767,0.752310976484073,
99.3413508841152));
#31248=CARTESIAN_POINT('Ctrl Pts',(-2.42710975634389,0.668934068856912,
99.3469335538277));
#31249=CARTESIAN_POINT('Ctrl Pts',(-2.43311614183059,0.646746051710752,
99.3484037148847));
#31250=CARTESIAN_POINT('Ctrl Pts',(-2.44210925342362,0.611624633902569,
99.3507071482415));
#31251=CARTESIAN_POINT('Ctrl Pts',(-2.44529890896816,0.598744983451393,
99.3515468762135));
#31252=CARTESIAN_POINT('Ctrl Pts',(-2.45108873153855,0.574547742247975,
99.3531153651944));
#31253=CARTESIAN_POINT('Ctrl Pts',(-2.45371269678936,0.563236262040109,
99.353844867736));
#31254=CARTESIAN_POINT('Ctrl Pts',(-2.45942266551899,0.537824079487287,
99.3554756174414));
#31255=CARTESIAN_POINT('Ctrl Pts',(-2.4624658658942,0.52371410250307,99.3563754841404));
#31256=CARTESIAN_POINT('Ctrl Pts',(-2.4699195078865,0.487652697582533,99.3586615322447));
#31257=CARTESIAN_POINT('Ctrl Pts',(-2.47415882993385,0.465666900772979,
99.3600423065247));
#31258=CARTESIAN_POINT('Ctrl Pts',(-2.50444437449513,0.296491547298753,
99.3705741160288));
#31259=CARTESIAN_POINT('Ctrl Pts',(-2.51763009975741,0.147294862717954,
99.3792994844789));
#31260=CARTESIAN_POINT('Ctrl Pts',(-2.51736624855715,-0.153667235191149,
99.3966409705038));
#31261=CARTESIAN_POINT('Ctrl Pts',(-2.50356545338128,-0.304793761042445,
99.4052239540686));
#31262=CARTESIAN_POINT('Ctrl Pts',(-2.4671480155389,-0.503536313841017,
99.4172876465437));
#31263=CARTESIAN_POINT('Ctrl Pts',(-2.45652651072161,-0.553032434548504,
99.4203597266038));
#31264=CARTESIAN_POINT('Ctrl Pts',(-2.4413360492093,-0.614695809172208,
99.4243102694106));
#31265=CARTESIAN_POINT('Ctrl Pts',(-2.43815446225405,-0.627196496088505,
99.4251175746218));
#31266=CARTESIAN_POINT('Ctrl Pts',(-2.43299484213032,-0.646836316304257,
99.4263968732795));
#31267=CARTESIAN_POINT('Ctrl Pts',(-2.43108107133862,-0.653992311233613,
99.4268652974623));
#31268=CARTESIAN_POINT('Ctrl Pts',(-2.42741138985683,-0.667475324425731,
99.4277524005593));
#31269=CARTESIAN_POINT('Ctrl Pts',(-2.42566228055569,-0.673804022803481,
99.4281706932355));
#31270=CARTESIAN_POINT('Ctrl Pts',(-2.4215080367134,-0.688609261340399,
99.4291536319278));
#31271=CARTESIAN_POINT('Ctrl Pts',(-2.41908313957884,-0.697080085015698,
99.4297193901709));
#31272=CARTESIAN_POINT('Ctrl Pts',(-2.41102350834638,-0.724685998092114,
99.4315737818691));
#31273=CARTESIAN_POINT('Ctrl Pts',(-2.40520596708076,-0.743766328134072,
99.4328721769997));
#31274=CARTESIAN_POINT('Ctrl Pts',(-2.37190210432902,-0.848517271839642,
99.4400851232568));
#31275=CARTESIAN_POINT('Ctrl Pts',(-2.34006731138586,-0.932728779619282,
99.4461958166118));
#31276=CARTESIAN_POINT('Ctrl Pts',(-2.30124781520773,-1.02083532040833,
99.4528094388848));
#31277=CARTESIAN_POINT('Ctrl Pts',(-2.29867571243539,-1.02661396197294,
99.4532442590251));
#31278=CARTESIAN_POINT('Ctrl Pts',(-2.27569957632008,-1.0777142786758,99.4570984021582));
#31279=CARTESIAN_POINT('Ctrl Pts',(-2.25397947675746,-1.12243176106848,
99.4605340104382));
#31280=CARTESIAN_POINT('Ctrl Pts',(-2.1468152438127,-1.32738921994537,99.4765107392243));
#31281=CARTESIAN_POINT('Ctrl Pts',(-2.04550368744715,-1.47875439981819,
99.4889251030126));
#31282=CARTESIAN_POINT('Ctrl Pts',(-1.90801155467121,-1.64266287107209,
99.5028235107663));
#31283=CARTESIAN_POINT('Ctrl Pts',(-1.88677973864446,-1.66700683165984,
99.5049028408222));
#31284=CARTESIAN_POINT('Ctrl Pts',(-1.85486588270896,-1.70220746786093,
99.5079333864175));
#31285=CARTESIAN_POINT('Ctrl Pts',(-1.84454512048291,-1.71338583557381,
99.5088994479938));
#31286=CARTESIAN_POINT('Ctrl Pts',(-1.82608709798173,-1.73301754220954,
99.5106028960883));
#31287=CARTESIAN_POINT('Ctrl Pts',(-1.81799096578936,-1.74150875589474,
99.5113419935818));
#31288=CARTESIAN_POINT('Ctrl Pts',(-1.80101437973741,-1.75906637213317,
99.5128752722766));
#31289=CARTESIAN_POINT('Ctrl Pts',(-1.79212411715161,-1.76812286216456,
99.5136690001466));
#31290=CARTESIAN_POINT('Ctrl Pts',(-1.76881427923021,-1.79151210525207,
99.5157266333546));
#31291=CARTESIAN_POINT('Ctrl Pts',(-1.75428871311169,-1.80573827734058,
99.5169858606241));
#31292=CARTESIAN_POINT('Ctrl Pts',(-1.6878884445282,-1.86921238954983,99.5226421387201));
#31293=CARTESIAN_POINT('Ctrl Pts',(-1.63409894406825,-1.91641446185513,
99.526952186908));
#31294=CARTESIAN_POINT('Ctrl Pts',(-1.39527342814532,-2.1086141768126,99.5451237231192));
#31295=CARTESIAN_POINT('Ctrl Pts',(-1.19247242616962,-2.22958136458589,
99.5580984578959));
#31296=CARTESIAN_POINT('Ctrl Pts',(-0.926826816288691,-2.34128764152677,
99.5752705816891));
#31297=CARTESIAN_POINT('Ctrl Pts',(-0.877155130666692,-2.36034610883845,
99.578493960378));
#31298=CARTESIAN_POINT('Ctrl Pts',(-0.814670057285158,-2.3820762356174,
99.5826076995543));
#31299=CARTESIAN_POINT('Ctrl Pts',(-0.802386401142647,-2.38624192844866,
99.5834191881031));
#31300=CARTESIAN_POINT('Ctrl Pts',(-0.782951577521749,-2.39266573248303,
99.584708299063));
#31301=CARTESIAN_POINT('Ctrl Pts',(-0.775821375847051,-2.39498719609388,
99.5851823433075));
#31302=CARTESIAN_POINT('Ctrl Pts',(-0.76307277731967,-2.39907500355149,
99.5860320564837));
#31303=CARTESIAN_POINT('Ctrl Pts',(-0.757458421221817,-2.40085353025583,
99.5864070109938));
#31304=CARTESIAN_POINT('Ctrl Pts',(-0.743936881683051,-2.40508476048013,
99.5873118180892));
#31305=CARTESIAN_POINT('Ctrl Pts',(-0.736023846607228,-2.40751815810598,
99.5878427666852));
#31306=CARTESIAN_POINT('Ctrl Pts',(-0.711739695433816,-2.41485505052959,
99.5894762824282));
#31307=CARTESIAN_POINT('Ctrl Pts',(-0.695330919672426,-2.41963079490134,
99.5905857371124));
#31308=CARTESIAN_POINT('Ctrl Pts',(-0.656916164928314,-2.43038832742408,
99.5931943085517));
#31309=CARTESIAN_POINT('Ctrl Pts',(-0.634875258379955,-2.43623882220654,
99.5946995337551));
#31310=CARTESIAN_POINT('Ctrl Pts',(-0.556854527964823,-2.45581786387308,
99.6000506865114));
#31311=CARTESIAN_POINT('Ctrl Pts',(-0.500488343834589,-2.46792198666117,
99.6039576994706));
#31312=CARTESIAN_POINT('Ctrl Pts',(-0.278042158974925,-2.50775636219712,
99.6194213700015));
#31313=CARTESIAN_POINT('Ctrl Pts',(-0.109748558572827,-2.52073636635111,
99.6311818878833));
#31314=CARTESIAN_POINT('Ctrl Pts',(0.15725323059623,-2.51452163981783,99.6492346988049));
#31315=CARTESIAN_POINT('Ctrl Pts',(0.255713856971508,-2.5064242014543,99.655769548375));
#31316=CARTESIAN_POINT('Ctrl Pts',(0.37612500224252,-2.48934940422941,99.6636012876936));
#31317=CARTESIAN_POINT('Ctrl Pts',(0.39874982503602,-2.48582563894636,99.6650660771872));
#31318=CARTESIAN_POINT('Ctrl Pts',(0.434516683811463,-2.4797541334284,99.6673716073837));
#31319=CARTESIAN_POINT('Ctrl Pts',(0.447691451196276,-2.47740947090541,
99.6682186718712));
#31320=CARTESIAN_POINT('Ctrl Pts',(0.472251899395199,-2.47283622032223,
99.6697938993378));
#31321=CARTESIAN_POINT('Ctrl Pts',(0.483642026420423,-2.47063377021909,
99.6705228640406));
#31322=CARTESIAN_POINT('Ctrl Pts',(0.509017696476248,-2.46554479723182,
99.6721435992095));
#31323=CARTESIAN_POINT('Ctrl Pts',(0.522994793607886,-2.46261783913498,
99.6730340664564));
#31324=CARTESIAN_POINT('Ctrl Pts',(0.564114795353025,-2.45364097696741,
99.6756476877903));
#31325=CARTESIAN_POINT('Ctrl Pts',(0.591183774112016,-2.44725997501708,
99.6773603358368));
#31326=CARTESIAN_POINT('Ctrl Pts',(0.652613089805557,-2.43170040762843,
99.6812326616919));
#31327=CARTESIAN_POINT('Ctrl Pts',(0.686896127418619,-2.42223958458449,
99.6833834357499));
#31328=CARTESIAN_POINT('Ctrl Pts',(0.802091440564606,-2.38780745940144,
99.6905898518851));
#31329=CARTESIAN_POINT('Ctrl Pts',(0.881943642260125,-2.35948133346607,
99.6955486757934));
#31330=CARTESIAN_POINT('Ctrl Pts',(1.13990184797048,-2.25304499243265,99.7117117745281));
#31331=CARTESIAN_POINT('Ctrl Pts',(1.310369432877,-2.15835649099085,99.7225908748216));
#31332=CARTESIAN_POINT('Ctrl Pts',(1.49666661801921,-2.02460387426945,99.736468233969));
#31333=CARTESIAN_POINT('Ctrl Pts',(1.52467384326875,-2.00359706627596,99.7386149116104));
#31334=CARTESIAN_POINT('Ctrl Pts',(1.56116154476958,-1.97502139580867,99.741506091522));
#31335=CARTESIAN_POINT('Ctrl Pts',(1.57004320118683,-1.96796829695185,99.7422174640866));
#31336=CARTESIAN_POINT('Ctrl Pts',(1.58437854132509,-1.95642551189073,99.7433786294224));
#31337=CARTESIAN_POINT('Ctrl Pts',(1.58986163259488,-1.95197236969748,99.7438258811177));
#31338=CARTESIAN_POINT('Ctrl Pts',(1.60051022876152,-1.94324938484815,99.7447007422064));
#31339=CARTESIAN_POINT('Ctrl Pts',(1.60567752318345,-1.93898191112802,99.7451281882358));
#31340=CARTESIAN_POINT('Ctrl Pts',(1.6182307175091,-1.92853011218795,99.7461736144245));
#31341=CARTESIAN_POINT('Ctrl Pts',(1.62559823757108,-1.9223239611282,99.7467931366474));
#31342=CARTESIAN_POINT('Ctrl Pts',(1.65193150097515,-1.89988206665984,99.7490283888691));
#31343=CARTESIAN_POINT('Ctrl Pts',(1.67069041255477,-1.88340728073437,99.7506600381524));
#31344=CARTESIAN_POINT('Ctrl Pts',(1.71708108420924,-1.8414268103847,99.7547882251664));
#31345=CARTESIAN_POINT('Ctrl Pts',(1.74439164039583,-1.81557639863167,99.7573039218401));
#31346=CARTESIAN_POINT('Ctrl Pts',(1.94085087424065,-1.62109522841749,99.77597832516));
#31347=CARTESIAN_POINT('Ctrl Pts',(2.08582754727152,-1.42975713546375,99.7928462800587));
#31348=CARTESIAN_POINT('Ctrl Pts',(2.23329401056134,-1.16381007579665,99.8130598913627));
#31349=CARTESIAN_POINT('Ctrl Pts',(2.26268275595813,-1.10558764396749,99.8173233836058));
#31350=CARTESIAN_POINT('Ctrl Pts',(2.29825613872131,-1.02773580990944,99.8228189056339));
#31351=CARTESIAN_POINT('Ctrl Pts',(2.30650655545125,-1.0090836059402,99.8241206163115));
#31352=CARTESIAN_POINT('Ctrl Pts',(2.31952722985832,-0.978652686080276,
99.8262207283625));
#31353=CARTESIAN_POINT('Ctrl Pts',(2.32443644003715,-0.96693479400513,99.8270237938747));
#31354=CARTESIAN_POINT('Ctrl Pts',(2.33370639022585,-0.944329533064323,
99.8285624282832));
#31355=CARTESIAN_POINT('Ctrl Pts',(2.3380801552854,-0.933447897704011,99.829298418254));
#31356=CARTESIAN_POINT('Ctrl Pts',(2.3480374689279,-0.908165641413657,99.8309978196828));
#31357=CARTESIAN_POINT('Ctrl Pts',(2.35356489082611,-0.893743312777121,
99.8319593424349));
#31358=CARTESIAN_POINT('Ctrl Pts',(2.37080160048548,-0.847499654454535,
99.8350179471396));
#31359=CARTESIAN_POINT('Ctrl Pts',(2.3820012059711,-0.81549145619755,99.8370982505718));
#31360=CARTESIAN_POINT('Ctrl Pts',(2.4068356229774,-0.739632620068523,99.8419500028941));
#31361=CARTESIAN_POINT('Ctrl Pts',(2.41992431723751,-0.695615400200794,
99.8447043948388));
#31362=CARTESIAN_POINT('Ctrl Pts',(2.46502712732749,-0.52720241740103,99.8550526473507));
#31363=CARTESIAN_POINT('Ctrl Pts',(2.48871107969751,-0.400775635599492,
99.8624211203637));
#31364=CARTESIAN_POINT('Ctrl Pts',(2.51882209365799,-0.124833290852954,
99.8783715774892));
#31365=CARTESIAN_POINT('Ctrl Pts',(2.52179178959734,0.0245492073282939,
99.8869276120713));
#31366=CARTESIAN_POINT('Ctrl Pts',(2.51007837505082,0.194310620125791,99.8973821092228));
#31367=CARTESIAN_POINT('Ctrl Pts',(2.50836451956261,0.215307770712928,99.8986882551669));
#31368=CARTESIAN_POINT('Ctrl Pts',(2.50560231962577,0.244608342566125,99.9005322689086));
#31369=CARTESIAN_POINT('Ctrl Pts',(2.50477571856571,0.252932442346295,99.9010585534075));
#31370=CARTESIAN_POINT('Ctrl Pts',(2.50327494596153,0.267316233350858,99.9019723680417));
#31371=CARTESIAN_POINT('Ctrl Pts',(2.5026202114308,0.273377941928626,99.9023588298144));
#31372=CARTESIAN_POINT('Ctrl Pts',(2.50118831913558,0.286198405402891,99.9031791768506));
#31373=CARTESIAN_POINT('Ctrl Pts',(2.50040577515912,0.292956466604461,99.9036133680493));
#31374=CARTESIAN_POINT('Ctrl Pts',(2.49838846916877,0.309780831070077,99.9046985478704));
#31375=CARTESIAN_POINT('Ctrl Pts',(2.49712026275552,0.319842916402753,99.9053513506574));
#31376=CARTESIAN_POINT('Ctrl Pts',(2.49205349760046,0.358174862206502,99.9078520028741));
#31377=CARTESIAN_POINT('Ctrl Pts',(2.48783553122931,0.38638591304184,99.9097209856019));
#31378=CARTESIAN_POINT('Ctrl Pts',(2.47570363209417,0.45906119966978,99.9145994787303));
#31379=CARTESIAN_POINT('Ctrl Pts',(2.46707106238824,0.503394046827024,99.9176373758836));
#31380=CARTESIAN_POINT('Ctrl Pts',(2.43570506126359,0.644176966686166,99.9274366972328));
#31381=CARTESIAN_POINT('Ctrl Pts',(2.40846892117756,0.739526469686777,99.9343008425818));
#31382=CARTESIAN_POINT('Ctrl Pts',(2.3191026329755,0.994389894783269,99.9529475504126));
#31383=CARTESIAN_POINT('Ctrl Pts',(2.24621594600339,1.14960031661482,99.9646037198963));
#31384=CARTESIAN_POINT('Ctrl Pts',(2.14109869930211,1.32461238864522,99.9778706347512));
#31385=CARTESIAN_POINT('Ctrl Pts',(2.123499187026,1.35264666236637,99.9800015895634));
#31386=CARTESIAN_POINT('Ctrl Pts',(2.09705392522325,1.39298244581963,99.9830775331366));
#31387=CARTESIAN_POINT('Ctrl Pts',(2.08864248956696,1.40556317066546,99.9840383718916));
#31388=CARTESIAN_POINT('Ctrl Pts',(2.07351628226033,1.4277513213686,99.9857358185416));
#31389=CARTESIAN_POINT('Ctrl Pts',(2.06684696104278,1.43738904114406,99.986474097569));
#31390=CARTESIAN_POINT('Ctrl Pts',(2.05279516786746,1.457395017114,99.9880088222405));
#31391=CARTESIAN_POINT('Ctrl Pts',(2.04540086811087,1.46775458961472,99.9888047919328));
#31392=CARTESIAN_POINT('Ctrl Pts',(2.02589224956218,1.49465283695458,99.9908751037702));
#31393=CARTESIAN_POINT('Ctrl Pts',(2.01365376730967,1.51110061005555,99.992144657532));
#31394=CARTESIAN_POINT('Ctrl Pts',(1.95668383846331,1.58574333173377,99.9979254903962));
#31395=CARTESIAN_POINT('Ctrl Pts',(1.90961931177131,1.64211727161478,100.002344811465));
#31396=CARTESIAN_POINT('Ctrl Pts',(1.76389951369148,1.80190746587991,100.015150560017));
#31397=CARTESIAN_POINT('Ctrl Pts',(1.65883485042892,1.89907385266144,100.02329753858));
#31398=CARTESIAN_POINT('Ctrl Pts',(1.44419225937166,2.06610414381818,100.038950030559));
#31399=CARTESIAN_POINT('Ctrl Pts',(1.33635521910781,2.13743403016492,100.046425109566));
#31400=CARTESIAN_POINT('Ctrl Pts',(1.20478495203594,2.21060173083181,100.055669691945));
#31401=CARTESIAN_POINT('Ctrl Pts',(1.18589784753166,2.22079107926653,100.056999742303));
#31402=CARTESIAN_POINT('Ctrl Pts',(1.15941309549036,2.23464507287224,100.058872184406));
#31403=CARTESIAN_POINT('Ctrl Pts',(1.15192320709902,2.23851518821925,100.059402521055));
#31404=CARTESIAN_POINT('Ctrl Pts',(1.13896873938926,2.2451266861324,100.060321425775));
#31405=CARTESIAN_POINT('Ctrl Pts',(1.133513296191,2.24788594718178,100.060708896916));
#31406=CARTESIAN_POINT('Ctrl Pts',(1.12198301678767,2.25366510016705,100.061528993487));
#31407=CARTESIAN_POINT('Ctrl Pts',(1.11590595980867,2.25668034048018,100.061961910039));
#31408=CARTESIAN_POINT('Ctrl Pts',(1.10079728291441,2.26410083023689,100.063039775806));
#31409=CARTESIAN_POINT('Ctrl Pts',(1.0917514027577,2.26847660204163,100.063686488898));
#31410=CARTESIAN_POINT('Ctrl Pts',(1.05754263982345,2.28477243421418,100.066136646998));
#31411=CARTESIAN_POINT('Ctrl Pts',(1.03220980906839,2.29632843239281,100.067960174099));
#31412=CARTESIAN_POINT('Ctrl Pts',(0.966666143371022,2.32492361230966,100.072691880931));
#31413=CARTESIAN_POINT('Ctrl Pts',(0.926195056687779,2.3413405399953,100.075626498917));
#31414=CARTESIAN_POINT('Ctrl Pts',(0.768639052117084,2.40052827063299,100.087049427278));
#31415=CARTESIAN_POINT('Ctrl Pts',(0.648867022426873,2.43563389143778,100.095719729962));
#31416=CARTESIAN_POINT('Ctrl Pts',(0.369239986869788,2.49549468436993,100.1154075499));
#31417=CARTESIAN_POINT('Ctrl Pts',(0.208585270639053,2.5140288243754,100.126302880078));
#31418=CARTESIAN_POINT('Ctrl Pts',(0.0250081221962085,2.5174739586208,100.138145005431));
#31419=CARTESIAN_POINT('Ctrl Pts',(0.0027743267229852,2.51759665025779,
100.139569857757));
#31420=CARTESIAN_POINT('Ctrl Pts',(-0.0338447596654966,2.51731359810553,
100.141901682248));
#31421=CARTESIAN_POINT('Ctrl Pts',(-0.0482297650618556,2.51707908551078,
100.142813901784));
#31422=CARTESIAN_POINT('Ctrl Pts',(-0.0742166170519933,2.5164325719562,
100.144455239401));
#31423=CARTESIAN_POINT('Ctrl Pts',(-0.0858190349131048,2.51606361127331,
100.145185670808));
#31424=CARTESIAN_POINT('Ctrl Pts',(-0.110710887058315,2.5150996596882,100.146747804681));
#31425=CARTESIAN_POINT('Ctrl Pts',(-0.123999038446791,2.51447955806498,
100.147578705901));
#31426=CARTESIAN_POINT('Ctrl Pts',(-0.160389147140787,2.5124922111058,100.149846270356));
#31427=CARTESIAN_POINT('Ctrl Pts',(-0.183478505368552,2.51091168349873,
100.151276299863));
#31428=CARTESIAN_POINT('Ctrl Pts',(-0.319638003657398,2.49970295503817,
100.159662995256));
#31429=CARTESIAN_POINT('Ctrl Pts',(-0.431981189574384,2.48275656701698,
100.166385835976));
#31430=CARTESIAN_POINT('Ctrl Pts',(-0.716732383987043,2.41988122040865,
100.183349575387));
#31431=CARTESIAN_POINT('Ctrl Pts',(-0.88607518290481,2.3631320803081,100.193346019235));
#31432=CARTESIAN_POINT('Ctrl Pts',(-1.1040166779255,2.26334904939646,100.20754577466));
#31433=CARTESIAN_POINT('Ctrl Pts',(-1.15906728588436,2.23565727376039,100.211260555814));
#31434=CARTESIAN_POINT('Ctrl Pts',(-1.22490312215346,2.19945489149915,100.215928039093));
#31435=CARTESIAN_POINT('Ctrl Pts',(-1.2367112009774,2.19283717245522,100.216774272211));
#31436=CARTESIAN_POINT('Ctrl Pts',(-1.25508846518467,2.1823421757574,100.218106478637));
#31437=CARTESIAN_POINT('Ctrl Pts',(-1.26169456921249,2.17852960455198,100.218588468017));
#31438=CARTESIAN_POINT('Ctrl Pts',(-1.2738114515064,2.17146300755805,100.219478436802));
#31439=CARTESIAN_POINT('Ctrl Pts',(-1.27932725244667,2.16821792844192,100.219885847926));
#31440=CARTESIAN_POINT('Ctrl Pts',(-1.29187069108932,2.16077379347895,100.220817525588));
#31441=CARTESIAN_POINT('Ctrl Pts',(-1.29889023902018,2.1565614787385,100.221342627287));
#31442=CARTESIAN_POINT('Ctrl Pts',(-1.31367741888495,2.14758955090531,100.22245646249));
#31443=CARTESIAN_POINT('Ctrl Pts',(-1.32143999531492,2.14282187149945,100.223045683224));
#31444=CARTESIAN_POINT('Ctrl Pts',(-1.34207234909262,2.12999498642356,100.22462350113));
#31445=CARTESIAN_POINT('Ctrl Pts',(-1.35489516581668,2.12186142268706,100.225616344208));
#31446=CARTESIAN_POINT('Ctrl Pts',(-1.39433617550252,2.09634055297995,100.228706409022));
#31447=CARTESIAN_POINT('Ctrl Pts',(-1.42069827649272,2.07856520277309,100.230823409188));
#31448=CARTESIAN_POINT('Ctrl Pts',(-1.52679116202141,2.00406804702355,100.239534748647));
#31449=CARTESIAN_POINT('Ctrl Pts',(-1.60351631104104,1.94322239379069,100.246282271396));
#31450=CARTESIAN_POINT('Ctrl Pts',(-1.82304009585914,1.74725961386189,100.266610225599));
#31451=CARTESIAN_POINT('Ctrl Pts',(-1.95379324117827,1.59972212968044,100.280094468558));
#31452=CARTESIAN_POINT('Ctrl Pts',(-2.08242009810825,1.4149740410807,100.29470727203));
#31453=CARTESIAN_POINT('Ctrl Pts',(-2.0983685382003,1.39121335166108,100.296549850248));
#31454=CARTESIAN_POINT('Ctrl Pts',(-2.12184816567641,1.35490971203528,100.299311062109));
#31455=CARTESIAN_POINT('Ctrl Pts',(-2.12968041605005,1.3425651962399,100.300240747771));
#31456=CARTESIAN_POINT('Ctrl Pts',(-2.14314531557536,1.32092863069683,100.301854462248));
#31457=CARTESIAN_POINT('Ctrl Pts',(-2.14882609944345,1.31166714200441,100.302540240768));
#31458=CARTESIAN_POINT('Ctrl Pts',(-2.16060852563175,1.29217603793948,100.303973240295));
#31459=CARTESIAN_POINT('Ctrl Pts',(-2.166697897209,1.28193929033195,100.30472000344));
#31460=CARTESIAN_POINT('Ctrl Pts',(-2.1810757595999,1.25737376156694,100.30649834743));
#31461=CARTESIAN_POINT('Ctrl Pts',(-2.18929609688322,1.2430055776523,100.307527464739));
#31462=CARTESIAN_POINT('Ctrl Pts',(-2.21711572337141,1.19324791288143,100.311054625445));
#31463=CARTESIAN_POINT('Ctrl Pts',(-2.2360040118263,1.15746665181497,100.313527601605));
#31464=CARTESIAN_POINT('Ctrl Pts',(-2.27985520585807,1.06931316215215,100.319481384804));
#31465=CARTESIAN_POINT('Ctrl Pts',(-2.30388655375325,1.01650273290238,100.322932025619));
#31466=CARTESIAN_POINT('Ctrl Pts',(-2.33844529612365,0.933019893775969,
100.328243924807));
#31467=CARTESIAN_POINT('Ctrl Pts',(-2.35023265669797,0.902915552522292,
100.330131448148));
#31468=CARTESIAN_POINT('Ctrl Pts',(-2.36143107613335,0.872610750948945,
100.332008666168));
#31469=CARTESIAN_POINT('Origin',(0.,0.,104.));
#31470=CARTESIAN_POINT('',(-2.36143112101024,0.872610629504535,101.328714168996));
#31471=CARTESIAN_POINT('',(-2.36143112101025,0.872610629504514,101.056345051278));
#31472=CARTESIAN_POINT('',(-2.36143112101026,0.872610629504505,104.));
#31473=CARTESIAN_POINT('',(-2.51749904018607,0.00219833169228679,100.112583302458));
#31474=CARTESIAN_POINT('Ctrl Pts',(-2.36143112101025,0.872610629504513,
101.056345051278));
#31475=CARTESIAN_POINT('Ctrl Pts',(-2.33221131544371,0.951684337618625,
101.051018578518));
#31476=CARTESIAN_POINT('Ctrl Pts',(-2.29904688773595,1.02920461468538,101.045692105757));
#31477=CARTESIAN_POINT('Ctrl Pts',(-2.26214154918255,1.10477231204533,101.040365632997));
#31478=CARTESIAN_POINT('Ctrl Pts',(-2.22516722098647,1.18048127320729,101.035029203102));
#31479=CARTESIAN_POINT('Ctrl Pts',(-2.18443823344539,1.25422997984213,101.029692773206));
#31480=CARTESIAN_POINT('Ctrl Pts',(-2.14020305802366,1.32564592573815,101.024356343311));
#31481=CARTESIAN_POINT('Ctrl Pts',(-2.12269098834624,1.35391847148228,101.022243727473));
#31482=CARTESIAN_POINT('Ctrl Pts',(-2.10462986862105,1.3818257619343,101.020131111636));
#31483=CARTESIAN_POINT('Ctrl Pts',(-2.08603685581883,1.40934612007324,101.018018495799));
#31484=CARTESIAN_POINT('Ctrl Pts',(-2.03978570225557,1.47780454173625,101.012763246392));
#31485=CARTESIAN_POINT('Ctrl Pts',(-1.99007561770263,1.5441102083388,101.007507996984));
#31486=CARTESIAN_POINT('Ctrl Pts',(-1.93713376492452,1.60789272863253,101.002252747577));
#31487=CARTESIAN_POINT('Ctrl Pts',(-1.88426697166669,1.67158481980214,100.99700494892));
#31488=CARTESIAN_POINT('Ctrl Pts',(-1.82817780344503,1.73276051803598,100.991757150262));
#31489=CARTESIAN_POINT('Ctrl Pts',(-1.76913659410922,1.79107843529635,100.986509351605));
#31490=CARTESIAN_POINT('Ctrl Pts',(-1.70966758031225,1.84981891614324,100.981223528122));
#31491=CARTESIAN_POINT('Ctrl Pts',(-1.64720383001774,1.90565963442698,100.975937704639));
#31492=CARTESIAN_POINT('Ctrl Pts',(-1.58206291381019,1.95828577759897,100.970651881156));
#31493=CARTESIAN_POINT('Ctrl Pts',(-1.51750611170184,2.01044002577772,100.965413455287));
#31494=CARTESIAN_POINT('Ctrl Pts',(-1.45032032884715,2.0594368223821,100.960175029419));
#31495=CARTESIAN_POINT('Ctrl Pts',(-1.38085022903176,2.10500805104943,100.95493660355));
#31496=CARTESIAN_POINT('Ctrl Pts',(-1.31140297677613,2.15056429209802,100.949699900513));
#31497=CARTESIAN_POINT('Ctrl Pts',(-1.23967328514353,2.19269694983349,100.944463197475));
#31498=CARTESIAN_POINT('Ctrl Pts',(-1.16603553866773,2.23118071266401,100.939226494438));
#31499=CARTESIAN_POINT('Ctrl Pts',(-1.09239979804728,2.26966342721609,100.933989934045));
#31500=CARTESIAN_POINT('Ctrl Pts',(-1.01685651534236,2.30449723168084,100.928753373653));
#31501=CARTESIAN_POINT('Ctrl Pts',(-0.939804222611727,2.33550300217344,
100.923516813261));
#31502=CARTESIAN_POINT('Ctrl Pts',(-0.861490791548369,2.36701625355101,
100.91819454449));
#31503=CARTESIAN_POINT('Ctrl Pts',(-0.781618959216873,2.39457483546007,
100.91287227572));
#31504=CARTESIAN_POINT('Ctrl Pts',(-0.700625999889945,2.41804248479596,
100.907550006949));
#31505=CARTESIAN_POINT('Ctrl Pts',(-0.62082288636162,2.44116537720239,100.902305926199));
#31506=CARTESIAN_POINT('Ctrl Pts',(-0.539931837104716,2.46031668865465,
100.897061845448));
#31507=CARTESIAN_POINT('Ctrl Pts',(-0.458382389107362,2.4754175072816,100.891817764698));
#31508=CARTESIAN_POINT('Ctrl Pts',(-0.37500911625304,2.49085605043088,100.886456401918));
#31509=CARTESIAN_POINT('Ctrl Pts',(-0.290948147124191,2.50206067115167,
100.881095039137));
#31510=CARTESIAN_POINT('Ctrl Pts',(-0.206663042294775,2.50900311616974,
100.875733676356));
#31511=CARTESIAN_POINT('Ctrl Pts',(-0.122377937465359,2.51594556118781,
100.870372313576));
#31512=CARTESIAN_POINT('Ctrl Pts',(-0.0378692069043505,2.51862588116019,
100.865010950795));
#31513=CARTESIAN_POINT('Ctrl Pts',(0.046402630135093,2.51707231638595,100.859649588015));
#31514=CARTESIAN_POINT('Ctrl Pts',(0.129006538839197,2.51554950013695,100.854394338607));
#31515=CARTESIAN_POINT('Ctrl Pts',(0.211687953583553,2.50995328840563,100.8491390892));
#31516=CARTESIAN_POINT('Ctrl Pts',(0.294012513924796,2.50027256347296,100.843883839793));
#31517=CARTESIAN_POINT('Ctrl Pts',(0.376220356741427,2.49060556360904,100.838636041135));
#31518=CARTESIAN_POINT('Ctrl Pts',(0.458071895656362,2.47686560642341,100.833388242478));
#31519=CARTESIAN_POINT('Ctrl Pts',(0.539133593330857,2.45909357661358,100.82814044382));
#31520=CARTESIAN_POINT('Ctrl Pts',(0.620782652888353,2.44119277312649,100.822854620337));
#31521=CARTESIAN_POINT('Ctrl Pts',(0.701629902940013,2.41920122751496,100.817568796854));
#31522=CARTESIAN_POINT('Ctrl Pts',(0.781238379348301,2.39321391535175,100.812282973371));
#31523=CARTESIAN_POINT('Ctrl Pts',(0.860133012043689,2.3674596296229,100.807044547503));
#31524=CARTESIAN_POINT('Ctrl Pts',(0.937810551388953,2.33778109568757,100.801806121634));
#31525=CARTESIAN_POINT('Ctrl Pts',(1.0138584507114,2.30432143849791,100.796567695766));
#31526=CARTESIAN_POINT('Ctrl Pts',(1.08988133914533,2.27087278563268,100.791330992728));
#31527=CARTESIAN_POINT('Ctrl Pts',(1.16427522999031,2.23364566494747,100.78609428969));
#31528=CARTESIAN_POINT('Ctrl Pts',(1.23664729937749,2.19283143605302,100.780857586653));
#31529=CARTESIAN_POINT('Ctrl Pts',(1.30901739738581,2.15201831891769,100.775621026261));
#31530=CARTESIAN_POINT('Ctrl Pts',(1.37936538202917,2.10761851540511,100.770384465868));
#31531=CARTESIAN_POINT('Ctrl Pts',(1.4473240241734,2.05986878685282,100.765147905476));
#31532=CARTESIAN_POINT('Ctrl Pts',(1.51639496610264,2.0113375239566,100.759825636705));
#31533=CARTESIAN_POINT('Ctrl Pts',(1.58299723579442,1.95934596013392,100.754503367935));
#31534=CARTESIAN_POINT('Ctrl Pts',(1.6467784621474,1.9041866890112,100.749181099164));
#31535=CARTESIAN_POINT('Ctrl Pts',(1.70962269564533,1.84983774791642,100.743937018414));
#31536=CARTESIAN_POINT('Ctrl Pts',(1.76972792598464,1.79241392127543,100.738692937664));
#31537=CARTESIAN_POINT('Ctrl Pts',(1.82679410041291,1.73223253770866,100.733448856913));
#31538=CARTESIAN_POINT('Ctrl Pts',(1.88513653985536,1.67070521856585,100.728087494133));
#31539=CARTESIAN_POINT('Ctrl Pts',(1.94030201513892,1.6062958994179,100.722726131352));
#31540=CARTESIAN_POINT('Ctrl Pts',(1.99201444135701,1.53937802875874,100.717364768572));
#31541=CARTESIAN_POINT('Ctrl Pts',(2.0437268675751,1.47246015809956,100.712003405791));
#31542=CARTESIAN_POINT('Ctrl Pts',(2.09198600956505,1.40303419126748,100.70664204301));
#31543=CARTESIAN_POINT('Ctrl Pts',(2.13656482464557,1.33150178373416,100.70128068023));
#31544=CARTESIAN_POINT('Ctrl Pts',(2.18026132516602,1.26138516270322,100.696025430823));
#31545=CARTESIAN_POINT('Ctrl Pts',(2.220583291266,1.18898576367459,100.690770181415));
#31546=CARTESIAN_POINT('Ctrl Pts',(2.25728490926713,1.11466187177766,100.685514932008));
#31547=CARTESIAN_POINT('Ctrl Pts',(2.2939344927115,1.04044335427516,100.68026713335));
#31548=CARTESIAN_POINT('Ctrl Pts',(2.32697372076107,0.964306173764744,100.675019334693));
#31549=CARTESIAN_POINT('Ctrl Pts',(2.35620084710383,0.88663623775886,100.669771536035));
#31550=CARTESIAN_POINT('Ctrl Pts',(2.38563974917372,0.808403516107192,100.664485712553));
#31551=CARTESIAN_POINT('Ctrl Pts',(2.41121082187184,0.728616135147747,100.65919988907));
#31552=CARTESIAN_POINT('Ctrl Pts',(2.43275582416911,0.647692326626838,100.653914065587));
#31553=CARTESIAN_POINT('Ctrl Pts',(2.45410763391796,0.567494156311032,100.648675639718));
#31554=CARTESIAN_POINT('Ctrl Pts',(2.47150516617165,0.486180311445731,100.64343721385));
#31555=CARTESIAN_POINT('Ctrl Pts',(2.48484386135593,0.404174757600901,100.638198787981));
#31556=CARTESIAN_POINT('Ctrl Pts',(2.49817816966534,0.322196174018033,100.632962084944));
#31557=CARTESIAN_POINT('Ctrl Pts',(2.50745621803731,0.239526788342451,100.627725381906));
#31558=CARTESIAN_POINT('Ctrl Pts',(2.51262464386841,0.15660028424354,100.622488678869));
#31559=CARTESIAN_POINT('Ctrl Pts',(2.51779292891417,0.0736760390211448,
100.617252118476));
#31560=CARTESIAN_POINT('Ctrl Pts',(2.51885178631918,-0.0095048501080237,
100.612015558084));
#31561=CARTESIAN_POINT('Ctrl Pts',(2.51579987119145,-0.0925054490994754,
100.606778997692));
#31562=CARTESIAN_POINT('Ctrl Pts',(2.51269800443971,-0.176864544163071,
100.601456728921));
#31563=CARTESIAN_POINT('Ctrl Pts',(2.50534959151306,-0.261036902240307,
100.596134460151));
#31564=CARTESIAN_POINT('Ctrl Pts',(2.49380820869186,-0.344567654113217,
100.59081219138));
#31565=CARTESIAN_POINT('Ctrl Pts',(2.48243637722391,-0.426871278159488,
100.58556811063));
#31566=CARTESIAN_POINT('Ctrl Pts',(2.46699410093658,-0.508551573722867,
100.58032402988));
#31567=CARTESIAN_POINT('Ctrl Pts',(2.44758418843908,-0.589184088806719,
100.575079949129));
#31568=CARTESIAN_POINT('Ctrl Pts',(2.42774018004335,-0.671619921863586,
100.569718586349));
#31569=CARTESIAN_POINT('Ctrl Pts',(2.40374906918176,-0.752960051295377,
100.564357223568));
#31570=CARTESIAN_POINT('Ctrl Pts',(2.37577378671153,-0.832769574596934,
100.558995860788));
#31571=CARTESIAN_POINT('Ctrl Pts',(2.3477985042413,-0.912579097898504,100.553634498007));
#31572=CARTESIAN_POINT('Ctrl Pts',(2.31583930406201,-0.990857569907529,
100.548273135227));
#31573=CARTESIAN_POINT('Ctrl Pts',(2.28010947794237,-1.06719586702601,100.542911772446));
#31574=CARTESIAN_POINT('Ctrl Pts',(2.24508682507885,-1.14202325832703,100.537656523039));
#31575=CARTESIAN_POINT('Ctrl Pts',(2.20631212510909,-1.21526297823443,100.532401273631));
#31576=CARTESIAN_POINT('Ctrl Pts',(2.16395207119459,-1.28651377123318,100.527146024224));
#31577=CARTESIAN_POINT('Ctrl Pts',(2.12165207421342,-1.35766354679385,100.521898225567));
#31578=CARTESIAN_POINT('Ctrl Pts',(2.07577705387272,-1.42682960317234,100.516650426909));
#31579=CARTESIAN_POINT('Ctrl Pts',(2.02654086532222,-1.49363260917103,100.511402628252));
#31580=CARTESIAN_POINT('Ctrl Pts',(1.97694791813915,-1.56091966053906,100.506116804769));
#31581=CARTESIAN_POINT('Ctrl Pts',(1.92394508898334,-1.62580884315666,100.500830981286));
#31582=CARTESIAN_POINT('Ctrl Pts',(1.8677970328417,-1.68793971874227,100.495545157803));
#31583=CARTESIAN_POINT('Ctrl Pts',(1.81215245244386,-1.74951347105509,100.490306731934));
#31584=CARTESIAN_POINT('Ctrl Pts',(1.75341914028613,-1.80837783666159,100.485068306066));
#31585=CARTESIAN_POINT('Ctrl Pts',(1.69189578779433,-1.86421428308116,100.479829880197));
#31586=CARTESIAN_POINT('Ctrl Pts',(1.63039266930932,-1.92003236582271,100.47459317716));
#31587=CARTESIAN_POINT('Ctrl Pts',(1.56610167430342,-1.97282419729981,100.469356474122));
#31588=CARTESIAN_POINT('Ctrl Pts',(1.49935751994002,-2.02230889762156,100.464119771085));
#31589=CARTESIAN_POINT('Ctrl Pts',(1.43261518365403,-2.0717922500048,100.458883210692));
#31590=CARTESIAN_POINT('Ctrl Pts',(1.36342019214502,-2.11796837636214,100.4536466503));
#31591=CARTESIAN_POINT('Ctrl Pts',(1.29213831009011,-2.16059825918598,100.448410089908));
#31592=CARTESIAN_POINT('Ctrl Pts',(1.21968973577056,-2.20392587828022,100.443087821137));
#31593=CARTESIAN_POINT('Ctrl Pts',(1.14508575630058,-2.24358985796055,100.437765552367));
#31594=CARTESIAN_POINT('Ctrl Pts',(1.06873708216042,-2.27938748334179,100.432443283596));
#31595=CARTESIAN_POINT('Ctrl Pts',(0.993510025873493,-2.31465921542911,
100.427199202846));
#31596=CARTESIAN_POINT('Ctrl Pts',(0.916589652673124,-2.34617731763915,
100.421955122096));
#31597=CARTESIAN_POINT('Ctrl Pts',(0.838387963927298,-2.373796931488,100.416711041345));
#31598=CARTESIAN_POINT('Ctrl Pts',(0.758437321787985,-2.40203424833205,
100.411349678565));
#31599=CARTESIAN_POINT('Ctrl Pts',(0.677147850984888,-2.42619645007273,
100.405988315784));
#31600=CARTESIAN_POINT('Ctrl Pts',(0.594973052343718,-2.44618341850827,
100.400626953004));
#31601=CARTESIAN_POINT('Ctrl Pts',(0.512798253702537,-2.46617038694381,
100.395265590223));
#31602=CARTESIAN_POINT('Ctrl Pts',(0.429738638858018,-2.48198209267392,
100.389904227443));
#31603=CARTESIAN_POINT('Ctrl Pts',(0.346253504564266,-2.49357469520706,
100.384542864662));
#31604=CARTESIAN_POINT('Ctrl Pts',(0.264420727997514,-2.50493785418077,
100.379287615255));
#31605=CARTESIAN_POINT('Ctrl Pts',(0.181876870043046,-2.51228941481946,
100.374032365847));
#31606=CARTESIAN_POINT('Ctrl Pts',(0.0990492570832516,-2.51555073386948,
100.36877711644));
#31607=CARTESIAN_POINT('Ctrl Pts',(0.0163390748624143,-2.51880742910996,
100.363529317783));
#31608=CARTESIAN_POINT('Ctrl Pts',(-0.0666536060613034,-2.51798538333177,
100.358281519125));
#31609=CARTESIAN_POINT('Ctrl Pts',(-0.149494171835672,-2.51305744912192,
100.353033720468));
#31610=CARTESIAN_POINT('Ctrl Pts',(-0.232934988926288,-2.50809380778033,
100.347747896985));
#31611=CARTESIAN_POINT('Ctrl Pts',(-0.316221007771172,-2.49896446036227,
100.342462073502));
#31612=CARTESIAN_POINT('Ctrl Pts',(-0.398905803699714,-2.48569515624396,
100.337176250019));
#31613=CARTESIAN_POINT('Ctrl Pts',(-0.48084917077028,-2.47254483705979,
100.33193782415));
#31614=CARTESIAN_POINT('Ctrl Pts',(-0.562201590002327,-2.45532858368273,
100.326699398282));
#31615=CARTESIAN_POINT('Ctrl Pts',(-0.642533255795456,-2.43412351067009,
100.321460972413));
#31616=CARTESIAN_POINT('Ctrl Pts',(-0.72283850184065,-2.41292541165306,
100.316224269376));
#31617=CARTESIAN_POINT('Ctrl Pts',(-0.802123215395963,-2.38774121609325,
100.310987566338));
#31618=CARTESIAN_POINT('Ctrl Pts',(-0.879969559293769,-2.35869875666994,
100.305750863301));
#31619=CARTESIAN_POINT('Ctrl Pts',(-0.957813782695915,-2.32965708834878,
100.300514302908));
#31620=CARTESIAN_POINT('Ctrl Pts',(-1.03421928238705,-2.29675752737585,
100.295277742516));
#31621=CARTESIAN_POINT('Ctrl Pts',(-1.10878643117635,-2.26017674088537,
100.290041182124));
#31622=CARTESIAN_POINT('Ctrl Pts',(-1.1845740431915,-2.22299722552555,100.284718913353));
#31623=CARTESIAN_POINT('Ctrl Pts',(-1.25846213642939,-2.18201509875608,
100.279396644583));
#31624=CARTESIAN_POINT('Ctrl Pts',(-1.33005706324611,-2.1374644929236,100.274074375812));
#31625=CARTESIAN_POINT('Ctrl Pts',(-1.40060020823375,-2.09356836806864,
100.268830295062));
#31626=CARTESIAN_POINT('Ctrl Pts',(-1.46891676647575,-2.04620823240409,
100.263586214312));
#31627=CARTESIAN_POINT('Ctrl Pts',(-1.53466091700543,-1.99565080107118,
100.258342133561));
#31628=CARTESIAN_POINT('Ctrl Pts',(-1.6018754124476,-1.94396267048442,100.252980770781));
#31629=CARTESIAN_POINT('Ctrl Pts',(-1.66640066013577,-1.88893283796383,
100.247619408));
#31630=CARTESIAN_POINT('Ctrl Pts',(-1.72790577246219,-1.8308871869921,100.24225804522));
#31631=CARTESIAN_POINT('Ctrl Pts',(-1.78941088478861,-1.77284153602037,
100.236896682439));
#31632=CARTESIAN_POINT('Ctrl Pts',(-1.84789555853221,-1.71178047974573,
100.231535319659));
#31633=CARTESIAN_POINT('Ctrl Pts',(-1.90307295579216,-1.64806540371809,
100.226173956878));
#31634=CARTESIAN_POINT('Ctrl Pts',(-1.95670661292151,-1.5861329329722,100.220962593033));
#31635=CARTESIAN_POINT('Ctrl Pts',(-2.00742189654769,-1.52145466982403,
100.215751229189));
#31636=CARTESIAN_POINT('Ctrl Pts',(-2.05492184315158,-1.45433918620744,
100.210539865344));
#31637=CARTESIAN_POINT('Ctrl Pts',(-2.10235895333139,-1.38731248789047,
100.205335395475));
#31638=CARTESIAN_POINT('Ctrl Pts',(-2.14658889768153,-1.31785534578256,
100.200130925606));
#31639=CARTESIAN_POINT('Ctrl Pts',(-2.18735350234669,-1.24631091857997,
100.194926455737));
#31640=CARTESIAN_POINT('Ctrl Pts',(-2.22807698574017,-1.17483866177749,
100.189727235874));
#31641=CARTESIAN_POINT('Ctrl Pts',(-2.2653418369109,-1.10128370482761,100.184528016011));
#31642=CARTESIAN_POINT('Ctrl Pts',(-2.29893280601451,-1.02601861748716,
100.179328796148));
#31643=CARTESIAN_POINT('Ctrl Pts',(-2.33250043822008,-0.950805819607697,
100.174133188376));
#31644=CARTESIAN_POINT('Ctrl Pts',(-2.36239906650357,-0.873885678468057,
100.168937580605));
#31645=CARTESIAN_POINT('Ctrl Pts',(-2.38845978937943,-0.79565450072098,
100.163741972834));
#31646=CARTESIAN_POINT('Ctrl Pts',(-2.41451585326278,-0.717437308713033,
100.158547293905));
#31647=CARTESIAN_POINT('Ctrl Pts',(-2.43673521726057,-0.637909987852045,
100.153352614975));
#31648=CARTESIAN_POINT('Ctrl Pts',(-2.45499791486481,-0.557486760389387,
100.148157936046));
#31649=CARTESIAN_POINT('Ctrl Pts',(-2.47325894911605,-0.477070857814841,
100.142963730245));
#31650=CARTESIAN_POINT('Ctrl Pts',(-2.48756393627921,-0.395759670401945,
100.137769524443));
#31651=CARTESIAN_POINT('Ctrl Pts',(-2.49784379623169,-0.313978692950392,
100.132575318641));
#31652=CARTESIAN_POINT('Ctrl Pts',(-2.50812919165291,-0.232153678318772,
100.127378315879));
#31653=CARTESIAN_POINT('Ctrl Pts',(-2.51438508505061,-0.149858835943071,
100.122181313117));
#31654=CARTESIAN_POINT('Ctrl Pts',(-2.51659425685113,-0.0675247834792372,
100.116984310354));
#31655=CARTESIAN_POINT('Ctrl Pts',(-2.51721785875581,-0.044283643100605,
100.115517307734));
#31656=CARTESIAN_POINT('Ctrl Pts',(-2.51751933182795,-0.021039381607636,
100.114050305113));
#31657=CARTESIAN_POINT('Ctrl Pts',(-2.51749904018654,0.00219833114783364,
100.112583302492));
#31658=CARTESIAN_POINT('Ctrl Pts',(-2.51749904018607,0.00219833169228797,
100.112583302458));
#31659=CARTESIAN_POINT('Ctrl Pts',(-2.51741017424848,0.103966373959212,
100.106158660485));
#31660=CARTESIAN_POINT('Ctrl Pts',(-2.51114671053894,0.205464160514488,
100.099734018512));
#31661=CARTESIAN_POINT('Ctrl Pts',(-2.49882897256204,0.30603923912551,100.093309376539));
#31662=CARTESIAN_POINT('Ctrl Pts',(-2.48631365676557,0.408227552631852,
100.08678168263));
#31663=CARTESIAN_POINT('Ctrl Pts',(-2.46754833857112,0.509463401282088,
100.080253988721));
#31664=CARTESIAN_POINT('Ctrl Pts',(-2.4427078667328,0.609084992264386,100.073726294811));
#31665=CARTESIAN_POINT('Ctrl Pts',(-2.43519696831913,0.639207111302466,
100.071752546239));
#31666=CARTESIAN_POINT('Ctrl Pts',(-2.42713098016373,0.669181796368386,
100.069778797666));
#31667=CARTESIAN_POINT('Ctrl Pts',(-2.41851558766757,0.698991131709841,
100.067805049094));
#31668=CARTESIAN_POINT('Ctrl Pts',(-2.40161875451569,0.757454326028318,
100.063934058849));
#31669=CARTESIAN_POINT('Ctrl Pts',(-2.38257788982076,0.815383916593283,
100.060063068603));
#31670=CARTESIAN_POINT('Ctrl Pts',(-2.36143112101026,0.8726106295045,100.056192078358));
#31671=CARTESIAN_POINT('',(-2.51749994369438,0.000532446056795771,100.385185287451));
#31672=CARTESIAN_POINT('Ctrl Pts',(-2.36143107613335,0.872610750948947,
100.332008666168));
#31673=CARTESIAN_POINT('Ctrl Pts',(-2.43054338807988,0.685581240945225,
100.343594129468));
#31674=CARTESIAN_POINT('Ctrl Pts',(-2.47722505275429,0.490913466893775,
100.354730759386));
#31675=CARTESIAN_POINT('Ctrl Pts',(-2.50506290388481,0.253091072209852,
100.369154925959));
#31676=CARTESIAN_POINT('Ctrl Pts',(-2.50875596153332,0.213397201095081,
100.371591126473));
#31677=CARTESIAN_POINT('Ctrl Pts',(-2.51232472874635,0.161777557736847,
100.374815693234));
#31678=CARTESIAN_POINT('Ctrl Pts',(-2.51306050061653,0.149914736060504,
100.375560598103));
#31679=CARTESIAN_POINT('Ctrl Pts',(-2.51410616662273,0.130874153104245,
100.376763043139));
#31680=CARTESIAN_POINT('Ctrl Pts',(-2.51446939378066,0.123699335771165,
100.377217698691));
#31681=CARTESIAN_POINT('Ctrl Pts',(-2.51509055639182,0.110293410338815,
100.378070273606));
#31682=CARTESIAN_POINT('Ctrl Pts',(-2.51535605427957,0.104062769533399,
100.378467771644));
#31683=CARTESIAN_POINT('Ctrl Pts',(-2.51585327150832,0.0912775083612031,
100.379285929411));
#31684=CARTESIAN_POINT('Ctrl Pts',(-2.516082532118,0.0847228219647258,100.379706719003));
#31685=CARTESIAN_POINT('Ctrl Pts',(-2.5166489074665,0.0664906381077124,
100.380880754559));
#31686=CARTESIAN_POINT('Ctrl Pts',(-2.51693035026904,0.0548117507589939,
100.381636892936));
#31687=CARTESIAN_POINT('Ctrl Pts',(-2.51737379221875,0.028932779951975,
100.383320851271));
#31688=CARTESIAN_POINT('Ctrl Pts',(-2.51749694040091,0.0147325533313436,
100.384250501894));
#31689=CARTESIAN_POINT('Ctrl Pts',(-2.51749994369438,0.000532446056795771,
100.385185287451));
#31690=CARTESIAN_POINT('Ctrl Pts',(-2.51749994318663,0.000534841376573433,
100.385185129769));
#31691=CARTESIAN_POINT('Ctrl Pts',(-2.51752973780924,-0.139708535471339,
100.394417271433));
#31692=CARTESIAN_POINT('Ctrl Pts',(-2.50584061409508,-0.279702207492776,
100.404120224013));
#31693=CARTESIAN_POINT('Ctrl Pts',(-2.46143942510912,-0.543416172880637,
100.422594579596));
#31694=CARTESIAN_POINT('Ctrl Pts',(-2.43084320016804,-0.667077391207286,
100.43134273588));
#31695=CARTESIAN_POINT('Ctrl Pts',(-2.36715576456412,-0.860347345119606,
100.444943440311));
#31696=CARTESIAN_POINT('Ctrl Pts',(-2.34000254505476,-0.931672720395224,
100.44994937167));
#31697=CARTESIAN_POINT('Ctrl Pts',(-2.30139294388001,-1.02069945985187,
100.456182180973));
#31698=CARTESIAN_POINT('Ctrl Pts',(-2.29290112967272,-1.03963518656407,
100.457507093384));
#31699=CARTESIAN_POINT('Ctrl Pts',(-2.27880177953355,-1.07006171928804,
100.459635240386));
#31700=CARTESIAN_POINT('Ctrl Pts',(-2.27333929020811,-1.08161828519615,
100.460443372284));
#31701=CARTESIAN_POINT('Ctrl Pts',(-2.26270711370638,-1.10367555908132,
100.461985646782));
#31702=CARTESIAN_POINT('Ctrl Pts',(-2.25755176746683,-1.11418277080741,
100.462720257459));
#31703=CARTESIAN_POINT('Ctrl Pts',(-2.24561386540841,-1.1380905855448,100.464391815965));
#31704=CARTESIAN_POINT('Ctrl Pts',(-2.23878424739747,-1.15146729107778,
100.465327104939));
#31705=CARTESIAN_POINT('Ctrl Pts',(-2.21681343613066,-1.1935654838543,100.468271364172));
#31706=CARTESIAN_POINT('Ctrl Pts',(-2.20123576423728,-1.22205631315929,
100.47026507277));
#31707=CARTESIAN_POINT('Ctrl Pts',(-2.09244022226173,-1.41220422413403,
100.483597045362));
#31708=CARTESIAN_POINT('Ctrl Pts',(-1.98204949032737,-1.56336674323794,
100.494267458906));
#31709=CARTESIAN_POINT('Ctrl Pts',(-1.78535499606566,-1.77798546479413,
100.511004895734));
#31710=CARTESIAN_POINT('Ctrl Pts',(-1.71003240461132,-1.85054337514874,
100.517028044717));
#31711=CARTESIAN_POINT('Ctrl Pts',(-1.60526470560482,-1.93959325553429,
100.525250826708));
#31712=CARTESIAN_POINT('Ctrl Pts',(-1.57968561426048,-1.96048206515904,
100.527247591794));
#31713=CARTESIAN_POINT('Ctrl Pts',(-1.54143627863174,-1.99048324446703,
100.530230060865));
#31714=CARTESIAN_POINT('Ctrl Pts',(-1.52907945201058,-1.99999133768001,
100.531193077928));
#31715=CARTESIAN_POINT('Ctrl Pts',(-1.5092341647605,-2.01497009201315,100.532740332215));
#31716=CARTESIAN_POINT('Ctrl Pts',(-1.50180220830475,-2.02051536912354,
100.533319910044));
#31717=CARTESIAN_POINT('Ctrl Pts',(-1.48778105545493,-2.03085701184175,
100.534413957143));
#31718=CARTESIAN_POINT('Ctrl Pts',(-1.48119884839694,-2.03566270257414,
100.53492780706));
#31719=CARTESIAN_POINT('Ctrl Pts',(-1.47456163479772,-2.04045932003837,
100.535446331092));
#31720=CARTESIAN_POINT('Ctrl Pts',(-1.47452973746517,-2.04048237063682,
100.53544882304));
#31721=CARTESIAN_POINT('Ctrl Pts',(-1.47446555227998,-2.04052875175198,
100.535453837463));
#31722=CARTESIAN_POINT('Ctrl Pts',(-1.47443326437138,-2.04055208228116,
100.535456359942));
#31723=CARTESIAN_POINT('Ctrl Pts',(-1.47436828569953,-2.04059903208592,
100.535461436392));
#31724=CARTESIAN_POINT('Ctrl Pts',(-1.47433559497287,-2.04062265130585,
100.53546399036));
#31725=CARTESIAN_POINT('Ctrl Pts',(-1.47426979792777,-2.04067018760653,
100.535469130782));
#31726=CARTESIAN_POINT('Ctrl Pts',(-1.47423669158589,-2.04069410467369,
100.535471717239));
#31727=CARTESIAN_POINT('Ctrl Pts',(-1.47417005008962,-2.04074224612766,
100.535476923672));
#31728=CARTESIAN_POINT('Ctrl Pts',(-1.47413651492153,-2.0407664704925,100.535479543651));
#31729=CARTESIAN_POINT('Ctrl Pts',(-1.47406900203198,-2.0408152363713,100.535484818203));
#31730=CARTESIAN_POINT('Ctrl Pts',(-1.47403502428251,-2.04083977787215,
100.535487472778));
#31731=CARTESIAN_POINT('Ctrl Pts',(-1.47396661192414,-2.04088918825523,
100.535492817643));
#31732=CARTESIAN_POINT('Ctrl Pts',(-1.47393217732338,-2.04091405709672,
100.535495507931));
#31733=CARTESIAN_POINT('Ctrl Pts',(-1.47386283644238,-2.04096413275879,
100.535500925381));
#31734=CARTESIAN_POINT('Ctrl Pts',(-1.47382793010014,-2.04098933958769,
100.535503652546));
#31735=CARTESIAN_POINT('Ctrl Pts',(-1.4737576302921,-2.04104010226688,100.535509144957));
#31736=CARTESIAN_POINT('Ctrl Pts',(-1.47372223678655,-2.04106565810771,
100.535511910206));
#31737=CARTESIAN_POINT('Ctrl Pts',(-1.47365094652265,-2.04111713034141,
100.535517480044));
#31738=CARTESIAN_POINT('Ctrl Pts',(-1.47361504978321,-2.04114304668063,
100.535520284632));
#31739=CARTESIAN_POINT('Ctrl Pts',(-1.47354273632298,-2.04119525186765,
100.535525934456));
#31740=CARTESIAN_POINT('Ctrl Pts',(-1.47350631956427,-2.04122154070092,
100.535528779696));
#31741=CARTESIAN_POINT('Ctrl Pts',(-1.47343294860229,-2.04127450335575,
100.53553451219));
#31742=CARTESIAN_POINT('Ctrl Pts',(-1.47339599441321,-2.04130117712311,
100.535537399443));
#31743=CARTESIAN_POINT('Ctrl Pts',(-1.47332153040682,-2.04135492263829,
100.535543217385));
#31744=CARTESIAN_POINT('Ctrl Pts',(-1.47328402057315,-2.04138199435178,
100.535546148076));
#31745=CARTESIAN_POINT('Ctrl Pts',(-1.46810454667195,-2.04511992320656,
100.535950828614));
#31746=CARTESIAN_POINT('Ctrl Pts',(-1.46294876346809,-2.04881121000888,
100.536353901632));
#31747=CARTESIAN_POINT('Ctrl Pts',(-1.45151404511931,-2.056932734988,100.537248441393));
#31748=CARTESIAN_POINT('Ctrl Pts',(-1.44522884787628,-2.06135365063044,
100.537740499733));
#31749=CARTESIAN_POINT('Ctrl Pts',(-1.42760949516564,-2.07362665364172,
100.539120687512));
#31750=CARTESIAN_POINT('Ctrl Pts',(-1.41623112356966,-2.08141436378788,
100.540012910354));
#31751=CARTESIAN_POINT('Ctrl Pts',(-1.35022360077575,-2.12580014252044,
100.545191419694));
#31752=CARTESIAN_POINT('Ctrl Pts',(-1.29424569805979,-2.16033712830925,
100.549592743342));
#31753=CARTESIAN_POINT('Ctrl Pts',(-1.08585130542124,-2.27790356877152,
100.565844555821));
#31754=CARTESIAN_POINT('Ctrl Pts',(-0.926305199992865,-2.34731358354033,
100.577998967716));
#31755=CARTESIAN_POINT('Ctrl Pts',(-0.652745184636279,-2.43404989738921,
100.59750089615));
#31756=CARTESIAN_POINT('Ctrl Pts',(-0.542404047051818,-2.46099152771537,
100.605043522307));
#31757=CARTESIAN_POINT('Ctrl Pts',(-0.407808109120123,-2.48435791799471,
100.613840533917));
#31758=CARTESIAN_POINT('Ctrl Pts',(-0.384954846368719,-2.48800151591862,
100.615320800282));
#31759=CARTESIAN_POINT('Ctrl Pts',(-0.34889035509464,-2.49324260955437,
100.617636402209));
#31760=CARTESIAN_POINT('Ctrl Pts',(-0.335711599323228,-2.49505128666623,
100.618478308275));
#31761=CARTESIAN_POINT('Ctrl Pts',(-0.311006546606393,-2.4982425671217,
100.620048777101));
#31762=CARTESIAN_POINT('Ctrl Pts',(-0.299483875279866,-2.49965005789153,
100.62077809936));
#31763=CARTESIAN_POINT('Ctrl Pts',(-0.273659274240288,-2.50262339029238,
100.622405775569));
#31764=CARTESIAN_POINT('Ctrl Pts',(-0.25935275315271,-2.50414644041181,
100.623302772622));
#31765=CARTESIAN_POINT('Ctrl Pts',(-0.222905182427715,-2.50771088550437,
100.625576459702));
#31766=CARTESIAN_POINT('Ctrl Pts',(-0.200748425042117,-2.50958178264796,
100.626947844484));
#31767=CARTESIAN_POINT('Ctrl Pts',(-0.0175577544293523,-2.52260852386498,
100.638203970951));
#31768=CARTESIAN_POINT('Ctrl Pts',(0.144189140867329,-2.51854738858078,
100.647583991415));
#31769=CARTESIAN_POINT('Ctrl Pts',(0.428316965986693,-2.4839326107074,100.664050429519));
#31770=CARTESIAN_POINT('Ctrl Pts',(0.550881788152934,-2.45965491945854,
100.671161290666));
#31771=CARTESIAN_POINT('Ctrl Pts',(0.713091661984844,-2.41478812658416,
100.681116238134));
#31772=CARTESIAN_POINT('Ctrl Pts',(0.754739344349178,-2.40209690002524,
100.683723091115));
#31773=CARTESIAN_POINT('Ctrl Pts',(0.822390400142762,-2.37954871150869,
100.688072658506));
#31774=CARTESIAN_POINT('Ctrl Pts',(0.848597674510532,-2.3703290657677,100.689786509709));
#31775=CARTESIAN_POINT('Ctrl Pts',(0.884060450968069,-2.35718988910627,
100.692152019308));
#31776=CARTESIAN_POINT('Ctrl Pts',(0.893454018587902,-2.35364546245515,
100.69278308648));
#31777=CARTESIAN_POINT('Ctrl Pts',(0.909157060713876,-2.34761276359627,
100.693845949014));
#31778=CARTESIAN_POINT('Ctrl Pts',(0.915478255372784,-2.34515496523902,
100.694275962354));
#31779=CARTESIAN_POINT('Ctrl Pts',(0.927479896712491,-2.34043258537347,
100.695096657117));
#31780=CARTESIAN_POINT('Ctrl Pts',(0.933162161070506,-2.33817279616173,
100.695487038634));
#31781=CARTESIAN_POINT('Ctrl Pts',(0.946664424333978,-2.33274599999782,
100.69641890245));
#31782=CARTESIAN_POINT('Ctrl Pts',(0.9544767879934,-2.32956036392274,100.696961468087));
#31783=CARTESIAN_POINT('Ctrl Pts',(0.98213832168642,-2.31811835900239,100.698894235719));
#31784=CARTESIAN_POINT('Ctrl Pts',(1.0018969496591,-2.30964734086693,100.70029623475));
#31785=CARTESIAN_POINT('Ctrl Pts',(1.13895276789552,-2.24879852893442,100.710159480568));
#31786=CARTESIAN_POINT('Ctrl Pts',(1.25218880544355,-2.18776716672089,100.719010663151));
#31787=CARTESIAN_POINT('Ctrl Pts',(1.46171080475726,-2.05322751427586,100.736210891805));
#31788=CARTESIAN_POINT('Ctrl Pts',(1.55835624891013,-1.98087644707488,100.744535329385));
#31789=CARTESIAN_POINT('Ctrl Pts',(1.71994735376084,-1.84073233757755,100.758951118939));
#31790=CARTESIAN_POINT('Ctrl Pts',(1.78699754995469,-1.77571331625135,100.765113382837));
#31791=CARTESIAN_POINT('Ctrl Pts',(1.86522348224368,-1.69092656821955,100.77253337927));
#31792=CARTESIAN_POINT('Ctrl Pts',(1.87994511134387,-1.6745440354028,100.773941005402));
#31793=CARTESIAN_POINT('Ctrl Pts',(1.90305106604264,-1.6481424225682,100.776169044908));
#31794=CARTESIAN_POINT('Ctrl Pts',(1.91157540483741,-1.63824793212065,100.776995221986));
#31795=CARTESIAN_POINT('Ctrl Pts',(1.9275515513349,-1.61940939010025,100.778551836963));
#31796=CARTESIAN_POINT('Ctrl Pts',(1.93501903943477,-1.6104791461357,100.779282902469));
#31797=CARTESIAN_POINT('Ctrl Pts',(1.95181042099421,-1.5901132114171,100.780934927466));
#31798=CARTESIAN_POINT('Ctrl Pts',(1.96109631449772,-1.57864663700044,100.781854346018));
#31799=CARTESIAN_POINT('Ctrl Pts',(1.98908614633528,-1.54345560040798,100.784644243067));
#31800=CARTESIAN_POINT('Ctrl Pts',(2.00746475018736,-1.51947500284881,100.786501910579));
#31801=CARTESIAN_POINT('Ctrl Pts',(2.15079634878779,-1.32531298603206,100.801217378728));
#31802=CARTESIAN_POINT('Ctrl Pts',(2.25432000658865,-1.14036354187834,100.813180005293));
#31803=CARTESIAN_POINT('Ctrl Pts',(2.37987546058945,-0.830206190917561,
100.83247331388));
#31804=CARTESIAN_POINT('Ctrl Pts',(2.41771590813143,-0.712524801985291,
100.839662104704));
#31805=CARTESIAN_POINT('Ctrl Pts',(2.45099165677794,-0.575124328726661,
100.848388804461));
#31806=CARTESIAN_POINT('Ctrl Pts',(2.45502768435253,-0.557644260879512,
100.849505138059));
#31807=CARTESIAN_POINT('Ctrl Pts',(2.46068773667247,-0.531877230564108,
100.851161686432));
#31808=CARTESIAN_POINT('Ctrl Pts',(2.46245753159908,-0.523622407856458,
100.85169403476));
#31809=CARTESIAN_POINT('Ctrl Pts',(2.46552146717394,-0.508972219075985,
100.852641990214));
#31810=CARTESIAN_POINT('Ctrl Pts',(2.46683231035741,-0.502580517009345,
100.85305665015));
#31811=CARTESIAN_POINT('Ctrl Pts',(2.46962277753576,-0.488700166624528,
100.853959536102));
#31812=CARTESIAN_POINT('Ctrl Pts',(2.47109317259254,-0.481209980026606,
100.854448246804));
#31813=CARTESIAN_POINT('Ctrl Pts',(2.47508136688199,-0.460393745800301,
100.855810356001));
#31814=CARTESIAN_POINT('Ctrl Pts',(2.47752553816796,-0.447054093272045,
100.856687683765));
#31815=CARTESIAN_POINT('Ctrl Pts',(2.4905503793018,-0.372578359732025,100.861608164114));
#31816=CARTESIAN_POINT('Ctrl Pts',(2.4989750429939,-0.311091946583115,100.865753776924));
#31817=CARTESIAN_POINT('Ctrl Pts',(2.52271833705488,-0.0725650432881702,
100.882005482591));
#31818=CARTESIAN_POINT('Ctrl Pts',(2.52155245773363,0.105600344880335,100.894460344976));
#31819=CARTESIAN_POINT('Ctrl Pts',(2.48892511090094,0.39486921629796,100.914242202577));
#31820=CARTESIAN_POINT('Ctrl Pts',(2.46861013541699,0.506596656144003,100.921783224797));
#31821=CARTESIAN_POINT('Ctrl Pts',(2.43515773256779,0.639021506479516,100.93057865893));
#31822=CARTESIAN_POINT('Ctrl Pts',(2.42918131339852,0.661377254858567,100.932058854489));
#31823=CARTESIAN_POINT('Ctrl Pts',(2.41928518229816,0.696449847755285,100.934374371168));
#31824=CARTESIAN_POINT('Ctrl Pts',(2.41557155146907,0.709223007592049,100.935216261984));
#31825=CARTESIAN_POINT('Ctrl Pts',(2.40842785420372,0.733086807857943,100.936786716888));
#31826=CARTESIAN_POINT('Ctrl Pts',(2.40502199129611,0.744184268444779,100.937516040346));
#31827=CARTESIAN_POINT('Ctrl Pts',(2.39722324296314,0.768982421632546,100.939143737769));
#31828=CARTESIAN_POINT('Ctrl Pts',(2.39278939897798,0.782669883859632,100.940040754674));
#31829=CARTESIAN_POINT('Ctrl Pts',(2.38120510360909,0.817412324265511,100.942314527208));
#31830=CARTESIAN_POINT('Ctrl Pts',(2.37389250883944,0.838412224459458,100.943685976889));
#31831=CARTESIAN_POINT('Ctrl Pts',(2.31108835374086,1.01135691993694,100.954963047209));
#31832=CARTESIAN_POINT('Ctrl Pts',(2.24134704658691,1.15773272525539,100.964361590552));
#31833=CARTESIAN_POINT('Ctrl Pts',(2.0941690288881,1.40272664227861,100.980802937861));
#31834=CARTESIAN_POINT('Ctrl Pts',(2.02254178811072,1.50416328124464,100.987871150068));
#31835=CARTESIAN_POINT('Ctrl Pts',(1.9159036005538,1.63371903738617,100.997793984006));
#31836=CARTESIAN_POINT('Ctrl Pts',(1.88719331809692,1.66680096401974,101.00041607461));
#31837=CARTESIAN_POINT('Ctrl Pts',(1.83880437782748,1.71970441338077,101.004788600888));
#31838=CARTESIAN_POINT('Ctrl Pts',(1.81963215780414,1.7399780085652,101.006509787682));
#31839=CARTESIAN_POINT('Ctrl Pts',(1.79309732213232,1.76711895047295,101.008883862739));
#31840=CARTESIAN_POINT('Ctrl Pts',(1.78602386268772,1.77426777731719,101.009515966861));
#31841=CARTESIAN_POINT('Ctrl Pts',(1.77410636777221,1.786168774638,101.010580085872));
#31842=CARTESIAN_POINT('Ctrl Pts',(1.76928551771567,1.79094417853476,101.011010309415));
#31843=CARTESIAN_POINT('Ctrl Pts',(1.76008578125356,1.79998379171951,101.011831012765));
#31844=CARTESIAN_POINT('Ctrl Pts',(1.75571056606676,1.8042516493297,101.012221190147));
#31845=CARTESIAN_POINT('Ctrl Pts',(1.745267702285,1.81436431733466,101.01315206251));
#31846=CARTESIAN_POINT('Ctrl Pts',(1.73918621542923,1.8201946412156,101.013693835635));
#31847=CARTESIAN_POINT('Ctrl Pts',(1.71753583431571,1.84074330911238,101.015621044044));
#31848=CARTESIAN_POINT('Ctrl Pts',(1.70180893731338,1.85529284519244,101.017018190788));
#31849=CARTESIAN_POINT('Ctrl Pts',(1.58893400648367,1.95707489480401,101.027014245241));
#31850=CARTESIAN_POINT('Ctrl Pts',(1.4853230278282,2.03682657618432,101.036016252602));
#31851=CARTESIAN_POINT('Ctrl Pts',(1.21961451622876,2.21025457964653,101.05793576285));
#31852=CARTESIAN_POINT('Ctrl Pts',(1.05232100302387,2.29463030545178,101.070765283594));
#31853=CARTESIAN_POINT('Ctrl Pts',(0.841749979897506,2.3729084213946,101.085419390914));
#31854=CARTESIAN_POINT('Ctrl Pts',(0.805996154787807,2.38528988948957,101.087861499123));
#31855=CARTESIAN_POINT('Ctrl Pts',(0.754622327257322,2.40179337757583,101.091307075695));
#31856=CARTESIAN_POINT('Ctrl Pts',(0.739222139259993,2.40657784705255,101.092331943959));
#31857=CARTESIAN_POINT('Ctrl Pts',(0.712441143248606,2.41461672758033,101.094100657476));
#31858=CARTESIAN_POINT('Ctrl Pts',(0.701081534144246,2.41793941485759,101.094846695066));
#31859=CARTESIAN_POINT('Ctrl Pts',(0.677731263547966,2.42459098138732,101.096371803482));
#31860=CARTESIAN_POINT('Ctrl Pts',(0.665738491730634,2.42791131677277,101.097150580848));
#31861=CARTESIAN_POINT('Ctrl Pts',(0.635191156459858,2.43612533393225,101.099123051274));
#31862=CARTESIAN_POINT('Ctrl Pts',(0.616604146978061,2.44089610706203,101.100312783088));
#31863=CARTESIAN_POINT('Ctrl Pts',(0.54442695384488,2.45854492113576,101.104894294869));
#31864=CARTESIAN_POINT('Ctrl Pts',(0.490471830884562,2.46987487344048,101.108237006871));
#31865=CARTESIAN_POINT('Ctrl Pts',(0.251030773908175,2.51199779071189,101.122780074389));
#31866=CARTESIAN_POINT('Ctrl Pts',(0.0628150882582449,2.52372867381365,
101.133397622241));
#31867=CARTESIAN_POINT('Ctrl Pts',(-0.240441823326435,2.5086576842004,101.15095578306));
#31868=CARTESIAN_POINT('Ctrl Pts',(-0.355378645883619,2.49496989932756,
101.15773259091));
#31869=CARTESIAN_POINT('Ctrl Pts',(-0.483649517092121,2.47065035617073,
101.165826760622));
#31870=CARTESIAN_POINT('Ctrl Pts',(-0.498321681213659,2.46773286938623,
101.166760628198));
#31871=CARTESIAN_POINT('Ctrl Pts',(-0.520650675099819,2.46308561115013,
101.168195298953));
#31872=CARTESIAN_POINT('Ctrl Pts',(-0.528327149139011,2.46145044087237,
101.168690957622));
#31873=CARTESIAN_POINT('Ctrl Pts',(-0.542353770502052,2.45839398424644,
101.169601300505));
#31874=CARTESIAN_POINT('Ctrl Pts',(-0.548706183004426,2.4569839470671,101.170015349237));
#31875=CARTESIAN_POINT('Ctrl Pts',(-0.563017731495372,2.45374896042638,
101.170952166158));
#31876=CARTESIAN_POINT('Ctrl Pts',(-0.570973438404357,2.45190991982809,
101.171475708719));
#31877=CARTESIAN_POINT('Ctrl Pts',(-0.591481206634859,2.44706412415595,
101.172832178246));
#31878=CARTESIAN_POINT('Ctrl Pts',(-0.604019169467984,2.44399952372491,
101.173668190619));
#31879=CARTESIAN_POINT('Ctrl Pts',(-0.686812521720767,2.42308670865737,
101.179230644361));
#31880=CARTESIAN_POINT('Ctrl Pts',(-0.756286362660291,2.40230921071231,
101.184097665248));
#31881=CARTESIAN_POINT('Ctrl Pts',(-0.969798124340045,2.32827471894551,
101.199493395555));
#31882=CARTESIAN_POINT('Ctrl Pts',(-1.10993300101494,2.26482286205766,101.210215688445));
#31883=CARTESIAN_POINT('Ctrl Pts',(-1.31581021125568,2.14787830702839,101.226371104731));
#31884=CARTESIAN_POINT('Ctrl Pts',(-1.38612282166367,2.10318888260151,101.231974675893));
#31885=CARTESIAN_POINT('Ctrl Pts',(-1.48280787509193,2.03477862282894,101.239780825843));
#31886=CARTESIAN_POINT('Ctrl Pts',(-1.51109087144459,2.01386390196833,101.242077806613));
#31887=CARTESIAN_POINT('Ctrl Pts',(-1.56074624829605,1.97550942366426,101.246135609531));
#31888=CARTESIAN_POINT('Ctrl Pts',(-1.58228735581412,1.95829853618454,101.247904731141));
#31889=CARTESIAN_POINT('Ctrl Pts',(-1.61451317864024,1.93167181019443,101.250565825627));
#31890=CARTESIAN_POINT('Ctrl Pts',(-1.62540735345955,1.92251391026502,101.251468009934));
#31891=CARTESIAN_POINT('Ctrl Pts',(-1.64503775469752,1.90572598983213,101.253098620193));
#31892=CARTESIAN_POINT('Ctrl Pts',(-1.65379995978832,1.89812709346959,101.253828282061));
#31893=CARTESIAN_POINT('Ctrl Pts',(-1.67258595652183,1.88160636930958,101.255396798162));
#31894=CARTESIAN_POINT('Ctrl Pts',(-1.68259159484296,1.87266437115923,101.256234789241));
#31895=CARTESIAN_POINT('Ctrl Pts',(-1.70959656273743,1.84813896429857,101.258503972631));
#31896=CARTESIAN_POINT('Ctrl Pts',(-1.72645429793493,1.83240106147024,101.259928660132));
#31897=CARTESIAN_POINT('Ctrl Pts',(-1.8164306964207,1.74605750913695,101.267582286731));
#31898=CARTESIAN_POINT('Ctrl Pts',(-1.88544308284351,1.67130044129759,101.273627577863));
#31899=CARTESIAN_POINT('Ctrl Pts',(-2.05555084997692,1.46304051714021,101.289331741976));
#31900=CARTESIAN_POINT('Ctrl Pts',(-2.14817370866746,1.32330005985822,101.298747639354));
#31901=CARTESIAN_POINT('Ctrl Pts',(-2.26509091513141,1.10185672581284,101.313408050624));
#31902=CARTESIAN_POINT('Ctrl Pts',(-2.30025380543939,1.02642806158329,101.318367374668));
#31903=CARTESIAN_POINT('Ctrl Pts',(-2.33694414465476,0.936321486141466,
101.324407073096));
#31904=CARTESIAN_POINT('Ctrl Pts',(-2.34216188340931,0.923192044570125,
101.325289923329));
#31905=CARTESIAN_POINT('Ctrl Pts',(-2.35004248008801,0.902865147073397,
101.326662084427));
#31906=CARTESIAN_POINT('Ctrl Pts',(-2.35278349490963,0.895698026344049,
101.327146916219));
#31907=CARTESIAN_POINT('Ctrl Pts',(-2.35748940257802,0.88322251231285,101.327992793097));
#31908=CARTESIAN_POINT('Ctrl Pts',(-2.35946921738775,0.877919870664267,
101.328352947803));
#31909=CARTESIAN_POINT('Ctrl Pts',(-2.3614311210104,0.872610629504102,101.328714168996));
#31910=CARTESIAN_POINT('Origin',(0.,0.,104.));
#31911=CARTESIAN_POINT('',(-2.36143111379333,0.872610649034711,102.332358906943));
#31912=CARTESIAN_POINT('',(-2.36143112101026,0.872610629504504,102.056173744947));
#31913=CARTESIAN_POINT('',(-2.36143112101026,0.872610629504505,104.));
#31914=CARTESIAN_POINT('',(-2.51749968849485,-0.00125236908425632,101.112583302546));
#31915=CARTESIAN_POINT('Ctrl Pts',(-2.36143112101026,0.872610629504504,
102.056173744947));
#31916=CARTESIAN_POINT('Ctrl Pts',(-2.33295402998363,0.949674427162242,
102.050996882856));
#31917=CARTESIAN_POINT('Ctrl Pts',(-2.30069008088684,1.02537084001563,102.045820020765));
#31918=CARTESIAN_POINT('Ctrl Pts',(-2.26480387283096,1.0993041742893,102.040643158674));
#31919=CARTESIAN_POINT('Ctrl Pts',(-2.22891712097872,1.17323862890085,102.035466218136));
#31920=CARTESIAN_POINT('Ctrl Pts',(-2.18940820972554,1.245409527097,102.030289277598));
#31921=CARTESIAN_POINT('Ctrl Pts',(-2.14648851258624,1.31544415135547,102.02511233706));
#31922=CARTESIAN_POINT('Ctrl Pts',(-2.10352677109179,1.38554738189058,102.019930325165));
#31923=CARTESIAN_POINT('Ctrl Pts',(-2.05714782123045,1.45350975648183,102.014748313269));
#31924=CARTESIAN_POINT('Ctrl Pts',(-2.00760697580321,1.51898666245174,102.009566301374));
#31925=CARTESIAN_POINT('Ctrl Pts',(-1.95804034278516,1.58449765124048,102.004381592076));
#31926=CARTESIAN_POINT('Ctrl Pts',(-1.90530884315185,1.64752023431275,101.999196882778));
#31927=CARTESIAN_POINT('Ctrl Pts',(-1.84970712889199,1.70774406376545,101.99401217348));
#31928=CARTESIAN_POINT('Ctrl Pts',(-1.79401193718764,1.76806914134962,101.988818747664));
#31929=CARTESIAN_POINT('Ctrl Pts',(-1.73543723557534,1.82558574091428,101.983625321847));
#31930=CARTESIAN_POINT('Ctrl Pts',(-1.67431308288007,1.88002179521851,101.978431896031));
#31931=CARTESIAN_POINT('Ctrl Pts',(-1.63429688170024,1.91565949332018,101.975031911522));
#31932=CARTESIAN_POINT('Ctrl Pts',(-1.59318868582522,1.9499777175966,101.971631927013));
#31933=CARTESIAN_POINT('Ctrl Pts',(-1.55108776789116,1.98291023152799,101.968231942504));
#31934=CARTESIAN_POINT('Ctrl Pts',(-1.48601369963049,2.03381298530937,101.962976693097));
#31935=CARTESIAN_POINT('Ctrl Pts',(-1.41831105347741,2.08160300135602,101.957721443689));
#31936=CARTESIAN_POINT('Ctrl Pts',(-1.34830995266693,2.12599777082181,101.952466194282));
#31937=CARTESIAN_POINT('Ctrl Pts',(-1.27840809751515,2.17032959858972,101.947218395625));
#31938=CARTESIAN_POINT('Ctrl Pts',(-1.20621464682185,2.21127549610306,101.941970596967));
#31939=CARTESIAN_POINT('Ctrl Pts',(-1.13209187433468,2.24859383572609,101.93672279831));
#31940=CARTESIAN_POINT('Ctrl Pts',(-1.05743201845937,2.28618257889195,101.931436974827));
#31941=CARTESIAN_POINT('Ctrl Pts',(-0.98081513687593,2.32009068081068,101.926151151344));
#31942=CARTESIAN_POINT('Ctrl Pts',(-0.90264026929864,2.3501163363205,101.920865327861));
#31943=CARTESIAN_POINT('Ctrl Pts',(-0.825166390362852,2.37987275384989,
101.915626901992));
#31944=CARTESIAN_POINT('Ctrl Pts',(-0.746162792910464,2.40581590487025,
101.910388476124));
#31945=CARTESIAN_POINT('Ctrl Pts',(-0.666039924684604,2.42779675193912,
101.905150050255));
#31946=CARTESIAN_POINT('Ctrl Pts',(-0.585943407536667,2.4497703698732,101.899913347218));
#31947=CARTESIAN_POINT('Ctrl Pts',(-0.504728795329403,2.46778414997604,
101.89467664418));
#31948=CARTESIAN_POINT('Ctrl Pts',(-0.422821641415984,2.48173892856406,
101.889439941143));
#31949=CARTESIAN_POINT('Ctrl Pts',(-0.340916718612409,2.4956933270309,101.88420338075));
#31950=CARTESIAN_POINT('Ctrl Pts',(-0.258319746649519,2.50558886733435,
101.878966820358));
#31951=CARTESIAN_POINT('Ctrl Pts',(-0.175465040666476,2.51137776320169,
101.873730259966));
#31952=CARTESIAN_POINT('Ctrl Pts',(-0.0912542264866104,2.51726140769004,
101.868407991195));
#31953=CARTESIAN_POINT('Ctrl Pts',(-0.00677765496019131,2.51890271813326,
101.863085722425));
#31954=CARTESIAN_POINT('Ctrl Pts',(0.0775066867450106,2.51630661158568,
101.857763453654));
#31955=CARTESIAN_POINT('Ctrl Pts',(0.160552829837627,2.51374864374169,101.852519372904));
#31956=CARTESIAN_POINT('Ctrl Pts',(0.243411892025474,2.50707703272406,101.847275292154));
#31957=CARTESIAN_POINT('Ctrl Pts',(0.325650897274851,2.496348882489,101.842031211403));
#31958=CARTESIAN_POINT('Ctrl Pts',(0.409729149087786,2.48538080092947,101.836669848623));
#31959=CARTESIAN_POINT('Ctrl Pts',(0.493158770837792,2.47017263631202,101.831308485842));
#31960=CARTESIAN_POINT('Ctrl Pts',(0.575490003805824,2.45084016319294,101.825947123061));
#31961=CARTESIAN_POINT('Ctrl Pts',(0.657821236773869,2.43150769007384,101.820585760281));
#31962=CARTESIAN_POINT('Ctrl Pts',(0.739053611328975,2.40805111359022,101.8152243975));
#31963=CARTESIAN_POINT('Ctrl Pts',(0.818757647879658,2.38063902430389,101.80986303472));
#31964=CARTESIAN_POINT('Ctrl Pts',(0.896884163093645,2.35376948163883,101.804607785312));
#31965=CARTESIAN_POINT('Ctrl Pts',(0.973830871246779,2.32300037319785,101.799352535905));
#31966=CARTESIAN_POINT('Ctrl Pts',(1.04918106998779,2.28845479142134,101.794097286498));
#31967=CARTESIAN_POINT('Ctrl Pts',(1.12442443926455,2.25395818743195,101.78884948784));
#31968=CARTESIAN_POINT('Ctrl Pts',(1.19807537913545,2.21569593576891,101.783601689183));
#31969=CARTESIAN_POINT('Ctrl Pts',(1.26973397369632,2.17384035431339,101.778353890525));
#31970=CARTESIAN_POINT('Ctrl Pts',(1.3419117965518,2.13168149308644,101.773068067042));
#31971=CARTESIAN_POINT('Ctrl Pts',(1.41206783162646,2.08587716292098,101.767782243559));
#31972=CARTESIAN_POINT('Ctrl Pts',(1.4798155485121,2.03665220211548,101.762496420076));
#31973=CARTESIAN_POINT('Ctrl Pts',(1.54695577629672,1.98786863813576,101.757257994208));
#31974=CARTESIAN_POINT('Ctrl Pts',(1.61173032318653,1.93572581916233,101.752019568339));
#31975=CARTESIAN_POINT('Ctrl Pts',(1.67379070881012,1.88048688192737,101.746781142471));
#31976=CARTESIAN_POINT('Ctrl Pts',(1.73583068380572,1.82526611185956,101.741544439433));
#31977=CARTESIAN_POINT('Ctrl Pts',(1.79515792597834,1.76695155239321,101.736307736395));
#31978=CARTESIAN_POINT('Ctrl Pts',(1.85145756440779,1.70584616457556,101.731071033358));
#31979=CARTESIAN_POINT('Ctrl Pts',(1.90775566926326,1.64474244123812,101.725834472966));
#31980=CARTESIAN_POINT('Ctrl Pts',(1.96102602244972,1.58084838074178,101.720597912573));
#31981=CARTESIAN_POINT('Ctrl Pts',(2.0109920776548,1.51450226596385,101.715361352181));
#31982=CARTESIAN_POINT('Ctrl Pts',(2.06177594249699,1.44707024412706,101.71003908341));
#31983=CARTESIAN_POINT('Ctrl Pts',(2.10914606227315,1.37710556168493,101.70471681464));
#31984=CARTESIAN_POINT('Ctrl Pts',(2.15285720954208,1.3049950518384,101.699394545869));
#31985=CARTESIAN_POINT('Ctrl Pts',(2.19592620809382,1.23394389811238,101.694150465119));
#31986=CARTESIAN_POINT('Ctrl Pts',(2.23544285799687,1.16080998695854,101.688906384369));
#31987=CARTESIAN_POINT('Ctrl Pts',(2.27121932313172,1.08598758567172,101.683662303618));
#31988=CARTESIAN_POINT('Ctrl Pts',(2.30779591638533,1.00949180757261,101.678300940838));
#31989=CARTESIAN_POINT('Ctrl Pts',(2.34046281303112,0.931231575526403,101.672939578057));
#31990=CARTESIAN_POINT('Ctrl Pts',(2.36907225203704,0.85164717731472,101.667578215277));
#31991=CARTESIAN_POINT('Ctrl Pts',(2.39768169104296,0.772062779103038,101.662216852496));
#31992=CARTESIAN_POINT('Ctrl Pts',(2.42223358878513,0.691154720335934,101.656855489715));
#31993=CARTESIAN_POINT('Ctrl Pts',(2.44263552689213,0.609375034575942,101.651494126935));
#31994=CARTESIAN_POINT('Ctrl Pts',(2.46263366496506,0.529213951897807,101.646238877528));
#31995=CARTESIAN_POINT('Ctrl Pts',(2.47871852955357,0.447919357606244,101.64098362812));
#31996=CARTESIAN_POINT('Ctrl Pts',(2.4907664954014,0.365907796290044,101.635728378713));
#31997=CARTESIAN_POINT('Ctrl Pts',(2.50279737997062,0.284012508737074,101.630480580055));
#31998=CARTESIAN_POINT('Ctrl Pts',(2.5108026676466,0.201402725930201,101.625232781398));
#31999=CARTESIAN_POINT('Ctrl Pts',(2.51470916250037,0.118507712983954,101.61998498274));
#32000=CARTESIAN_POINT('Ctrl Pts',(2.51864396327716,0.0350120542048318,
101.614699159258));
#32001=CARTESIAN_POINT('Ctrl Pts',(2.51842020731909,-0.0487725258357472,
101.609413335775));
#32002=CARTESIAN_POINT('Ctrl Pts',(2.51401604017221,-0.132399394850828,
101.604127512292));
#32003=CARTESIAN_POINT('Ctrl Pts',(2.50965136488813,-0.215276387503841,
101.598889086423));
#32004=CARTESIAN_POINT('Ctrl Pts',(2.50118097377524,-0.297998016898339,
101.593650660555));
#32005=CARTESIAN_POINT('Ctrl Pts',(2.48863585321228,-0.380128715182637,
101.588412234686));
#32006=CARTESIAN_POINT('Ctrl Pts',(2.47609485853068,-0.462232402047155,
101.583175531649));
#32007=CARTESIAN_POINT('Ctrl Pts',(2.45948186554945,-0.543745088015556,
101.577938828611));
#32008=CARTESIAN_POINT('Ctrl Pts',(2.4388795636937,-0.624237714174042,101.572702125574));
#32009=CARTESIAN_POINT('Ctrl Pts',(2.41827782303442,-0.704728147753364,
101.567465565181));
#32010=CARTESIAN_POINT('Ctrl Pts',(2.3936871049706,-0.78419813001327,101.562229004789));
#32011=CARTESIAN_POINT('Ctrl Pts',(2.36524059249845,-0.862231517399819,
101.556992444397));
#32012=CARTESIAN_POINT('Ctrl Pts',(2.33632848729637,-0.941542100994302,
101.551670175626));
#32013=CARTESIAN_POINT('Ctrl Pts',(2.30343338708735,-1.01936817258397,101.546347906856));
#32014=CARTESIAN_POINT('Ctrl Pts',(2.26674625011283,-1.09529342534292,101.541025638085));
#32015=CARTESIAN_POINT('Ctrl Pts',(2.23059807400799,-1.17010328061838,101.535781557335));
#32016=CARTESIAN_POINT('Ctrl Pts',(2.19076881527365,-1.24306741378589,101.530537476585));
#32017=CARTESIAN_POINT('Ctrl Pts',(2.14748691460656,-1.31381360991337,101.525293395834));
#32018=CARTESIAN_POINT('Ctrl Pts',(2.10323702938233,-1.38614201995179,101.519932033054));
#32019=CARTESIAN_POINT('Ctrl Pts',(2.0553784933784,-1.45615166634403,101.514570670273));
#32020=CARTESIAN_POINT('Ctrl Pts',(2.00420016786468,-1.52347889290636,101.509209307493));
#32021=CARTESIAN_POINT('Ctrl Pts',(1.95302184235097,-1.59080611946867,101.503847944712));
#32022=CARTESIAN_POINT('Ctrl Pts',(1.89852410590013,-1.65545058077782,101.498486581932));
#32023=CARTESIAN_POINT('Ctrl Pts',(1.84103580345049,-1.71708864663809,101.493125219151));
#32024=CARTESIAN_POINT('Ctrl Pts',(1.78468532321976,-1.77750675717042,101.487869969744));
#32025=CARTESIAN_POINT('Ctrl Pts',(1.72525347433516,-1.83525958626159,101.482614720336));
#32026=CARTESIAN_POINT('Ctrl Pts',(1.66302234322044,-1.89001664964878,101.477359470929));
#32027=CARTESIAN_POINT('Ctrl Pts',(1.6008794417125,-1.94469607995933,101.472111672272));
#32028=CARTESIAN_POINT('Ctrl Pts',(1.53594548458515,-1.99638787870892,101.466863873614));
#32029=CARTESIAN_POINT('Ctrl Pts',(1.46854068446697,-2.0447969356553,101.461616074957));
#32030=CARTESIAN_POINT('Ctrl Pts',(1.40064747846208,-2.09355675795282,101.456330251474));
#32031=CARTESIAN_POINT('Ctrl Pts',(1.33024779482609,-2.13898571857547,101.451044427991));
#32032=CARTESIAN_POINT('Ctrl Pts',(1.25770436658405,-2.18082231653003,101.445758604508));
#32033=CARTESIAN_POINT('Ctrl Pts',(1.18581143025572,-2.22228376859851,101.440520178639));
#32034=CARTESIAN_POINT('Ctrl Pts',(1.11181344803786,-2.26021679013602,101.435281752771));
#32035=CARTESIAN_POINT('Ctrl Pts',(1.03609264146641,-2.29441022668118,101.430043326902));
#32036=CARTESIAN_POINT('Ctrl Pts',(0.960396738207992,-2.32859241757414,
101.424806623865));
#32037=CARTESIAN_POINT('Ctrl Pts',(0.882979556110991,-2.35903727634764,
101.419569920827));
#32038=CARTESIAN_POINT('Ctrl Pts',(0.80424600686878,-2.38558056045811,101.41433321779));
#32039=CARTESIAN_POINT('Ctrl Pts',(0.725514602289,-2.41212312154282,101.409096657397));
#32040=CARTESIAN_POINT('Ctrl Pts',(0.645467339428495,-2.43476417284098,
101.403860097005));
#32041=CARTESIAN_POINT('Ctrl Pts',(0.564525787980021,-2.45338885721476,
101.398623536613));
#32042=CARTESIAN_POINT('Ctrl Pts',(0.482259441517519,-2.4723183774677,101.393301267842));
#32043=CARTESIAN_POINT('Ctrl Pts',(0.399069744422781,-2.4870987473585,101.387978999072));
#32044=CARTESIAN_POINT('Ctrl Pts',(0.31540985916229,-2.49766348228564,101.382656730301));
#32045=CARTESIAN_POINT('Ctrl Pts',(0.232978998792484,-2.50807301353125,
101.377412649551));
#32046=CARTESIAN_POINT('Ctrl Pts',(0.150092144703488,-2.51438997478319,
101.372168568801));
#32047=CARTESIAN_POINT('Ctrl Pts',(0.0671858828026818,-2.51660332733469,
101.36692448805));
#32048=CARTESIAN_POINT('Ctrl Pts',(-0.0175745486229646,-2.51886618074119,
101.36156312527));
#32049=CARTESIAN_POINT('Ctrl Pts',(-0.102354754541292,-2.51683967122694,
101.356201762489));
#32050=CARTESIAN_POINT('Ctrl Pts',(-0.186692431981587,-2.51056810021971,
101.350840399709));
#32051=CARTESIAN_POINT('Ctrl Pts',(-0.271030109421882,-2.50429652921248,
101.345479036928));
#32052=CARTESIAN_POINT('Ctrl Pts',(-0.354924762531309,-2.49378002618988,
101.340117674148));
#32053=CARTESIAN_POINT('Ctrl Pts',(-0.437925892658451,-2.47911822278392,
101.334756311367));
#32054=CARTESIAN_POINT('Ctrl Pts',(-0.519284244585212,-2.46474660929437,
101.32950106196));
#32055=CARTESIAN_POINT('Ctrl Pts',(-0.600084634975024,-2.4463392509089,
101.324245812552));
#32056=CARTESIAN_POINT('Ctrl Pts',(-0.679896273784101,-2.42395282687071,
101.318990563145));
#32057=CARTESIAN_POINT('Ctrl Pts',(-0.759594757820063,-2.40159814169631,
101.313742764488));
#32058=CARTESIAN_POINT('Ctrl Pts',(-0.838306834140659,-2.37527571993368,
101.30849496583));
#32059=CARTESIAN_POINT('Ctrl Pts',(-0.915610626285933,-2.3450934802332,
101.303247167173));
#32060=CARTESIAN_POINT('Ctrl Pts',(-0.993474551049313,-2.31469254418583,
101.29796134369));
#32061=CARTESIAN_POINT('Ctrl Pts',(-1.06990923039576,-2.28037570120002,
101.292675520207));
#32062=CARTESIAN_POINT('Ctrl Pts',(-1.14449782874786,-2.24230483431478,
101.287389696724));
#32063=CARTESIAN_POINT('Ctrl Pts',(-1.21841759628706,-2.20457534626504,
101.282151270855));
#32064=CARTESIAN_POINT('Ctrl Pts',(-1.29052383903869,-2.16315910245258,
101.276912844987));
#32065=CARTESIAN_POINT('Ctrl Pts',(-1.36043134115765,-2.11826174397688,
101.271674419118));
#32066=CARTESIAN_POINT('Ctrl Pts',(-1.43031585186252,-2.07337915149524,
101.266437716081));
#32067=CARTESIAN_POINT('Ctrl Pts',(-1.49800267016906,-2.02501796729658,
101.261201013043));
#32068=CARTESIAN_POINT('Ctrl Pts',(-1.56313357589532,-1.97342840607627,
101.255964310006));
#32069=CARTESIAN_POINT('Ctrl Pts',(-1.62826270748839,-1.92184025012971,
101.250727749613));
#32070=CARTESIAN_POINT('Ctrl Pts',(-1.69083570386698,-1.86702417931519,
101.245491189221));
#32071=CARTESIAN_POINT('Ctrl Pts',(-1.75052669947269,-1.80927126889067,
101.240254628829));
#32072=CARTESIAN_POINT('Ctrl Pts',(-1.8111946757756,-1.75057309899913,101.234932360058));
#32073=CARTESIAN_POINT('Ctrl Pts',(-1.86888509645779,-1.6888414183291,101.229610091288));
#32074=CARTESIAN_POINT('Ctrl Pts',(-1.92329546973613,-1.62442013841631,
101.224287822517));
#32075=CARTESIAN_POINT('Ctrl Pts',(-1.9769065148435,-1.56094525421343,101.219043741767));
#32076=CARTESIAN_POINT('Ctrl Pts',(-2.02733301030583,-1.49485967987507,
101.213799661017));
#32077=CARTESIAN_POINT('Ctrl Pts',(-2.07432799706226,-1.42652361025105,
101.208555580266));
#32078=CARTESIAN_POINT('Ctrl Pts',(-2.12237401024619,-1.35665922835195,
101.203194217486));
#32079=CARTESIAN_POINT('Ctrl Pts',(-2.16683290515724,-1.28444290942289,
101.197832854705));
#32080=CARTESIAN_POINT('Ctrl Pts',(-2.20749013991719,-1.21028654961061,
101.192471491925));
#32081=CARTESIAN_POINT('Ctrl Pts',(-2.24814737467715,-1.13613018979832,
101.187110129144));
#32082=CARTESIAN_POINT('Ctrl Pts',(-2.28500278792296,-1.06003427551463,
101.181748766363));
#32083=CARTESIAN_POINT('Ctrl Pts',(-2.3178946752049,-0.982430926150415,
101.176387403583));
#32084=CARTESIAN_POINT('Ctrl Pts',(-2.35361447071378,-0.898155562248903,
101.170565093038));
#32085=CARTESIAN_POINT('Ctrl Pts',(-2.38477328167377,-0.811838041542081,
101.164742782493));
#32086=CARTESIAN_POINT('Ctrl Pts',(-2.41115846466788,-0.723962090347565,
101.158920471948));
#32087=CARTESIAN_POINT('Ctrl Pts',(-2.4374644137324,-0.636350028053568,
101.15311564563));
#32088=CARTESIAN_POINT('Ctrl Pts',(-2.45902521036231,-0.547189130622515,
101.147310819312));
#32089=CARTESIAN_POINT('Ctrl Pts',(-2.47567650290214,-0.456981512731327,
101.141505992995));
#32090=CARTESIAN_POINT('Ctrl Pts',(-2.49224191268966,-0.367239160733822,
101.135731106363));
#32091=CARTESIAN_POINT('Ctrl Pts',(-2.50394821153258,-0.276461124818012,
101.129956219731));
#32092=CARTESIAN_POINT('Ctrl Pts',(-2.51068155182442,-0.18516045832883,
101.124181333099));
#32093=CARTESIAN_POINT('Ctrl Pts',(-2.51518920085722,-0.12403903223759,
101.120315322914));
#32094=CARTESIAN_POINT('Ctrl Pts',(-2.51746912850001,-0.0626837621585557,
101.11644931273));
#32095=CARTESIAN_POINT('Ctrl Pts',(-2.51749968849485,-0.00125236908424377,
101.112583302546));
#32096=CARTESIAN_POINT('Ctrl Pts',(-2.51749968849528,-0.00125236822532715,
101.112583302492));
#32097=CARTESIAN_POINT('Ctrl Pts',(-2.51754167409677,0.083146721867559,
101.107271885552));
#32098=CARTESIAN_POINT('Ctrl Pts',(-2.51333509775226,0.167540685368797,
101.101960468612));
#32099=CARTESIAN_POINT('Ctrl Pts',(-2.50490792305447,0.251480709039413,
101.096649051672));
#32100=CARTESIAN_POINT('Ctrl Pts',(-2.49647888961856,0.335439246924613,
101.09133646322));
#32101=CARTESIAN_POINT('Ctrl Pts',(-2.48382745953182,0.418943205939949,
101.086023874768));
#32102=CARTESIAN_POINT('Ctrl Pts',(-2.46703330865219,0.501550499950555,
101.080711286317));
#32103=CARTESIAN_POINT('Ctrl Pts',(-2.45022206899961,0.584241850446145,
101.075393292077));
#32104=CARTESIAN_POINT('Ctrl Pts',(-2.42925979038389,0.666034281971585,
101.070075297837));
#32105=CARTESIAN_POINT('Ctrl Pts',(-2.4042768382142,0.746497913745721,101.064757303598));
#32106=CARTESIAN_POINT('Ctrl Pts',(-2.39110377033219,0.788924960645322,
101.061953219491));
#32107=CARTESIAN_POINT('Ctrl Pts',(-2.37681368205517,0.830982832244095,
101.059149135384));
#32108=CARTESIAN_POINT('Ctrl Pts',(-2.36143112101025,0.872610629504513,
101.056345051278));
#32109=CARTESIAN_POINT('Ctrl Pts',(-2.3614311210104,0.872610629504102,101.328714168996));
#32110=CARTESIAN_POINT('Ctrl Pts',(-2.36172918736716,0.87180401181328,101.32876904829));
#32111=CARTESIAN_POINT('Ctrl Pts',(-2.36202684029789,0.870997241779622,
101.32882395201));
#32112=CARTESIAN_POINT('Ctrl Pts',(-2.36522277224922,0.862321177659682,
101.329414540597));
#32113=CARTESIAN_POINT('Ctrl Pts',(-2.36808207781547,0.854437735427849,
101.329952500584));
#32114=CARTESIAN_POINT('Ctrl Pts',(-2.37548955523205,0.833691644041302,
101.33137140068));
#32115=CARTESIAN_POINT('Ctrl Pts',(-2.37997257734536,0.820806247606163,
101.332255900535));
#32116=CARTESIAN_POINT('Ctrl Pts',(-2.41665618100022,0.712540185518066,
101.339710875365));
#32117=CARTESIAN_POINT('Ctrl Pts',(-2.44321033835195,0.61535305269985,101.346550076335));
#32118=CARTESIAN_POINT('Ctrl Pts',(-2.49940153361352,0.347484055687169,
101.365365167741));
#32119=CARTESIAN_POINT('Ctrl Pts',(-2.51737555155781,0.174885346556131,
101.377416472145));
#32120=CARTESIAN_POINT('Ctrl Pts',(-2.51755617191668,-0.0776304462386804,
101.394332960011));
#32121=CARTESIAN_POINT('Ctrl Pts',(-2.51385374182857,-0.157026032853185,
101.399556554048));
#32122=CARTESIAN_POINT('Ctrl Pts',(-2.50435559508939,-0.257847910187009,
101.406068721468));
#32123=CARTESIAN_POINT('Ctrl Pts',(-2.50202630676959,-0.279547671549114,
101.407463286211));
#32124=CARTESIAN_POINT('Ctrl Pts',(-2.49785775514308,-0.314137389021349,
101.40967556161));
#32125=CARTESIAN_POINT('Ctrl Pts',(-2.49620020432483,-0.327047724918777,
101.410498895477));
#32126=CARTESIAN_POINT('Ctrl Pts',(-2.49286963686515,-0.351486718145176,
101.412053127542));
#32127=CARTESIAN_POINT('Ctrl Pts',(-2.4912165884664,-0.363017707715161,
101.412784628888));
#32128=CARTESIAN_POINT('Ctrl Pts',(-2.48727744870282,-0.389200500062406,
101.414441645585));
#32129=CARTESIAN_POINT('Ctrl Pts',(-2.48494180482339,-0.403844496752386,
101.415365582878));
#32130=CARTESIAN_POINT('Ctrl Pts',(-2.47739135894408,-0.44863607148298,
101.418183580184));
#32131=CARTESIAN_POINT('Ctrl Pts',(-2.47175616434693,-0.478710620372423,
101.420064440261));
#32132=CARTESIAN_POINT('Ctrl Pts',(-2.4417557181073,-0.624124042715217,
101.429114724524));
#32133=CARTESIAN_POINT('Ctrl Pts',(-2.40985715131089,-0.737763463489458,
101.436043690325));
#32134=CARTESIAN_POINT('Ctrl Pts',(-2.30850872053919,-1.02077256024703,
101.453445916921));
#32135=CARTESIAN_POINT('Ctrl Pts',(-2.22837341446319,-1.1855497579761,101.463702586228));
#32136=CARTESIAN_POINT('Ctrl Pts',(-2.10829047188926,-1.3765019799792,101.477254844456));
#32137=CARTESIAN_POINT('Ctrl Pts',(-2.08453131581174,-1.41222346464157,
101.479871221915));
#32138=CARTESIAN_POINT('Ctrl Pts',(-2.05285448779753,-1.45730701588315,
101.483302949146));
#32139=CARTESIAN_POINT('Ctrl Pts',(-2.04576364091668,-1.46724449157694,
101.484067706087));
#32140=CARTESIAN_POINT('Ctrl Pts',(-2.03434391142491,-1.48300496984466,
101.4852946045));
#32141=CARTESIAN_POINT('Ctrl Pts',(-2.03006154129942,-1.48886165439053,
101.485753650007));
#32142=CARTESIAN_POINT('Ctrl Pts',(-2.02182807915965,-1.50002039695321,
101.486634429349));
#32143=CARTESIAN_POINT('Ctrl Pts',(-2.01788134988087,-1.50532548861657,
101.48705587088));
#32144=CARTESIAN_POINT('Ctrl Pts',(-2.00843843572285,-1.51791454468206,
101.48806231573));
#32145=CARTESIAN_POINT('Ctrl Pts',(-2.00292349153935,-1.52518424983481,
101.488648594527));
#32146=CARTESIAN_POINT('Ctrl Pts',(-1.98411891016749,-1.54969424217938,
101.49064211295));
#32147=CARTESIAN_POINT('Ctrl Pts',(-1.97064564706049,-1.56679154717359,
101.492061184998));
#32148=CARTESIAN_POINT('Ctrl Pts',(-1.93727145438188,-1.60803121257369,
101.495549793263));
#32149=CARTESIAN_POINT('Ctrl Pts',(-1.91713922736513,-1.63198102623633,
101.497632072998));
#32150=CARTESIAN_POINT('Ctrl Pts',(-1.83396174471256,-1.72726768161193,
101.506127287737));
#32151=CARTESIAN_POINT('Ctrl Pts',(-1.76734236855021,-1.79537410662982,
101.512686630651));
#32152=CARTESIAN_POINT('Ctrl Pts',(-1.54888968240569,-1.9947357411201,101.533114330001));
#32153=CARTESIAN_POINT('Ctrl Pts',(-1.38509360214154,-2.11177056368132,
101.546896691837));
#32154=CARTESIAN_POINT('Ctrl Pts',(-1.18159057604464,-2.22320374128811,
101.561952462386));
#32155=CARTESIAN_POINT('Ctrl Pts',(-1.15378344491456,-2.23776117406832,
101.563971101042));
#32156=CARTESIAN_POINT('Ctrl Pts',(-1.11231236310428,-2.25849326398709,
101.566926417194));
#32157=CARTESIAN_POINT('Ctrl Pts',(-1.0988546673236,-2.26507153363681,101.567877012767));
#32158=CARTESIAN_POINT('Ctrl Pts',(-1.07481286846283,-2.27655872698203,
101.569560553352));
#32159=CARTESIAN_POINT('Ctrl Pts',(-1.06425194631923,-2.28151487870729,
101.570295107451));
#32160=CARTESIAN_POINT('Ctrl Pts',(-1.04191223017021,-2.29180984882758,
101.571838628463));
#32161=CARTESIAN_POINT('Ctrl Pts',(-1.03012595204267,-2.29713169222341,
101.57264699892));
#32162=CARTESIAN_POINT('Ctrl Pts',(-0.998694193774606,-2.31103346814054,
101.574787272472));
#32163=CARTESIAN_POINT('Ctrl Pts',(-0.978978975170113,-2.31945381363046,
101.576113760895));
#32164=CARTESIAN_POINT('Ctrl Pts',(-0.880682351119668,-2.35995954239794,
101.582652075516));
#32165=CARTESIAN_POINT('Ctrl Pts',(-0.800616476209311,-2.38831026217681,
101.587738382793));
#32166=CARTESIAN_POINT('Ctrl Pts',(-0.53273968207224,-2.46817311667891,
101.604193756111));
#32167=CARTESIAN_POINT('Ctrl Pts',(-0.340408869308689,-2.50196042748617,
101.615080348334));
#32168=CARTESIAN_POINT('Ctrl Pts',(-0.0706608672599164,-2.51764290021729,
101.630953348771));
#32169=CARTESIAN_POINT('Ctrl Pts',(0.00494464605481614,-2.518628991865,
101.635474852003));
#32170=CARTESIAN_POINT('Ctrl Pts',(0.0934973024873506,-2.51579695911163,
101.640972057355));
#32171=CARTESIAN_POINT('Ctrl Pts',(0.106518970630747,-2.51527926427425,
101.641785548451));
#32172=CARTESIAN_POINT('Ctrl Pts',(0.127729731795672,-2.51427099957564,
101.643119835508));
#32173=CARTESIAN_POINT('Ctrl Pts',(0.135921663376561,-2.51384145097431,
101.643637397917));
#32174=CARTESIAN_POINT('Ctrl Pts',(0.150609338600618,-2.5129992919997,101.644569609295));
#32175=CARTESIAN_POINT('Ctrl Pts',(0.157105756180925,-2.51260151914006,
101.644983435099));
#32176=CARTESIAN_POINT('Ctrl Pts',(0.171400691760376,-2.51167058975998,
101.645897384837));
#32177=CARTESIAN_POINT('Ctrl Pts',(0.179198195729925,-2.51112631130291,
101.646398095255));
#32178=CARTESIAN_POINT('Ctrl Pts',(0.201757361004582,-2.5094460375886,101.647852766465));
#32179=CARTESIAN_POINT('Ctrl Pts',(0.21651140642045,-2.50821614584709,101.648811649398));
#32180=CARTESIAN_POINT('Ctrl Pts',(0.338067315599042,-2.49700281527279,
101.656768964609));
#32181=CARTESIAN_POINT('Ctrl Pts',(0.444130892964582,-2.48033367283814,
101.664072657662));
#32182=CARTESIAN_POINT('Ctrl Pts',(0.711067452958561,-2.42070969192047,
101.682898692485));
#32183=CARTESIAN_POINT('Ctrl Pts',(0.869368700839968,-2.36847221888829,
101.694460466903));
#32184=CARTESIAN_POINT('Ctrl Pts',(1.09454319307913,-2.26852173666696,101.710969828079));
#32185=CARTESIAN_POINT('Ctrl Pts',(1.16613199664307,-2.23256671433604,101.716235893064));
#32186=CARTESIAN_POINT('Ctrl Pts',(1.25494705283373,-2.18251976536889,101.722791932291));
#32187=CARTESIAN_POINT('Ctrl Pts',(1.27386171536046,-2.17153425280453,101.724189682161));
#32188=CARTESIAN_POINT('Ctrl Pts',(1.30380961784052,-2.15361473400303,101.726405802222));
#32189=CARTESIAN_POINT('Ctrl Pts',(1.31493600915743,-2.14683936154327,101.727229829755));
#32190=CARTESIAN_POINT('Ctrl Pts',(1.33590956352097,-2.13384337083717,101.728784639368));
#32191=CARTESIAN_POINT('Ctrl Pts',(1.34576708713398,-2.12764020635169,101.729516030584));
#32192=CARTESIAN_POINT('Ctrl Pts',(1.36806117869079,-2.11339400127814,101.731171810828));
#32193=CARTESIAN_POINT('Ctrl Pts',(1.38047060334552,-2.1053091272699,101.732094630978));
#32194=CARTESIAN_POINT('Ctrl Pts',(1.4182143928178,-2.08024142402063,101.734905665642));
#32195=CARTESIAN_POINT('Ctrl Pts',(1.44331267452209,-2.06290695201871,101.73678077715));
#32196=CARTESIAN_POINT('Ctrl Pts',(1.56324554824217,-1.97681307029793,101.745780547244));
#32197=CARTESIAN_POINT('Ctrl Pts',(1.65352296875486,-1.90194450478809,101.752667972112));
#32198=CARTESIAN_POINT('Ctrl Pts',(1.87087562321093,-1.69447290384077,101.770066608593));
#32199=CARTESIAN_POINT('Ctrl Pts',(1.9892475516853,-1.55380028613859,101.780355127044));
#32200=CARTESIAN_POINT('Ctrl Pts',(2.11530275363044,-1.36570904831162,101.793955891469));
#32201=CARTESIAN_POINT('Ctrl Pts',(2.1383907588902,-1.3292672435408,101.796586418493));
#32202=CARTESIAN_POINT('Ctrl Pts',(2.16680766557815,-1.28175675262042,101.800034256593));
#32203=CARTESIAN_POINT('Ctrl Pts',(2.17300890448883,-1.27121521363664,101.800800389005));
#32204=CARTESIAN_POINT('Ctrl Pts',(2.18276851790485,-1.2543446732966,101.802028981774));
#32205=CARTESIAN_POINT('Ctrl Pts',(2.18637683743974,-1.24804458403013,101.8024883313));
#32206=CARTESIAN_POINT('Ctrl Pts',(2.19321837662858,-1.23597860081223,101.803369296461));
#32207=CARTESIAN_POINT('Ctrl Pts',(2.19645619243537,-1.23021548514261,101.803790616648));
#32208=CARTESIAN_POINT('Ctrl Pts',(2.20410387926704,-1.21647663338506,101.804796211397));
#32209=CARTESIAN_POINT('Ctrl Pts',(2.20849318307504,-1.20848962112337,101.805381755583));
#32210=CARTESIAN_POINT('Ctrl Pts',(2.22318708358302,-1.18140440554198,101.807370167952));
#32211=CARTESIAN_POINT('Ctrl Pts',(2.23328775291323,-1.16219745139941,101.808784788955));
#32212=CARTESIAN_POINT('Ctrl Pts',(2.29188988975984,-1.0471769328964,101.817272767998));
#32213=CARTESIAN_POINT('Ctrl Pts',(2.33446419818119,-0.948478350966228,
101.824619422664));
#32214=CARTESIAN_POINT('Ctrl Pts',(2.43567639175228,-0.665328501455818,
101.845352659632));
#32215=CARTESIAN_POINT('Ctrl Pts',(2.47957350143165,-0.476360166230241,
101.858745741571));
#32216=CARTESIAN_POINT('Ctrl Pts',(2.50698160996559,-0.23513613647249,101.874724462154));
#32217=CARTESIAN_POINT('Ctrl Pts',(2.51111250586123,-0.185904105703202,
101.877933024791));
#32218=CARTESIAN_POINT('Ctrl Pts',(2.5147912768141,-0.118195043006874,101.882276357249));
#32219=CARTESIAN_POINT('Ctrl Pts',(2.51558845086623,-0.0997998467113807,
101.883449381315));
#32220=CARTESIAN_POINT('Ctrl Pts',(2.51654109464776,-0.0703513128390186,
101.885316482728));
#32221=CARTESIAN_POINT('Ctrl Pts',(2.51682568664899,-0.0593030994945107,
101.886014540997));
#32222=CARTESIAN_POINT('Ctrl Pts',(2.51726322565758,-0.0364797112806158,
101.887451719616));
#32223=CARTESIAN_POINT('Ctrl Pts',(2.51740632533036,-0.0247046013295393,
101.88819051691));
#32224=CARTESIAN_POINT('Ctrl Pts',(2.51754775425828,0.00283420997172765,
101.889912318829));
#32225=CARTESIAN_POINT('Ctrl Pts',(2.51748065830297,0.0185978641871937,
101.890893272061));
#32226=CARTESIAN_POINT('Ctrl Pts',(2.51677818651749,0.0700618057000397,
101.894081507818));
#32227=CARTESIAN_POINT('Ctrl Pts',(2.51553138671735,0.105750335333389,101.896269895965));
#32228=CARTESIAN_POINT('Ctrl Pts',(2.5107664008115,0.19045169630388,101.901418908085));
#32229=CARTESIAN_POINT('Ctrl Pts',(2.50657174313088,0.239412390919124,101.90435937046));
#32230=CARTESIAN_POINT('Ctrl Pts',(2.48429458526032,0.432715221182628,101.915877200006));
#32231=CARTESIAN_POINT('Ctrl Pts',(2.45515175006029,0.575494889199207,101.924163957067));
#32232=CARTESIAN_POINT('Ctrl Pts',(2.40050256925057,0.759999869101461,101.935243793087));
#32233=CARTESIAN_POINT('Ctrl Pts',(2.38590588137352,0.80465229124762,101.937957072073));
#32234=CARTESIAN_POINT('Ctrl Pts',(2.33998842558295,0.932855257071136,101.945903207168));
#32235=CARTESIAN_POINT('Ctrl Pts',(2.30546799976501,1.01517414679257,101.951200755784));
#32236=CARTESIAN_POINT('Ctrl Pts',(2.26077090167604,1.10765705734199,101.957568574702));
#32237=CARTESIAN_POINT('Ctrl Pts',(2.25478682874172,1.11978817860489,101.958412392653));
#32238=CARTESIAN_POINT('Ctrl Pts',(2.24495060009248,1.13932997879792,101.959786495274));
#32239=CARTESIAN_POINT('Ctrl Pts',(2.24115872768089,1.14677092309987,101.960313218542));
#32240=CARTESIAN_POINT('Ctrl Pts',(2.23434183455633,1.15998504131652,101.961255109214));
#32241=CARTESIAN_POINT('Ctrl Pts',(2.2313313294498,1.1657655108954,101.961669376467));
#32242=CARTESIAN_POINT('Ctrl Pts',(2.22471559754283,1.17834885922855,101.962576136081));
#32243=CARTESIAN_POINT('Ctrl Pts',(2.22110165356873,1.18514681147389,101.963069149946));
#32244=CARTESIAN_POINT('Ctrl Pts',(2.21071077874187,1.2044779413438,101.964479893279));
#32245=CARTESIAN_POINT('Ctrl Pts',(2.20385867773175,1.21697007552952,101.965402110189));
#32246=CARTESIAN_POINT('Ctrl Pts',(2.15462284931333,1.30495281456214,101.971968880341));
#32247=CARTESIAN_POINT('Ctrl Pts',(2.10847983104193,1.37826379468537,101.97781401008));
#32248=CARTESIAN_POINT('Ctrl Pts',(1.95902734123117,1.59059108685737,101.995589684895));
#32249=CARTESIAN_POINT('Ctrl Pts',(1.84505144901853,1.72149991230264,102.007682034587));
#32250=CARTESIAN_POINT('Ctrl Pts',(1.65049431142722,1.90324624530085,102.025634751009));
#32251=CARTESIAN_POINT('Ctrl Pts',(1.5789650858613,1.96299530129438,102.031788447827));
#32252=CARTESIAN_POINT('Ctrl Pts',(1.4862001328979,2.03212299867471,102.039235810936));
#32253=CARTESIAN_POINT('Ctrl Pts',(1.46793845223857,2.04535362987872,102.040678027916));
#32254=CARTESIAN_POINT('Ctrl Pts',(1.43862464046938,2.06599669703487,102.042956121989));
#32255=CARTESIAN_POINT('Ctrl Pts',(1.42768760277896,2.07356970662602,102.043798072823));
#32256=CARTESIAN_POINT('Ctrl Pts',(1.40709532834494,2.08758801767768,102.045368582532));
#32257=CARTESIAN_POINT('Ctrl Pts',(1.39745458616321,2.0940538869551,102.046097901273));
#32258=CARTESIAN_POINT('Ctrl Pts',(1.37576658061112,2.10838315308245,102.047725515224));
#32259=CARTESIAN_POINT('Ctrl Pts',(1.36369588030189,2.11621047255517,102.048622454014));
#32260=CARTESIAN_POINT('Ctrl Pts',(1.32765221650936,2.13914674143955,102.051274941111));
#32261=CARTESIAN_POINT('Ctrl Pts',(1.30349004682474,2.15395519601591,102.053019494989));
#32262=CARTESIAN_POINT('Ctrl Pts',(1.24771043709163,2.18685883634807,102.056974960525));
#32263=CARTESIAN_POINT('Ctrl Pts',(1.21593967212873,2.20468224660051,102.059176393726));
#32264=CARTESIAN_POINT('Ctrl Pts',(1.10625261587917,2.26312407522971,102.066619203297));
#32265=CARTESIAN_POINT('Ctrl Pts',(1.0265995718532,2.30035225228205,102.071756184157));
#32266=CARTESIAN_POINT('Ctrl Pts',(0.832735420481711,2.37888013945891,102.083856062264));
#32267=CARTESIAN_POINT('Ctrl Pts',(0.717171235759592,2.41623327313614,102.090750583046));
#32268=CARTESIAN_POINT('Ctrl Pts',(0.505797278098832,2.46804718008178,102.103413272922));
#32269=CARTESIAN_POINT('Ctrl Pts',(0.410997770687885,2.48559133947329,102.1091137378));
#32270=CARTESIAN_POINT('Ctrl Pts',(0.301976193924167,2.4993600686096,102.115925550792));
#32271=CARTESIAN_POINT('Ctrl Pts',(0.288500707560359,2.50095135844207,102.116771963719));
#32272=CARTESIAN_POINT('Ctrl Pts',(0.266699318406875,2.50334729546376,102.118149469117));
#32273=CARTESIAN_POINT('Ctrl Pts',(0.258380915102101,2.50421954031975,102.118676971487));
#32274=CARTESIAN_POINT('Ctrl Pts',(0.24357211845672,2.50569778005592,102.119619696994));
#32275=CARTESIAN_POINT('Ctrl Pts',(0.237083520288757,2.50632004036768,102.120034013459));
#32276=CARTESIAN_POINT('Ctrl Pts',(0.222935205337559,2.50762143751097,102.120940213473));
#32277=CARTESIAN_POINT('Ctrl Pts',(0.215274884125142,2.50829067297999,102.121432613296));
#32278=CARTESIAN_POINT('Ctrl Pts',(0.193456111303942,2.51009616088944,102.1228398761));
#32279=CARTESIAN_POINT('Ctrl Pts',(0.17929120698126,2.51114767485487,102.123759192873));
#32280=CARTESIAN_POINT('Ctrl Pts',(0.0800077748094564,2.51767355857795,
102.130239263557));
#32281=CARTESIAN_POINT('Ctrl Pts',(-0.00532378543316241,2.51893826357532,
102.135994793692));
#32282=CARTESIAN_POINT('Ctrl Pts',(-0.259645833197371,2.50978533121428,
102.153409511484));
#32283=CARTESIAN_POINT('Ctrl Pts',(-0.427719297121613,2.48666482807939,
102.165230256701));
#32284=CARTESIAN_POINT('Ctrl Pts',(-0.687266663619545,2.42384763050094,
102.183273992997));
#32285=CARTESIAN_POINT('Ctrl Pts',(-0.780918006447934,2.39531708987386,
102.189747966364));
#32286=CARTESIAN_POINT('Ctrl Pts',(-0.894110023229313,2.35348579646905,
102.197518661793));
#32287=CARTESIAN_POINT('Ctrl Pts',(-0.915429978700684,2.34527527981217,
102.198980112063));
#32288=CARTESIAN_POINT('Ctrl Pts',(-0.949045752935968,2.33180126902361,
102.201281584918));
#32289=CARTESIAN_POINT('Ctrl Pts',(-0.961416063958937,2.32672820986001,
102.202127894035));
#32290=CARTESIAN_POINT('Ctrl Pts',(-0.9844443545709,2.31706930496512,102.203702418765));
#32291=CARTESIAN_POINT('Ctrl Pts',(-0.995112130544635,2.3125078823973,102.204431429945));
#32292=CARTESIAN_POINT('Ctrl Pts',(-1.00588014631224,2.3078152876672,102.205166988493));
#32293=CARTESIAN_POINT('Ctrl Pts',(-1.00601214941439,2.30775774854429,102.205176005522));
#32294=CARTESIAN_POINT('Ctrl Pts',(-1.00626873776199,2.30764587748561,102.205193532784));
#32295=CARTESIAN_POINT('Ctrl Pts',(-1.00639332353623,2.30759154678967,102.205202043057));
#32296=CARTESIAN_POINT('Ctrl Pts',(-1.006635523316,2.3074859023761,102.205218587293));
#32297=CARTESIAN_POINT('Ctrl Pts',(-1.00675313779619,2.30743458975627,102.205226621292));
#32298=CARTESIAN_POINT('Ctrl Pts',(-1.00698181168126,2.30733480354001,102.205242241457));
#32299=CARTESIAN_POINT('Ctrl Pts',(-1.0070928715131,2.30728633091591,102.205249827656));
#32300=CARTESIAN_POINT('Ctrl Pts',(-1.00730882554319,2.30719205812677,102.205264578833));
#32301=CARTESIAN_POINT('Ctrl Pts',(-1.00741372011044,2.30714625883009,102.20527174384));
#32302=CARTESIAN_POINT('Ctrl Pts',(-1.00761770774491,2.30705717673657,102.205285677517));
#32303=CARTESIAN_POINT('Ctrl Pts',(-1.00771680115004,2.30701389470735,102.205292446213));
#32304=CARTESIAN_POINT('Ctrl Pts',(-1.00790952710494,2.30692970105548,102.205305610545));
#32305=CARTESIAN_POINT('Ctrl Pts',(-1.00800315995954,2.30688879011373,102.205312006204));
#32306=CARTESIAN_POINT('Ctrl Pts',(-1.00818528366029,2.30680920171942,102.20532444625));
#32307=CARTESIAN_POINT('Ctrl Pts',(-1.00827377476478,2.30677052487849,102.205330490657));
#32308=CARTESIAN_POINT('Ctrl Pts',(-1.0084459135437,2.30669527631879,102.2053422486));
#32309=CARTESIAN_POINT('Ctrl Pts',(-1.00852956144568,2.30665870514574,102.205347962153));
#32310=CARTESIAN_POINT('Ctrl Pts',(-1.00869229353554,2.30658754752828,102.205359077502));
#32311=CARTESIAN_POINT('Ctrl Pts',(-1.00877137795136,2.30655296155901,102.205364479314));
#32312=CARTESIAN_POINT('Ctrl Pts',(-1.00892524528203,2.30648566136781,102.205374989096));
#32313=CARTESIAN_POINT('Ctrl Pts',(-1.00900002838378,2.30645294757648,102.205380097081));
#32314=CARTESIAN_POINT('Ctrl Pts',(-1.02195129036639,2.30078668084318,102.20626471746));
#32315=CARTESIAN_POINT('Ctrl Pts',(-1.03478056851933,2.29504531072591,102.207140578595));
#32316=CARTESIAN_POINT('Ctrl Pts',(-1.07383726669698,2.27717254103202,102.209806223099));
#32317=CARTESIAN_POINT('Ctrl Pts',(-1.09990504095687,2.26469650567027,102.211584259757));
#32318=CARTESIAN_POINT('Ctrl Pts',(-1.1594819676016,2.23491158575601,102.215649616219));
#32319=CARTESIAN_POINT('Ctrl Pts',(-1.19282887405432,2.21729287995418,102.217926350863));
#32320=CARTESIAN_POINT('Ctrl Pts',(-1.3067695500755,2.15377796747743,102.225728165427));
#32321=CARTESIAN_POINT('Ctrl Pts',(-1.3852178436821,2.10418146640345,102.231136726129));
#32322=CARTESIAN_POINT('Ctrl Pts',(-1.55484898303669,1.98333015279238,102.243164782171));
#32323=CARTESIAN_POINT('Ctrl Pts',(-1.64421455413009,1.90989820394562,102.249739042851));
#32324=CARTESIAN_POINT('Ctrl Pts',(-1.79710703433492,1.76555590827235,102.261980744939));
#32325=CARTESIAN_POINT('Ctrl Pts',(-1.86226116432162,1.69669107390033,102.267590972833));
#32326=CARTESIAN_POINT('Ctrl Pts',(-1.93211057729572,1.61398214365726,102.27430205417));
#32327=CARTESIAN_POINT('Ctrl Pts',(-1.94076440164278,1.60356576468318,102.275146814554));
#32328=CARTESIAN_POINT('Ctrl Pts',(-1.95462129051345,1.58661012369885,102.276522153058));
#32329=CARTESIAN_POINT('Ctrl Pts',(-1.95987669833531,1.58011372899273,102.277049159366));
#32330=CARTESIAN_POINT('Ctrl Pts',(-1.96917371556974,1.56850362192962,102.277991353126));
#32331=CARTESIAN_POINT('Ctrl Pts',(-1.97322793209571,1.56340022404815,102.278405638058));
#32332=CARTESIAN_POINT('Ctrl Pts',(-1.98202574031839,1.55223691364614,102.279312193489));
#32333=CARTESIAN_POINT('Ctrl Pts',(-1.98676130965998,1.54617106623109,102.279804983587));
#32334=CARTESIAN_POINT('Ctrl Pts',(-2.00017537856742,1.52882544968786,102.281214458159));
#32335=CARTESIAN_POINT('Ctrl Pts',(-2.00878597807941,1.51749387896731,102.282135617796));
#32336=CARTESIAN_POINT('Ctrl Pts',(-2.06881130035086,1.43709426650933,102.288670502877));
#32337=CARTESIAN_POINT('Ctrl Pts',(-2.11674395867628,1.36550796291995,102.294482661709));
#32338=CARTESIAN_POINT('Ctrl Pts',(-2.22849033970987,1.17855304495393,102.309391289842));
#32339=CARTESIAN_POINT('Ctrl Pts',(-2.28709287016483,1.06036032991809,102.318564208382));
#32340=CARTESIAN_POINT('Ctrl Pts',(-2.3449014233359,0.916401356570871,102.329174466241));
#32341=CARTESIAN_POINT('Ctrl Pts',(-2.35331951990706,0.89456198575824,102.330769975562));
#32342=CARTESIAN_POINT('Ctrl Pts',(-2.36143111379333,0.872610649034711,
102.332358906943));
#32343=CARTESIAN_POINT('Origin',(0.,0.,104.));
#32344=CARTESIAN_POINT('',(-2.36143100149827,0.872610952923958,103.332666057199));
#32345=CARTESIAN_POINT('',(-2.36143112101026,0.872610629504504,103.05616702425));
#32346=CARTESIAN_POINT('',(-2.36143112101026,0.872610629504505,104.));
#32347=CARTESIAN_POINT('',(-2.51749968066629,-0.00126800832535854,102.11258330245));
#32348=CARTESIAN_POINT('Ctrl Pts',(-2.36143112101026,0.872610629504504,
103.05616702425));
#32349=CARTESIAN_POINT('Ctrl Pts',(-2.33272565502948,0.950292448196763,
103.050921177399));
#32350=CARTESIAN_POINT('Ctrl Pts',(-2.30014405188381,1.02666168444337,103.045675330547));
#32351=CARTESIAN_POINT('Ctrl Pts',(-2.26383053884827,1.10130719664312,103.040429483695));
#32352=CARTESIAN_POINT('Ctrl Pts',(-2.22755357146253,1.17587758615385,103.035188916225));
#32353=CARTESIAN_POINT('Ctrl Pts',(-2.1875523595261,1.24872728615334,103.029948348755));
#32354=CARTESIAN_POINT('Ctrl Pts',(-2.14401936121982,1.319464750842,103.024707781285));
#32355=CARTESIAN_POINT('Ctrl Pts',(-2.1005098519192,1.39016404786996,103.019470041456));
#32356=CARTESIAN_POINT('Ctrl Pts',(-2.05347258115096,1.45875298021808,103.014232301627));
#32357=CARTESIAN_POINT('Ctrl Pts',(-2.00314554584338,1.5248652964009,103.008994561799));
#32358=CARTESIAN_POINT('Ctrl Pts',(-1.95283048431597,1.59096188317835,103.00375806813));
#32359=CARTESIAN_POINT('Ctrl Pts',(-1.89922749246793,1.65458265733426,102.998521574462));
#32360=CARTESIAN_POINT('Ctrl Pts',(-1.84261661039682,1.71539216422652,102.993285080793));
#32361=CARTESIAN_POINT('Ctrl Pts',(-1.78600212094128,1.77620554604988,102.988048253442));
#32362=CARTESIAN_POINT('Ctrl Pts',(-1.72637967611523,1.83420696813375,102.982811426092));
#32363=CARTESIAN_POINT('Ctrl Pts',(-1.66406718599625,1.88909678166327,102.977574598741));
#32364=CARTESIAN_POINT('Ctrl Pts',(-1.60169040302655,1.94404322946596,102.972332368131));
#32365=CARTESIAN_POINT('Ctrl Pts',(-1.53661837932049,1.99587135211307,102.96709013752));
#32366=CARTESIAN_POINT('Ctrl Pts',(-1.46920282596402,2.04432123360771,102.96184790691));
#32367=CARTESIAN_POINT('Ctrl Pts',(-1.40175133933086,2.09279693945459,102.95660288213));
#32368=CARTESIAN_POINT('Ctrl Pts',(-1.33195422328854,2.13789056774503,102.951357857349));
#32369=CARTESIAN_POINT('Ctrl Pts',(-1.2601908859708,2.17938642303657,102.946112832569));
#32370=CARTESIAN_POINT('Ctrl Pts',(-1.18830350299189,2.22095400549406,102.940858741563));
#32371=CARTESIAN_POINT('Ctrl Pts',(-1.11444352097549,2.25891118210886,102.935604650558));
#32372=CARTESIAN_POINT('Ctrl Pts',(-1.03901334447018,2.29308907808068,102.930350559552));
#32373=CARTESIAN_POINT('Ctrl Pts',(-0.982041288511566,2.31890348144108,
102.926382169438));
#32374=CARTESIAN_POINT('Ctrl Pts',(-0.924173959955293,2.34256289199948,
102.922413779323));
#32375=CARTESIAN_POINT('Ctrl Pts',(-0.865590384616286,2.36401343821473,
102.918445389209));
#32376=CARTESIAN_POINT('Ctrl Pts',(-0.788009478833714,2.39241991213306,
102.913190139802));
#32377=CARTESIAN_POINT('Ctrl Pts',(-0.708885477545965,2.41705578739818,
102.907934890394));
#32378=CARTESIAN_POINT('Ctrl Pts',(-0.628619422757687,2.43775385782318,
102.902679640987));
#32379=CARTESIAN_POINT('Ctrl Pts',(-0.548467167000853,2.45842258308635,
102.89743184233));
#32380=CARTESIAN_POINT('Ctrl Pts',(-0.46717651696939,2.47516447854799,102.892184043672));
#32381=CARTESIAN_POINT('Ctrl Pts',(-0.385166524085117,2.4878611293085,102.886936245015));
#32382=CARTESIAN_POINT('Ctrl Pts',(-0.302562298101391,2.50064977824959,
102.881650421532));
#32383=CARTESIAN_POINT('Ctrl Pts',(-0.219228705756596,2.50933414962651,
102.876364598049));
#32384=CARTESIAN_POINT('Ctrl Pts',(-0.135607525173053,2.51384503283644,
102.871078774566));
#32385=CARTESIAN_POINT('Ctrl Pts',(-0.0527361699438051,2.51831546726799,
102.865840348697));
#32386=CARTESIAN_POINT('Ctrl Pts',(0.0304171673725803,2.51868693520644,
102.860601922829));
#32387=CARTESIAN_POINT('Ctrl Pts',(0.113416093058451,2.51494394367655,102.85536349696));
#32388=CARTESIAN_POINT('Ctrl Pts',(0.19638772177894,2.51120218315428,102.850126793923));
#32389=CARTESIAN_POINT('Ctrl Pts',(0.279204579138952,2.50334867141904,102.844890090885));
#32390=CARTESIAN_POINT('Ctrl Pts',(0.361431247096607,2.49142001750451,102.839653387848));
#32391=CARTESIAN_POINT('Ctrl Pts',(0.443655675240946,2.47949168852056,102.834416827455));
#32392=CARTESIAN_POINT('Ctrl Pts',(0.525289489454487,2.46348850532888,102.829180267063));
#32393=CARTESIAN_POINT('Ctrl Pts',(0.605904746065709,2.44349865739579,102.823943706671));
#32394=CARTESIAN_POINT('Ctrl Pts',(0.687839457124257,2.42318162953591,102.8186214379));
#32395=CARTESIAN_POINT('Ctrl Pts',(0.768721487248275,2.39874636322157,102.81329916913));
#32396=CARTESIAN_POINT('Ctrl Pts',(0.84811658852575,2.37033847841768,102.807976900359));
#32397=CARTESIAN_POINT('Ctrl Pts',(0.926345317707781,2.34234792621483,102.802732819609));
#32398=CARTESIAN_POINT('Ctrl Pts',(1.00313010739013,2.31050093807368,102.797488738859));
#32399=CARTESIAN_POINT('Ctrl Pts',(1.07807656706824,2.27498509127826,102.792244658108));
#32400=CARTESIAN_POINT('Ctrl Pts',(1.15469917808106,2.23867494500205,102.786883295328));
#32401=CARTESIAN_POINT('Ctrl Pts',(1.22939978860889,2.19853009672539,102.781521932547));
#32402=CARTESIAN_POINT('Ctrl Pts',(1.30178609528669,2.15479911177776,102.776160569766));
#32403=CARTESIAN_POINT('Ctrl Pts',(1.3741724019645,2.11106812683013,102.770799206986));
#32404=CARTESIAN_POINT('Ctrl Pts',(1.44424402108161,2.06375134491817,102.765437844205));
#32405=CARTESIAN_POINT('Ctrl Pts',(1.51164419791891,2.0131413434973,102.760076481425));
#32406=CARTESIAN_POINT('Ctrl Pts',(1.57771037435099,1.9635330273178,102.754821232017));
#32407=CARTESIAN_POINT('Ctrl Pts',(1.64145394247886,1.91057746621046,102.74956598261));
#32408=CARTESIAN_POINT('Ctrl Pts',(1.70251630309744,1.85452001544535,102.744310733203));
#32409=CARTESIAN_POINT('Ctrl Pts',(1.76349209116036,1.7985420414107,102.739062934545));
#32410=CARTESIAN_POINT('Ctrl Pts',(1.82179388522043,1.73947122242562,102.733815135888));
#32411=CARTESIAN_POINT('Ctrl Pts',(1.87709420657265,1.67759458441288,102.72856733723));
#32412=CARTESIAN_POINT('Ctrl Pts',(1.93279522642758,1.61526959681376,102.723281513747));
#32413=CARTESIAN_POINT('Ctrl Pts',(1.9854507145793,1.55009824201116,102.717995690264));
#32414=CARTESIAN_POINT('Ctrl Pts',(2.03476209091976,1.48241339826509,102.712709866781));
#32415=CARTESIAN_POINT('Ctrl Pts',(2.08363129555232,1.41533547984091,102.707471440913));
#32416=CARTESIAN_POINT('Ctrl Pts',(2.12921584430077,1.34578934831167,102.702233015044));
#32417=CARTESIAN_POINT('Ctrl Pts',(2.1712651465362,1.27413261218647,102.696994589176));
#32418=CARTESIAN_POINT('Ctrl Pts',(2.21330061945593,1.20249944276924,102.691757886138));
#32419=CARTESIAN_POINT('Ctrl Pts',(2.25180292167082,1.12875744500863,102.6865211831));
#32420=CARTESIAN_POINT('Ctrl Pts',(2.28656569652326,1.05329177604455,102.681284480063));
#32421=CARTESIAN_POINT('Ctrl Pts',(2.32132752445511,0.977828162727556,102.676047919671));
#32422=CARTESIAN_POINT('Ctrl Pts',(2.35234983543767,0.900641391084837,102.670811359278));
#32423=CARTESIAN_POINT('Ctrl Pts',(2.37947360751494,0.822138431859156,102.665574798886));
#32424=CARTESIAN_POINT('Ctrl Pts',(2.40704132262729,0.742350590800591,102.660252530115));
#32425=CARTESIAN_POINT('Ctrl Pts',(2.43058155731741,0.66120354903341,102.654930261345));
#32426=CARTESIAN_POINT('Ctrl Pts',(2.44998002953487,0.579140833373282,102.649607992574));
#32427=CARTESIAN_POINT('Ctrl Pts',(2.46909352401034,0.498283679014527,102.644363911824));
#32428=CARTESIAN_POINT('Ctrl Pts',(2.48418611465781,0.416538047401716,102.639119831074));
#32429=CARTESIAN_POINT('Ctrl Pts',(2.49520041333014,0.334336876992537,102.633875750323));
#32430=CARTESIAN_POINT('Ctrl Pts',(2.50646104293656,0.250297306182818,102.628514387543));
#32431=CARTESIAN_POINT('Ctrl Pts',(2.51345871792467,0.165782085061767,102.623153024762));
#32432=CARTESIAN_POINT('Ctrl Pts',(2.51618834279569,0.0812556064470767,
102.617791661982));
#32433=CARTESIAN_POINT('Ctrl Pts',(2.51891796766671,-0.00327087216761331,
102.612430299201));
#32434=CARTESIAN_POINT('Ctrl Pts',(2.51737961845209,-0.087808101468579,
102.60706893642));
#32435=CARTESIAN_POINT('Ctrl Pts',(2.51162447120052,-0.171897544097395,
102.60170757364));
#32436=CARTESIAN_POINT('Ctrl Pts',(2.50598323119854,-0.254322668384581,
102.596452324233));
#32437=CARTESIAN_POINT('Ctrl Pts',(2.49626980025757,-0.336622019470838,
102.591197074825));
#32438=CARTESIAN_POINT('Ctrl Pts',(2.48249474058826,-0.41836122304967,102.585941825418));
#32439=CARTESIAN_POINT('Ctrl Pts',(2.46873921082425,-0.499984539006743,
102.58069402676));
#32440=CARTESIAN_POINT('Ctrl Pts',(2.45093356636748,-0.581048833684912,
102.575446228103));
#32441=CARTESIAN_POINT('Ctrl Pts',(2.42914026605549,-0.661123148761145,
102.570198429445));
#32442=CARTESIAN_POINT('Ctrl Pts',(2.40718905449469,-0.741777671282336,
102.564912605963));
#32443=CARTESIAN_POINT('Ctrl Pts',(2.38119218759281,-0.821427334373817,
102.55962678248));
#32444=CARTESIAN_POINT('Ctrl Pts',(2.35126631866033,-0.899640455256151,
102.554340958997));
#32445=CARTESIAN_POINT('Ctrl Pts',(2.32160879292891,-0.977152244482249,
102.549102533128));
#32446=CARTESIAN_POINT('Ctrl Pts',(2.2880926130632,-1.0532527121713,102.54386410726));
#32447=CARTESIAN_POINT('Ctrl Pts',(2.25088130386266,-1.12753696432602,102.538625681391));
#32448=CARTESIAN_POINT('Ctrl Pts',(2.21368223284243,-1.20179678562646,102.533388978354));
#32449=CARTESIAN_POINT('Ctrl Pts',(2.17279065257134,-1.27424116548096,102.528152275316));
#32450=CARTESIAN_POINT('Ctrl Pts',(2.12841727868255,-1.34448731411106,102.522915572279));
#32451=CARTESIAN_POINT('Ctrl Pts',(2.08404511350229,-1.41473154927118,102.517679011886));
#32452=CARTESIAN_POINT('Ctrl Pts',(2.0361915905717,-1.4827772827043,102.512442451494));
#32453=CARTESIAN_POINT('Ctrl Pts',(1.98511149405792,-1.54826955216433,102.507205891102));
#32454=CARTESIAN_POINT('Ctrl Pts',(1.93319535405377,-1.61483375353694,102.501883622331));
#32455=CARTESIAN_POINT('Ctrl Pts',(1.8779463589783,-1.67875975435023,102.496561353561));
#32456=CARTESIAN_POINT('Ctrl Pts',(1.81967431466198,-1.73971021683482,102.49123908479));
#32457=CARTESIAN_POINT('Ctrl Pts',(1.76225832928811,-1.79976527245548,102.48599500404));
#32458=CARTESIAN_POINT('Ctrl Pts',(1.70190790868203,-1.85693135779367,102.48075092329));
#32459=CARTESIAN_POINT('Ctrl Pts',(1.63895495321572,-1.91092462209519,102.475506842539));
#32460=CARTESIAN_POINT('Ctrl Pts',(1.57459407693793,-1.96612542685176,102.470145479759));
#32461=CARTESIAN_POINT('Ctrl Pts',(1.50751325655197,-2.0180094667169,102.464784116978));
#32462=CARTESIAN_POINT('Ctrl Pts',(1.43809924691835,-2.06631962823104,102.459422754198));
#32463=CARTESIAN_POINT('Ctrl Pts',(1.36868523728473,-2.11462978974519,102.454061391417));
#32464=CARTESIAN_POINT('Ctrl Pts',(1.29693850490501,-2.15936586075086,102.448700028637));
#32465=CARTESIAN_POINT('Ctrl Pts',(1.22327153025748,-2.20032111594229,102.443338665856));
#32466=CARTESIAN_POINT('Ctrl Pts',(1.15106258997487,-2.24046577493673,102.438083416449));
#32467=CARTESIAN_POINT('Ctrl Pts',(1.0767420365693,-2.27712623417218,102.432828167041));
#32468=CARTESIAN_POINT('Ctrl Pts',(1.00067997047002,-2.31007485738019,102.427572917634));
#32469=CARTESIAN_POINT('Ctrl Pts',(0.92472574310124,-2.34297676692552,102.422325118977));
#32470=CARTESIAN_POINT('Ctrl Pts',(0.847035327201603,-2.37217711150451,
102.417077320319));
#32471=CARTESIAN_POINT('Ctrl Pts',(0.768004213099297,-2.39749364517651,
102.411829521662));
#32472=CARTESIAN_POINT('Ctrl Pts',(0.688400450442436,-2.42299361896039,
102.406543698179));
#32473=CARTESIAN_POINT('Ctrl Pts',(0.607436892757032,-2.44455303097053,
102.401257874696));
#32474=CARTESIAN_POINT('Ctrl Pts',(0.525539144305114,-2.46203469874067,
102.395972051213));
#32475=CARTESIAN_POINT('Ctrl Pts',(0.444375767310515,-2.4793596096026,102.390733625344));
#32476=CARTESIAN_POINT('Ctrl Pts',(0.362295345666176,-2.49267951493152,
102.385495199476));
#32477=CARTESIAN_POINT('Ctrl Pts',(0.279726532665683,-2.50191113289878,
102.380256773607));
#32478=CARTESIAN_POINT('Ctrl Pts',(0.19718487517368,-2.51113971474052,102.37502007057));
#32479=CARTESIAN_POINT('Ctrl Pts',(0.11415560353496,-2.51628262838044,102.369783367532));
#32480=CARTESIAN_POINT('Ctrl Pts',(0.0310745233179384,-2.51730820997361,
102.364546664495));
#32481=CARTESIAN_POINT('Ctrl Pts',(-0.0520042938120273,-2.51833376363045,
102.359310104102));
#32482=CARTESIAN_POINT('Ctrl Pts',(-0.13513445531612,-2.51524220356714,
102.35407354371));
#32483=CARTESIAN_POINT('Ctrl Pts',(-0.217879503963275,-2.50805398102846,
102.348836983318));
#32484=CARTESIAN_POINT('Ctrl Pts',(-0.301978866012361,-2.50074810666312,
102.343514714547));
#32485=CARTESIAN_POINT('Ctrl Pts',(-0.385679903931832,-2.48921028676346,
102.338192445777));
#32486=CARTESIAN_POINT('Ctrl Pts',(-0.468530987135187,-2.47351671999486,
102.332870177006));
#32487=CARTESIAN_POINT('Ctrl Pts',(-0.550164927341432,-2.45805370319801,
102.327626096256));
#32488=CARTESIAN_POINT('Ctrl Pts',(-0.630973279405555,-2.43855640038693,
102.322382015506));
#32489=CARTESIAN_POINT('Ctrl Pts',(-0.710537247829162,-2.41514866404687,
102.317137934755));
#32490=CARTESIAN_POINT('Ctrl Pts',(-0.791880636554139,-2.39121742187774,
102.311776571975));
#32491=CARTESIAN_POINT('Ctrl Pts',(-0.871922826292059,-2.36319889375182,
102.306415209194));
#32492=CARTESIAN_POINT('Ctrl Pts',(-0.950237582969059,-2.33127750083792,
102.301053846414));
#32493=CARTESIAN_POINT('Ctrl Pts',(-1.02855233964605,-2.29935610792404,
102.295692483633));
#32494=CARTESIAN_POINT('Ctrl Pts',(-1.10513923131857,-2.26353212601061,
102.290331120853));
#32495=CARTESIAN_POINT('Ctrl Pts',(-1.17960028275469,-2.22403898862521,
102.284969758072));
#32496=CARTESIAN_POINT('Ctrl Pts',(-1.25258758326841,-2.18532750885178,
102.279714508665));
#32497=CARTESIAN_POINT('Ctrl Pts',(-1.32380203496534,-2.14294784628376,
102.274459259257));
#32498=CARTESIAN_POINT('Ctrl Pts',(-1.39285119654326,-2.09708650138425,
102.26920400985));
#32499=CARTESIAN_POINT('Ctrl Pts',(-1.46180246209607,-2.0512901774534,102.263956211193));
#32500=CARTESIAN_POINT('Ctrl Pts',(-1.52859415406789,-2.00202222915303,
102.258708412535));
#32501=CARTESIAN_POINT('Ctrl Pts',(-1.59285808064314,-1.94951516663242,
102.253460613878));
#32502=CARTESIAN_POINT('Ctrl Pts',(-1.65758765476851,-1.89662764517739,
102.248174790395));
#32503=CARTESIAN_POINT('Ctrl Pts',(-1.71975225860477,-1.8404540931339,102.242888966912));
#32504=CARTESIAN_POINT('Ctrl Pts',(-1.77900510365269,-1.78127681486558,
102.237603143429));
#32505=CARTESIAN_POINT('Ctrl Pts',(-1.83772663252902,-1.72263017516676,
102.23236471756));
#32506=CARTESIAN_POINT('Ctrl Pts',(-1.89358808005325,-1.66103379397616,
102.227126291692));
#32507=CARTESIAN_POINT('Ctrl Pts',(-1.94628620911516,-1.59680187944784,
102.221887865823));
#32508=CARTESIAN_POINT('Ctrl Pts',(-1.99896700663946,-1.5325910897272,102.216651162786));
#32509=CARTESIAN_POINT('Ctrl Pts',(-2.04848625947963,-1.46574684459179,
102.211414459748));
#32510=CARTESIAN_POINT('Ctrl Pts',(-2.09458013322477,-1.39661745496041,
102.206177756711));
#32511=CARTESIAN_POINT('Ctrl Pts',(-2.14067275139581,-1.32748994837909,
102.200941196318));
#32512=CARTESIAN_POINT('Ctrl Pts',(-2.18333992086581,-1.25607780554095,
102.195704635926));
#32513=CARTESIAN_POINT('Ctrl Pts',(-2.22236116616033,-1.18275825811638,
102.190468075534));
#32514=CARTESIAN_POINT('Ctrl Pts',(-2.26202108405615,-1.10823866733784,
102.185145806763));
#32515=CARTESIAN_POINT('Ctrl Pts',(-2.29791441049229,-1.03174909841384,
102.179823537993));
#32516=CARTESIAN_POINT('Ctrl Pts',(-2.32985916934359,-0.953709862078392,
102.174501269222));
#32517=CARTESIAN_POINT('Ctrl Pts',(-2.36133463632777,-0.876817079190902,
102.169257188472));
#32518=CARTESIAN_POINT('Ctrl Pts',(-2.38897668257423,-0.79842031994964,
102.164013107722));
#32519=CARTESIAN_POINT('Ctrl Pts',(-2.41266118072925,-0.718938298466652,
102.158769026971));
#32520=CARTESIAN_POINT('Ctrl Pts',(-2.43687537439444,-0.637678689396935,
102.153407664191));
#32521=CARTESIAN_POINT('Ctrl Pts',(-2.456952744312,-0.555285186779454,102.14804630141));
#32522=CARTESIAN_POINT('Ctrl Pts',(-2.47281591772869,-0.472215720860313,
102.14268493863));
#32523=CARTESIAN_POINT('Ctrl Pts',(-2.48867909114538,-0.38914625494116,
102.137323575849));
#32524=CARTESIAN_POINT('Ctrl Pts',(-2.50032806421808,-0.305401338184696,
102.131962213068));
#32525=CARTESIAN_POINT('Ctrl Pts',(-2.50774196095251,-0.221441882393651,
102.126600850288));
#32526=CARTESIAN_POINT('Ctrl Pts',(-2.51420329401792,-0.148269834375223,
102.121928334356));
#32527=CARTESIAN_POINT('Ctrl Pts',(-2.51746263872295,-0.0748109262768815,
102.117255818424));
#32528=CARTESIAN_POINT('Ctrl Pts',(-2.51749968066596,-0.00126800898220263,
102.112583302492));
#32529=CARTESIAN_POINT('Ctrl Pts',(-2.51749968066629,-0.00126800832534177,
102.11258330245));
#32530=CARTESIAN_POINT('Ctrl Pts',(-2.51754083200824,0.0804337345976501,
102.107392419228));
#32531=CARTESIAN_POINT('Ctrl Pts',(-2.51360049225428,0.162294868972713,
102.102201536007));
#32532=CARTESIAN_POINT('Ctrl Pts',(-2.50565839985951,0.243889797272241,
102.097010652785));
#32533=CARTESIAN_POINT('Ctrl Pts',(-2.49772544325755,0.325390866885326,
102.091825740638));
#32534=CARTESIAN_POINT('Ctrl Pts',(-2.48579990849483,0.406625870881061,
102.086640828492));
#32535=CARTESIAN_POINT('Ctrl Pts',(-2.46991353078061,0.487168759740263,
102.081455916346));
#32536=CARTESIAN_POINT('Ctrl Pts',(-2.45404174187781,0.567637684286298,
102.076275765619));
#32537=CARTESIAN_POINT('Ctrl Pts',(-2.43421642245339,0.647415293431656,
102.071095614892));
#32538=CARTESIAN_POINT('Ctrl Pts',(-2.41052097619079,0.726081864078853,
102.065915464165));
#32539=CARTESIAN_POINT('Ctrl Pts',(-2.39566720092542,0.775394949316457,
102.062668224425));
#32540=CARTESIAN_POINT('Ctrl Pts',(-2.37929366785987,0.824271573567107,
102.059420984686));
#32541=CARTESIAN_POINT('Ctrl Pts',(-2.36143112101026,0.872610629504504,
102.056173744947));
#32542=CARTESIAN_POINT('',(-2.51749892479438,-0.00189520973707386,102.388647960208));
#32543=CARTESIAN_POINT('Ctrl Pts',(-2.36143111379333,0.872610649034711,
102.332358906943));
#32544=CARTESIAN_POINT('Ctrl Pts',(-2.38167255387254,0.81783390932394,102.336323881003));
#32545=CARTESIAN_POINT('Ctrl Pts',(-2.400005456087,0.762359938864054,102.340247356964));
#32546=CARTESIAN_POINT('Ctrl Pts',(-2.43298340665052,0.649533881196489,
102.348032574994));
#32547=CARTESIAN_POINT('Ctrl Pts',(-2.44756857832329,0.592209019412611,
102.351890070134));
#32548=CARTESIAN_POINT('Ctrl Pts',(-2.46430302505784,0.515174439931453,
102.356947278273));
#32549=CARTESIAN_POINT('Ctrl Pts',(-2.46825782248767,0.495880490231162,
102.358203518278));
#32550=CARTESIAN_POINT('Ctrl Pts',(-2.474361959814,0.464216225329726,102.36024870174));
#32551=CARTESIAN_POINT('Ctrl Pts',(-2.47664583673482,0.451873013884803,
102.361041864692));
#32552=CARTESIAN_POINT('Ctrl Pts',(-2.48089469194113,0.427909627950764,
102.362574010339));
#32553=CARTESIAN_POINT('Ctrl Pts',(-2.4828705790581,0.416291745552828,102.363313318437));
#32554=CARTESIAN_POINT('Ctrl Pts',(-2.48662534698678,0.393236070607597,
102.364773717817));
#32555=CARTESIAN_POINT('Ctrl Pts',(-2.48840706519073,0.381799041999803,
102.36549488103));
#32556=CARTESIAN_POINT('Ctrl Pts',(-2.49236442873955,0.355191048042248,
102.367165254244));
#32557=CARTESIAN_POINT('Ctrl Pts',(-2.49448055866104,0.340011594931609,
102.368112601438));
#32558=CARTESIAN_POINT('Ctrl Pts',(-2.50142524011857,0.28663602605955,102.3714251183));
#32559=CARTESIAN_POINT('Ctrl Pts',(-2.5055162804201,0.248348235283293,102.373767724152));
#32560=CARTESIAN_POINT('Ctrl Pts',(-2.51462593031466,0.139511104565593,
102.380346387944));
#32561=CARTESIAN_POINT('Ctrl Pts',(-2.51755260110758,0.0688228082331917,
102.384522807845));
#32562=CARTESIAN_POINT('Ctrl Pts',(-2.51749928456623,-0.00189794850746936,
102.388648747491));
#32563=CARTESIAN_POINT('Ctrl Pts',(-2.51749928665677,-0.001895173516098,
102.388648585595));
#32564=CARTESIAN_POINT('Ctrl Pts',(-2.51738362772184,-0.155533499352556,
102.397612045468));
#32565=CARTESIAN_POINT('Ctrl Pts',(-2.50320419797107,-0.308839288588633,
102.40629201102));
#32566=CARTESIAN_POINT('Ctrl Pts',(-2.46354884846836,-0.522261120674775,
102.418941987187));
#32567=CARTESIAN_POINT('Ctrl Pts',(-2.4496094044207,-0.58415948973351,102.422683426095));
#32568=CARTESIAN_POINT('Ctrl Pts',(-2.42408646069048,-0.680379425043883,
102.428704454135));
#32569=CARTESIAN_POINT('Ctrl Pts',(-2.4140741531442,-0.715092305514733,
102.430919516845));
#32570=CARTESIAN_POINT('Ctrl Pts',(-2.40002439675338,-0.760139190160104,
102.43386476658));
#32571=CARTESIAN_POINT('Ctrl Pts',(-2.39666017356873,-0.770680670101884,
102.434559106641));
#32572=CARTESIAN_POINT('Ctrl Pts',(-2.39105361636841,-0.787856517963723,
102.435699331359));
#32573=CARTESIAN_POINT('Ctrl Pts',(-2.38885285789073,-0.794504442866894,
102.436142843075));
#32574=CARTESIAN_POINT('Ctrl Pts',(-2.38450457701741,-0.807458076994481,
102.437011466609));
#32575=CARTESIAN_POINT('Ctrl Pts',(-2.38235971969409,-0.813764576692406,
102.437436423997));
#32576=CARTESIAN_POINT('Ctrl Pts',(-2.37751496396946,-0.827826237226315,
102.438388463557));
#32577=CARTESIAN_POINT('Ctrl Pts',(-2.37480210062592,-0.835576843466313,
102.438916286986));
#32578=CARTESIAN_POINT('Ctrl Pts',(-2.36529464143894,-0.862319177183936,
102.440747760597));
#32579=CARTESIAN_POINT('Ctrl Pts',(-2.35830995182773,-0.881241859515909,
102.442061700365));
#32580=CARTESIAN_POINT('Ctrl Pts',(-2.2912579183836,-1.05638888913749,102.454378340713));
#32581=CARTESIAN_POINT('Ctrl Pts',(-2.21598289091404,-1.2063299337195,102.466044872105));
#32582=CARTESIAN_POINT('Ctrl Pts',(-2.06414888723597,-1.44589649694668,
102.485603242282));
#32583=CARTESIAN_POINT('Ctrl Pts',(-1.99516590995544,-1.5396900257187,102.493544571162));
#32584=CARTESIAN_POINT('Ctrl Pts',(-1.89189916779521,-1.66144604537815,
102.504149853271));
#32585=CARTESIAN_POINT('Ctrl Pts',(-1.86300912178895,-1.69377767128789,
102.506998936773));
#32586=CARTESIAN_POINT('Ctrl Pts',(-1.81125385555683,-1.7487710627214,102.511903753183));
#32587=CARTESIAN_POINT('Ctrl Pts',(-1.78876303182323,-1.77176966091257,
102.51397404432));
#32588=CARTESIAN_POINT('Ctrl Pts',(-1.75539796790109,-1.80460486755361,
102.516959343884));
#32589=CARTESIAN_POINT('Ctrl Pts',(-1.74486954165176,-1.81478677841368,
102.517889357872));
#32590=CARTESIAN_POINT('Ctrl Pts',(-1.72622127333777,-1.83250896993319,
102.519515950083));
#32591=CARTESIAN_POINT('Ctrl Pts',(-1.718139469951,-1.84008852437888,102.520214204376));
#32592=CARTESIAN_POINT('Ctrl Pts',(-1.70087545799637,-1.85606674582451,
102.521691837917));
#32593=CARTESIAN_POINT('Ctrl Pts',(-1.69168046265567,-1.86445120872301,
102.522470605455));
#32594=CARTESIAN_POINT('Ctrl Pts',(-1.66814980582276,-1.88559026410293,
102.524443019386));
#32595=CARTESIAN_POINT('Ctrl Pts',(-1.65372963604511,-1.8982499153901,102.525632704994));
#32596=CARTESIAN_POINT('Ctrl Pts',(-1.59733936071315,-1.9466253254089,102.530213812539));
#32597=CARTESIAN_POINT('Ctrl Pts',(-1.55434395182887,-1.98112562449927,
102.533556177902));
#32598=CARTESIAN_POINT('Ctrl Pts',(-1.34101933116887,-2.14107742255326,
102.549505816003));
#32599=CARTESIAN_POINT('Ctrl Pts',(-1.15648519806792,-2.24612681314428,
102.561340359612));
#32600=CARTESIAN_POINT('Ctrl Pts',(-0.902554173308147,-2.35099964323332,
102.577352426539));
#32601=CARTESIAN_POINT('Ctrl Pts',(-0.843234281619375,-2.37292188018799,
102.581082163725));
#32602=CARTESIAN_POINT('Ctrl Pts',(-0.760125206045787,-2.40012566221989,
102.586371767267));
#32603=CARTESIAN_POINT('Ctrl Pts',(-0.736987121664504,-2.40733118141019,
102.587851193457));
#32604=CARTESIAN_POINT('Ctrl Pts',(-0.696571593415484,-2.41927988015266,
102.590452825256));
#32605=CARTESIAN_POINT('Ctrl Pts',(-0.679340515732245,-2.42417481726747,
102.591567502736));
#32606=CARTESIAN_POINT('Ctrl Pts',(-0.65391888261364,-2.43110417997221,
102.593222049707));
#32607=CARTESIAN_POINT('Ctrl Pts',(-0.645767556050396,-2.43328208344487,
102.593754079877));
#32608=CARTESIAN_POINT('Ctrl Pts',(-0.631293804746132,-2.43707138819131,
102.594701690055));
#32609=CARTESIAN_POINT('Ctrl Pts',(-0.624975860400547,-2.43869924172159,
102.595116325528));
#32610=CARTESIAN_POINT('Ctrl Pts',(-0.61124888880824,-2.44217922500546,
102.596019420535));
#32611=CARTESIAN_POINT('Ctrl Pts',(-0.603837855717199,-2.444022179,102.59650836678));
#32612=CARTESIAN_POINT('Ctrl Pts',(-0.583227450922472,-2.44904804890784,
102.597871745425));
#32613=CARTESIAN_POINT('Ctrl Pts',(-0.570010768033392,-2.45215788854564,
102.598750118524));
#32614=CARTESIAN_POINT('Ctrl Pts',(-0.495995283226894,-2.46894277684054,
102.603689511775));
#32615=CARTESIAN_POINT('Ctrl Pts',(-0.434735010062842,-2.48046242671523,
102.607853896467));
#32616=CARTESIAN_POINT('Ctrl Pts',(-0.231744205592185,-2.51088347797545,
102.62177198319));
#32617=CARTESIAN_POINT('Ctrl Pts',(-0.088826954223493,-2.51999019966902,
102.631743944321));
#32618=CARTESIAN_POINT('Ctrl Pts',(0.186648054686333,-2.51407012709301,
102.650653081945));
#32619=CARTESIAN_POINT('Ctrl Pts',(0.318789920484328,-2.50075355891401,
102.659584459724));
#32620=CARTESIAN_POINT('Ctrl Pts',(0.481158364700997,-2.47130374948898,
102.670301829104));
#32621=CARTESIAN_POINT('Ctrl Pts',(0.512918502786566,-2.46490777987964,
102.672386686747));
#32622=CARTESIAN_POINT('Ctrl Pts',(0.559356598471792,-2.45461942400073,
102.675419405697));
#32623=CARTESIAN_POINT('Ctrl Pts',(0.574135898987559,-2.45120466441293,
102.676382256309));
#32624=CARTESIAN_POINT('Ctrl Pts',(0.600248772738025,-2.44492214645146,
102.678079588396));
#32625=CARTESIAN_POINT('Ctrl Pts',(0.611594811928431,-2.44210865541391,
102.678815773851));
#32626=CARTESIAN_POINT('Ctrl Pts',(0.635355540528583,-2.43604069931775,
102.680354913031));
#32627=CARTESIAN_POINT('Ctrl Pts',(0.647765796243572,-2.43277011543186,
102.681157327286));
#32628=CARTESIAN_POINT('Ctrl Pts',(0.680403551654847,-2.42390134343649,
102.683264020846));
#32629=CARTESIAN_POINT('Ctrl Pts',(0.700587262337777,-2.4181447940243,102.684563189834));
#32630=CARTESIAN_POINT('Ctrl Pts',(0.788341933381007,-2.39192548969818,
102.690198597133));
#32631=CARTESIAN_POINT('Ctrl Pts',(0.855110519443737,-2.36887692477376,
102.694450997935));
#32632=CARTESIAN_POINT('Ctrl Pts',(1.10160037687089,-2.27200557293898,102.710147068473));
#32633=CARTESIAN_POINT('Ctrl Pts',(1.27353554913689,-2.18028383510349,102.72103888105));
#32634=CARTESIAN_POINT('Ctrl Pts',(1.5082181965256,-2.01777279508252,102.737688709874));
#32635=CARTESIAN_POINT('Ctrl Pts',(1.58033430860803,-1.96180245939454,102.743104498823));
#32636=CARTESIAN_POINT('Ctrl Pts',(1.6601241095028,-1.8926176305945,102.749657701103));
#32637=CARTESIAN_POINT('Ctrl Pts',(1.67092089174682,-1.88309237838327,102.750557112652));
#32638=CARTESIAN_POINT('Ctrl Pts',(1.68738818347471,-1.86831130524999,102.751949586056));
#32639=CARTESIAN_POINT('Ctrl Pts',(1.69311737844635,-1.86312091772818,102.752437957361));
#32640=CARTESIAN_POINT('Ctrl Pts',(1.70363036797095,-1.85350809594487,102.753341548518));
#32641=CARTESIAN_POINT('Ctrl Pts',(1.70842099312952,-1.84909339936437,102.753756197223));
#32642=CARTESIAN_POINT('Ctrl Pts',(1.71928318439554,-1.83900533761206,102.754702958101));
#32643=CARTESIAN_POINT('Ctrl Pts',(1.72534380085671,-1.8333205022769,102.755235920716));
#32644=CARTESIAN_POINT('Ctrl Pts',(1.74109414425502,-1.81839946924077,102.756633080516));
#32645=CARTESIAN_POINT('Ctrl Pts',(1.75073839842545,-1.80911594179759,102.757500668789));
#32646=CARTESIAN_POINT('Ctrl Pts',(1.82154010904192,-1.73986611105077,102.763956873288));
#32647=CARTESIAN_POINT('Ctrl Pts',(1.87966989575546,-1.67689608128999,102.769740836745));
#32648=CARTESIAN_POINT('Ctrl Pts',(1.96320419216849,-1.57659484543098,102.778677205794));
#32649=CARTESIAN_POINT('Ctrl Pts',(1.99100792627152,-1.54133360746604,102.781771417119));
#32650=CARTESIAN_POINT('Ctrl Pts',(2.10750504768939,-1.38517435215583,102.795223097379));
#32651=CARTESIAN_POINT('Ctrl Pts',(2.18625148611282,-1.25721863938396,102.805587850679));
#32652=CARTESIAN_POINT('Ctrl Pts',(2.28673886885793,-1.05560544542765,102.82063621328));
#32653=CARTESIAN_POINT('Ctrl Pts',(2.31729350216908,-0.986727046111983,
102.82557694532));
#32654=CARTESIAN_POINT('Ctrl Pts',(2.35224131080748,-0.897326164255197,
102.831741764531));
#32655=CARTESIAN_POINT('Ctrl Pts',(2.35952910329158,-0.877983987129867,
102.833061280816));
#32656=CARTESIAN_POINT('Ctrl Pts',(2.37093102798794,-0.846554919300016,
102.835182907652));
#32657=CARTESIAN_POINT('Ctrl Pts',(2.37519275210273,-0.834522960119893,
102.835989860898));
#32658=CARTESIAN_POINT('Ctrl Pts',(2.38318807275546,-0.811392602715328,
102.837531271266));
#32659=CARTESIAN_POINT('Ctrl Pts',(2.38693609781429,-0.800299580314415,
102.838266185632));
#32660=CARTESIAN_POINT('Ctrl Pts',(2.39532634855802,-0.774883613867455,
102.839940333077));
#32661=CARTESIAN_POINT('Ctrl Pts',(2.39991777942336,-0.760544277904604,
102.840877888933));
#32662=CARTESIAN_POINT('Ctrl Pts',(2.41406377516442,-0.714961352578325,
102.843836904041));
#32663=CARTESIAN_POINT('Ctrl Pts',(2.4231391695579,-0.683571767506233,102.845842878585));
#32664=CARTESIAN_POINT('Ctrl Pts',(2.47888434173951,-0.475677175089883,
102.858939292507));
#32665=CARTESIAN_POINT('Ctrl Pts',(2.50684786037321,-0.294718525591058,
102.869394955126));
#32666=CARTESIAN_POINT('Ctrl Pts',(2.52160117602881,0.0356550025147606,
102.88840324135));
#32667=CARTESIAN_POINT('Ctrl Pts',(2.5151369975468,0.183895567378174,102.896924479903));
#32668=CARTESIAN_POINT('Ctrl Pts',(2.49332445685361,0.348515283333323,102.907174362191));
#32669=CARTESIAN_POINT('Ctrl Pts',(2.49077096611955,0.366319125114966,102.908293509865));
#32670=CARTESIAN_POINT('Ctrl Pts',(2.48673761854896,0.392445779545791,102.9099534585));
#32671=CARTESIAN_POINT('Ctrl Pts',(2.48540619074844,0.400791386509681,102.910486346817));
#32672=CARTESIAN_POINT('Ctrl Pts',(2.48297226810997,0.415568948198591,102.911434888883));
#32673=CARTESIAN_POINT('Ctrl Pts',(2.48188675281953,0.422003530456306,102.911849590931));
#32674=CARTESIAN_POINT('Ctrl Pts',(2.4794782033649,0.435949839461696,102.912752124723));
#32675=CARTESIAN_POINT('Ctrl Pts',(2.47814606783039,0.443459678349607,102.91324043773));
#32676=CARTESIAN_POINT('Ctrl Pts',(2.4743553013391,0.464279322736735,102.914600404419));
#32677=CARTESIAN_POINT('Ctrl Pts',(2.47182346836101,0.477575301788284,102.915475968119));
#32678=CARTESIAN_POINT('Ctrl Pts',(2.45715687160118,0.55135455191865,102.920371306461));
#32679=CARTESIAN_POINT('Ctrl Pts',(2.4429102956263,0.611391593122609,102.924492378826));
#32680=CARTESIAN_POINT('Ctrl Pts',(2.41832586866082,0.700315277299747,102.930746284369));
#32681=CARTESIAN_POINT('Ctrl Pts',(2.40964051525969,0.729639626790019,102.93283360638));
#32682=CARTESIAN_POINT('Ctrl Pts',(2.38845956461168,0.79664464058407,102.937651241461));
#32683=CARTESIAN_POINT('Ctrl Pts',(2.37560253685304,0.834202769407093,102.940387134229));
#32684=CARTESIAN_POINT('Ctrl Pts',(2.32808391915122,0.96299235943133,102.949864906768));
#32685=CARTESIAN_POINT('Ctrl Pts',(2.28900872840419,1.05250626518966,102.956618001894));
#32686=CARTESIAN_POINT('Ctrl Pts',(2.20789218951705,1.21230330659508,102.96883600389));
#32687=CARTESIAN_POINT('Ctrl Pts',(2.16743014891732,1.28324428050476,102.974324647245));
#32688=CARTESIAN_POINT('Ctrl Pts',(2.10494478236901,1.38138294537662,102.981988990236));
#32689=CARTESIAN_POINT('Ctrl Pts',(2.0856956596084,1.41027840716407,102.984255345133));
#32690=CARTESIAN_POINT('Ctrl Pts',(2.05025860344977,1.46116069627317,102.988264450922));
#32691=CARTESIAN_POINT('Ctrl Pts',(2.03429941089601,1.4832993372348,102.990015219669));
#32692=CARTESIAN_POINT('Ctrl Pts',(2.00950821673279,1.5165368083286,102.992654513098));
#32693=CARTESIAN_POINT('Ctrl Pts',(2.00093760430525,1.52782717647838,102.993552997161));
#32694=CARTESIAN_POINT('Ctrl Pts',(1.9858678342209,1.5473347835457,102.995109033521));
#32695=CARTESIAN_POINT('Ctrl Pts',(1.97941196298716,1.55558486541144,102.995768253427));
#32696=CARTESIAN_POINT('Ctrl Pts',(1.96478871033027,1.57403376246048,102.997245131064));
#32697=CARTESIAN_POINT('Ctrl Pts',(1.95659300885593,1.58420982497115,102.998061643811));
#32698=CARTESIAN_POINT('Ctrl Pts',(1.93435331534736,1.61138752724046,103.00024782837));
#32699=CARTESIAN_POINT('Ctrl Pts',(1.9201643499337,1.62826945817043,103.0016116579));
#32700=CARTESIAN_POINT('Ctrl Pts',(1.85188088878139,1.70737855336194,103.008034207367));
#32701=CARTESIAN_POINT('Ctrl Pts',(1.79496974808412,1.76711346006148,103.012975902951));
#32702=CARTESIAN_POINT('Ctrl Pts',(1.60296239432799,1.94978046202481,103.028585409076));
#32703=CARTESIAN_POINT('Ctrl Pts',(1.45741348575376,2.06084339030448,103.038839083895));
#32704=CARTESIAN_POINT('Ctrl Pts',(1.24940878521563,2.18642063792493,103.05302422054));
#32705=CARTESIAN_POINT('Ctrl Pts',(1.1965749310008,2.21577638896681,103.056595815593));
#32706=CARTESIAN_POINT('Ctrl Pts',(1.12177728622576,2.25388008633242,103.061678696079));
#32707=CARTESIAN_POINT('Ctrl Pts',(1.10066669833238,2.26426422060688,103.063116142953));
#32708=CARTESIAN_POINT('Ctrl Pts',(1.06359804418931,2.28185712923467,103.065650488227));
#32709=CARTESIAN_POINT('Ctrl Pts',(1.04770424088273,2.28919823123452,103.06674037892));
#32710=CARTESIAN_POINT('Ctrl Pts',(1.02411018956133,2.29979878590641,103.068364944057));
#32711=CARTESIAN_POINT('Ctrl Pts',(1.01646780542663,2.30318677745033,103.068892179867));
#32712=CARTESIAN_POINT('Ctrl Pts',(1.0028367834599,2.3091485711002,103.069834619553));
#32713=CARTESIAN_POINT('Ctrl Pts',(0.996854843031237,2.31173725973907,103.070248918987));
#32714=CARTESIAN_POINT('Ctrl Pts',(0.983790943167309,2.31733053511908,103.0711553096));
#32715=CARTESIAN_POINT('Ctrl Pts',(0.976705348806667,2.32032585787243,103.071647918837));
#32716=CARTESIAN_POINT('Ctrl Pts',(0.956847061234565,2.32861355819018,103.073031089374));
#32717=CARTESIAN_POINT('Ctrl Pts',(0.944044559690628,2.33383316690007,103.073925771448));
#32718=CARTESIAN_POINT('Ctrl Pts',(0.869170460330283,2.36364263600486,103.07917273897));
#32719=CARTESIAN_POINT('Ctrl Pts',(0.806188476133523,2.38585881677424,103.083643654219));
#32720=CARTESIAN_POINT('Ctrl Pts',(0.53058432282325,2.47091640141351,103.103243642836));
#32721=CARTESIAN_POINT('Ctrl Pts',(0.311012600706783,2.50803561483774,103.118838266533));
#32722=CARTESIAN_POINT('Ctrl Pts',(0.0430231587831401,2.51756045804307,
103.136699712326));
#32723=CARTESIAN_POINT('Ctrl Pts',(-0.00341280010986838,2.51792582277355,
103.139757752228));
#32724=CARTESIAN_POINT('Ctrl Pts',(-0.0840253450051838,2.51632975651196,
103.145002104969));
#32725=CARTESIAN_POINT('Ctrl Pts',(-0.118199842720637,2.5149561998046,103.147205316341));
#32726=CARTESIAN_POINT('Ctrl Pts',(-0.167805709718507,2.51194897418758,
103.150375681418));
#32727=CARTESIAN_POINT('Ctrl Pts',(-0.183265536838815,2.51086840866851,
103.151359830341));
#32728=CARTESIAN_POINT('Ctrl Pts',(-0.210413127081642,2.50871885181465,
103.153081410469));
#32729=CARTESIAN_POINT('Ctrl Pts',(-0.222105103615359,2.50771076720999,
103.153820711617));
#32730=CARTESIAN_POINT('Ctrl Pts',(-0.244871979625545,2.50558732584508,
103.155256259153));
#32731=CARTESIAN_POINT('Ctrl Pts',(-0.255947355615494,2.50448020382286,
103.15595274391));
#32732=CARTESIAN_POINT('Ctrl Pts',(-0.285734991922991,2.50130289713291,
103.157821161271));
#32733=CARTESIAN_POINT('Ctrl Pts',(-0.304432209953688,2.49909618228299,
103.158988822031));
#32734=CARTESIAN_POINT('Ctrl Pts',(-0.374995315988209,2.48996438536853,
103.163377928873));
#32735=CARTESIAN_POINT('Ctrl Pts',(-0.426667793213562,2.48163238620764,
103.166555579521));
#32736=CARTESIAN_POINT('Ctrl Pts',(-0.688858428111269,2.43092259228202,
103.182559213639));
#32737=CARTESIAN_POINT('Ctrl Pts',(-0.893575907568189,2.36335167336494,
103.194568682619));
#32738=CARTESIAN_POINT('Ctrl Pts',(-1.14447771162261,2.24321308626393,103.210779304644));
#32739=CARTESIAN_POINT('Ctrl Pts',(-1.20065933392525,2.21365089432038,103.214522779327));
#32740=CARTESIAN_POINT('Ctrl Pts',(-1.27671698230111,2.16988253611406,103.219830309439));
#32741=CARTESIAN_POINT('Ctrl Pts',(-1.29759653687485,2.15746138122721,103.221313339242));
#32742=CARTESIAN_POINT('Ctrl Pts',(-1.33358240917717,2.13534220311773,103.223920738389));
#32743=CARTESIAN_POINT('Ctrl Pts',(-1.3487711160743,2.12578098599448,103.225037534022));
#32744=CARTESIAN_POINT('Ctrl Pts',(-1.37095325482857,2.11148400967517,103.226694640719));
#32745=CARTESIAN_POINT('Ctrl Pts',(-1.37802753581731,2.10687390598048,103.227227077759));
#32746=CARTESIAN_POINT('Ctrl Pts',(-1.39052710240531,2.09863841668815,103.228175129535));
#32747=CARTESIAN_POINT('Ctrl Pts',(-1.39596166328973,2.09502741265236,103.228589796338));
#32748=CARTESIAN_POINT('Ctrl Pts',(-1.40772264917479,2.08714672313838,103.229492624206));
#32749=CARTESIAN_POINT('Ctrl Pts',(-1.41404361611555,2.08286945077209,103.229981269393));
#32750=CARTESIAN_POINT('Ctrl Pts',(-1.4315385735023,2.07091462077226,103.231343025565));
#32751=CARTESIAN_POINT('Ctrl Pts',(-1.44266995044122,2.06317557391335,103.232220062645));
#32752=CARTESIAN_POINT('Ctrl Pts',(-1.50433122448289,2.0195628276572,103.237135299966));
#32753=CARTESIAN_POINT('Ctrl Pts',(-1.55358165593755,1.9819256114295,103.241275710444));
#32754=CARTESIAN_POINT('Ctrl Pts',(-1.73853897458603,1.82944863505302,103.257526741096));
#32755=CARTESIAN_POINT('Ctrl Pts',(-1.86333045345889,1.70217638075084,103.269987037853));
#32756=CARTESIAN_POINT('Ctrl Pts',(-2.04409315011653,1.47389109263844,103.289774592164));
#32757=CARTESIAN_POINT('Ctrl Pts',(-2.10842329333798,1.38030041793534,103.297316178222));
#32758=CARTESIAN_POINT('Ctrl Pts',(-2.17801818550521,1.26276619749444,103.306112166897));
#32759=CARTESIAN_POINT('Ctrl Pts',(-2.18953308782272,1.2426932854245,103.307592387349));
#32760=CARTESIAN_POINT('Ctrl Pts',(-2.20722906075781,1.21083568632134,103.309907934));
#32761=CARTESIAN_POINT('Ctrl Pts',(-2.21359603568314,1.19915628162888,103.310749830178));
#32762=CARTESIAN_POINT('Ctrl Pts',(-2.22534539612983,1.17719109089835,103.312320289976));
#32763=CARTESIAN_POINT('Ctrl Pts',(-2.23074976104873,1.16691752382361,103.313049613013));
#32764=CARTESIAN_POINT('Ctrl Pts',(-2.24269275756942,1.14382797361972,103.314677302977));
#32765=CARTESIAN_POINT('Ctrl Pts',(-2.24919300793412,1.13099251311799,103.315574312901));
#32766=CARTESIAN_POINT('Ctrl Pts',(-2.2654581616758,1.09818029223132,103.31784805539));
#32767=CARTESIAN_POINT('Ctrl Pts',(-2.27506922062494,1.0781283440497,103.319219482253));
#32768=CARTESIAN_POINT('Ctrl Pts',(-2.31255454723068,0.997187001461094,
103.324686558703));
#32769=CARTESIAN_POINT('Ctrl Pts',(-2.33824458908796,0.93535725801648,103.328707268518));
#32770=CARTESIAN_POINT('Ctrl Pts',(-2.36143100149827,0.872610952923958,
103.332666057199));
#32771=CARTESIAN_POINT('Origin',(0.,0.,104.));
#32772=CARTESIAN_POINT('',(-2.36143112095504,0.87261062965393,104.32884037888));
#32773=CARTESIAN_POINT('',(-2.36143112101026,0.872610629504495,104.05635151795));
#32774=CARTESIAN_POINT('',(-2.36143112101026,0.872610629504505,104.));
#32775=CARTESIAN_POINT('',(-2.51749898433586,0.00226138628059867,103.112583302554));
#32776=CARTESIAN_POINT('Ctrl Pts',(-2.36143112101026,0.872610629504494,
104.05635151795));
#32777=CARTESIAN_POINT('Ctrl Pts',(-2.33167841640509,0.953126452041245,
104.050918934233));
#32778=CARTESIAN_POINT('Ctrl Pts',(-2.29784078860177,1.03201888497832,104.045486350517));
#32779=CARTESIAN_POINT('Ctrl Pts',(-2.26013251530705,1.10887657710488,104.0400537668));
#32780=CARTESIAN_POINT('Ctrl Pts',(-2.22999407261371,1.17030530208506,104.035711759099));
#32781=CARTESIAN_POINT('Ctrl Pts',(-2.19738399262468,1.23043463114403,104.031369751399));
#32782=CARTESIAN_POINT('Ctrl Pts',(-2.16243151429358,1.28906795631184,104.027027743698));
#32783=CARTESIAN_POINT('Ctrl Pts',(-2.12012758401577,1.36003345627892,104.021772494291));
#32784=CARTESIAN_POINT('Ctrl Pts',(-2.07424846759187,1.42904534370445,104.016517244883));
#32785=CARTESIAN_POINT('Ctrl Pts',(-2.02500000847352,1.49572096852395,104.011261995476));
#32786=CARTESIAN_POINT('Ctrl Pts',(-1.97582137248236,1.56230206245426,104.006014196819));
#32787=CARTESIAN_POINT('Ctrl Pts',(-1.92328315409511,1.62655310489617,104.000766398161));
#32788=CARTESIAN_POINT('Ctrl Pts',(-1.86763593960146,1.68811796006943,103.995518599504));
#32789=CARTESIAN_POINT('Ctrl Pts',(-1.81158551306518,1.75012890569366,103.990232776021));
#32790=CARTESIAN_POINT('Ctrl Pts',(-1.75238108825241,1.80941416526036,103.984946952538));
#32791=CARTESIAN_POINT('Ctrl Pts',(-1.69032191607632,1.86564146342004,103.979661129055));
#32792=CARTESIAN_POINT('Ctrl Pts',(-1.62881922421346,1.92136457527826,103.974422703186));
#32793=CARTESIAN_POINT('Ctrl Pts',(-1.56451312482664,1.97408403161967,103.969184277318));
#32794=CARTESIAN_POINT('Ctrl Pts',(-1.49773256054301,2.023512645646,103.963945851449));
#32795=CARTESIAN_POINT('Ctrl Pts',(-1.43097395927558,2.07292500342379,103.958709148412));
#32796=CARTESIAN_POINT('Ctrl Pts',(-1.36174287997084,2.11904839410438,103.953472445374));
#32797=CARTESIAN_POINT('Ctrl Pts',(-1.29040036014548,2.16163668560108,103.948235742337));
#32798=CARTESIAN_POINT('Ctrl Pts',(-1.21905978365467,2.20422381701402,103.942999181944));
#32799=CARTESIAN_POINT('Ctrl Pts',(-1.1456082777217,2.2432758050749,103.937762621552));
#32800=CARTESIAN_POINT('Ctrl Pts',(-1.07043360185127,2.27859126523993,103.93252606116));
#32801=CARTESIAN_POINT('Ctrl Pts',(-0.994028519174909,2.31448474429283,
103.927203792389));
#32802=CARTESIAN_POINT('Ctrl Pts',(-0.915843789831181,2.34651805717611,
103.921881523619));
#32803=CARTESIAN_POINT('Ctrl Pts',(-0.836308278398951,2.37453041957381,
103.916559254848));
#32804=CARTESIAN_POINT('Ctrl Pts',(-0.757941201789924,2.40213125988388,
103.911315174098));
#32805=CARTESIAN_POINT('Ctrl Pts',(-0.678263233698182,2.42582843231033,
103.906071093348));
#32806=CARTESIAN_POINT('Ctrl Pts',(-0.597698758545896,2.44551884965802,
103.900827012597));
#32807=CARTESIAN_POINT('Ctrl Pts',(-0.515332487109612,2.46564963629678,
103.895465649817));
#32808=CARTESIAN_POINT('Ctrl Pts',(-0.43204008019191,2.48159218961269,103.890104287036));
#32809=CARTESIAN_POINT('Ctrl Pts',(-0.348282757392524,2.49329207492886,
103.884742924256));
#32810=CARTESIAN_POINT('Ctrl Pts',(-0.264525434593138,2.50499196024503,
103.879381561475));
#32811=CARTESIAN_POINT('Ctrl Pts',(-0.180303707930204,2.51244919928506,
103.874020198695));
#32812=CARTESIAN_POINT('Ctrl Pts',(-0.0960789567654115,2.515665932525,103.868658835914));
#32813=CARTESIAN_POINT('Ctrl Pts',(-0.0135212020010645,2.51881899941202,
103.863403586507));
#32814=CARTESIAN_POINT('Ctrl Pts',(0.0693443933134434,2.5179095803437,103.858148337099));
#32815=CARTESIAN_POINT('Ctrl Pts',(0.152084793467522,2.51290200079429,103.852893087692));
#32816=CARTESIAN_POINT('Ctrl Pts',(0.234707886530424,2.5079015208551,103.847645289035));
#32817=CARTESIAN_POINT('Ctrl Pts',(0.317205680260782,2.49881444895048,103.842397490377));
#32818=CARTESIAN_POINT('Ctrl Pts',(0.39914301861702,2.48565707624549,103.83714969172));
#32819=CARTESIAN_POINT('Ctrl Pts',(0.48167406362809,2.47240436703224,103.831863868237));
#32820=CARTESIAN_POINT('Ctrl Pts',(0.563636023487427,2.45502210436827,103.826578044754));
#32821=CARTESIAN_POINT('Ctrl Pts',(0.644587260568504,2.43358038977815,103.821292221271));
#32822=CARTESIAN_POINT('Ctrl Pts',(0.724812613494425,2.41233094156273,103.816053795402));
#32823=CARTESIAN_POINT('Ctrl Pts',(0.804044842948165,2.38709467180903,103.810815369534));
#32824=CARTESIAN_POINT('Ctrl Pts',(0.881863965532047,2.35799113575435,103.805576943665));
#32825=CARTESIAN_POINT('Ctrl Pts',(0.959657494701617,2.32889717136832,103.800340240628));
#32826=CARTESIAN_POINT('Ctrl Pts',(1.03603840817087,2.29593862820904,103.79510353759));
#32827=CARTESIAN_POINT('Ctrl Pts',(1.11060368480481,2.25928433476134,103.789866834553));
#32828=CARTESIAN_POINT('Ctrl Pts',(1.1851669303178,2.22263103975831,103.78463027416));
#32829=CARTESIAN_POINT('Ctrl Pts',(1.25791422369009,2.18228239910811,103.779393713768));
#32830=CARTESIAN_POINT('Ctrl Pts',(1.32846552885237,2.13845401836256,103.774157153376));
#32831=CARTESIAN_POINT('Ctrl Pts',(1.40017156870476,2.09390828516632,103.768834884605));
#32832=CARTESIAN_POINT('Ctrl Pts',(1.46960866236069,2.04576812457823,103.763512615835));
#32833=CARTESIAN_POINT('Ctrl Pts',(1.53640844918693,1.9943057256266,103.758190347064));
#32834=CARTESIAN_POINT('Ctrl Pts',(1.60222689829729,1.94359934694748,103.752946266314));
#32835=CARTESIAN_POINT('Ctrl Pts',(1.66548469781709,1.88966804453295,103.747702185564));
#32836=CARTESIAN_POINT('Ctrl Pts',(1.72586432224121,1.83281166277796,103.742458104813));
#32837=CARTESIAN_POINT('Ctrl Pts',(1.78759431582893,1.7746837079483,103.737096742033));
#32838=CARTESIAN_POINT('Ctrl Pts',(1.8463154875255,1.71349862765116,103.731735379252));
#32839=CARTESIAN_POINT('Ctrl Pts',(1.90173106621282,1.64961365228379,103.726374016472));
#32840=CARTESIAN_POINT('Ctrl Pts',(1.95714664490014,1.58572867691641,103.721012653691));
#32841=CARTESIAN_POINT('Ctrl Pts',(2.00925637003074,1.51914424778308,103.715651290911));
#32842=CARTESIAN_POINT('Ctrl Pts',(2.0578108383057,1.45024853171848,103.71028992813));
#32843=CARTESIAN_POINT('Ctrl Pts',(2.10540430494247,1.38271641612886,103.705034678723));
#32844=CARTESIAN_POINT('Ctrl Pts',(2.14975779396932,1.31271425944062,103.699779429315));
#32845=CARTESIAN_POINT('Ctrl Pts',(2.19060561490067,1.24058586561578,103.694524179908));
#32846=CARTESIAN_POINT('Ctrl Pts',(2.23139552290158,1.16855973346755,103.689276381251));
#32847=CARTESIAN_POINT('Ctrl Pts',(2.26868940967196,1.09441375005787,103.684028582593));
#32848=CARTESIAN_POINT('Ctrl Pts',(2.30226401872926,1.01852179066753,103.678780783936));
#32849=CARTESIAN_POINT('Ctrl Pts',(2.33608190477382,0.942079928605025,103.673494960453));
#32850=CARTESIAN_POINT('Ctrl Pts',(2.36612611394342,0.863867068954772,103.66820913697));
#32851=CARTESIAN_POINT('Ctrl Pts',(2.39221499656092,0.784291820835234,103.662923313487));
#32852=CARTESIAN_POINT('Ctrl Pts',(2.41806994196878,0.705430118472858,103.657684887618));
#32853=CARTESIAN_POINT('Ctrl Pts',(2.44004006460321,0.625230809207092,103.65244646175));
#32854=CARTESIAN_POINT('Ctrl Pts',(2.45799698585843,0.544111263907379,103.647208035881));
#32855=CARTESIAN_POINT('Ctrl Pts',(2.4759480013811,0.463018397476046,103.641971332844));
#32856=CARTESIAN_POINT('Ctrl Pts',(2.48988833722011,0.381006346250213,103.636734629806));
#32857=CARTESIAN_POINT('Ctrl Pts',(2.49974017991996,0.298505080180794,103.631497926769));
#32858=CARTESIAN_POINT('Ctrl Pts',(2.50959175426053,0.216006061404678,103.626261366376));
#32859=CARTESIAN_POINT('Ctrl Pts',(2.5153550032034,0.133018312568258,103.621024805984));
#32860=CARTESIAN_POINT('Ctrl Pts',(2.51700386379089,0.0499779917738332,
103.615788245592));
#32861=CARTESIAN_POINT('Ctrl Pts',(2.51867971178159,-0.0344214752316504,
103.610465976821));
#32862=CARTESIAN_POINT('Ctrl Pts',(2.51610525050778,-0.118874759276591,
103.605143708051));
#32863=CARTESIAN_POINT('Ctrl Pts',(2.50930823550474,-0.202924688562287,
103.59982143928));
#32864=CARTESIAN_POINT('Ctrl Pts',(2.5026110736224,-0.285739862925301,103.59457735853));
#32865=CARTESIAN_POINT('Ctrl Pts',(2.49181472092363,-0.36816299892866,103.589333277779));
#32866=CARTESIAN_POINT('Ctrl Pts',(2.47699780731675,-0.449764507879434,
103.584089197029));
#32867=CARTESIAN_POINT('Ctrl Pts',(2.46184951862391,-0.533191006012152,
103.578727834249));
#32868=CARTESIAN_POINT('Ctrl Pts',(2.44249877889859,-0.615758184288129,
103.573366471468));
#32869=CARTESIAN_POINT('Ctrl Pts',(2.41908365274352,-0.697022618735634,
103.568005108687));
#32870=CARTESIAN_POINT('Ctrl Pts',(2.39566852658844,-0.778287053183139,
103.562643745907));
#32871=CARTESIAN_POINT('Ctrl Pts',(2.36818924231077,-0.858248284988129,
103.557282383126));
#32872=CARTESIAN_POINT('Ctrl Pts',(2.33683560324135,-0.936485778548516,
103.551921020346));
#32873=CARTESIAN_POINT('Ctrl Pts',(2.3061025228883,-1.01317477694163,103.546665770938));
#32874=CARTESIAN_POINT('Ctrl Pts',(2.27153358025019,-1.08849092484336,103.541410521531));
#32875=CARTESIAN_POINT('Ctrl Pts',(2.23327249983834,-1.16202417852032,103.536155272124));
#32876=CARTESIAN_POINT('Ctrl Pts',(2.19506566494663,-1.23545317874833,103.530907473466));
#32877=CARTESIAN_POINT('Ctrl Pts',(2.15317730095472,-1.30710389966781,103.525659674809));
#32878=CARTESIAN_POINT('Ctrl Pts',(2.10779945922329,-1.37658551848332,103.520411876151));
#32879=CARTESIAN_POINT('Ctrl Pts',(2.06209281590823,-1.44657059152734,103.515126052668));
#32880=CARTESIAN_POINT('Ctrl Pts',(2.01284608921407,-1.51435455592313,103.509840229185));
#32881=CARTESIAN_POINT('Ctrl Pts',(1.96030311786674,-1.57956257745046,103.504554405702));
#32882=CARTESIAN_POINT('Ctrl Pts',(1.90823129571663,-1.64418588314982,103.499315979834));
#32883=CARTESIAN_POINT('Ctrl Pts',(1.85292240139199,-1.70627889164413,103.494077553965));
#32884=CARTESIAN_POINT('Ctrl Pts',(1.79465662642586,-1.76550668172787,103.488839128097));
#32885=CARTESIAN_POINT('Ctrl Pts',(1.73641001410332,-1.82471499277725,103.483602425059));
#32886=CARTESIAN_POINT('Ctrl Pts',(1.67520877585189,-1.88105962824586,103.478365722021));
#32887=CARTESIAN_POINT('Ctrl Pts',(1.61137120149195,-1.9342412209966,103.473129018984));
#32888=CARTESIAN_POINT('Ctrl Pts',(1.54753536603575,-1.98742136510721,103.467892458592));
#32889=CARTESIAN_POINT('Ctrl Pts',(1.48106369243062,-2.03743834325917,103.462655898199));
#32890=CARTESIAN_POINT('Ctrl Pts',(1.41230783670988,-2.08403282708499,103.457419337807));
#32891=CARTESIAN_POINT('Ctrl Pts',(1.34242663296675,-2.13138993701266,103.452097069036));
#32892=CARTESIAN_POINT('Ctrl Pts',(1.27018620039215,-2.17521122109078,103.446774800266));
#32893=CARTESIAN_POINT('Ctrl Pts',(1.19598512270835,-2.21527105254871,103.441452531495));
#32894=CARTESIAN_POINT('Ctrl Pts',(1.12287411311507,-2.25474237578889,103.436208450745));
#32895=CARTESIAN_POINT('Ctrl Pts',(1.04786013143435,-2.29056188349983,103.430964369995));
#32896=CARTESIAN_POINT('Ctrl Pts',(0.971346323523955,-2.32256163960755,
103.425720289244));
#32897=CARTESIAN_POINT('Ctrl Pts',(0.893121311084641,-2.35527705905854,
103.420358926464));
#32898=CARTESIAN_POINT('Ctrl Pts',(0.813329058486849,-2.38399963696721,
103.414997563683));
#32899=CARTESIAN_POINT('Ctrl Pts',(0.732416675825609,-2.40860375798357,
103.409636200903));
#32900=CARTESIAN_POINT('Ctrl Pts',(0.651504293164368,-2.43320787899992,
103.404274838122));
#32901=CARTESIAN_POINT('Ctrl Pts',(0.569472289591547,-2.45369348482422,
103.398913475341));
#32902=CARTESIAN_POINT('Ctrl Pts',(0.486776745845593,-2.46999081976107,
103.393552112561));
#32903=CARTESIAN_POINT('Ctrl Pts',(0.405717932061407,-2.48596559395063,
103.388296863154));
#32904=CARTESIAN_POINT('Ctrl Pts',(0.323722213469075,-2.49797542585536,
103.383041613746));
#32905=CARTESIAN_POINT('Ctrl Pts',(0.241211782623291,-2.50591762153581,
103.377786364339));
#32906=CARTESIAN_POINT('Ctrl Pts',(0.158818332824318,-2.51384855698704,
103.372538565681));
#32907=CARTESIAN_POINT('Ctrl Pts',(0.0759120757246245,-2.51772326728586,
103.367290767024));
#32908=CARTESIAN_POINT('Ctrl Pts',(-0.00707460686697792,-2.51749005955092,
103.362042968367));
#32909=CARTESIAN_POINT('Ctrl Pts',(-0.0906625995170283,-2.51725516202488,
103.356757144884));
#32910=CARTESIAN_POINT('Ctrl Pts',(-0.174331723136054,-2.51285247283201,
103.351471321401));
#32911=CARTESIAN_POINT('Ctrl Pts',(-0.257634811296941,-2.50428244293809,
103.346185497918));
#32912=CARTESIAN_POINT('Ctrl Pts',(-0.340190926416332,-2.49578925991069,
103.340947072049));
#32913=CARTESIAN_POINT('Ctrl Pts',(-0.422387076759521,-2.48320322145352,
103.335708646181));
#32914=CARTESIAN_POINT('Ctrl Pts',(-0.503789782285635,-2.46657700168971,
103.330470220312));
#32915=CARTESIAN_POINT('Ctrl Pts',(-0.585165715816659,-2.44995625001287,
103.325233517275));
#32916=CARTESIAN_POINT('Ctrl Pts',(-0.665748271062551,-2.42929804826103,
103.319996814237));
#32917=CARTESIAN_POINT('Ctrl Pts',(-0.745113047788685,-2.40470638457485,
103.3147601112));
#32918=CARTESIAN_POINT('Ctrl Pts',(-0.824475662658091,-2.38011539075326,
103.309523550807));
#32919=CARTESIAN_POINT('Ctrl Pts',(-0.902620124519449,-2.35159128558332,
103.304286990415));
#32920=CARTESIAN_POINT('Ctrl Pts',(-0.979137451062491,-2.31928784369833,
103.299050430023));
#32921=CARTESIAN_POINT('Ctrl Pts',(-1.05690715998365,-2.28645568154569,
103.293728161252));
#32922=CARTESIAN_POINT('Ctrl Pts',(-1.13299553128059,-2.24971953054689,
103.288405892482));
#32923=CARTESIAN_POINT('Ctrl Pts',(-1.20699630142899,-2.20929087680566,
103.283083623711));
#32924=CARTESIAN_POINT('Ctrl Pts',(-1.27990994615088,-2.16945614955134,
103.277839542961));
#32925=CARTESIAN_POINT('Ctrl Pts',(-1.35079655230355,-2.12603698732565,
103.272595462211));
#32926=CARTESIAN_POINT('Ctrl Pts',(-1.41929576301218,-2.07928011270624,
103.26735138146));
#32927=CARTESIAN_POINT('Ctrl Pts',(-1.48932693458919,-2.03147753695387,
103.26199001868));
#32928=CARTESIAN_POINT('Ctrl Pts',(-1.55686222783535,-1.98018646343684,
103.256628655899));
#32929=CARTESIAN_POINT('Ctrl Pts',(-1.62155284777497,-1.92571353318007,
103.251267293119));
#32930=CARTESIAN_POINT('Ctrl Pts',(-1.68624346771459,-1.87124060292331,
103.245905930338));
#32931=CARTESIAN_POINT('Ctrl Pts',(-1.74808908823779,-1.81358621125809,
103.240544567558));
#32932=CARTESIAN_POINT('Ctrl Pts',(-1.80678288493539,-1.75309493659201,
103.235183204777));
#32933=CARTESIAN_POINT('Ctrl Pts',(-1.86353796867853,-1.69460174731868,
103.229998933002));
#32934=CARTESIAN_POINT('Ctrl Pts',(-1.91756794793409,-1.63322734809459,
103.224814661227));
#32935=CARTESIAN_POINT('Ctrl Pts',(-1.96856067929322,-1.5692594119331,103.219630389452));
#32936=CARTESIAN_POINT('Ctrl Pts',(-2.01948810385429,-1.50537340001803,
103.214452757215));
#32937=CARTESIAN_POINT('Ctrl Pts',(-2.06738570242004,-1.4389008061749,103.209275124979));
#32938=CARTESIAN_POINT('Ctrl Pts',(-2.11197797192584,-1.37016615638397,
103.204097492742));
#32939=CARTESIAN_POINT('Ctrl Pts',(-2.1565274487315,-1.30149746738154,103.198924829188));
#32940=CARTESIAN_POINT('Ctrl Pts',(-2.19777763273914,-1.23057142519621,
103.193752165635));
#32941=CARTESIAN_POINT('Ctrl Pts',(-2.23549414426031,-1.15774443681577,
103.188579502081));
#32942=CARTESIAN_POINT('Ctrl Pts',(-2.2731865640472,-1.08496396727765,103.18341014261));
#32943=CARTESIAN_POINT('Ctrl Pts',(-2.30734957417599,-1.01028538234433,
103.178240783138));
#32944=CARTESIAN_POINT('Ctrl Pts',(-2.33779370789912,-0.93409144590199,
103.173071423666));
#32945=CARTESIAN_POINT('Ctrl Pts',(-2.36823897829903,-0.857894664646306,
103.167901871188));
#32946=CARTESIAN_POINT('Ctrl Pts',(-2.39496490115959,-0.780182852656354,
103.162732318711));
#32947=CARTESIAN_POINT('Ctrl Pts',(-2.41782980818628,-0.701359585837319,
103.157562766234));
#32948=CARTESIAN_POINT('Ctrl Pts',(-2.44069380324843,-0.622539462876451,
103.152393419943));
#32949=CARTESIAN_POINT('Ctrl Pts',(-2.45969696387433,-0.542608431845804,
103.147224073653));
#32950=CARTESIAN_POINT('Ctrl Pts',(-2.47474785657926,-0.46198408669169,
103.142054727362));
#32951=CARTESIAN_POINT('Ctrl Pts',(-2.48981318905338,-0.381282390847674,
103.136880421621));
#32952=CARTESIAN_POINT('Ctrl Pts',(-2.50091860016243,-0.29988652146086,
103.131706115879));
#32953=CARTESIAN_POINT('Ctrl Pts',(-2.50802417071423,-0.218222384537388,
103.126531810138));
#32954=CARTESIAN_POINT('Ctrl Pts',(-2.51440905979744,-0.144841020925352,
103.12188230761));
#32955=CARTESIAN_POINT('Ctrl Pts',(-2.5175650112416,-0.0712433791665783,
103.117232805082));
#32956=CARTESIAN_POINT('Ctrl Pts',(-2.51749898433586,0.00226138628061706,
103.112583302554));
#32957=CARTESIAN_POINT('Ctrl Pts',(-2.51749898433498,0.00226138726559125,
103.112583302492));
#32958=CARTESIAN_POINT('Ctrl Pts',(-2.5173983212915,0.114324948237909,103.105494785076));
#32959=CARTESIAN_POINT('Ctrl Pts',(-2.50981145266269,0.226062019319086,
103.09840626766));
#32960=CARTESIAN_POINT('Ctrl Pts',(-2.49489001405843,0.33664531446545,103.091317750244));
#32961=CARTESIAN_POINT('Ctrl Pts',(-2.48471334971802,0.41206492420996,103.086483265827));
#32962=CARTESIAN_POINT('Ctrl Pts',(-2.47112602227995,0.486948560769381,
103.08164878141));
#32963=CARTESIAN_POINT('Ctrl Pts',(-2.45418827016786,0.561040270007863,
103.076814296993));
#32964=CARTESIAN_POINT('Ctrl Pts',(-2.43577686875584,0.641578241697638,
103.071559193917));
#32965=CARTESIAN_POINT('Ctrl Pts',(-2.41336280068244,0.721357683945833,
103.066304090841));
#32966=CARTESIAN_POINT('Ctrl Pts',(-2.38702415539055,0.79995120575071,103.061048987765));
#32967=CARTESIAN_POINT('Ctrl Pts',(-2.37886800041174,0.824288863859839,
103.059421666594));
#32968=CARTESIAN_POINT('Ctrl Pts',(-2.37033588202498,0.848512848576402,
103.057794345422));
#32969=CARTESIAN_POINT('Ctrl Pts',(-2.36143112101026,0.872610629504504,
103.05616702425));
#32970=CARTESIAN_POINT('Ctrl Pts',(-2.36143100149827,0.872610952923958,
103.332666057199));
#32971=CARTESIAN_POINT('Ctrl Pts',(-2.39387776714414,0.784804585105903,
103.338205934878));
#32972=CARTESIAN_POINT('Ctrl Pts',(-2.42142173855965,0.695203230517513,
103.343622852339));
#32973=CARTESIAN_POINT('Ctrl Pts',(-2.47308432792982,0.486240117551232,
103.356007258809));
#32974=CARTESIAN_POINT('Ctrl Pts',(-2.49366949579794,0.366312548876271,
103.362934183258));
#32975=CARTESIAN_POINT('Ctrl Pts',(-2.51219498632938,0.177149514409093,
103.374151232098));
#32976=CARTESIAN_POINT('Ctrl Pts',(-2.51608648166396,0.108685954016836,
103.378271619745));
#32977=CARTESIAN_POINT('Ctrl Pts',(-2.51739500684821,0.0266607260762851,
103.38336960666));
#32978=CARTESIAN_POINT('Ctrl Pts',(-2.51750175646071,0.0131644323603149,
103.384213655136));
#32979=CARTESIAN_POINT('Ctrl Pts',(-2.51749898494065,-0.00786943934477994,
103.385538157595));
#32980=CARTESIAN_POINT('Ctrl Pts',(-2.51746413837851,-0.0154070020419334,
103.386014610995));
#32981=CARTESIAN_POINT('Ctrl Pts',(-2.51734182315744,-0.0288272163592207,
103.386866318177));
#32982=CARTESIAN_POINT('Ctrl Pts',(-2.51726758336298,-0.0347098592457373,
103.387240835722));
#32983=CARTESIAN_POINT('Ctrl Pts',(-2.51704014568502,-0.0488135624563618,
103.388141547836));
#32984=CARTESIAN_POINT('Ctrl Pts',(-2.51686729162727,-0.0570341183803992,
103.388668810118));
#32985=CARTESIAN_POINT('Ctrl Pts',(-2.51621865873184,-0.0820501507030038,
103.390279931391));
#32986=CARTESIAN_POINT('Ctrl Pts',(-2.51561501371179,-0.0988414524631855,
103.391370414343));
#32987=CARTESIAN_POINT('Ctrl Pts',(-2.51381866011755,-0.137912167079226,
103.393926978865));
#32988=CARTESIAN_POINT('Ctrl Pts',(-2.51249776720093,-0.160184015435006,
103.395398855545));
#32989=CARTESIAN_POINT('Ctrl Pts',(-2.50683959371106,-0.238058532460376,
103.400589689845));
#32990=CARTESIAN_POINT('Ctrl Pts',(-2.50095106569157,-0.293529571549378,
103.404366174094));
#32991=CARTESIAN_POINT('Ctrl Pts',(-2.47018418420475,-0.513479547637946,
103.419549570944));
#32992=CARTESIAN_POINT('Ctrl Pts',(-2.43087166419543,-0.675529644001177,
103.431171483305));
#32993=CARTESIAN_POINT('Ctrl Pts',(-2.37335574321666,-0.839670302552693,
103.442949384595));
#32994=CARTESIAN_POINT('Ctrl Pts',(-2.37081691040832,-0.846812186781872,
103.443461942661));
#32995=CARTESIAN_POINT('Ctrl Pts',(-2.3356075428061,-0.944458614156251,
103.450470848504));
#32996=CARTESIAN_POINT('Ctrl Pts',(-2.29780380514396,-1.03303738765478,
103.456836237442));
#32997=CARTESIAN_POINT('Ctrl Pts',(-2.24490261732576,-1.13962099139342,
103.464497698606));
#32998=CARTESIAN_POINT('Ctrl Pts',(-2.23451276328894,-1.15986056553296,
103.465952919309));
#32999=CARTESIAN_POINT('Ctrl Pts',(-2.21759348130645,-1.19174811536402,
103.468246821602));
#33000=CARTESIAN_POINT('Ctrl Pts',(-2.2112434812625,-1.20348938364089,103.46909172047));
#33001=CARTESIAN_POINT('Ctrl Pts',(-2.19919929437049,-1.22534213934016,
103.470664938552));
#33002=CARTESIAN_POINT('Ctrl Pts',(-2.19352802346135,-1.23546578760557,
103.471394041815));
#33003=CARTESIAN_POINT('Ctrl Pts',(-2.18069997767442,-1.25799802660365,
103.473017634773));
#33004=CARTESIAN_POINT('Ctrl Pts',(-2.17350684911057,-1.27038553905599,
103.473910799068));
#33005=CARTESIAN_POINT('Ctrl Pts',(-2.15192767687599,-1.30682786656698,
103.476540582205));
#33006=CARTESIAN_POINT('Ctrl Pts',(-2.137244929362,-1.33070507902403,103.478266493266));
#33007=CARTESIAN_POINT('Ctrl Pts',(-2.03592203954007,-1.48947254348868,
103.489773361189));
#33008=CARTESIAN_POINT('Ctrl Pts',(-1.93696376566969,-1.61607151098729,
103.499068104887));
#33009=CARTESIAN_POINT('Ctrl Pts',(-1.70652830626777,-1.85903878799125,
103.518323913763));
#33010=CARTESIAN_POINT('Ctrl Pts',(-1.57360687543323,-1.97281731350898,
103.528226249721));
#33011=CARTESIAN_POINT('Ctrl Pts',(-1.41370660726907,-2.08317846930345,
103.540185219019));
#33012=CARTESIAN_POINT('Ctrl Pts',(-1.39726650007648,-2.09424095507144,
103.54141556868));
#33013=CARTESIAN_POINT('Ctrl Pts',(-1.37396967275914,-2.10952087815147,
103.543162743387));
#33014=CARTESIAN_POINT('Ctrl Pts',(-1.3672202161803,-2.11390157607166,103.543669355663));
#33015=CARTESIAN_POINT('Ctrl Pts',(-1.35488060431832,-2.12182671548781,
103.54459656563));
#33016=CARTESIAN_POINT('Ctrl Pts',(-1.34929718746911,-2.12538165075333,
103.545016481409));
#33017=CARTESIAN_POINT('Ctrl Pts',(-1.33771808202371,-2.13268999591267,
103.545888218649));
#33018=CARTESIAN_POINT('Ctrl Pts',(-1.33172053129223,-2.1364401955636,103.546340228764));
#33019=CARTESIAN_POINT('Ctrl Pts',(-1.31602757920993,-2.14616106367415,
103.547524031721));
#33020=CARTESIAN_POINT('Ctrl Pts',(-1.3063074618291,-2.15209123969874,103.548258352521));
#33021=CARTESIAN_POINT('Ctrl Pts',(-1.26295253481293,-2.17813984870985,
103.55153729419));
#33022=CARTESIAN_POINT('Ctrl Pts',(-1.22889272951616,-2.19753602221635,
103.554122828524));
#33023=CARTESIAN_POINT('Ctrl Pts',(-1.13123724558799,-2.25016807087677,
103.561534060052));
#33024=CARTESIAN_POINT('Ctrl Pts',(-1.06665563573238,-2.28149040835823,
103.566432224306));
#33025=CARTESIAN_POINT('Ctrl Pts',(-0.960599112610984,-2.3274401971895,
103.574383870678));
#33026=CARTESIAN_POINT('Ctrl Pts',(-0.919920804693266,-2.34381615501612,
103.577413000992));
#33027=CARTESIAN_POINT('Ctrl Pts',(-0.703194079703188,-2.42455268033462,
103.593390992463));
#33028=CARTESIAN_POINT('Ctrl Pts',(-0.520762904952517,-2.47017565024896,
103.606226448787));
#33029=CARTESIAN_POINT('Ctrl Pts',(-0.302801517057759,-2.49943362395204,
103.62050961445));
#33030=CARTESIAN_POINT('Ctrl Pts',(-0.270589889383164,-2.50312574016055,
103.622596096085));
#33031=CARTESIAN_POINT('Ctrl Pts',(-0.223372238297469,-2.50761567791858,
103.625620326093));
#33032=CARTESIAN_POINT('Ctrl Pts',(-0.208417147586175,-2.50890291830514,
103.626573182138));
#33033=CARTESIAN_POINT('Ctrl Pts',(-0.181783521121086,-2.51095558385689,
103.628261495969));
#33034=CARTESIAN_POINT('Ctrl Pts',(-0.170109588218879,-2.51177346273865,
103.628998564153));
#33035=CARTESIAN_POINT('Ctrl Pts',(-0.145669004281273,-2.51331460171821,
103.630535701862));
#33036=CARTESIAN_POINT('Ctrl Pts',(-0.13290166478888,-2.5140220570073,103.63133525981));
#33037=CARTESIAN_POINT('Ctrl Pts',(-0.0993813966819019,-2.51562339110421,
103.633425838072));
#33038=CARTESIAN_POINT('Ctrl Pts',(-0.0786215600205884,-2.51635776433888,
103.634711891664));
#33039=CARTESIAN_POINT('Ctrl Pts',(0.018637267882308,-2.51859345419065,
103.640699272084));
#33040=CARTESIAN_POINT('Ctrl Pts',(0.0951740369102882,-2.51686390333626,
103.645300077656));
#33041=CARTESIAN_POINT('Ctrl Pts',(0.305818486820041,-2.50247911687551,
103.657781794824));
#33042=CARTESIAN_POINT('Ctrl Pts',(0.439167412864043,-2.48255130475694,
103.665470898837));
#33043=CARTESIAN_POINT('Ctrl Pts',(0.700407224694442,-2.42179326969231,
103.680898401929));
#33044=CARTESIAN_POINT('Ctrl Pts',(0.827895161868327,-2.38122525506859,
103.688615973074));
#33045=CARTESIAN_POINT('Ctrl Pts',(0.97148404881323,-2.3226038801022,103.698138909585));
#33046=CARTESIAN_POINT('Ctrl Pts',(0.991316228323331,-2.31420874279741,
103.699473548711));
#33047=CARTESIAN_POINT('Ctrl Pts',(1.01877019545961,-2.30216959236784,103.701351459402));
#33048=CARTESIAN_POINT('Ctrl Pts',(1.02648565514014,-2.29873981524347,103.701882584412));
#33049=CARTESIAN_POINT('Ctrl Pts',(1.03976048072132,-2.29275855872406,103.702802481271));
#33050=CARTESIAN_POINT('Ctrl Pts',(1.04532812808651,-2.29022548422419,103.703190150617));
#33051=CARTESIAN_POINT('Ctrl Pts',(1.05704787279382,-2.28484179304104,103.70401020839));
#33052=CARTESIAN_POINT('Ctrl Pts',(1.06319774976688,-2.28198658323001,103.704442885096));
#33053=CARTESIAN_POINT('Ctrl Pts',(1.07841713219861,-2.27484578869245,103.705519366091));
#33054=CARTESIAN_POINT('Ctrl Pts',(1.08747263111089,-2.27053080619043,103.706164924753));
#33055=CARTESIAN_POINT('Ctrl Pts',(1.12145091404538,-2.254090121947,103.708605612451));
#33056=CARTESIAN_POINT('Ctrl Pts',(1.14619766165188,-2.24160772683778,103.710420629532));
#33057=CARTESIAN_POINT('Ctrl Pts',(1.20914684358895,-2.2085409324695,103.715125021244));
#33058=CARTESIAN_POINT('Ctrl Pts',(1.24703141732688,-2.18737316481083,103.71804047918));
#33059=CARTESIAN_POINT('Ctrl Pts',(1.39178567227098,-2.10150972186441,103.729461005882));
#33060=CARTESIAN_POINT('Ctrl Pts',(1.49432852909416,-2.02987476963691,103.738150507394));
#33061=CARTESIAN_POINT('Ctrl Pts',(1.71627785401383,-1.84885825314889,103.757869425521));
#33062=CARTESIAN_POINT('Ctrl Pts',(1.83133409454045,-1.7349694099233,103.768776753568));
#33063=CARTESIAN_POINT('Ctrl Pts',(1.94892500024888,-1.59373520128016,103.78062981604));
#33064=CARTESIAN_POINT('Ctrl Pts',(1.96292405764026,-1.5764611457634,103.782054682875));
#33065=CARTESIAN_POINT('Ctrl Pts',(1.98560188846137,-1.5477074534434,103.784386526103));
#33066=CARTESIAN_POINT('Ctrl Pts',(1.99441411087351,-1.53633511619186,103.785298750011));
#33067=CARTESIAN_POINT('Ctrl Pts',(2.0101596528762,-1.51565139973249,103.786940092334));
#33068=CARTESIAN_POINT('Ctrl Pts',(2.01712691793259,-1.50636648920261,103.787670524108));
#33069=CARTESIAN_POINT('Ctrl Pts',(2.03193994857154,-1.48633887212167,103.789232655357));
#33070=CARTESIAN_POINT('Ctrl Pts',(2.03976531693737,-1.47558146504539,103.790063553612));
#33071=CARTESIAN_POINT('Ctrl Pts',(2.06096964222586,-1.44594118579236,103.792331101244));
#33072=CARTESIAN_POINT('Ctrl Pts',(2.07417428590734,-1.42693477969431,103.793761117063));
#33073=CARTESIAN_POINT('Ctrl Pts',(2.15056737226987,-1.31367507366855,103.802147504405));
#33074=CARTESIAN_POINT('Ctrl Pts',(2.20759088404041,-1.21541322704999,103.80887007214));
#33075=CARTESIAN_POINT('Ctrl Pts',(2.33656453993592,-0.953929202174542,
103.825831001799));
#33076=CARTESIAN_POINT('Ctrl Pts',(2.39816219060529,-0.786336391452298,
103.835825090898));
#33077=CARTESIAN_POINT('Ctrl Pts',(2.45659294105046,-0.553858763133373,
103.8500250316));
#33078=CARTESIAN_POINT('Ctrl Pts',(2.46941998587658,-0.493530153092568,
103.853742986836));
#33079=CARTESIAN_POINT('Ctrl Pts',(2.48234532074541,-0.41946526816815,103.858413674917));
#33080=CARTESIAN_POINT('Ctrl Pts',(2.48456431889281,-0.406115167208964,
103.859259736029));
#33081=CARTESIAN_POINT('Ctrl Pts',(2.48786535012506,-0.385214768027129,
103.860591729263));
#33082=CARTESIAN_POINT('Ctrl Pts',(2.48902092522443,-0.377676115230287,
103.861073679511));
#33083=CARTESIAN_POINT('Ctrl Pts',(2.49110165857439,-0.363677553379477,
103.861971605708));
#33084=CARTESIAN_POINT('Ctrl Pts',(2.49203597222829,-0.357219184753035,
103.86238706839));
#33085=CARTESIAN_POINT('Ctrl Pts',(2.49412272673484,-0.342387947188415,
103.863343863585));
#33086=CARTESIAN_POINT('Ctrl Pts',(2.49525811751567,-0.334012880657101,
103.863886121089));
#33087=CARTESIAN_POINT('Ctrl Pts',(2.49867811721182,-0.307794603119102,
103.865589472183));
#33088=CARTESIAN_POINT('Ctrl Pts',(2.50081360349901,-0.289932971700124,
103.866758307899));
#33089=CARTESIAN_POINT('Ctrl Pts',(2.50539061636632,-0.247826272509079,
103.869531071063));
#33090=CARTESIAN_POINT('Ctrl Pts',(2.50767186666554,-0.22356591512065,103.871142153422));
#33091=CARTESIAN_POINT('Ctrl Pts',(2.51464730060758,-0.135720698402123,
103.877015825201));
#33092=CARTESIAN_POINT('Ctrl Pts',(2.5172775419411,-0.0719992546959435,
103.881351696753));
#33093=CARTESIAN_POINT('Ctrl Pts',(2.51819290377348,0.207284718027779,103.900513238944));
#33094=CARTESIAN_POINT('Ctrl Pts',(2.49121506644567,0.422064839390602,103.915558581474));
#33095=CARTESIAN_POINT('Ctrl Pts',(2.42432877236368,0.680494037955959,103.933150916291));
#33096=CARTESIAN_POINT('Ctrl Pts',(2.40994657293799,0.729794679059438,103.936489037007));
#33097=CARTESIAN_POINT('Ctrl Pts',(2.38828658793369,0.796393480172014,103.940976328755));
#33098=CARTESIAN_POINT('Ctrl Pts',(2.38230964334191,0.814098394141081,103.942167130181));
#33099=CARTESIAN_POINT('Ctrl Pts',(2.37246759445412,0.842215561312557,103.944055243054));
#33100=CARTESIAN_POINT('Ctrl Pts',(2.36872985157804,0.85267135234073,103.944756701115));
#33101=CARTESIAN_POINT('Ctrl Pts',(2.36089530244754,0.87413822529171,103.946195633144));
#33102=CARTESIAN_POINT('Ctrl Pts',(2.35679034440409,0.885146059170485,103.946932817321));
#33103=CARTESIAN_POINT('Ctrl Pts',(2.347061143097,0.910688258471362,103.948641988885));
#33104=CARTESIAN_POINT('Ctrl Pts',(2.34137865830064,0.925200037389391,103.949612016571));
#33105=CARTESIAN_POINT('Ctrl Pts',(2.32261512723451,0.971837608401551,103.952726895427));
#33106=CARTESIAN_POINT('Ctrl Pts',(2.30900446000084,1.00374695449878,103.954854065937));
#33107=CARTESIAN_POINT('Ctrl Pts',(2.275286842434,1.07847714596994,103.959834170742));
#33108=CARTESIAN_POINT('Ctrl Pts',(2.25462371775412,1.12103320564527,103.962668745218));
#33109=CARTESIAN_POINT('Ctrl Pts',(2.12517940517811,1.36954893250977,103.979280379542));
#33110=CARTESIAN_POINT('Ctrl Pts',(1.98945662788042,1.56015938306679,103.992149818749));
#33111=CARTESIAN_POINT('Ctrl Pts',(1.79149926896549,1.76957470315813,104.009295266606));
#33112=CARTESIAN_POINT('Ctrl Pts',(1.75220083533936,1.80849536997681,104.012642042198));
#33113=CARTESIAN_POINT('Ctrl Pts',(1.70203370257971,1.85500935870737,104.0168950149));
#33114=CARTESIAN_POINT('Ctrl Pts',(1.6923417025111,1.86385567850046,104.01771581325));
#33115=CARTESIAN_POINT('Ctrl Pts',(1.67697763586337,1.87766051496428,104.019016477323));
#33116=CARTESIAN_POINT('Ctrl Pts',(1.67135155468716,1.88267017232798,104.019492657996));
#33117=CARTESIAN_POINT('Ctrl Pts',(1.66129129872783,1.89154753882451,104.020344137058));
#33118=CARTESIAN_POINT('Ctrl Pts',(1.65686594389805,1.89542504794065,104.020718701669));
#33119=CARTESIAN_POINT('Ctrl Pts',(1.64621903116203,1.90468812753593,104.021619866632));
#33120=CARTESIAN_POINT('Ctrl Pts',(1.63998467141384,1.91005869928306,104.022147537837));
#33121=CARTESIAN_POINT('Ctrl Pts',(1.62091631724366,1.92632290297196,104.023761134662));
#33122=CARTESIAN_POINT('Ctrl Pts',(1.60799958550767,1.93711820263747,104.02485371313));
#33123=CARTESIAN_POINT('Ctrl Pts',(1.5776721507108,1.9619523525148,104.02741601137));
#33124=CARTESIAN_POINT('Ctrl Pts',(1.56018088840414,1.97589017175661,104.028891560371));
#33125=CARTESIAN_POINT('Ctrl Pts',(1.49826972460489,2.0238891435732,104.034099951038));
#33126=CARTESIAN_POINT('Ctrl Pts',(1.4529036240984,2.0566987418208,104.037890704739));
#33127=CARTESIAN_POINT('Ctrl Pts',(1.26818883053807,2.18112530640414,104.053118223817));
#33128=CARTESIAN_POINT('Ctrl Pts',(1.12096607590401,2.26032119749295,104.064769256644));
#33129=CARTESIAN_POINT('Ctrl Pts',(0.928852586041864,2.34024478674086,104.078855894059));
#33130=CARTESIAN_POINT('Ctrl Pts',(0.890325110723717,2.3551718104359,104.081630622758));
#33131=CARTESIAN_POINT('Ctrl Pts',(0.788900541379837,2.39162275689454,104.088799878732));
#33132=CARTESIAN_POINT('Ctrl Pts',(0.725485101710259,2.41161692201443,104.093148762845));
#33133=CARTESIAN_POINT('Ctrl Pts',(0.641536230320368,2.4344730632923,104.098735719866));
#33134=CARTESIAN_POINT('Ctrl Pts',(0.621659241682069,2.43962449133796,104.100046408423));
#33135=CARTESIAN_POINT('Ctrl Pts',(0.589355628408675,2.44757601700117,104.102157368533));
#33136=CARTESIAN_POINT('Ctrl Pts',(0.576967198032266,2.45052591861508,104.102962393943));
#33137=CARTESIAN_POINT('Ctrl Pts',(0.55313736990064,2.45600948835446,104.104502413175));
#33138=CARTESIAN_POINT('Ctrl Pts',(0.541699650689299,2.4585575146338,104.105237846392));
#33139=CARTESIAN_POINT('Ctrl Pts',(0.515212124770009,2.46426442892456,104.10693254275));
#33140=CARTESIAN_POINT('Ctrl Pts',(0.500150234825214,2.46736549142861,104.107889951416));
#33141=CARTESIAN_POINT('Ctrl Pts',(0.452155487794997,2.4767894858813,104.110921587775));
#33142=CARTESIAN_POINT('Ctrl Pts',(0.4191234489377,2.48259268487586,104.112979460435));
#33143=CARTESIAN_POINT('Ctrl Pts',(0.341264757513149,2.49467283942801,104.117770072956));
#33144=CARTESIAN_POINT('Ctrl Pts',(0.296364760548544,2.50040446389215,104.120486356639));
#33145=CARTESIAN_POINT('Ctrl Pts',(0.126747036677982,2.51742314238566,104.130610212274));
#33146=CARTESIAN_POINT('Ctrl Pts',(0.00139654736664436,2.52061201911248,
104.137803709537));
#33147=CARTESIAN_POINT('Ctrl Pts',(-0.277374990281951,2.5069005376098,104.153840800988));
#33148=CARTESIAN_POINT('Ctrl Pts',(-0.430038592648369,2.4852648650098,104.162650889239));
#33149=CARTESIAN_POINT('Ctrl Pts',(-0.600042952386263,2.44503366335934,
104.173386903523));
#33150=CARTESIAN_POINT('Ctrl Pts',(-0.620275712715725,2.43997933083985,
104.174680132825));
#33151=CARTESIAN_POINT('Ctrl Pts',(-0.648497803208608,2.43255549282413,
104.176508763767));
#33152=CARTESIAN_POINT('Ctrl Pts',(-0.656542324134751,2.43039663397824,
104.177032833131));
#33153=CARTESIAN_POINT('Ctrl Pts',(-0.670447958610272,2.42659078737335,
104.177943872225));
#33154=CARTESIAN_POINT('Ctrl Pts',(-0.6763141433339,2.42496236923534,104.178329789151));
#33155=CARTESIAN_POINT('Ctrl Pts',(-0.688733643045075,2.42146621979154,
104.179150310578));
#33156=CARTESIAN_POINT('Ctrl Pts',(-0.69528536085527,2.41959313697012,104.179585229249));
#33157=CARTESIAN_POINT('Ctrl Pts',(-0.711619539386714,2.41485150832662,
104.180674551665));
#33158=CARTESIAN_POINT('Ctrl Pts',(-0.721392245235629,2.41195012306551,
104.181330798121));
#33159=CARTESIAN_POINT('Ctrl Pts',(-0.758815515955138,2.40059187240579,
104.183860411409));
#33160=CARTESIAN_POINT('Ctrl Pts',(-0.786336071535937,2.39171857432284,
104.185755527085));
#33161=CARTESIAN_POINT('Ctrl Pts',(-0.857252244842686,2.36749725907046,
104.190719090296));
#33162=CARTESIAN_POINT('Ctrl Pts',(-0.900389641879886,2.35142992405045,
104.193817085444));
#33163=CARTESIAN_POINT('Ctrl Pts',(-1.14147464116673,2.25402674091749,104.211493028684));
#33164=CARTESIAN_POINT('Ctrl Pts',(-1.32889471629403,2.1488740421352,104.226536632923));
#33165=CARTESIAN_POINT('Ctrl Pts',(-1.56048454409993,1.97692434033028,104.245809189719));
#33166=CARTESIAN_POINT('Ctrl Pts',(-1.61822985796482,1.92994192730616,104.250692770374));
#33167=CARTESIAN_POINT('Ctrl Pts',(-1.6897690692209,1.86626444817063,104.256848527777));
#33168=CARTESIAN_POINT('Ctrl Pts',(-1.70554305239767,1.85185999474962,104.258212990566));
#33169=CARTESIAN_POINT('Ctrl Pts',(-1.73055744801084,1.82842663642423,104.260388918363));
#33170=CARTESIAN_POINT('Ctrl Pts',(-1.73991474752255,1.81952458820983,104.261205688064));
#33171=CARTESIAN_POINT('Ctrl Pts',(-1.75759580607391,1.80244262307174,104.262754584547));
#33172=CARTESIAN_POINT('Ctrl Pts',(-1.76593197332259,1.79427609356988,104.263487257118));
#33173=CARTESIAN_POINT('Ctrl Pts',(-1.77430838224018,1.78595521598048,104.264226006925));
#33174=CARTESIAN_POINT('Ctrl Pts',(-1.77440558691462,1.78585863995499,104.264234580152));
#33175=CARTESIAN_POINT('Ctrl Pts',(-1.77459141069251,1.78567398780044,104.264250970046));
#33176=CARTESIAN_POINT('Ctrl Pts',(-1.77468003113393,1.78558591300034,104.264258786772));
#33177=CARTESIAN_POINT('Ctrl Pts',(-1.77484958072505,1.78541738224506,104.264273742372));
#33178=CARTESIAN_POINT('Ctrl Pts',(-1.77493051095504,1.78533692739034,104.264280881293));
#33179=CARTESIAN_POINT('Ctrl Pts',(-1.7853627920837,1.77496451387658,104.265201152514));
#33180=CARTESIAN_POINT('Ctrl Pts',(-1.79562460687889,1.7645825597548,104.266110347399));
#33181=CARTESIAN_POINT('Ctrl Pts',(-1.82707988470309,1.73220046922871,104.268910249619));
#33182=CARTESIAN_POINT('Ctrl Pts',(-1.8479641503524,1.70990291917768,104.270787696295));
#33183=CARTESIAN_POINT('Ctrl Pts',(-1.89568954674353,1.65705182649992,104.275127247451));
#33184=CARTESIAN_POINT('Ctrl Pts',(-1.92220679614154,1.62621674548608,104.277576437106));
#33185=CARTESIAN_POINT('Ctrl Pts',(-2.01421626505934,1.51382847889194,104.28623859431));
#33186=CARTESIAN_POINT('Ctrl Pts',(-2.07536241552043,1.42885164841835,104.292302871935));
#33187=CARTESIAN_POINT('Ctrl Pts',(-2.21685757591394,1.20387962267085,104.307603582226));
#33188=CARTESIAN_POINT('Ctrl Pts',(-2.28935763884659,1.05953511150167,104.316735614932));
#33189=CARTESIAN_POINT('Ctrl Pts',(-2.35227831645096,0.897086230223406,
104.327251000269));
#33190=CARTESIAN_POINT('Ctrl Pts',(-2.35690249744092,0.884865846514591,
104.328043545471));
#33191=CARTESIAN_POINT('Ctrl Pts',(-2.36143112095504,0.87261062965393,104.32884037888));
#33192=CARTESIAN_POINT('Origin',(0.,0.,104.));
#33193=CARTESIAN_POINT('',(-2.36143106504625,0.872610780952508,105.331623435588));
#33194=CARTESIAN_POINT('',(-2.36143112101025,0.872610629504508,105.056194669753));
#33195=CARTESIAN_POINT('',(-2.36143112101026,0.872610629504505,104.));
#33196=CARTESIAN_POINT('',(-2.51749994136415,-0.000543352100661543,104.112583302546));
#33197=CARTESIAN_POINT('Ctrl Pts',(-2.36143112101026,0.872610629504506,
105.056194669753));
#33198=CARTESIAN_POINT('Ctrl Pts',(-2.33303020666493,0.949468280251065,
105.051033590384));
#33199=CARTESIAN_POINT('Ctrl Pts',(-2.30086848333539,1.02495005197359,105.045872511015));
#33200=CARTESIAN_POINT('Ctrl Pts',(-2.265114379073,1.09866423429397,105.040711431645));
#33201=CARTESIAN_POINT('Ctrl Pts',(-2.22847279274693,1.17420813703378,105.035422244875));
#33202=CARTESIAN_POINT('Ctrl Pts',(-2.18805831165858,1.24789504763111,105.030133058105));
#33203=CARTESIAN_POINT('Ctrl Pts',(-2.14410262607408,1.31932944288462,105.024843871335));
#33204=CARTESIAN_POINT('Ctrl Pts',(-2.10115760903028,1.38912135446288,105.01967629829));
#33205=CARTESIAN_POINT('Ctrl Pts',(-2.05483282336813,1.45676286489124,105.014508725245));
#33206=CARTESIAN_POINT('Ctrl Pts',(-2.00538749260778,1.52191565288366,105.0093411522));
#33207=CARTESIAN_POINT('Ctrl Pts',(-1.95419669134617,1.58936840060466,105.003991158567));
#33208=CARTESIAN_POINT('Ctrl Pts',(-1.89966127698031,1.65415300688264,104.998641164935));
#33209=CARTESIAN_POINT('Ctrl Pts',(-1.84211170893855,1.71593435241314,104.993291171302));
#33210=CARTESIAN_POINT('Ctrl Pts',(-1.78456214089678,1.77771569794364,104.987941177669));
#33211=CARTESIAN_POINT('Ctrl Pts',(-1.72399887340572,1.83649345024587,104.982591184036));
#33212=CARTESIAN_POINT('Ctrl Pts',(-1.66078955074686,1.89197894230619,104.977241190403));
#33213=CARTESIAN_POINT('Ctrl Pts',(-1.59869961602271,1.94648182946345,104.971985940996));
#33214=CARTESIAN_POINT('Ctrl Pts',(-1.53380920573794,1.9980256805317,104.966730691588));
#33215=CARTESIAN_POINT('Ctrl Pts',(-1.46643193098218,2.04630976193632,104.961475442181));
#33216=CARTESIAN_POINT('Ctrl Pts',(-1.39915018189582,2.09452538748228,104.956227643524));
#33217=CARTESIAN_POINT('Ctrl Pts',(-1.32938894355345,2.13949015670352,104.950979844866));
#33218=CARTESIAN_POINT('Ctrl Pts',(-1.25749623897844,2.18094233278991,104.945732046209));
#33219=CARTESIAN_POINT('Ctrl Pts',(-1.18508260977988,2.22269486562808,104.940446222726));
#33220=CARTESIAN_POINT('Ctrl Pts',(-1.11050685153569,2.26088337439192,104.935160399243));
#33221=CARTESIAN_POINT('Ctrl Pts',(-1.03415594736465,2.29528380086871,104.92987457576));
#33222=CARTESIAN_POINT('Ctrl Pts',(-0.958489676481174,2.32937576109578,
104.924636149891));
#33223=CARTESIAN_POINT('Ctrl Pts',(-0.881080395830975,2.35974710885148,
104.919397724023));
#33224=CARTESIAN_POINT('Ctrl Pts',(-0.802329463704414,2.38622582369561,
104.914159298154));
#33225=CARTESIAN_POINT('Ctrl Pts',(-0.72360443144881,2.4126958301311,104.908922595117));
#33226=CARTESIAN_POINT('Ctrl Pts',(-0.643539061072373,2.43527559930734,
104.903685892079));
#33227=CARTESIAN_POINT('Ctrl Pts',(-0.56255261396542,2.45384205003514,104.898449189042));
#33228=CARTESIAN_POINT('Ctrl Pts',(-0.481568372888753,2.47240799502212,
104.893212628649));
#33229=CARTESIAN_POINT('Ctrl Pts',(-0.399663554949806,2.48696073681588,
104.887976068257));
#33230=CARTESIAN_POINT('Ctrl Pts',(-0.317269076047356,2.49742799363346,
104.882739507865));
#33231=CARTESIAN_POINT('Ctrl Pts',(-0.233526021624755,2.50806657123,104.877417239094));
#33232=CARTESIAN_POINT('Ctrl Pts',(-0.14927761891385,2.51448464551234,104.872094970324));
#33233=CARTESIAN_POINT('Ctrl Pts',(-0.0649813996979932,2.51666121432609,
104.866772701553));
#33234=CARTESIAN_POINT('Ctrl Pts',(0.0180764464160268,2.51880580775236,
104.861528620803));
#33235=CARTESIAN_POINT('Ctrl Pts',(0.101180247008966,2.51683276258219,104.856284540053));
#33236=CARTESIAN_POINT('Ctrl Pts',(0.183894488815563,2.5107745950171,104.851040459302));
#33237=CARTESIAN_POINT('Ctrl Pts',(0.26845860568486,2.50458093865516,104.845679096522));
#33238=CARTESIAN_POINT('Ctrl Pts',(0.352615020686807,2.49411729347779,104.840317733741));
#33239=CARTESIAN_POINT('Ctrl Pts',(0.435908145372231,2.47947380280537,104.834956370961));
#33240=CARTESIAN_POINT('Ctrl Pts',(0.51920127005765,2.46483031213296,104.82959500818));
#33241=CARTESIAN_POINT('Ctrl Pts',(0.60163062394185,2.44600715420394,104.8242336454));
#33242=CARTESIAN_POINT('Ctrl Pts',(0.682757877074153,2.42314835106999,104.818872282619));
#33243=CARTESIAN_POINT('Ctrl Pts',(0.762279440227179,2.40074197482975,104.813617033212));
#33244=CARTESIAN_POINT('Ctrl Pts',(0.840843710027796,2.3743755294766,104.808361783804));
#33245=CARTESIAN_POINT('Ctrl Pts',(0.918027687426422,2.3441483347089,104.803106534397));
#33246=CARTESIAN_POINT('Ctrl Pts',(0.99510223547909,2.31396399523662,104.79785873574));
#33247=CARTESIAN_POINT('Ctrl Pts',(1.07079995212236,2.2799299455045,104.792610937082));
#33248=CARTESIAN_POINT('Ctrl Pts',(1.1447118128608,2.24219560152475,104.787363138425));
#33249=CARTESIAN_POINT('Ctrl Pts',(1.21915922874995,2.20418783969196,104.782077314942));
#33250=CARTESIAN_POINT('Ctrl Pts',(1.29179434327542,2.16242606222529,104.776791491459));
#33251=CARTESIAN_POINT('Ctrl Pts',(1.3622185245738,2.11711287873556,104.771505667976));
#33252=CARTESIAN_POINT('Ctrl Pts',(1.43201121709949,2.07220601543446,104.766267242107));
#33253=CARTESIAN_POINT('Ctrl Pts',(1.49963207297644,2.02381143571998,104.761028816239));
#33254=CARTESIAN_POINT('Ctrl Pts',(1.56471828263879,1.97217213903247,104.75579039037));
#33255=CARTESIAN_POINT('Ctrl Pts',(1.62978308653003,1.9205498256502,104.750553687333));
#33256=CARTESIAN_POINT('Ctrl Pts',(1.69231453860289,1.86568520124402,104.745316984295));
#33257=CARTESIAN_POINT('Ctrl Pts',(1.75198113178698,1.80786292728802,104.740080281258));
#33258=CARTESIAN_POINT('Ctrl Pts',(1.8116460996829,1.75004222838186,104.734843720865));
#33259=CARTESIAN_POINT('Ctrl Pts',(1.8684460332112,1.6892643619624,104.729607160473));
#33260=CARTESIAN_POINT('Ctrl Pts',(1.92208569013621,1.62585142303151,104.724370600081));
#33261=CARTESIAN_POINT('Ctrl Pts',(1.97660328365608,1.56140058522383,104.71904833131));
#33262=CARTESIAN_POINT('Ctrl Pts',(2.02785588922083,1.4942280055528,104.71372606254));
#33263=CARTESIAN_POINT('Ctrl Pts',(2.07557678649174,1.42470602349278,104.708403793769));
#33264=CARTESIAN_POINT('Ctrl Pts',(2.12259662888583,1.35620537018719,104.703159713019));
#33265=CARTESIAN_POINT('Ctrl Pts',(2.16618764777983,1.28542431585759,104.697915632269));
#33266=CARTESIAN_POINT('Ctrl Pts',(2.20614000163562,1.21274586916765,104.692671551518));
#33267=CARTESIAN_POINT('Ctrl Pts',(2.24698587589954,1.13844199445953,104.687310188738));
#33268=CARTESIAN_POINT('Ctrl Pts',(2.28402814256915,1.06215529485621,104.681948825957));
#33269=CARTESIAN_POINT('Ctrl Pts',(2.31709436732378,0.98431699310558,104.676587463177));
#33270=CARTESIAN_POINT('Ctrl Pts',(2.35016059207842,0.906478691354946,104.671226100396));
#33271=CARTESIAN_POINT('Ctrl Pts',(2.37925066282247,0.827089287526055,104.665864737616));
#33272=CARTESIAN_POINT('Ctrl Pts',(2.40424673471588,0.746594862430761,104.660503374835));
#33273=CARTESIAN_POINT('Ctrl Pts',(2.42874807838157,0.667693602231119,104.655248125428));
#33274=CARTESIAN_POINT('Ctrl Pts',(2.44940654676645,0.587439246499782,104.64999287602));
#33275=CARTESIAN_POINT('Ctrl Pts',(2.46607514597444,0.506240678341004,104.644737626613));
#33276=CARTESIAN_POINT('Ctrl Pts',(2.48272011289541,0.425157231305679,104.639489827956));
#33277=CARTESIAN_POINT('Ctrl Pts',(2.4953863545401,0.343132679074028,104.634242029298));
#33278=CARTESIAN_POINT('Ctrl Pts',(2.50397650588177,0.260591458018378,104.628994230641));
#33279=CARTESIAN_POINT('Ctrl Pts',(2.51262890027548,0.177452154657314,104.623708407158));
#33280=CARTESIAN_POINT('Ctrl Pts',(2.5171457450105,0.0937891160265086,104.618422583675));
#33281=CARTESIAN_POINT('Ctrl Pts',(2.51747995172501,0.0100470225765003,
104.613136760192));
#33282=CARTESIAN_POINT('Ctrl Pts',(2.51781116163097,-0.072944161301868,
104.607898334323));
#33283=CARTESIAN_POINT('Ctrl Pts',(2.51403444206276,-0.156012518000315,
104.602659908455));
#33284=CARTESIAN_POINT('Ctrl Pts',(2.50615608684174,-0.238721424229384,
104.597421482586));
#33285=CARTESIAN_POINT('Ctrl Pts',(2.49828032268064,-0.321403128875668,
104.592184779549));
#33286=CARTESIAN_POINT('Ctrl Pts',(2.48630564569435,-0.403725158859374,
104.586948076511));
#33287=CARTESIAN_POINT('Ctrl Pts',(2.47029033818926,-0.485254464223448,
104.581711373474));
#33288=CARTESIAN_POINT('Ctrl Pts',(2.45427546693312,-0.56678154877009,104.576474813081));
#33289=CARTESIAN_POINT('Ctrl Pts',(2.43422027394694,-0.647515499061263,
104.571238252689));
#33290=CARTESIAN_POINT('Ctrl Pts',(2.41023418493731,-0.727033303060847,
104.566001692297));
#33291=CARTESIAN_POINT('Ctrl Pts',(2.38585550830661,-0.807852599166646,
104.560679423526));
#33292=CARTESIAN_POINT('Ctrl Pts',(2.35741622780974,-0.887415105170729,
104.555357154756));
#33293=CARTESIAN_POINT('Ctrl Pts',(2.32508344262049,-0.96529437730261,104.550034885985));
#33294=CARTESIAN_POINT('Ctrl Pts',(2.29322564968901,-1.04202954597769,104.544790805235));
#33295=CARTESIAN_POINT('Ctrl Pts',(2.25758824566432,-1.11713021185096,104.539546724484));
#33296=CARTESIAN_POINT('Ctrl Pts',(2.21837824670566,-1.19021183179429,104.534302643734));
#33297=CARTESIAN_POINT('Ctrl Pts',(2.17829132984629,-1.26492789658442,104.528941280954));
#33298=CARTESIAN_POINT('Ctrl Pts',(2.13447035466966,-1.33753307677803,104.523579918173));
#33299=CARTESIAN_POINT('Ctrl Pts',(2.08718314535484,-1.40764795589902,104.518218555392));
#33300=CARTESIAN_POINT('Ctrl Pts',(2.03989593604002,-1.47776283502,104.512857192612));
#33301=CARTESIAN_POINT('Ctrl Pts',(1.98914285101044,-1.54538704678005,104.507495829831));
#33302=CARTESIAN_POINT('Ctrl Pts',(1.93523389860253,-1.61017887444211,104.502134467051));
#33303=CARTESIAN_POINT('Ctrl Pts',(1.88239192506217,-1.67368832676914,104.496879217643));
#33304=CARTESIAN_POINT('Ctrl Pts',(1.8263227259832,-1.73471109993217,104.491623968236));
#33305=CARTESIAN_POINT('Ctrl Pts',(1.76728923830282,-1.7929012795408,104.486368718829));
#33306=CARTESIAN_POINT('Ctrl Pts',(1.70833944669724,-1.85100895869389,104.481120920171));
#33307=CARTESIAN_POINT('Ctrl Pts',(1.64643404012584,-1.90629169997362,104.475873121514));
#33308=CARTESIAN_POINT('Ctrl Pts',(1.58187602200247,-1.95843674930125,104.470625322856));
#33309=CARTESIAN_POINT('Ctrl Pts',(1.5168502253821,-2.01095963446569,104.465339499373));
#33310=CARTESIAN_POINT('Ctrl Pts',(1.44913351719056,-2.06029880096661,104.46005367589));
#33311=CARTESIAN_POINT('Ctrl Pts',(1.37907325462703,-2.10617264448393,104.454767852407));
#33312=CARTESIAN_POINT('Ctrl Pts',(1.30964121760201,-2.15163514041286,104.449529426539));
#33313=CARTESIAN_POINT('Ctrl Pts',(1.23790787999602,-2.19369395365314,104.44429100067));
#33314=CARTESIAN_POINT('Ctrl Pts',(1.16424290473668,-2.23211664318205,104.439052574802));
#33315=CARTESIAN_POINT('Ctrl Pts',(1.09060215666171,-2.27052669612783,104.433815871764));
#33316=CARTESIAN_POINT('Ctrl Pts',(1.01503144143266,-2.3053027871867,104.428579168726));
#33317=CARTESIAN_POINT('Ctrl Pts',(0.937925729905276,-2.33625802838249,
104.423342465689));
#33318=CARTESIAN_POINT('Ctrl Pts',(0.860822118699087,-2.36721242637293,
104.418105905297));
#33319=CARTESIAN_POINT('Ctrl Pts',(0.78218402291449,-2.39434601048306,104.412869344904));
#33320=CARTESIAN_POINT('Ctrl Pts',(0.702425838780685,-2.41752025658799,
104.407632784512));
#33321=CARTESIAN_POINT('Ctrl Pts',(0.621362228165491,-2.44107380263411,
104.402310515741));
#33322=CARTESIAN_POINT('Ctrl Pts',(0.539142001278009,-2.46053708415131,
104.396988246971));
#33323=CARTESIAN_POINT('Ctrl Pts',(0.456213833269011,-2.47581808466091,
104.3916659782));
#33324=CARTESIAN_POINT('Ctrl Pts',(0.374503940689362,-2.49087459609877,
104.38642189745));
#33325=CARTESIAN_POINT('Ctrl Pts',(0.292107241290161,-2.50187089130869,
104.3811778167));
#33326=CARTESIAN_POINT('Ctrl Pts',(0.209458997151658,-2.50877124874155,
104.375933735949));
#33327=CARTESIAN_POINT('Ctrl Pts',(0.124962353964994,-2.51582593025284,
104.370572373169));
#33328=CARTESIAN_POINT('Ctrl Pts',(0.0402032906129579,-2.51859923804143,
104.365211010388));
#33329=CARTESIAN_POINT('Ctrl Pts',(-0.0443541239990409,-2.5171092470698,
104.359849647608));
#33330=CARTESIAN_POINT('Ctrl Pts',(-0.12891153861104,-2.51561925609817,
104.354488284827));
#33331=CARTESIAN_POINT('Ctrl Pts',(-0.213266802098999,-2.50986606758289,
104.349126922046));
#33332=CARTESIAN_POINT('Ctrl Pts',(-0.296964500577455,-2.49992366591398,
104.343765559266));
#33333=CARTESIAN_POINT('Ctrl Pts',(-0.379005634207852,-2.49017804663466,
104.338510309859));
#33334=CARTESIAN_POINT('Ctrl Pts',(-0.460718028522092,-2.47637157911839,
104.333255060451));
#33335=CARTESIAN_POINT('Ctrl Pts',(-0.541668376772253,-2.45853647920972,
104.327999811044));
#33336=CARTESIAN_POINT('Ctrl Pts',(-0.622503955818408,-2.44072666542105,
104.322752012386));
#33337=CARTESIAN_POINT('Ctrl Pts',(-0.702579187952239,-2.41889966276607,
104.317504213729));
#33338=CARTESIAN_POINT('Ctrl Pts',(-0.781466766783666,-2.39313934872432,
104.312256415071));
#33339=CARTESIAN_POINT('Ctrl Pts',(-0.860925954132904,-2.36719237899932,
104.306970591589));
#33340=CARTESIAN_POINT('Ctrl Pts',(-0.939179733834524,-2.33725491281204,
104.301684768106));
#33341=CARTESIAN_POINT('Ctrl Pts',(-1.01580277918804,-2.30346499078971,
104.296398944623));
#33342=CARTESIAN_POINT('Ctrl Pts',(-1.09173875098279,-2.2699780606658,104.291160518754));
#33343=CARTESIAN_POINT('Ctrl Pts',(-1.1660726866908,-2.23270767701558,104.285922092886));
#33344=CARTESIAN_POINT('Ctrl Pts',(-1.23840835301748,-2.19183735737316,
104.280683667017));
#33345=CARTESIAN_POINT('Ctrl Pts',(-1.31072022934732,-2.15098047929869,
104.27544696398));
#33346=CARTESIAN_POINT('Ctrl Pts',(-1.38103474011157,-2.10652624344265,
104.270210260942));
#33347=CARTESIAN_POINT('Ctrl Pts',(-1.44898008261864,-2.05870419686133,
104.264973557905));
#33348=CARTESIAN_POINT('Ctrl Pts',(-1.51692357432857,-2.01088345292865,
104.259736997512));
#33349=CARTESIAN_POINT('Ctrl Pts',(-1.58249764935668,-1.95969534708828,
104.25450043712));
#33350=CARTESIAN_POINT('Ctrl Pts',(-1.6453604960618,-1.90541205202425,104.249263876728));
#33351=CARTESIAN_POINT('Ctrl Pts',(-1.70925223811683,-1.85024028574396,
104.243941607957));
#33352=CARTESIAN_POINT('Ctrl Pts',(-1.77034281937563,-1.79187140774975,
104.238619339187));
#33353=CARTESIAN_POINT('Ctrl Pts',(-1.8283107752395,-1.73063166478114,104.233297070416));
#33354=CARTESIAN_POINT('Ctrl Pts',(-1.88542713944256,-1.67029157841842,
104.228052989666));
#33355=CARTESIAN_POINT('Ctrl Pts',(-1.93951175864249,-1.6071648127306,104.222808908916));
#33356=CARTESIAN_POINT('Ctrl Pts',(-1.99029769076042,-1.54159701353945,
104.217564828165));
#33357=CARTESIAN_POINT('Ctrl Pts',(-2.04221943247203,-1.47456281347207,
104.212203465385));
#33358=CARTESIAN_POINT('Ctrl Pts',(-2.09069286600373,-1.40497749678778,
104.206842102604));
#33359=CARTESIAN_POINT('Ctrl Pts',(-2.13548048945464,-1.33324016184578,
104.201480739824));
#33360=CARTESIAN_POINT('Ctrl Pts',(-2.18026811290555,-1.26150282690377,
104.196119377043));
#33361=CARTESIAN_POINT('Ctrl Pts',(-2.2213697376516,-1.1876139502074,104.190758014263));
#33362=CARTESIAN_POINT('Ctrl Pts',(-2.25859947042747,-1.11199581032698,
104.185396651482));
#33363=CARTESIAN_POINT('Ctrl Pts',(-2.29771370768151,-1.03255001140606,
104.17976390582));
#33364=CARTESIAN_POINT('Ctrl Pts',(-2.33268319210157,-0.950935265154256,
104.174131160157));
#33365=CARTESIAN_POINT('Ctrl Pts',(-2.3632800928912,-0.867590601922441,
104.168498414495));
#33366=CARTESIAN_POINT('Ctrl Pts',(-2.39377456178273,-0.784524958847305,
104.162884526064));
#33367=CARTESIAN_POINT('Ctrl Pts',(-2.41992549446131,-0.699741274927147,
104.157270637633));
#33368=CARTESIAN_POINT('Ctrl Pts',(-2.44155272692772,-0.613699056241603,
104.151656749201));
#33369=CARTESIAN_POINT('Ctrl Pts',(-2.46313411560349,-0.527839223419127,
104.146054760671));
#33370=CARTESIAN_POINT('Ctrl Pts',(-2.48021080455414,-0.44072651169474,
104.140452772141));
#33371=CARTESIAN_POINT('Ctrl Pts',(-2.49265158327774,-0.352837546730744,
104.134850783611));
#33372=CARTESIAN_POINT('Ctrl Pts',(-2.50505613088024,-0.265204539677777,
104.12926510968));
#33373=CARTESIAN_POINT('Ctrl Pts',(-2.51285161508245,-0.176800136803316,
104.12367943575));
#33374=CARTESIAN_POINT('Ctrl Pts',(-2.51595758515502,-0.0881117455332033,
104.118093761819));
#33375=CARTESIAN_POINT('Ctrl Pts',(-2.51697896722405,-0.0589470303370983,
104.116256942062));
#33376=CARTESIAN_POINT('Ctrl Pts',(-2.51749363732475,-0.0297517030198697,
104.114420122304));
#33377=CARTESIAN_POINT('Ctrl Pts',(-2.51749994136415,-0.000543352100661293,
104.112583302546));
#33378=CARTESIAN_POINT('Ctrl Pts',(-2.51749994136434,-0.000543351236957333,
104.112583302492));
#33379=CARTESIAN_POINT('Ctrl Pts',(-2.51751848517037,0.0853753463440664,
104.107180150438));
#33380=CARTESIAN_POINT('Ctrl Pts',(-2.51313426361846,0.171241893100704,
104.101776998384));
#33381=CARTESIAN_POINT('Ctrl Pts',(-2.50438935623882,0.256593457355597,
104.096373846329));
#33382=CARTESIAN_POINT('Ctrl Pts',(-2.49563786309435,0.342009299630279,
104.090966625177));
#33383=CARTESIAN_POINT('Ctrl Pts',(-2.48251919937096,0.426908972259079,
104.085559404024));
#33384=CARTESIAN_POINT('Ctrl Pts',(-2.46512690395723,0.510838132275033,
104.080152182872));
#33385=CARTESIAN_POINT('Ctrl Pts',(-2.44770570697484,0.594906761195075,
104.074735976293));
#33386=CARTESIAN_POINT('Ctrl Pts',(-2.42599679375752,0.678001249607856,
104.069319769715));
#33387=CARTESIAN_POINT('Ctrl Pts',(-2.40014407058638,0.759680650292643,
104.063903563137));
#33388=CARTESIAN_POINT('Ctrl Pts',(-2.38812822328385,0.797643660993429,
104.061386214742));
#33389=CARTESIAN_POINT('Ctrl Pts',(-2.37521791696454,0.835301240958594,
104.058868866346));
#33390=CARTESIAN_POINT('Ctrl Pts',(-2.36143112101026,0.872610629504494,
104.05635151795));
#33391=CARTESIAN_POINT('',(-2.51749878614078,0.00217395721947723,104.388357324048));
#33392=CARTESIAN_POINT('Ctrl Pts',(-2.36143112095504,0.87261062965393,104.32884037888));
#33393=CARTESIAN_POINT('Ctrl Pts',(-2.36994372294453,0.849574097006755,
104.330338212745));
#33394=CARTESIAN_POINT('Ctrl Pts',(-2.37811868251946,0.82641448493804,104.331851197041));
#33395=CARTESIAN_POINT('Ctrl Pts',(-2.38967067758178,0.792096000718289,
104.334108788615));
#33396=CARTESIAN_POINT('Ctrl Pts',(-2.39331116459058,0.781027322701226,
104.334839298037));
#33397=CARTESIAN_POINT('Ctrl Pts',(-2.39905590931377,0.763143410196021,
104.336024015738));
#33398=CARTESIAN_POINT('Ctrl Pts',(-2.40120831839551,0.756343658132843,
104.33647548894));
#33399=CARTESIAN_POINT('Ctrl Pts',(-2.40531609083367,0.743172371081131,
104.337352148091));
#33400=CARTESIAN_POINT('Ctrl Pts',(-2.40727508292726,0.736802104376359,
104.337777122774));
#33401=CARTESIAN_POINT('Ctrl Pts',(-2.41194565227788,0.721396843246568,
104.338807098303));
#33402=CARTESIAN_POINT('Ctrl Pts',(-2.4146317722416,0.712354288755783,104.339413535808));
#33403=CARTESIAN_POINT('Ctrl Pts',(-2.4238789211069,0.680571376831846,104.341551062752));
#33404=CARTESIAN_POINT('Ctrl Pts',(-2.43016979895327,0.657754571033595,
104.343096343929));
#33405=CARTESIAN_POINT('Ctrl Pts',(-2.48997770515915,0.428252319084638,
104.358724032165));
#33406=CARTESIAN_POINT('Ctrl Pts',(-2.51731451133507,0.215658486073652,
104.373797644526));
#33407=CARTESIAN_POINT('Ctrl Pts',(-2.51749905933581,0.00217629118206962,
104.388357642272));
#33408=CARTESIAN_POINT('Ctrl Pts',(-2.51749906132417,0.00217398986072041,
104.388357799227));
#33409=CARTESIAN_POINT('Ctrl Pts',(-2.51759705576998,-0.111304425924101,
104.396097297547));
#33410=CARTESIAN_POINT('Ctrl Pts',(-2.51002239620448,-0.224674609144805,
104.403685278352));
#33411=CARTESIAN_POINT('Ctrl Pts',(-2.49202450093169,-0.35784890421739,
104.412393645945));
#33412=CARTESIAN_POINT('Ctrl Pts',(-2.48897173933918,-0.378499240382162,
104.41373838398));
#33413=CARTESIAN_POINT('Ctrl Pts',(-2.48347979364576,-0.412703174110995,
104.415956789967));
#33414=CARTESIAN_POINT('Ctrl Pts',(-2.4811856609536,-0.426278692344601,
104.416834930007));
#33415=CARTESIAN_POINT('Ctrl Pts',(-2.47684388210193,-0.450747680262971,
104.418413657293));
#33416=CARTESIAN_POINT('Ctrl Pts',(-2.47483545520061,-0.461647661793919,
104.419115458553));
#33417=CARTESIAN_POINT('Ctrl Pts',(-2.47079094447573,-0.482812447619622,
104.42047544179));
#33418=CARTESIAN_POINT('Ctrl Pts',(-2.46876271547497,-0.493078503782115,
104.421133856617));
#33419=CARTESIAN_POINT('Ctrl Pts',(-2.46404228637102,-0.516211841699916,
104.422614827664));
#33420=CARTESIAN_POINT('Ctrl Pts',(-2.46131318076387,-0.529071347882821,
104.423436195842));
#33421=CARTESIAN_POINT('Ctrl Pts',(-2.4536577064387,-0.563802001677604,
104.425649793425));
#33422=CARTESIAN_POINT('Ctrl Pts',(-2.44853964364161,-0.585630003466548,
104.427035918781));
#33423=CARTESIAN_POINT('Ctrl Pts',(-2.42208859806725,-0.692025641742305,
104.433771175174));
#33424=CARTESIAN_POINT('Ctrl Pts',(-2.39666137425239,-0.775518712718171,
104.438988286628));
#33425=CARTESIAN_POINT('Ctrl Pts',(-2.33319474884591,-0.950698787142168,
104.449937633954));
#33426=CARTESIAN_POINT('Ctrl Pts',(-2.29396787372504,-1.0417958409853,104.455632884603));
#33427=CARTESIAN_POINT('Ctrl Pts',(-2.21290939211794,-1.20310827165754,
104.466006020939));
#33428=CARTESIAN_POINT('Ctrl Pts',(-2.17283888657701,-1.27405172977227,
104.470679265308));
#33429=CARTESIAN_POINT('Ctrl Pts',(-2.08366744399577,-1.41544588724591,
104.480453786612));
#33430=CARTESIAN_POINT('Ctrl Pts',(-2.03426223784131,-1.48557430605187,
104.485558513338));
#33431=CARTESIAN_POINT('Ctrl Pts',(-1.97261100150029,-1.56422961146285,
104.49176165647));
#33432=CARTESIAN_POINT('Ctrl Pts',(-1.96374468859346,-1.57534606256729,
104.492650095827));
#33433=CARTESIAN_POINT('Ctrl Pts',(-1.94993732297004,-1.5923598420077,104.494029114021));
#33434=CARTESIAN_POINT('Ctrl Pts',(-1.94506244473924,-1.5983108309357,104.494515142902));
#33435=CARTESIAN_POINT('Ctrl Pts',(-1.93600676094677,-1.60926273793144,
104.495416634101));
#33436=CARTESIAN_POINT('Ctrl Pts',(-1.93183373327006,-1.61426985413066,
104.495831546242));
#33437=CARTESIAN_POINT('Ctrl Pts',(-1.92226434411328,-1.6256616885958,104.496781817996));
#33438=CARTESIAN_POINT('Ctrl Pts',(-1.9168556175426,-1.63203574444419,104.497318054359));
#33439=CARTESIAN_POINT('Ctrl Pts',(-1.90259415430328,-1.64867384778636,
104.498729443671));
#33440=CARTESIAN_POINT('Ctrl Pts',(-1.89369022706055,-1.65889338937834,
104.499608097677));
#33441=CARTESIAN_POINT('Ctrl Pts',(-1.82139122917186,-1.74053446506236,
104.506719063702));
#33442=CARTESIAN_POINT('Ctrl Pts',(-1.75406773897452,-1.80836075757747,
104.513193656654));
#33443=CARTESIAN_POINT('Ctrl Pts',(-1.59779231913719,-1.94884927253105,
104.527621178152));
#33444=CARTESIAN_POINT('Ctrl Pts',(-1.50738300055502,-2.01959182732876,
104.53558998574));
#33445=CARTESIAN_POINT('Ctrl Pts',(-1.33565847272146,-2.13598501867354,
104.549802292006));
#33446=CARTESIAN_POINT('Ctrl Pts',(-1.25602695061295,-2.18376161411814,
104.556075890789));
#33447=CARTESIAN_POINT('Ctrl Pts',(-1.14056181732992,-2.2446264702294,104.564700606796));
#33448=CARTESIAN_POINT('Ctrl Pts',(-1.1067990198121,-2.26146532669062,104.567169314603));
#33449=CARTESIAN_POINT('Ctrl Pts',(-1.04652949196028,-2.28985089286147,
104.571483857217));
#33450=CARTESIAN_POINT('Ctrl Pts',(-1.02017910749754,-2.30171149173258,
104.573339907378));
#33451=CARTESIAN_POINT('Ctrl Pts',(-0.980712421350819,-2.31866492494391,
104.576076160567));
#33452=CARTESIAN_POINT('Ctrl Pts',(-0.967748930751122,-2.32410539942738,
104.576968033364));
#33453=CARTESIAN_POINT('Ctrl Pts',(-0.954667741871376,-2.32946684002677,
104.577861214339));
#33454=CARTESIAN_POINT('Ctrl Pts',(-0.954595152639167,-2.32949658740079,
104.577866170508));
#33455=CARTESIAN_POINT('Ctrl Pts',(-0.954445826567376,-2.32955777370407,
104.577876365601));
#33456=CARTESIAN_POINT('Ctrl Pts',(-0.954369089564325,-2.32958921223488,
104.577881604512));
#33457=CARTESIAN_POINT('Ctrl Pts',(-0.954211215777274,-2.32965388274147,
104.577892382229));
#33458=CARTESIAN_POINT('Ctrl Pts',(-0.954130078808578,-2.32968711427099,
104.577897921021));
#33459=CARTESIAN_POINT('Ctrl Pts',(-0.953963136003445,-2.32975547938909,
104.577909316785));
#33460=CARTESIAN_POINT('Ctrl Pts',(-0.953877329947913,-2.32979061248183,
104.577915173741));
#33461=CARTESIAN_POINT('Ctrl Pts',(-0.953700761651266,-2.32986289657649,
104.577927225353));
#33462=CARTESIAN_POINT('Ctrl Pts',(-0.953609999195669,-2.32990004700889,
104.577933419987));
#33463=CARTESIAN_POINT('Ctrl Pts',(-0.953423211188627,-2.32997648939459,
104.577946167795));
#33464=CARTESIAN_POINT('Ctrl Pts',(-0.953327185384246,-2.33001578071311,
104.577952720947));
#33465=CARTESIAN_POINT('Ctrl Pts',(-0.953129542660793,-2.33009663682879,
104.577966208055));
#33466=CARTESIAN_POINT('Ctrl Pts',(-0.953027925444611,-2.33013820091779,
104.577973141988));
#33467=CARTESIAN_POINT('Ctrl Pts',(-0.952818749103518,-2.33022374351904,
104.577987414462));
#33468=CARTESIAN_POINT('Ctrl Pts',(-0.95271118963862,-2.33026772123729,
104.577994752977));
#33469=CARTESIAN_POINT('Ctrl Pts',(-0.952489753423229,-2.33035824172119,
104.578009860074));
#33470=CARTESIAN_POINT('Ctrl Pts',(-0.952375876312009,-2.33040478358441,
104.578017628626));
#33471=CARTESIAN_POINT('Ctrl Pts',(-0.952141402930466,-2.33050059339113,
104.578033623044));
#33472=CARTESIAN_POINT('Ctrl Pts',(-0.95202080624327,-2.33054986032282,
104.578041848876));
#33473=CARTESIAN_POINT('Ctrl Pts',(-0.951772463216978,-2.33065129251508,
104.578058787026));
#33474=CARTESIAN_POINT('Ctrl Pts',(-0.951644716414116,-2.33070345663309,
104.578067499306));
#33475=CARTESIAN_POINT('Ctrl Pts',(-0.951381611756175,-2.3308108675279,
104.578085441605));
#33476=CARTESIAN_POINT('Ctrl Pts',(-0.951246253372611,-2.33086611301862,
104.578094671581));
#33477=CARTESIAN_POINT('Ctrl Pts',(-0.950967430754681,-2.33097988400824,
104.578113682769));
#33478=CARTESIAN_POINT('Ctrl Pts',(-0.950823965931995,-2.33103840805264,
104.578123463932));
#33479=CARTESIAN_POINT('Ctrl Pts',(-0.950528399567668,-2.33115894751862,
104.578143613415));
#33480=CARTESIAN_POINT('Ctrl Pts',(-0.950376297342477,-2.33122096130556,
104.578153981681));
#33481=CARTESIAN_POINT('Ctrl Pts',(-0.950062886302104,-2.33134870673876,
104.578175343907));
#33482=CARTESIAN_POINT('Ctrl Pts',(-0.949901576727771,-2.33141443653232,
104.578186337805));
#33483=CARTESIAN_POINT('Ctrl Pts',(-0.949569138981177,-2.33154985673396,
104.578208992657));
#33484=CARTESIAN_POINT('Ctrl Pts',(-0.949398009956761,-2.33161954504412,
104.578220653541));
#33485=CARTESIAN_POINT('Ctrl Pts',(-0.94904527580149,-2.33176314254297,
104.578244686773));
#33486=CARTESIAN_POINT('Ctrl Pts',(-0.948863669699855,-2.33183704935974,
104.578257059043));
#33487=CARTESIAN_POINT('Ctrl Pts',(-0.948489274743593,-2.33198936297135,
104.578282562742));
#33488=CARTESIAN_POINT('Ctrl Pts',(-0.948296484791196,-2.33206776707879,
104.578295694082));
#33489=CARTESIAN_POINT('Ctrl Pts',(-0.94789896247512,-2.33222937460635,
104.57832276716));
#33490=CARTESIAN_POINT('Ctrl Pts',(-0.947694228862453,-2.33231257498196,
104.578336708796));
#33491=CARTESIAN_POINT('Ctrl Pts',(-0.947272002425946,-2.33248409609232,
104.578365457515));
#33492=CARTESIAN_POINT('Ctrl Pts',(-0.947054508193853,-2.33257241336971,
104.578380264481));
#33493=CARTESIAN_POINT('Ctrl Pts',(-0.946605882228841,-2.33275451257663,
104.578410803006));
#33494=CARTESIAN_POINT('Ctrl Pts',(-0.946374748899497,-2.33284829058008,
104.578426534432));
#33495=CARTESIAN_POINT('Ctrl Pts',(-0.945897900405061,-2.33304168036229,
104.578458985413));
#33496=CARTESIAN_POINT('Ctrl Pts',(-0.945652183424224,-2.33314128768137,
104.578475704817));
#33497=CARTESIAN_POINT('Ctrl Pts',(-0.945231257997559,-2.3333118425611,
104.578504341919));
#33498=CARTESIAN_POINT('Ctrl Pts',(-0.945056057322434,-2.33338280919564,
104.578516260256));
#33499=CARTESIAN_POINT('Ctrl Pts',(-0.944646797051759,-2.33354853015362,
104.578544098091));
#33500=CARTESIAN_POINT('Ctrl Pts',(-0.944412731158613,-2.33364326900832,
104.57856001707));
#33501=CARTESIAN_POINT('Ctrl Pts',(-0.943865901467322,-2.33386450417965,
104.578597202294));
#33502=CARTESIAN_POINT('Ctrl Pts',(-0.943553126433803,-2.33399097286593,
104.578618467611));
#33503=CARTESIAN_POINT('Ctrl Pts',(-0.942822351462466,-2.33428628638717,
104.578668143423));
#33504=CARTESIAN_POINT('Ctrl Pts',(-0.942404331476356,-2.33445508186545,
104.578696552262));
#33505=CARTESIAN_POINT('Ctrl Pts',(-0.931175254538073,-2.3389858488409,
104.579459501581));
#33506=CARTESIAN_POINT('Ctrl Pts',(-0.920333931203409,-2.3432728433032,
104.580191520365));
#33507=CARTESIAN_POINT('Ctrl Pts',(-0.895558632189609,-2.35287129652931,
104.581854153513));
#33508=CARTESIAN_POINT('Ctrl Pts',(-0.88160637719201,-2.35813460440708,
104.582783148238));
#33509=CARTESIAN_POINT('Ctrl Pts',(-0.838480638018669,-2.37396697850917,
104.585632796169));
#33510=CARTESIAN_POINT('Ctrl Pts',(-0.809157214191989,-2.3841211645656,
104.587539804161));
#33511=CARTESIAN_POINT('Ctrl Pts',(-0.585919781147914,-2.45683093528707,
104.601845315785));
#33512=CARTESIAN_POINT('Ctrl Pts',(-0.385245473996142,-2.49618004428777,
104.613421818613));
#33513=CARTESIAN_POINT('Ctrl Pts',(-0.0528506681205948,-2.52027423854299,
104.632617043671));
#33514=CARTESIAN_POINT('Ctrl Pts',(0.0768201698871136,-2.51965581059027,
104.640134829666));
#33515=CARTESIAN_POINT('Ctrl Pts',(0.223761401582444,-2.50760046651374,
104.649235348058));
#33516=CARTESIAN_POINT('Ctrl Pts',(0.241656982558344,-2.50593917017126,
104.650353671097));
#33517=CARTESIAN_POINT('Ctrl Pts',(0.26793630722683,-2.50321548521441,104.652012623391));
#33518=CARTESIAN_POINT('Ctrl Pts',(0.276335387717901,-2.5023022157141,104.652545353551));
#33519=CARTESIAN_POINT('Ctrl Pts',(0.291213183389695,-2.50060866866025,
104.653493723728));
#33520=CARTESIAN_POINT('Ctrl Pts',(0.297693673143479,-2.49984545673397,
104.653908413365));
#33521=CARTESIAN_POINT('Ctrl Pts',(0.311744289574365,-2.4981352942714,104.654811049956));
#33522=CARTESIAN_POINT('Ctrl Pts',(0.319312982675524,-2.49717914175093,
104.655299479174));
#33523=CARTESIAN_POINT('Ctrl Pts',(0.340305308334726,-2.49443018666976,
104.656660071816));
#33524=CARTESIAN_POINT('Ctrl Pts',(0.353718767410586,-2.49256347430356,
104.657536150878));
#33525=CARTESIAN_POINT('Ctrl Pts',(0.428274013284006,-2.4815739297311,104.6624405244));
#33526=CARTESIAN_POINT('Ctrl Pts',(0.489073902976107,-2.47031033844066,
104.666570544537));
#33527=CARTESIAN_POINT('Ctrl Pts',(0.72300867334983,-2.41799809231037,104.682820772379));
#33528=CARTESIAN_POINT('Ctrl Pts',(0.892022280454537,-2.36088061983492,
104.695292560618));
#33529=CARTESIAN_POINT('Ctrl Pts',(1.1566397939054,-2.23894173065663,104.715092162913));
#33530=CARTESIAN_POINT('Ctrl Pts',(1.25635434969884,-2.18454931396937,104.722634943283));
#33531=CARTESIAN_POINT('Ctrl Pts',(1.37159134604528,-2.111179505125,104.731432106561));
#33532=CARTESIAN_POINT('Ctrl Pts',(1.39093930183575,-2.09848269957238,104.732912379732));
#33533=CARTESIAN_POINT('Ctrl Pts',(1.42112940635216,-2.07806987394011,104.735227989854));
#33534=CARTESIAN_POINT('Ctrl Pts',(1.43208976878401,-2.07053183886651,104.736069897385));
#33535=CARTESIAN_POINT('Ctrl Pts',(1.4525019688657,-2.05625363868356,104.73764036755));
#33536=CARTESIAN_POINT('Ctrl Pts',(1.46196788666106,-2.0495343133963,104.738369689694));
#33537=CARTESIAN_POINT('Ctrl Pts',(1.48306088740548,-2.03434108137355,104.739997363864));
#33538=CARTESIAN_POINT('Ctrl Pts',(1.49466254736297,-2.02583244968708,104.740894359008));
#33539=CARTESIAN_POINT('Ctrl Pts',(1.52400650935799,-2.00392234392493,104.743168037876));
#33540=CARTESIAN_POINT('Ctrl Pts',(1.54164560485165,-1.99038425396033,104.744539416419));
#33541=CARTESIAN_POINT('Ctrl Pts',(1.68579856627099,-1.87668001410425,104.755792241897));
#33542=CARTESIAN_POINT('Ctrl Pts',(1.80259850823902,-1.76479254080282,104.765169338915));
#33543=CARTESIAN_POINT('Ctrl Pts',(1.98924918055955,-1.54798015692163,104.781627760049));
#33544=CARTESIAN_POINT('Ctrl Pts',(2.06346452103391,-1.44757227243226,104.788733640141));
#33545=CARTESIAN_POINT('Ctrl Pts',(2.15318648358678,-1.30518085087529,104.798687823221));
#33546=CARTESIAN_POINT('Ctrl Pts',(2.17547683047469,-1.26767867569951,104.801299750945));
#33547=CARTESIAN_POINT('Ctrl Pts',(2.2103693348331,-1.20534131971021,104.805656966285));
#33548=CARTESIAN_POINT('Ctrl Pts',(2.22355418953852,-1.18084161150694,104.807373262537));
#33549=CARTESIAN_POINT('Ctrl Pts',(2.24094307285037,-1.14720587126872,104.809741627424));
#33550=CARTESIAN_POINT('Ctrl Pts',(2.24550290235323,-1.13825474931395,104.810373040634));
#33551=CARTESIAN_POINT('Ctrl Pts',(2.25305177911631,-1.12321411363711,104.811436322397));
#33552=CARTESIAN_POINT('Ctrl Pts',(2.25607006405686,-1.11713926110719,104.811866405819));
#33553=CARTESIAN_POINT('Ctrl Pts',(2.2617621010825,-1.10556584199093,104.81268710315));
#33554=CARTESIAN_POINT('Ctrl Pts',(2.26444043949696,-1.10006960094475,104.81307741631));
#33555=CARTESIAN_POINT('Ctrl Pts',(2.27076518559023,-1.08696956552533,104.814008948343));
#33556=CARTESIAN_POINT('Ctrl Pts',(2.27439343345416,-1.07935715567501,104.814551248814));
#33557=CARTESIAN_POINT('Ctrl Pts',(2.28712477982981,-1.05229634620056,104.8164821568));
#33558=CARTESIAN_POINT('Ctrl Pts',(2.29601692548621,-1.03275048511012,104.817882532695));
#33559=CARTESIAN_POINT('Ctrl Pts',(2.35652724839298,-0.89509734690931,104.82777244643));
#33560=CARTESIAN_POINT('Ctrl Pts',(2.39925346854901,-0.773302294330039,
104.836654676793));
#33561=CARTESIAN_POINT('Ctrl Pts',(2.46931439236541,-0.510625801779804,
104.855434305709));
#33562=CARTESIAN_POINT('Ctrl Pts',(2.49433017729159,-0.369563542430787,
104.865296078724));
#33563=CARTESIAN_POINT('Ctrl Pts',(2.51385894751855,-0.153989521823215,
104.879741376855));
#33564=CARTESIAN_POINT('Ctrl Pts',(2.51728161193147,-0.0805894472093046,
104.88455613113));
#33565=CARTESIAN_POINT('Ctrl Pts',(2.51754801788225,0.0133656453069901,
104.890589233768));
#33566=CARTESIAN_POINT('Ctrl Pts',(2.51735566210889,0.0338699555761138,
104.89189807357));
#33567=CARTESIAN_POINT('Ctrl Pts',(2.51663792898245,0.0670953968228259,
104.894006799795));
#33568=CARTESIAN_POINT('Ctrl Pts',(2.51626653245155,0.0798185767291909,
104.894811421546));
#33569=CARTESIAN_POINT('Ctrl Pts',(2.51536785665976,0.104250410665722,104.896351153088));
#33570=CARTESIAN_POINT('Ctrl Pts',(2.51485527703259,0.115959240586989,104.897086698517));
#33571=CARTESIAN_POINT('Ctrl Pts',(2.51349362407948,0.142776078541068,104.898766112685));
#33572=CARTESIAN_POINT('Ctrl Pts',(2.51259006313106,0.157880959224034,104.899708266891));
#33573=CARTESIAN_POINT('Ctrl Pts',(2.50927696888736,0.205985627054936,104.90269736361));
#33574=CARTESIAN_POINT('Ctrl Pts',(2.50635299467243,0.238947289144724,104.904728361448));
#33575=CARTESIAN_POINT('Ctrl Pts',(2.48427372609774,0.442224775271648,104.917165384629));
#33576=CARTESIAN_POINT('Ctrl Pts',(2.44841789532362,0.61027616968858,104.927022652062));
#33577=CARTESIAN_POINT('Ctrl Pts',(2.36539923989853,0.867444251348764,104.942549959779));
#33578=CARTESIAN_POINT('Ctrl Pts',(2.32952862069943,0.959618406818162,104.948221790185));
#33579=CARTESIAN_POINT('Ctrl Pts',(2.26953520044176,1.0904358375706,104.956722348909));
#33580=CARTESIAN_POINT('Ctrl Pts',(2.24963730313713,1.13091639256554,104.959419483739));
#33581=CARTESIAN_POINT('Ctrl Pts',(2.21541065616835,1.19606603827347,104.963904857656));
#33582=CARTESIAN_POINT('Ctrl Pts',(2.20173040474449,1.22106568607888,104.965661910853));
#33583=CARTESIAN_POINT('Ctrl Pts',(2.18261239492136,1.25463626855605,104.968077826023));
#33584=CARTESIAN_POINT('Ctrl Pts',(2.1775422749966,1.26341547608539,104.968714947705));
#33585=CARTESIAN_POINT('Ctrl Pts',(2.16898186732908,1.27803371762194,104.969785154701));
#33586=CARTESIAN_POINT('Ctrl Pts',(2.16552062631111,1.28388976909503,104.970216403368));
#33587=CARTESIAN_POINT('Ctrl Pts',(2.15891186501839,1.29496833567877,104.971037185294));
#33588=CARTESIAN_POINT('Ctrl Pts',(2.15576902399851,1.30019357966128,104.971426404097));
#33589=CARTESIAN_POINT('Ctrl Pts',(2.14826837977797,1.31256208828681,104.972352594519));
#33590=CARTESIAN_POINT('Ctrl Pts',(2.14389391624238,1.31969509294647,104.972890619782));
#33591=CARTESIAN_POINT('Ctrl Pts',(2.1283732376717,1.34472229610727,104.97479171101));
#33592=CARTESIAN_POINT('Ctrl Pts',(2.11703823794499,1.36249760481806,104.976166090807));
#33593=CARTESIAN_POINT('Ctrl Pts',(2.0238963654023,1.50459206985361,104.987335888974));
#33594=CARTESIAN_POINT('Ctrl Pts',(1.93144244473804,1.62156599097165,104.997654366076));
#33595=CARTESIAN_POINT('Ctrl Pts',(1.70246116578491,1.86372352780306,105.020671661358));
#33596=CARTESIAN_POINT('Ctrl Pts',(1.56133922687283,1.98345234380917,105.033250747543));
#33597=CARTESIAN_POINT('Ctrl Pts',(1.38547032736212,2.10215169548993,105.046973723862));
#33598=CARTESIAN_POINT('Ctrl Pts',(1.36231316589544,2.11723232456532,105.04874692172));
#33599=CARTESIAN_POINT('Ctrl Pts',(1.3268490498326,2.13950478974092,105.051412855372));
#33600=CARTESIAN_POINT('Ctrl Pts',(1.31472218944968,2.1469780447203,105.052315858959));
#33601=CARTESIAN_POINT('Ctrl Pts',(1.29260678411515,2.1603491572363,105.053947339268));
#33602=CARTESIAN_POINT('Ctrl Pts',(1.28263973558793,2.1662816288428,105.054677058231));
#33603=CARTESIAN_POINT('Ctrl Pts',(1.26106254025512,2.17892343044826,105.056245025315));
#33604=CARTESIAN_POINT('Ctrl Pts',(1.24943903019509,2.18560933541595,105.057082415493));
#33605=CARTESIAN_POINT('Ctrl Pts',(1.2177196178447,2.20351876873095,105.059348323905));
#33606=CARTESIAN_POINT('Ctrl Pts',(1.19752201611124,2.21456025131756,105.060770369337));
#33607=CARTESIAN_POINT('Ctrl Pts',(1.08802984425337,2.27248058597765,105.068373070932));
#33608=CARTESIAN_POINT('Ctrl Pts',(0.996125567614707,2.31424160906338,105.07437313917));
#33609=CARTESIAN_POINT('Ctrl Pts',(0.745434497035487,2.4104439287012,105.090059656377));
#33610=CARTESIAN_POINT('Ctrl Pts',(0.583314222531473,2.45472067248762,105.099497837987));
#33611=CARTESIAN_POINT('Ctrl Pts',(0.362245593961423,2.49194328174458,105.112619621451));
#33612=CARTESIAN_POINT('Ctrl Pts',(0.306191907154722,2.49944971927846,105.115970895383));
#33613=CARTESIAN_POINT('Ctrl Pts',(0.227532768844672,2.5072977543434,105.120764643803));
#33614=CARTESIAN_POINT('Ctrl Pts',(0.205100498085318,2.50923233337952,105.12214204862));
#33615=CARTESIAN_POINT('Ctrl Pts',(0.165768996766808,2.51209339676708,105.124579824829));
#33616=CARTESIAN_POINT('Ctrl Pts',(0.148880456153644,2.51315084470318,105.125633899139));
#33617=CARTESIAN_POINT('Ctrl Pts',(0.12374846507899,2.51447023507061,105.127215050591));
#33618=CARTESIAN_POINT('Ctrl Pts',(0.115511919892945,2.51486207126377,105.127735250478));
#33619=CARTESIAN_POINT('Ctrl Pts',(0.10139330866418,2.51546422937995,105.128630611878));
#33620=CARTESIAN_POINT('Ctrl Pts',(0.0955122084070213,2.51569439904605,
105.129004670631));
#33621=CARTESIAN_POINT('Ctrl Pts',(0.0821137823100427,2.51617172421599,
105.129859406256));
#33622=CARTESIAN_POINT('Ctrl Pts',(0.0745962689008002,2.51640581229185,
105.130340782879));
#33623=CARTESIAN_POINT('Ctrl Pts',(0.0540130574060407,2.51695443979007,
105.131663546601));
#33624=CARTESIAN_POINT('Ctrl Pts',(0.0409459926615565,2.51720091981361,
105.132508516053));
#33625=CARTESIAN_POINT('Ctrl Pts',(-0.0266678848650488,2.51794969876221,
105.136905709292));
#33626=CARTESIAN_POINT('Ctrl Pts',(-0.0812146599716767,2.51678069612995,
105.140537058365));
#33627=CARTESIAN_POINT('Ctrl Pts',(-0.349818292313885,2.50228376583181,
105.158700921316));
#33628=CARTESIAN_POINT('Ctrl Pts',(-0.561613107896594,2.46341283872791,
105.173813682377));
#33629=CARTESIAN_POINT('Ctrl Pts',(-0.821319004749718,2.38046668827618,
105.192141388752));
#33630=CARTESIAN_POINT('Ctrl Pts',(-0.876076989834283,2.36086350903953,
105.196000664315));
#33631=CARTESIAN_POINT('Ctrl Pts',(-0.967768752494942,2.32440792596896,
105.202450348893));
#33632=CARTESIAN_POINT('Ctrl Pts',(-1.0050615898854,2.30852768580505,105.205070055219));
#33633=CARTESIAN_POINT('Ctrl Pts',(-1.05703555986599,2.28489747057786,105.208718066688));
#33634=CARTESIAN_POINT('Ctrl Pts',(-1.07204677304168,2.27789296580849,105.209771353353));
#33635=CARTESIAN_POINT('Ctrl Pts',(-1.09773316138717,2.2655970670739,105.211573412267));
#33636=CARTESIAN_POINT('Ctrl Pts',(-1.10844176623854,2.26037718593465,105.212324606801));
#33637=CARTESIAN_POINT('Ctrl Pts',(-1.12884317540422,2.25025272505381,105.213755745863));
#33638=CARTESIAN_POINT('Ctrl Pts',(-1.13854204952455,2.24536105084339,105.214436115717));
#33639=CARTESIAN_POINT('Ctrl Pts',(-1.16121066431388,2.23374337916769,105.216026484743));
#33640=CARTESIAN_POINT('Ctrl Pts',(-1.17415420572936,2.22696690728908,105.216934707069));
#33641=CARTESIAN_POINT('Ctrl Pts',(-1.21223835509208,2.2066039556023,105.219608012372));
#33642=CARTESIAN_POINT('Ctrl Pts',(-1.23720795864221,2.19270139642965,105.221362041804));
#33643=CARTESIAN_POINT('Ctrl Pts',(-1.43230114220424,2.07968365901404,105.235091694373));
#33644=CARTESIAN_POINT('Ctrl Pts',(-1.59050117252569,1.96134789102037,105.246306601521));
#33645=CARTESIAN_POINT('Ctrl Pts',(-1.83285101434336,1.73127218128131,105.265537561742));
#33646=CARTESIAN_POINT('Ctrl Pts',(-1.92448718562338,1.62879864978661,105.273484019249));
#33647=CARTESIAN_POINT('Ctrl Pts',(-2.01737907981476,1.50607654231052,105.283001658974));
#33648=CARTESIAN_POINT('Ctrl Pts',(-2.02732080192222,1.49266715463548,105.284041732361));
#33649=CARTESIAN_POINT('Ctrl Pts',(-2.04194656879639,1.47252426623806,105.285605883881));
#33650=CARTESIAN_POINT('Ctrl Pts',(-2.04673247305317,1.46586482451579,105.286123298558));
#33651=CARTESIAN_POINT('Ctrl Pts',(-2.05489438791523,1.45438986883172,105.287015581725));
#33652=CARTESIAN_POINT('Ctrl Pts',(-2.0582861883408,1.44958573457389,105.287389369799));
#33653=CARTESIAN_POINT('Ctrl Pts',(-2.06599586401125,1.43858416158218,105.288245907235));
#33654=CARTESIAN_POINT('Ctrl Pts',(-2.07030261921346,1.43237926590076,105.288729374126));
#33655=CARTESIAN_POINT('Ctrl Pts',(-2.0820643543736,1.41526985426939,105.290063317241));
#33656=CARTESIAN_POINT('Ctrl Pts',(-2.08946141076274,1.40432607724334,105.290917472962));
#33657=CARTESIAN_POINT('Ctrl Pts',(-2.12808095540209,1.34620871086016,105.295456201663));
#33658=CARTESIAN_POINT('Ctrl Pts',(-2.15779058112502,1.29805438528717,105.299225912155));
#33659=CARTESIAN_POINT('Ctrl Pts',(-2.25471729885706,1.12841730702219,105.31243368686));
#33660=CARTESIAN_POINT('Ctrl Pts',(-2.31341953218434,1.00253803793281,105.322096532151));
#33661=CARTESIAN_POINT('Ctrl Pts',(-2.36143106504627,0.872610780952442,
105.331623435588));
#33662=CARTESIAN_POINT('Origin',(0.,0.,104.));
#33663=CARTESIAN_POINT('',(-2.36143111532954,0.872610644877486,106.333142274553));
#33664=CARTESIAN_POINT('',(-2.36143112101026,0.872610629504504,106.056155979185));
#33665=CARTESIAN_POINT('',(-2.36143112101026,0.872610629504505,104.));
#33666=CARTESIAN_POINT('',(-2.51749930935125,-0.00186478308576427,105.112583302455));
#33667=CARTESIAN_POINT('Ctrl Pts',(-2.36143112101026,0.872610629504504,
106.056155979185));
#33668=CARTESIAN_POINT('Ctrl Pts',(-2.3320450272244,0.952134341506782,106.050793423265));
#33669=CARTESIAN_POINT('Ctrl Pts',(-2.29860300576651,1.03026510446364,106.045430867345));
#33670=CARTESIAN_POINT('Ctrl Pts',(-2.26126535934404,1.10656460481558,106.040068311425));
#33671=CARTESIAN_POINT('Ctrl Pts',(-2.22479013631369,1.18110174250636,106.034829619597));
#33672=CARTESIAN_POINT('Ctrl Pts',(-2.18459753161513,1.25389086788927,106.029590927769));
#33673=CARTESIAN_POINT('Ctrl Pts',(-2.14088583146978,1.3245429802811,106.024352235941));
#33674=CARTESIAN_POINT('Ctrl Pts',(-2.09718985896252,1.39516967177075,106.019115429014));
#33675=CARTESIAN_POINT('Ctrl Pts',(-2.04997754811381,1.46366048524139,106.013878622088));
#33676=CARTESIAN_POINT('Ctrl Pts',(-1.99949227582444,1.52965253862385,106.008641815161));
#33677=CARTESIAN_POINT('Ctrl Pts',(-1.94900993972484,1.5956407539525,106.003405312804));
#33678=CARTESIAN_POINT('Ctrl Pts',(-1.89525530153011,1.65913013206876,105.998168810447));
#33679=CARTESIAN_POINT('Ctrl Pts',(-1.83851322315744,1.71978934124946,105.99293230809));
#33680=CARTESIAN_POINT('Ctrl Pts',(-1.7793875752057,1.78299666727467,105.987475835508));
#33681=CARTESIAN_POINT('Ctrl Pts',(-1.71701832140262,1.84313039699446,105.982019362926));
#33682=CARTESIAN_POINT('Ctrl Pts',(-1.65177038710584,1.8998581100388,105.976562890344));
#33683=CARTESIAN_POINT('Ctrl Pts',(-1.58906500733386,1.95437528101715,105.97131904333));
#33684=CARTESIAN_POINT('Ctrl Pts',(-1.52370154234258,2.005746707741,105.966075196316));
#33685=CARTESIAN_POINT('Ctrl Pts',(-1.45603627926231,2.0537196993436,105.960831349301));
#33686=CARTESIAN_POINT('Ctrl Pts',(-1.38832327795329,2.10172653616519,105.955583802723));
#33687=CARTESIAN_POINT('Ctrl Pts',(-1.31830563575006,2.14632991980948,105.950336256144));
#33688=CARTESIAN_POINT('Ctrl Pts',(-1.24636624928542,2.18732197507413,105.945088709566));
#33689=CARTESIAN_POINT('Ctrl Pts',(-1.17431585319227,2.22837728515718,105.939833065501));
#33690=CARTESIAN_POINT('Ctrl Pts',(-1.10033820878909,2.2658099456108,105.934577421437));
#33691=CARTESIAN_POINT('Ctrl Pts',(-1.02483761825963,2.29945952480141,105.929321777372));
#33692=CARTESIAN_POINT('Ctrl Pts',(-1.01589674182243,2.30344435098088,105.928699397284));
#33693=CARTESIAN_POINT('Ctrl Pts',(-1.00693452631,2.30737618201483,105.928077017196));
#33694=CARTESIAN_POINT('Ctrl Pts',(-0.997951656852982,2.31125479784994,
105.927454637108));
#33695=CARTESIAN_POINT('Ctrl Pts',(-0.922102155402193,2.34400503192829,
105.922199387701));
#33696=CARTESIAN_POINT('Ctrl Pts',(-0.844498702622488,2.37307800987231,
105.916944138294));
#33697=CARTESIAN_POINT('Ctrl Pts',(-0.765532238206415,2.39828410374307,
105.911688888886));
#33698=CARTESIAN_POINT('Ctrl Pts',(-0.68667773029783,2.42345446109886,105.906441090229));
#33699=CARTESIAN_POINT('Ctrl Pts',(-0.606464485047457,2.44476868481448,
105.901193291571));
#33700=CARTESIAN_POINT('Ctrl Pts',(-0.525304183161289,2.46208484117693,
105.895945492914));
#33701=CARTESIAN_POINT('Ctrl Pts',(-0.443555804919529,2.47952646802052,
105.890659669431));
#33702=CARTESIAN_POINT('Ctrl Pts',(-0.360847022713129,2.49291165629843,
105.885373845948));
#33703=CARTESIAN_POINT('Ctrl Pts',(-0.277614991355664,2.50214631198389,
105.880088022465));
#33704=CARTESIAN_POINT('Ctrl Pts',(-0.195129295878244,2.51129816114925,
105.874849596596));
#33705=CARTESIAN_POINT('Ctrl Pts',(-0.112130164600841,2.51637356285532,
105.869611170728));
#33706=CARTESIAN_POINT('Ctrl Pts',(-0.0290524157146699,2.5173323592925,
105.864372744859));
#33707=CARTESIAN_POINT('Ctrl Pts',(0.0539980102825035,2.51829084039748,
105.859136041822));
#33708=CARTESIAN_POINT('Ctrl Pts',(0.137126541510933,2.51513539979876,105.853899338784));
#33709=CARTESIAN_POINT('Ctrl Pts',(0.2198963861406,2.50787795344237,105.848662635747));
#33710=CARTESIAN_POINT('Ctrl Pts',(0.302663976161101,2.50062070477519,105.843426075354));
#33711=CARTESIAN_POINT('Ctrl Pts',(0.385072439441943,2.4892617138423,105.838189514962));
#33712=CARTESIAN_POINT('Ctrl Pts',(0.466689528308689,2.47386481727822,105.83295295457));
#33713=CARTESIAN_POINT('Ctrl Pts',(0.549642468916212,2.45821591502069,105.827630685799));
#33714=CARTESIAN_POINT('Ctrl Pts',(0.631777410420446,2.43839581358489,105.822308417029));
#33715=CARTESIAN_POINT('Ctrl Pts',(0.712652561784847,2.41452533144332,105.816986148258));
#33716=CARTESIAN_POINT('Ctrl Pts',(0.792339598035796,2.39100552413969,105.811742067508));
#33717=CARTESIAN_POINT('Ctrl Pts',(0.870803191428542,2.36355376477662,105.806497986758));
#33718=CARTESIAN_POINT('Ctrl Pts',(0.947638970692687,2.33233501693571,105.801253906007));
#33719=CARTESIAN_POINT('Ctrl Pts',(1.02619315526263,2.3004180727279,105.795892543227));
#33720=CARTESIAN_POINT('Ctrl Pts',(1.1030453720852,2.26456382854632,105.790531180446));
#33721=CARTESIAN_POINT('Ctrl Pts',(1.17778988319344,2.22499825641442,105.785169817666));
#33722=CARTESIAN_POINT('Ctrl Pts',(1.25253439430167,2.18543268428251,105.779808454885));
#33723=CARTESIAN_POINT('Ctrl Pts',(1.32517079738007,2.14215610165379,105.774447092105));
#33724=CARTESIAN_POINT('Ctrl Pts',(1.39532635611388,2.09544043340152,105.769085729324));
#33725=CARTESIAN_POINT('Ctrl Pts',(1.46409337926563,2.04964937281796,105.763830479917));
#33726=CARTESIAN_POINT('Ctrl Pts',(1.53073088988028,2.00038502354845,105.758575230509));
#33727=CARTESIAN_POINT('Ctrl Pts',(1.59486698177971,1.94787205956368,105.753319981102));
#33728=CARTESIAN_POINT('Ctrl Pts',(1.65891214327077,1.89543354703236,105.748072182445));
#33729=CARTESIAN_POINT('Ctrl Pts',(1.72046257628061,1.8397558581212,105.742824383787));
#33730=CARTESIAN_POINT('Ctrl Pts',(1.77917508770272,1.78110703139874,105.73757658513));
#33731=CARTESIAN_POINT('Ctrl Pts',(1.83831302188627,1.72203324336537,105.732290761647));
#33732=CARTESIAN_POINT('Ctrl Pts',(1.89457134013341,1.65994534158647,105.727004938164));
#33733=CARTESIAN_POINT('Ctrl Pts',(1.9476331074797,1.59515877850733,105.721719114681));
#33734=CARTESIAN_POINT('Ctrl Pts',(2.00021907362082,1.53095315206737,105.716480688812));
#33735=CARTESIAN_POINT('Ctrl Pts',(2.04966528800493,1.46409743145675,105.711242262944));
#33736=CARTESIAN_POINT('Ctrl Pts',(2.09570132912817,1.39493447483759,105.706003837075));
#33737=CARTESIAN_POINT('Ctrl Pts',(2.14172222976363,1.32579426476382,105.700767134038));
#33738=CARTESIAN_POINT('Ctrl Pts',(2.18433492912726,1.25434870953106,105.695530431));
#33739=CARTESIAN_POINT('Ctrl Pts',(2.22331161022896,1.18097067441199,105.690293727963));
#33740=CARTESIAN_POINT('Ctrl Pts',(2.26228722962535,1.10759463807392,105.68505716757));
#33741=CARTESIAN_POINT('Ctrl Pts',(2.29762681213943,1.03228663449493,105.679820607178));
#33742=CARTESIAN_POINT('Ctrl Pts',(2.32914856552666,0.955443985644953,105.674584046786));
#33743=CARTESIAN_POINT('Ctrl Pts',(2.36118624504798,0.877343629767458,105.669261778015));
#33744=CARTESIAN_POINT('Ctrl Pts',(2.3892797939899,0.79765838932308,105.663939509245));
#33745=CARTESIAN_POINT('Ctrl Pts',(2.41329002013555,0.716824615030886,105.658617240474));
#33746=CARTESIAN_POINT('Ctrl Pts',(2.43694751850165,0.637178347992719,105.653373159724));
#33747=CARTESIAN_POINT('Ctrl Pts',(2.45664082044059,0.556417537948684,105.648129078974));
#33748=CARTESIAN_POINT('Ctrl Pts',(2.47228813556255,0.474971183080256,105.642884998223));
#33749=CARTESIAN_POINT('Ctrl Pts',(2.48828539740965,0.391703308996611,105.637523635443));
#33750=CARTESIAN_POINT('Ctrl Pts',(2.50005344341742,0.307719363212086,105.632162272662));
#33751=CARTESIAN_POINT('Ctrl Pts',(2.50756091250629,0.22348270642411,105.626800909882));
#33752=CARTESIAN_POINT('Ctrl Pts',(2.51506838159515,0.139246049636133,105.621439547101));
#33753=CARTESIAN_POINT('Ctrl Pts',(2.51831532100137,0.0547571921418939,
105.616078184321));
#33754=CARTESIAN_POINT('Ctrl Pts',(2.51732688234237,-0.0295231677916568,
105.61071682154));
#33755=CARTESIAN_POINT('Ctrl Pts',(2.51635800709749,-0.112135430702664,
105.605461572133));
#33756=CARTESIAN_POINT('Ctrl Pts',(2.51131634767354,-0.194852512373357,
105.600206322725));
#33757=CARTESIAN_POINT('Ctrl Pts',(2.50218787396461,-0.277240136676642,
105.594951073318));
#33758=CARTESIAN_POINT('Ctrl Pts',(2.49307234235765,-0.359510954044879,
105.589703274661));
#33759=CARTESIAN_POINT('Ctrl Pts',(2.47988155577697,-0.441452787045925,
105.584455476003));
#33760=CARTESIAN_POINT('Ctrl Pts',(2.4626534908834,-0.522631833932654,105.579207677346));
#33761=CARTESIAN_POINT('Ctrl Pts',(2.44530059380732,-0.604399092998717,
105.573921853863));
#33762=CARTESIAN_POINT('Ctrl Pts',(2.42385166998305,-0.685391991366922,
105.56863603038));
#33763=CARTESIAN_POINT('Ctrl Pts',(2.3983987627519,-0.76517293785794,105.563350206897));
#33764=CARTESIAN_POINT('Ctrl Pts',(2.373174089983,-0.84423849410868,105.558111781028));
#33765=CARTESIAN_POINT('Ctrl Pts',(2.34401709592337,-0.922113298716373,
105.55287335516));
#33766=CARTESIAN_POINT('Ctrl Pts',(2.31106813594437,-0.998383854548242,
105.547634929291));
#33767=CARTESIAN_POINT('Ctrl Pts',(2.27813001232997,-1.07462932626362,105.542398226254));
#33768=CARTESIAN_POINT('Ctrl Pts',(2.24140258247874,-1.14927117381638,105.537161523216));
#33769=CARTESIAN_POINT('Ctrl Pts',(2.20107456758893,-1.22191529899303,105.531924820179));
#33770=CARTESIAN_POINT('Ctrl Pts',(2.16074765121408,-1.29455744538003,105.526688259786));
#33771=CARTESIAN_POINT('Ctrl Pts',(2.11682056966576,-1.36520157466171,105.521451699394));
#33772=CARTESIAN_POINT('Ctrl Pts',(2.06952761647574,-1.43347887833907,105.516215139002));
#33773=CARTESIAN_POINT('Ctrl Pts',(2.02146060512309,-1.50287369743192,105.510892870231));
#33774=CARTESIAN_POINT('Ctrl Pts',(1.96991681677193,-1.56982310309953,105.505570601461));
#33775=CARTESIAN_POINT('Ctrl Pts',(1.9151864756193,-1.63397277015406,105.50024833269));
#33776=CARTESIAN_POINT('Ctrl Pts',(1.86126016319977,-1.69718003169011,105.49500425194));
#33777=CARTESIAN_POINT('Ctrl Pts',(1.80424066777238,-1.7576689705255,105.48976017119));
#33778=CARTESIAN_POINT('Ctrl Pts',(1.74444329879669,-1.81513741278266,105.484516090439));
#33779=CARTESIAN_POINT('Ctrl Pts',(1.68330858259673,-1.87389111663331,105.479154727659));
#33780=CARTESIAN_POINT('Ctrl Pts',(1.61927062781272,-1.9294872532209,105.473793364878));
#33781=CARTESIAN_POINT('Ctrl Pts',(1.55270102323422,-1.98164723965882,105.468432002097));
#33782=CARTESIAN_POINT('Ctrl Pts',(1.48613141865572,-2.03380722609673,105.463070639317));
#33783=CARTESIAN_POINT('Ctrl Pts',(1.41703061803392,-2.08253082417426,105.457709276536));
#33784=CARTESIAN_POINT('Ctrl Pts',(1.3457987453583,-2.12758830298346,105.452347913756));
#33785=CARTESIAN_POINT('Ctrl Pts',(1.27597671092749,-2.1717539934056,105.447092664348));
#33786=CARTESIAN_POINT('Ctrl Pts',(1.20384932162565,-2.21256053261647,105.441837414941));
#33787=CARTESIAN_POINT('Ctrl Pts',(1.12977320620474,-2.24975970995612,105.436582165534));
#33788=CARTESIAN_POINT('Ctrl Pts',(1.05580211388747,-2.28690614731293,105.431334366876));
#33789=CARTESIAN_POINT('Ctrl Pts',(0.979888192187262,-2.32045517618535,
105.426086568219));
#33790=CARTESIAN_POINT('Ctrl Pts',(0.90241598711519,-2.35020246706511,105.420838769561));
#33791=CARTESIAN_POINT('Ctrl Pts',(0.824382429128403,-2.38016530271249,
105.415552946078));
#33792=CARTESIAN_POINT('Ctrl Pts',(0.744768310763816,-2.40627082083284,
105.410267122595));
#33793=CARTESIAN_POINT('Ctrl Pts',(0.663990793267582,-2.42835797947005,
105.404981299112));
#33794=CARTESIAN_POINT('Ctrl Pts',(0.583937602195017,-2.45024708408035,
105.399742873244));
#33795=CARTESIAN_POINT('Ctrl Pts',(0.502742245948962,-2.46818948133825,
105.394504447375));
#33796=CARTESIAN_POINT('Ctrl Pts',(0.420827979435382,-2.48207777108703,
105.389266021507));
#33797=CARTESIAN_POINT('Ctrl Pts',(0.338940653160792,-2.49596149320844,
105.384029318469));
#33798=CARTESIAN_POINT('Ctrl Pts',(0.256335340766251,-2.50579367881354,
105.378792615431));
#33799=CARTESIAN_POINT('Ctrl Pts',(0.173445358343819,-2.51151805839994,
105.373555912394));
#33800=CARTESIAN_POINT('Ctrl Pts',(0.090557633803088,-2.51724228205709,
105.368319352002));
#33801=CARTESIAN_POINT('Ctrl Pts',(0.00738571504727582,-2.51885889140939,
105.363082791609));
#33802=CARTESIAN_POINT('Ctrl Pts',(-0.0756334827208372,-2.51636361170072,
105.357846231217));
#33803=CARTESIAN_POINT('Ctrl Pts',(-0.160011480972994,-2.51382749098941,
105.352523962446));
#33804=CARTESIAN_POINT('Ctrl Pts',(-0.244231221974189,-2.50704366739769,
105.347201693676));
#33805=CARTESIAN_POINT('Ctrl Pts',(-0.327837487473301,-2.49606266584138,
105.341879424905));
#33806=CARTESIAN_POINT('Ctrl Pts',(-0.410215515795193,-2.48524298322779,
105.336635344155));
#33807=CARTESIAN_POINT('Ctrl Pts',(-0.491997524324338,-2.47034876753276,
105.331391263405));
#33808=CARTESIAN_POINT('Ctrl Pts',(-0.572758381215976,-2.45147997885907,
105.326147182654));
#33809=CARTESIAN_POINT('Ctrl Pts',(-0.65532542640052,-2.43218919633198,
105.320785819874));
#33810=CARTESIAN_POINT('Ctrl Pts',(-0.736824601304015,-2.4087440572531,
105.315424457093));
#33811=CARTESIAN_POINT('Ctrl Pts',(-0.816819920653845,-2.38130457254486,
105.310063094313));
#33812=CARTESIAN_POINT('Ctrl Pts',(-0.896815240003676,-2.35386508783662,
105.304701731532));
#33813=CARTESIAN_POINT('Ctrl Pts',(-0.975306256944999,-2.32243150840783,
105.299340368751));
#33814=CARTESIAN_POINT('Ctrl Pts',(-1.05188242683387,-2.28721437782253,
105.293979005971));
#33815=CARTESIAN_POINT('Ctrl Pts',(-1.1269429828705,-2.25269427310087,105.288723756564));
#33816=CARTESIAN_POINT('Ctrl Pts',(-1.20044106284464,-2.21441155937803,
105.283468507156));
#33817=CARTESIAN_POINT('Ctrl Pts',(-1.2719743024889,-2.17253023541857,105.278213257749));
#33818=CARTESIAN_POINT('Ctrl Pts',(-1.34340612424973,-2.13070828966221,
105.272965459091));
#33819=CARTESIAN_POINT('Ctrl Pts',(-1.41287824401757,-2.08529809894299,
105.267717660434));
#33820=CARTESIAN_POINT('Ctrl Pts',(-1.48000990510123,-2.03651096996855,
105.262469861776));
#33821=CARTESIAN_POINT('Ctrl Pts',(-1.54762799294376,-1.98737033618523,
105.257184038294));
#33822=CARTESIAN_POINT('Ctrl Pts',(-1.61287113116811,-1.93480381800172,
105.251898214811));
#33823=CARTESIAN_POINT('Ctrl Pts',(-1.67537711493227,-1.87907364750859,
105.246612391328));
#33824=CARTESIAN_POINT('Ctrl Pts',(-1.73732261185454,-1.82384320560745,
105.241373965459));
#33825=CARTESIAN_POINT('Ctrl Pts',(-1.79657949470942,-1.76550593339141,
105.236135539591));
#33826=CARTESIAN_POINT('Ctrl Pts',(-1.85282723527973,-1.70435837962726,
105.230897113722));
#33827=CARTESIAN_POINT('Ctrl Pts',(-1.90905647690427,-1.64323093627591,
105.225660410685));
#33828=CARTESIAN_POINT('Ctrl Pts',(-1.9622782296196,-1.57929538632537,105.220423707647));
#33829=CARTESIAN_POINT('Ctrl Pts',(-2.01220937537848,-1.51288455595229,
105.21518700461));
#33830=CARTESIAN_POINT('Ctrl Pts',(-2.06213916103795,-1.44647553457697,
105.209950444217));
#33831=CARTESIAN_POINT('Ctrl Pts',(-2.10877824149203,-1.37759173626612,
105.204713883825));
#33832=CARTESIAN_POINT('Ctrl Pts',(-2.15188515194408,-1.30659731472347,
105.199477323433));
#33833=CARTESIAN_POINT('Ctrl Pts',(-2.19569760632283,-1.23444090587015,
105.194155054662));
#33834=CARTESIAN_POINT('Ctrl Pts',(-2.2358609568884,-1.16010457351394,105.188832785892));
#33835=CARTESIAN_POINT('Ctrl Pts',(-2.27216973926298,-1.08399765958124,
105.183510517121));
#33836=CARTESIAN_POINT('Ctrl Pts',(-2.30794511907369,-1.00900881186736,
105.178266436371));
#33837=CARTESIAN_POINT('Ctrl Pts',(-2.33997830806341,-0.932301515060755,
105.173022355621));
#33838=CARTESIAN_POINT('Ctrl Pts',(-2.36812168829864,-0.854286789907003,
105.16777827487));
#33839=CARTESIAN_POINT('Ctrl Pts',(-2.39689448538084,-0.774527292735347,
105.16241691209));
#33840=CARTESIAN_POINT('Ctrl Pts',(-2.42160123659599,-0.693401671007281,
105.157055549309));
#33841=CARTESIAN_POINT('Ctrl Pts',(-2.44213878500912,-0.611362744002423,
105.151694186529));
#33842=CARTESIAN_POINT('Ctrl Pts',(-2.46267633342225,-0.529323816997564,
105.146332823748));
#33843=CARTESIAN_POINT('Ctrl Pts',(-2.47904464620291,-0.446372096142003,
105.140971460968));
#33844=CARTESIAN_POINT('Ctrl Pts',(-2.49119680399604,-0.362966573887916,
105.135610098187));
#33845=CARTESIAN_POINT('Ctrl Pts',(-2.50859444872508,-0.24355900287716,
105.127934499622));
#33846=CARTESIAN_POINT('Ctrl Pts',(-2.51740967623069,-0.12287148413773,
105.120258901057));
#33847=CARTESIAN_POINT('Ctrl Pts',(-2.51749930935083,-0.00186478366199865,
105.112583302492));
#33848=CARTESIAN_POINT('Ctrl Pts',(-2.51749930935125,-0.00186478308577434,
105.112583302455));
#33849=CARTESIAN_POINT('Ctrl Pts',(-2.5175597065367,0.0796727822241211,
105.107411277957));
#33850=CARTESIAN_POINT('Ctrl Pts',(-2.51365459987842,0.161358302924671,
105.102239253459));
#33851=CARTESIAN_POINT('Ctrl Pts',(-2.50576736565954,0.242767706245406,
105.097067228961));
#33852=CARTESIAN_POINT('Ctrl Pts',(-2.49788815038873,0.324094340656303,
105.091900462859));
#33853=CARTESIAN_POINT('Ctrl Pts',(-2.48603488237869,0.40514494382945,105.086733696756));
#33854=CARTESIAN_POINT('Ctrl Pts',(-2.47024295923186,0.485495594589114,
105.081566930653));
#33855=CARTESIAN_POINT('Ctrl Pts',(-2.45446208158943,0.565790044881075,
105.076403778394));
#33856=CARTESIAN_POINT('Ctrl Pts',(-2.43474810616352,0.645385048417688,
105.071240626135));
#33857=CARTESIAN_POINT('Ctrl Pts',(-2.41118805019035,0.72386354834269,105.066077473876));
#33858=CARTESIAN_POINT('Ctrl Pts',(-2.39615592726708,0.7739355201177,105.062783205835));
#33859=CARTESIAN_POINT('Ctrl Pts',(-2.37955915543172,0.823553119547407,
105.059488937794));
#33860=CARTESIAN_POINT('Ctrl Pts',(-2.36143112101026,0.872610629504506,
105.056194669753));
#33861=CARTESIAN_POINT('Ctrl Pts',(-2.36143106504627,0.872610780952441,
105.331623435588));
#33862=CARTESIAN_POINT('Ctrl Pts',(-2.39352196172693,0.785767434547548,
105.337991215488));
#33863=CARTESIAN_POINT('Ctrl Pts',(-2.42083637768937,0.697115782413577,
105.344302156859));
#33864=CARTESIAN_POINT('Ctrl Pts',(-2.4545969372037,0.561238145578153,105.353634028697));
#33865=CARTESIAN_POINT('Ctrl Pts',(-2.46468897516356,0.515114648938842,
105.356744922903));
#33866=CARTESIAN_POINT('Ctrl Pts',(-2.47992709244794,0.434703781335813,
105.362070098137));
#33867=CARTESIAN_POINT('Ctrl Pts',(-2.48567292855367,0.400544689760486,
105.36430198973));
#33868=CARTESIAN_POINT('Ctrl Pts',(-2.49297832660727,0.350867338513951,
105.367505577799));
#33869=CARTESIAN_POINT('Ctrl Pts',(-2.49510134151263,0.335437236340905,
105.368494773181));
#33870=CARTESIAN_POINT('Ctrl Pts',(-2.49857412633694,0.308336777931283,
105.370222144256));
#33871=CARTESIAN_POINT('Ctrl Pts',(-2.49998564241973,0.296674954585462,
105.370962229453));
#33872=CARTESIAN_POINT('Ctrl Pts',(-2.50274744007373,0.272436210589003,
105.372493933803));
#33873=CARTESIAN_POINT('Ctrl Pts',(-2.50408466476423,0.259858112501073,
105.373285125583));
#33874=CARTESIAN_POINT('Ctrl Pts',(-2.50730502910332,0.227229582499644,
105.375328395664));
#33875=CARTESIAN_POINT('Ctrl Pts',(-2.50904250889579,0.207165434328679,
105.376575919717));
#33876=CARTESIAN_POINT('Ctrl Pts',(-2.51521141134491,0.124382165587546,
105.381688661802));
#33877=CARTESIAN_POINT('Ctrl Pts',(-2.51753349719247,0.0615258153455552,
105.385488569262));
#33878=CARTESIAN_POINT('Ctrl Pts',(-2.51743889339061,-0.114151683195328,
105.395946872353));
#33879=CARTESIAN_POINT('Ctrl Pts',(-2.50979754438263,-0.22682169639588,
105.402462588056));
#33880=CARTESIAN_POINT('Ctrl Pts',(-2.47136408136718,-0.50997548796669,
105.418892328511));
#33881=CARTESIAN_POINT('Ctrl Pts',(-2.43050971079906,-0.678469643761034,
105.42871156683));
#33882=CARTESIAN_POINT('Ctrl Pts',(-2.36596485482824,-0.860479801024286,
105.440596079517));
#33883=CARTESIAN_POINT('Ctrl Pts',(-2.35897690821076,-0.879456121124482,
105.44185163018));
#33884=CARTESIAN_POINT('Ctrl Pts',(-2.34891331819353,-0.905801399600665,
105.443620530715));
#33885=CARTESIAN_POINT('Ctrl Pts',(-2.34602985661011,-0.913243592765757,
105.444123115966));
#33886=CARTESIAN_POINT('Ctrl Pts',(-2.34069627491772,-0.92681756567609,
105.445045308973));
#33887=CARTESIAN_POINT('Ctrl Pts',(-2.33825729966128,-0.932953723978231,
105.445464261891));
#33888=CARTESIAN_POINT('Ctrl Pts',(-2.33314425558839,-0.945671507567461,
105.446337019053));
#33889=CARTESIAN_POINT('Ctrl Pts',(-2.33046644529192,-0.952251469932218,
105.446791031924));
#33890=CARTESIAN_POINT('Ctrl Pts',(-2.32337172682301,-0.969475567765736,
105.447985786039));
#33891=CARTESIAN_POINT('Ctrl Pts',(-2.31890957668818,-0.980100719606244,
105.448729139318));
#33892=CARTESIAN_POINT('Ctrl Pts',(-2.29840204664799,-1.02800863051862,
105.452108377022));
#33893=CARTESIAN_POINT('Ctrl Pts',(-2.28153031238456,-1.06492849979142,
105.45478821802));
#33894=CARTESIAN_POINT('Ctrl Pts',(-2.23063600162743,-1.16953261093582,
105.462567809591));
#33895=CARTESIAN_POINT('Ctrl Pts',(-2.19444225908793,-1.2361088958505,105.467747986373));
#33896=CARTESIAN_POINT('Ctrl Pts',(-2.06528675333901,-1.45008331740098,
105.484960912937));
#33897=CARTESIAN_POINT('Ctrl Pts',(-1.96001973139913,-1.58949264202145,
105.497063780135));
#33898=CARTESIAN_POINT('Ctrl Pts',(-1.79300813828961,-1.7685925837549,105.513392617223));
#33899=CARTESIAN_POINT('Ctrl Pts',(-1.742666851341,-1.81821664089991,105.518023378132));
#33900=CARTESIAN_POINT('Ctrl Pts',(-1.67474239029629,-1.87975660669075,
105.52391209139));
#33901=CARTESIAN_POINT('Ctrl Pts',(-1.65900856701762,-1.89365720034632,
105.525252732417));
#33902=CARTESIAN_POINT('Ctrl Pts',(-1.63337802386371,-1.91573672964483,
105.527399883355));
#33903=CARTESIAN_POINT('Ctrl Pts',(-1.62358967771431,-1.92403938485612,
105.528211451082));
#33904=CARTESIAN_POINT('Ctrl Pts',(-1.60476639536951,-1.93975970146391,
105.529756300674));
#33905=CARTESIAN_POINT('Ctrl Pts',(-1.59574248203678,-1.94718998085793,
105.530490081863));
#33906=CARTESIAN_POINT('Ctrl Pts',(-1.57489279768188,-1.96411530074756,
105.532170095239));
#33907=CARTESIAN_POINT('Ctrl Pts',(-1.56303225094643,-1.97356693253041,
105.53311458007));
#33908=CARTESIAN_POINT('Ctrl Pts',(-1.5255834322984,-2.00286041539864,105.536062537394));
#33909=CARTESIAN_POINT('Ctrl Pts',(-1.49969671931488,-2.02231662922032,
105.538050932682));
#33910=CARTESIAN_POINT('Ctrl Pts',(-1.36602901649228,-2.11880145803573,
105.548084030797));
#33911=CARTESIAN_POINT('Ctrl Pts',(-1.25265952444321,-2.18773965820178,
105.555820311298));
#33912=CARTESIAN_POINT('Ctrl Pts',(-1.00701172452887,-2.31172858399199,
105.571688766981));
#33913=CARTESIAN_POINT('Ctrl Pts',(-0.874418169902418,-2.36506863001192,
105.579778102985));
#33914=CARTESIAN_POINT('Ctrl Pts',(-0.678075839251542,-2.42527358735326,
105.591935241963));
#33915=CARTESIAN_POINT('Ctrl Pts',(-0.61746012150452,-2.4414095161025,105.595714113065));
#33916=CARTESIAN_POINT('Ctrl Pts',(-0.543046757652888,-2.45827000997418,
105.600453557576));
#33917=CARTESIAN_POINT('Ctrl Pts',(-0.529758707412121,-2.46116779511449,
105.601303740268));
#33918=CARTESIAN_POINT('Ctrl Pts',(-0.508968740001284,-2.4655253945856,
105.602640841554));
#33919=CARTESIAN_POINT('Ctrl Pts',(-0.501482321399643,-2.46705900361328,
105.603123728906));
#33920=CARTESIAN_POINT('Ctrl Pts',(-0.48759206646943,-2.46983861581964,
105.60402246342));
#33921=CARTESIAN_POINT('Ctrl Pts',(-0.48119025622526,-2.47109383583127,
105.604437788788));
#33922=CARTESIAN_POINT('Ctrl Pts',(-0.466504900406724,-2.47391400282253,
105.605393036766));
#33923=CARTESIAN_POINT('Ctrl Pts',(-0.458218349779135,-2.47546223047425,
105.605933872992));
#33924=CARTESIAN_POINT('Ctrl Pts',(-0.432337658382364,-2.48016327985293,
105.607628350653));
#33925=CARTESIAN_POINT('Ctrl Pts',(-0.41471805298476,-2.48317027996274,
105.608789622871));
#33926=CARTESIAN_POINT('Ctrl Pts',(-0.37320472754113,-2.48980089371614,
105.611541353253));
#33927=CARTESIAN_POINT('Ctrl Pts',(-0.349288192518539,-2.493268522841,105.61313882741));
#33928=CARTESIAN_POINT('Ctrl Pts',(-0.262901163276538,-2.50452636639286,
105.618944134036));
#33929=CARTESIAN_POINT('Ctrl Pts',(-0.200196549302332,-2.51031664788374,
105.623223602155));
#33930=CARTESIAN_POINT('Ctrl Pts',(0.0731473964442369,-2.52525149692107,
105.641999497277));
#33931=CARTESIAN_POINT('Ctrl Pts',(0.284293349342089,-2.51026864132188,
105.656720343178));
#33932=CARTESIAN_POINT('Ctrl Pts',(0.54598044546324,-2.45821917704242,105.674356487106));
#33933=CARTESIAN_POINT('Ctrl Pts',(0.600475436914682,-2.44547873122814,
105.678001354921));
#33934=CARTESIAN_POINT('Ctrl Pts',(0.673136360955237,-2.42591549906605,
105.682826434895));
#33935=CARTESIAN_POINT('Ctrl Pts',(0.691710543507755,-2.42068484667083,
105.68405681457));
#33936=CARTESIAN_POINT('Ctrl Pts',(0.722183342883347,-2.4117240480384,105.686070783091));
#33937=CARTESIAN_POINT('Ctrl Pts',(0.734117383096413,-2.40811821585418,
105.686858345729));
#33938=CARTESIAN_POINT('Ctrl Pts',(0.757316978604474,-2.40092004126222,
105.688387258258));
#33939=CARTESIAN_POINT('Ctrl Pts',(0.768584961307669,-2.39733669214709,
105.689128876702));
#33940=CARTESIAN_POINT('Ctrl Pts',(0.795095098629307,-2.38870003900381,
105.690871603665));
#33941=CARTESIAN_POINT('Ctrl Pts',(0.810315091568749,-2.38357998886868,
105.691870508782));
#33942=CARTESIAN_POINT('Ctrl Pts',(0.86084055752127,-2.36604318706098,105.695182005602));
#33943=CARTESIAN_POINT('Ctrl Pts',(0.895919053097665,-2.35298450937276,
105.697473566341));
#33944=CARTESIAN_POINT('Ctrl Pts',(1.06267081978998,-2.28663770236431,105.708351249084));
#33945=CARTESIAN_POINT('Ctrl Pts',(1.18997206271003,-2.2230505754236,105.716589461816));
#33946=CARTESIAN_POINT('Ctrl Pts',(1.4611171104913,-2.05761224115616,105.734861481182));
#33947=CARTESIAN_POINT('Ctrl Pts',(1.60099470020489,-1.95075122194353,105.744808463872));
#33948=CARTESIAN_POINT('Ctrl Pts',(1.74433326219988,-1.81537215380788,105.756912877276));
#33949=CARTESIAN_POINT('Ctrl Pts',(1.75987354532094,-1.80031097834116,105.75825391033));
#33950=CARTESIAN_POINT('Ctrl Pts',(1.78121673688669,-1.77908537772112,105.760139445103));
#33951=CARTESIAN_POINT('Ctrl Pts',(1.78718612260268,-1.77308871840858,105.760671672328));
#33952=CARTESIAN_POINT('Ctrl Pts',(1.79742175495483,-1.762702117921,105.761592957279));
#33953=CARTESIAN_POINT('Ctrl Pts',(1.80170247390046,-1.75832645300342,105.7619809047));
#33954=CARTESIAN_POINT('Ctrl Pts',(1.81068758573955,-1.74907479079575,105.762800913492));
#33955=CARTESIAN_POINT('Ctrl Pts',(1.81538830113156,-1.74419536450768,105.763233259183));
#33956=CARTESIAN_POINT('Ctrl Pts',(1.82698263233916,-1.73206259852588,105.764307824333));
#33957=CARTESIAN_POINT('Ctrl Pts',(1.83385275588654,-1.72478707259447,105.764951785019));
#33958=CARTESIAN_POINT('Ctrl Pts',(1.85946764254119,-1.69733462036419,105.767379416451));
#33959=CARTESIAN_POINT('Ctrl Pts',(1.87792351697907,-1.67689231744877,105.769182709327));
#33960=CARTESIAN_POINT('Ctrl Pts',(2.01978754316611,-1.51447985755666,105.783447587917));
#33961=CARTESIAN_POINT('Ctrl Pts',(2.12726146304627,-1.35939157789997,105.796653099726));
#33962=CARTESIAN_POINT('Ctrl Pts',(2.28378925633807,-1.06877275823182,105.819290044746));
#33963=CARTESIAN_POINT('Ctrl Pts',(2.34043375793168,-0.938269778745885,
105.828824043614));
#33964=CARTESIAN_POINT('Ctrl Pts',(2.39287916441563,-0.782579484474979,
105.83942010666));
#33965=CARTESIAN_POINT('Ctrl Pts',(2.39970261433892,-0.761399211744634,
105.840846142309));
#33966=CARTESIAN_POINT('Ctrl Pts',(2.41047568794179,-0.72637478974724,105.843179494826));
#33967=CARTESIAN_POINT('Ctrl Pts',(2.41458886372809,-0.712582634159106,
105.844092070889));
#33968=CARTESIAN_POINT('Ctrl Pts',(2.42180562879597,-0.68760344755235,105.845733792333));
#33969=CARTESIAN_POINT('Ctrl Pts',(2.4249505146959,-0.676428867885624,105.846464253785));
#33970=CARTESIAN_POINT('Ctrl Pts',(2.43153201033684,-0.652407216277687,
105.848026174135));
#33971=CARTESIAN_POINT('Ctrl Pts',(2.4349443561787,-0.639553818089912,105.848856833913));
#33972=CARTESIAN_POINT('Ctrl Pts',(2.44401077611605,-0.604278301621236,
105.85112302857));
#33973=CARTESIAN_POINT('Ctrl Pts',(2.44945811710471,-0.58180402789837,105.852551943408));
#33974=CARTESIAN_POINT('Ctrl Pts',(2.47971691079009,-0.448997376902675,
105.860913634063));
#33975=CARTESIAN_POINT('Ctrl Pts',(2.49738270605797,-0.33716284815677,105.867614316008));
#33976=CARTESIAN_POINT('Ctrl Pts',(2.52302803343273,-0.050736749581071,
105.884345417257));
#33977=CARTESIAN_POINT('Ctrl Pts',(2.52048013210104,0.124167879640361,105.894146345345));
#33978=CARTESIAN_POINT('Ctrl Pts',(2.49215911842413,0.362233327032045,105.908315257117));
#33979=CARTESIAN_POINT('Ctrl Pts',(2.48192636097651,0.426743534254404,105.912244249825));
#33980=CARTESIAN_POINT('Ctrl Pts',(2.46651932795349,0.504259472625395,105.917152249462));
#33981=CARTESIAN_POINT('Ctrl Pts',(2.46372922549626,0.517719513436078,105.918011390141));
#33982=CARTESIAN_POINT('Ctrl Pts',(2.45920981896702,0.538657795058667,105.91935959002));
#33983=CARTESIAN_POINT('Ctrl Pts',(2.45755625753106,0.546152351681175,105.919844509758));
#33984=CARTESIAN_POINT('Ctrl Pts',(2.45443459094082,0.559999643923158,105.920745019647));
#33985=CARTESIAN_POINT('Ctrl Pts',(2.45297605102233,0.566354352231889,105.921160069608));
#33986=CARTESIAN_POINT('Ctrl Pts',(2.4495855564149,0.580867579425493,105.922112062175));
#33987=CARTESIAN_POINT('Ctrl Pts',(2.44763752804677,0.58902212989969,105.922649894333));
#33988=CARTESIAN_POINT('Ctrl Pts',(2.44146596947612,0.614297260154735,105.924325709525));
#33989=CARTESIAN_POINT('Ctrl Pts',(2.43710336671447,0.631382881225102,105.925471091796));
#33990=CARTESIAN_POINT('Ctrl Pts',(2.40674080226692,0.74528858406175,105.933184858485));
#33991=CARTESIAN_POINT('Ctrl Pts',(2.37515929513042,0.840517973094675,105.940007705263));
#33992=CARTESIAN_POINT('Ctrl Pts',(2.32177709389228,0.974201565986207,105.949910775536));
#33993=CARTESIAN_POINT('Ctrl Pts',(2.30450959601247,1.01437321334719,105.952931225032));
#33994=CARTESIAN_POINT('Ctrl Pts',(2.2076733664515,1.22440342367536,105.968909392239));
#33995=CARTESIAN_POINT('Ctrl Pts',(2.11033867889845,1.38545309421955,105.981754034073));
#33996=CARTESIAN_POINT('Ctrl Pts',(1.97624426696516,1.55990875298976,105.996044919658));
#33997=CARTESIAN_POINT('Ctrl Pts',(1.95599730945183,1.5852228252493,105.99813091688));
#33998=CARTESIAN_POINT('Ctrl Pts',(1.92566725984355,1.62167725173096,106.001154582924));
#33999=CARTESIAN_POINT('Ctrl Pts',(1.91596500831242,1.63312877852177,106.002107351422));
#34000=CARTESIAN_POINT('Ctrl Pts',(1.89851668046733,1.65335344140096,106.003795565375));
#34001=CARTESIAN_POINT('Ctrl Pts',(1.89081081908427,1.66216053439715,106.004532620561));
#34002=CARTESIAN_POINT('Ctrl Pts',(1.87455659397339,1.68047830663406,106.006069786151));
#34003=CARTESIAN_POINT('Ctrl Pts',(1.86599659409139,1.68997824942282,106.00686938458));
#34004=CARTESIAN_POINT('Ctrl Pts',(1.8433407587136,1.71473982930815,106.008960191329));
#34005=CARTESIAN_POINT('Ctrl Pts',(1.82912756565793,1.72989312487497,106.010246430901));
#34006=CARTESIAN_POINT('Ctrl Pts',(1.76167297888014,1.80004837774472,106.016236194987));
#34007=CARTESIAN_POINT('Ctrl Pts',(1.70612562779904,1.85278246456659,106.020839096882));
#34008=CARTESIAN_POINT('Ctrl Pts',(1.54642075545973,1.99111536460875,106.033329483093));
#34009=CARTESIAN_POINT('Ctrl Pts',(1.43766720439114,2.07100769537146,106.041024783751));
#34010=CARTESIAN_POINT('Ctrl Pts',(1.20941287214989,2.21200449930339,106.056457087221));
#34011=CARTESIAN_POINT('Ctrl Pts',(1.09039575888854,2.27303138479676,106.064173169772));
#34012=CARTESIAN_POINT('Ctrl Pts',(0.947312211208525,2.33256640444476,106.073689800145));
#34013=CARTESIAN_POINT('Ctrl Pts',(0.927402113636948,2.340553717791,106.075019374245));
#34014=CARTESIAN_POINT('Ctrl Pts',(0.899530277256461,2.35132358175623,106.076891250466));
#34015=CARTESIAN_POINT('Ctrl Pts',(0.891652326545413,2.35432228669465,106.077421506985));
#34016=CARTESIAN_POINT('Ctrl Pts',(0.878035388899877,2.35942736228369,106.078340310896));
#34017=CARTESIAN_POINT('Ctrl Pts',(0.872303456056896,2.36155251914801,106.078727761924));
#34018=CARTESIAN_POINT('Ctrl Pts',(0.860194062657157,2.36599206534157,106.079547862615));
#34019=CARTESIAN_POINT('Ctrl Pts',(0.853814919065881,2.36830157692148,106.079980803691));
#34020=CARTESIAN_POINT('Ctrl Pts',(0.837962599137786,2.37396839620913,106.081058810891));
#34021=CARTESIAN_POINT('Ctrl Pts',(0.828478578015414,2.37729478639092,106.081705641863));
#34022=CARTESIAN_POINT('Ctrl Pts',(0.792633749318139,2.38962632581186,106.084156768804));
#34023=CARTESIAN_POINT('Ctrl Pts',(0.766145082158192,2.3982501534697,106.085981166771));
#34024=CARTESIAN_POINT('Ctrl Pts',(0.697750561326767,2.41926845721426,106.090715671808));
#34025=CARTESIAN_POINT('Ctrl Pts',(0.655656143056743,2.43101425473521,106.093652253629));
#34026=CARTESIAN_POINT('Ctrl Pts',(0.492902173102709,2.47189374712834,106.105041670535));
#34027=CARTESIAN_POINT('Ctrl Pts',(0.370456339809665,2.4931851583422,106.113674704845));
#34028=CARTESIAN_POINT('Ctrl Pts',(0.0859199573453927,2.52123068446959,
106.13336083853));
#34029=CARTESIAN_POINT('Ctrl Pts',(-0.0762816828006424,2.52154407170327,
106.144290082977));
#34030=CARTESIAN_POINT('Ctrl Pts',(-0.259550307404212,2.50418334522028,
106.156163154833));
#34031=CARTESIAN_POINT('Ctrl Pts',(-0.28165675068904,2.50179337978175,106.15758808061));
#34032=CARTESIAN_POINT('Ctrl Pts',(-0.318010893627006,2.49737508202679,
106.159919999951));
#34033=CARTESIAN_POINT('Ctrl Pts',(-0.33227765635651,2.49551694081023,106.16083224162));
#34034=CARTESIAN_POINT('Ctrl Pts',(-0.358025473566206,2.49193875452469,
106.16247360306));
#34035=CARTESIAN_POINT('Ctrl Pts',(-0.369511958688839,2.4902614151307,106.163204036326));
#34036=CARTESIAN_POINT('Ctrl Pts',(-0.394135342293437,2.48649160949141,
106.164766156918));
#34037=CARTESIAN_POINT('Ctrl Pts',(-0.407268129954352,2.48437434240983,
106.16559704313));
#34038=CARTESIAN_POINT('Ctrl Pts',(-0.443199399477272,2.47828893167073,
106.167864522431));
#34039=CARTESIAN_POINT('Ctrl Pts',(-0.465961272990795,2.47411032160621,
106.169294482643));
#34040=CARTESIAN_POINT('Ctrl Pts',(-0.599957824267533,2.44759645053261,
106.177679618943));
#34041=CARTESIAN_POINT('Ctrl Pts',(-0.709644186108853,2.41807516523421,
106.184401078037));
#34042=CARTESIAN_POINT('Ctrl Pts',(-0.974362659558696,2.3272537335617,106.200681700565));
#34043=CARTESIAN_POINT('Ctrl Pts',(-1.12599858094617,2.25778976432643,106.210048264149));
#34044=CARTESIAN_POINT('Ctrl Pts',(-1.33207323811583,2.1374307820088,106.224093335637));
#34045=CARTESIAN_POINT('Ctrl Pts',(-1.39287605639833,2.09831449564818,106.228424762657));
#34046=CARTESIAN_POINT('Ctrl Pts',(-1.46244223111181,2.04920357798446,106.233709590173));
#34047=CARTESIAN_POINT('Ctrl Pts',(-1.47292073709227,2.04168486046258,106.234514799906));
#34048=CARTESIAN_POINT('Ctrl Pts',(-1.4899358914265,2.02927669776175,106.23583819953));
#34049=CARTESIAN_POINT('Ctrl Pts',(-1.4965074894668,2.02443528081114,106.236353242984));
#34050=CARTESIAN_POINT('Ctrl Pts',(-1.50810604285753,2.01580307900998,106.237269464396));
#34051=CARTESIAN_POINT('Ctrl Pts',(-1.51314246973389,2.01202528674545,106.23766975048));
#34052=CARTESIAN_POINT('Ctrl Pts',(-1.5182151886982,2.00819045282177,106.238075406396));
#34053=CARTESIAN_POINT('Ctrl Pts',(-1.51826562863857,2.00815231864845,106.238079440231));
#34054=CARTESIAN_POINT('Ctrl Pts',(-1.51836532222937,2.008076941271,106.238087413521));
#34055=CARTESIAN_POINT('Ctrl Pts',(-1.51841457594033,2.00803969815961,106.238091352968));
#34056=CARTESIAN_POINT('Ctrl Pts',(-1.5185119423902,2.00796606905025,106.23809914107));
#34057=CARTESIAN_POINT('Ctrl Pts',(-1.51856005518335,2.0079296831414,106.238102989719));
#34058=CARTESIAN_POINT('Ctrl Pts',(-1.51865518282569,2.00785773628304,106.238110599635));
#34059=CARTESIAN_POINT('Ctrl Pts',(-1.5187021977253,2.00782217541776,106.238114360896));
#34060=CARTESIAN_POINT('Ctrl Pts',(-1.51879517046939,2.00775184808275,106.238121799278));
#34061=CARTESIAN_POINT('Ctrl Pts',(-1.51884112836308,2.00771708169094,106.238125476392));
#34062=CARTESIAN_POINT('Ctrl Pts',(-1.51893202591893,2.00764831427555,106.238132749558));
#34063=CARTESIAN_POINT('Ctrl Pts',(-1.51897696565627,2.00761431330356,106.238136345607));
#34064=CARTESIAN_POINT('Ctrl Pts',(-1.51906586390531,2.00754704905175,106.238143459576));
#34065=CARTESIAN_POINT('Ctrl Pts',(-1.51910982246958,2.00751378583442,106.238146977491));
#34066=CARTESIAN_POINT('Ctrl Pts',(-1.51919679355273,2.00744797077504,106.238153937985));
#34067=CARTESIAN_POINT('Ctrl Pts',(-1.51923980612523,2.00741541898887,106.238157380559));
#34068=CARTESIAN_POINT('Ctrl Pts',(-1.51932491883692,2.00735100164097,106.238164193035));
#34069=CARTESIAN_POINT('Ctrl Pts',(-1.51936701897824,2.00731913616869,106.238167562929));
#34070=CARTESIAN_POINT('Ctrl Pts',(-1.51945033873661,2.00725606756734,106.238174232578));
#34071=CARTESIAN_POINT('Ctrl Pts',(-1.51949155840269,2.0072248644872,106.238177532329));
#34072=CARTESIAN_POINT('Ctrl Pts',(-1.51957314759574,2.00716309792448,106.238184064103));
#34073=CARTESIAN_POINT('Ctrl Pts',(-1.51961351722166,2.00713253444835,106.238187296126));
#34074=CARTESIAN_POINT('Ctrl Pts',(-1.51969343548718,2.00707202526417,106.238193694758));
#34075=CARTESIAN_POINT('Ctrl Pts',(-1.51973298416023,2.00704207960777,106.238196861363));
#34076=CARTESIAN_POINT('Ctrl Pts',(-1.51981128834638,2.0069827852222,106.238203131366));
#34077=CARTESIAN_POINT('Ctrl Pts',(-1.5198500438576,2.00695343656732,106.238206234758));
#34078=CARTESIAN_POINT('Ctrl Pts',(-1.51992678814661,2.00689531638929,106.238212380436));
#34079=CARTESIAN_POINT('Ctrl Pts',(-1.51996477697941,2.00686654489353,106.238215422719));
#34080=CARTESIAN_POINT('Ctrl Pts',(-1.52004001333529,2.00680955998396,106.238221448197));
#34081=CARTESIAN_POINT('Ctrl Pts',(-1.52007726086863,2.00678134662785,106.238224431387));
#34082=CARTESIAN_POINT('Ctrl Pts',(-1.52015103876086,2.00672545991089,106.238230340595));
#34083=CARTESIAN_POINT('Ctrl Pts',(-1.52018756919179,2.00669778655757,106.238233266613));
#34084=CARTESIAN_POINT('Ctrl Pts',(-1.52025993610152,2.00664296243901,106.238239063324));
#34085=CARTESIAN_POINT('Ctrl Pts',(-1.52029577260332,2.00661581171531,106.238241934012));
#34086=CARTESIAN_POINT('Ctrl Pts',(-1.5203667740048,2.00656201609837,106.238247621838));
#34087=CARTESIAN_POINT('Ctrl Pts',(-1.52040193884303,2.00653537130769,106.238250438965));
#34088=CARTESIAN_POINT('Ctrl Pts',(-1.520471617968,2.00648257177307,106.238256021341));
#34089=CARTESIAN_POINT('Ctrl Pts',(-1.52050613232808,2.0064564170268,106.238258786592));
#34090=CARTESIAN_POINT('Ctrl Pts',(-1.52057453095547,2.00640458223589,106.238264266839));
#34091=CARTESIAN_POINT('Ctrl Pts',(-1.52060841522901,2.00637890223714,106.238266981833));
#34092=CARTESIAN_POINT('Ctrl Pts',(-1.52067557317113,2.00632800232261,106.238272363117));
#34093=CARTESIAN_POINT('Ctrl Pts',(-1.52070884686618,2.00630278243493,106.238275029406));
#34094=CARTESIAN_POINT('Ctrl Pts',(-1.52077480241013,2.00625278866754,106.23828031477));
#34095=CARTESIAN_POINT('Ctrl Pts',(-1.52080748427373,2.00622801482255,106.238282933843));
#34096=CARTESIAN_POINT('Ctrl Pts',(-1.52087227396967,2.00617889977284,106.238288126193));
#34097=CARTESIAN_POINT('Ctrl Pts',(-1.52090438189069,2.00615455854456,106.238290699474));
#34098=CARTESIAN_POINT('Ctrl Pts',(-1.52096804114101,2.00610629563725,106.238295801626));
#34099=CARTESIAN_POINT('Ctrl Pts',(-1.5209995924226,2.00608237403602,106.23829833049));
#34100=CARTESIAN_POINT('Ctrl Pts',(-1.52106215488206,2.00603493800586,106.238303345121));
#34101=CARTESIAN_POINT('Ctrl Pts',(-1.52109316607101,2.00601142360822,106.238305830885));
#34102=CARTESIAN_POINT('Ctrl Pts',(-1.52115466419343,2.00596479008643,106.238310760576));
#34103=CARTESIAN_POINT('Ctrl Pts',(-1.52118515117764,2.0059416709617,106.238313204504));
#34104=CARTESIAN_POINT('Ctrl Pts',(-1.52124561616672,2.00589581651419,106.238318051737));
#34105=CARTESIAN_POINT('Ctrl Pts',(-1.52127559421915,2.00587308119152,106.238320455043));
#34106=CARTESIAN_POINT('Ctrl Pts',(-1.52133505606685,2.00582798329055,106.238325222206));
#34107=CARTESIAN_POINT('Ctrl Pts',(-1.52136453987596,2.00580562073632,106.238327586059));
#34108=CARTESIAN_POINT('Ctrl Pts',(-1.52142302745861,2.00576125768844,106.238332275448));
#34109=CARTESIAN_POINT('Ctrl Pts',(-1.52145203119468,2.00573925725624,106.238334600978));
#34110=CARTESIAN_POINT('Ctrl Pts',(-1.52150957216221,2.00569560828701,106.238339214794));
#34111=CARTESIAN_POINT('Ctrl Pts',(-1.52153810941493,2.00567395976542,106.23834150308));
#34112=CARTESIAN_POINT('Ctrl Pts',(-1.52159473045282,2.0056310048214,106.238346043448));
#34113=CARTESIAN_POINT('Ctrl Pts',(-1.52162281428758,2.00560969839154,106.238348295531));
#34114=CARTESIAN_POINT('Ctrl Pts',(-1.52167854116102,2.00556741810743,106.238352764501));
#34115=CARTESIAN_POINT('Ctrl Pts',(-1.52170618420044,2.0055464442815,106.238354981386));
#34116=CARTESIAN_POINT('Ctrl Pts',(-1.52176104161755,2.00550482008449,106.238359380926));
#34117=CARTESIAN_POINT('Ctrl Pts',(-1.52178825599615,2.00548416974038,106.238361563578));
#34118=CARTESIAN_POINT('Ctrl Pts',(-1.5218422678636,2.00544318365678,106.238365895591));
#34119=CARTESIAN_POINT('Ctrl Pts',(-1.52186906532566,2.0054228479641,106.238368044947));
#34120=CARTESIAN_POINT('Ctrl Pts',(-1.52849164415888,2.00039698644006,106.238899242306));
#34121=CARTESIAN_POINT('Ctrl Pts',(-1.53506258031548,1.99535903523944,106.239430527626));
#34122=CARTESIAN_POINT('Ctrl Pts',(-1.54896739544983,1.98458884964416,106.240563591107));
#34123=CARTESIAN_POINT('Ctrl Pts',(-1.55629455755438,1.97884818472817,106.241165919939));
#34124=CARTESIAN_POINT('Ctrl Pts',(-1.57587883034914,1.96332830474971,106.24278964481));
#34125=CARTESIAN_POINT('Ctrl Pts',(-1.58807648536065,1.9534751520086,106.243815600405));
#34126=CARTESIAN_POINT('Ctrl Pts',(-1.62588329083977,1.92234705799058,106.247039602589));
#34127=CARTESIAN_POINT('Ctrl Pts',(-1.65116209677604,1.90067835341579,106.249259302077));
#34128=CARTESIAN_POINT('Ctrl Pts',(-1.75509558929767,1.80794940734993,106.258632655889));
#34129=CARTESIAN_POINT('Ctrl Pts',(-1.82964894287989,1.7324618421866,106.265960816481));
#34130=CARTESIAN_POINT('Ctrl Pts',(-2.02028319468862,1.51336651497345,106.28602408217));
#34131=CARTESIAN_POINT('Ctrl Pts',(-2.12571178610571,1.36132099860141,106.298643650481));
#34132=CARTESIAN_POINT('Ctrl Pts',(-2.2291063244802,1.17044976988128,106.31274427953));
#34133=CARTESIAN_POINT('Ctrl Pts',(-2.24406707185061,1.14150374904687,106.314841325137));
#34134=CARTESIAN_POINT('Ctrl Pts',(-2.26510692023375,1.09878253947643,106.317877850261));
#34135=CARTESIAN_POINT('Ctrl Pts',(-2.27163060166272,1.08523124482096,106.318832612282));
#34136=CARTESIAN_POINT('Ctrl Pts',(-2.28301563303063,1.06102917464459,106.320523102128));
#34137=CARTESIAN_POINT('Ctrl Pts',(-2.28792481215159,1.05040151919514,106.321260454836));
#34138=CARTESIAN_POINT('Ctrl Pts',(-2.29803470469356,1.0281079094436,106.322796993301));
#34139=CARTESIAN_POINT('Ctrl Pts',(-2.30322113915874,1.01643581752206,106.323595676108));
#34140=CARTESIAN_POINT('Ctrl Pts',(-2.31658205675916,0.985739589933278,
106.325681314138));
#34141=CARTESIAN_POINT('Ctrl Pts',(-2.32461116787492,0.966652948400143,
106.326963346341));
#34142=CARTESIAN_POINT('Ctrl Pts',(-2.34247802360866,0.922669737893518,
106.329885333479));
#34143=CARTESIAN_POINT('Ctrl Pts',(-2.35215484568137,0.897713790146171,
106.331519808921));
#34144=CARTESIAN_POINT('Ctrl Pts',(-2.36143111532954,0.872610644877486,
106.333142274553));
#34145=CARTESIAN_POINT('Origin',(0.,0.,104.));
#34146=CARTESIAN_POINT('',(-2.36143111856514,0.872610636121403,107.329309102664));
#34147=CARTESIAN_POINT('',(-2.36143112101026,0.872610629504506,107.056339385048));
#34148=CARTESIAN_POINT('',(-2.36143112101026,0.872610629504505,104.));
#34149=CARTESIAN_POINT('',(-2.51749917428736,0.00203898565078566,106.11258330255));
#34150=CARTESIAN_POINT('Ctrl Pts',(-2.36143112101026,0.872610629504506,
107.056339385048));
#34151=CARTESIAN_POINT('Ctrl Pts',(-2.33100317881425,0.954953758525005,
107.050773684733));
#34152=CARTESIAN_POINT('Ctrl Pts',(-2.29630452944505,1.03559491387476,107.045207984417));
#34153=CARTESIAN_POINT('Ctrl Pts',(-2.25755960665741,1.11410541349948,107.039642284101));
#34154=CARTESIAN_POINT('Ctrl Pts',(-2.24919367653911,1.13105765668792,107.038440519933));
#34155=CARTESIAN_POINT('Ctrl Pts',(-2.2406392610389,1.14791066565236,107.037238755765));
#34156=CARTESIAN_POINT('Ctrl Pts',(-2.23189888544177,1.16466030032959,107.036036991597));
#34157=CARTESIAN_POINT('Ctrl Pts',(-2.19367769787657,1.23790554265723,107.03078174219));
#34158=CARTESIAN_POINT('Ctrl Pts',(-2.15177652201512,1.30940257330399,107.025526492782));
#34159=CARTESIAN_POINT('Ctrl Pts',(-2.10637922258263,1.37875770919774,107.020271243375));
#34160=CARTESIAN_POINT('Ctrl Pts',(-2.06104628620771,1.44801451526437,107.015023444718));
#34161=CARTESIAN_POINT('Ctrl Pts',(-2.01222732233027,1.51513507554309,107.00977564606));
#34162=CARTESIAN_POINT('Ctrl Pts',(-1.96015236693402,1.57974964738181,107.004527847403));
#34163=CARTESIAN_POINT('Ctrl Pts',(-1.90770008359203,1.64483240749782,106.99924202392));
#34164=CARTESIAN_POINT('Ctrl Pts',(-1.8519446439376,1.70737228971902,106.993956200437));
#34165=CARTESIAN_POINT('Ctrl Pts',(-1.79316602057087,1.76702062032961,106.988670376954));
#34166=CARTESIAN_POINT('Ctrl Pts',(-1.73491446106262,1.8261340884769,106.983431951085));
#34167=CARTESIAN_POINT('Ctrl Pts',(-1.67369404788836,1.88240731928923,106.978193525217));
#34168=CARTESIAN_POINT('Ctrl Pts',(-1.60981694875851,1.9355349755274,106.972955099348));
#34169=CARTESIAN_POINT('Ctrl Pts',(-1.54596085774349,1.9886451589636,106.967718396311));
#34170=CARTESIAN_POINT('Ctrl Pts',(-1.47945017054332,2.03861152763026,106.962481693273));
#34171=CARTESIAN_POINT('Ctrl Pts',(-1.41063142108424,2.08516791742293,106.957244990236));
#34172=CARTESIAN_POINT('Ctrl Pts',(-1.34181454621347,2.13172303904282,106.952008429843));
#34173=CARTESIAN_POINT('Ctrl Pts',(-1.27069011684476,2.17486810877624,106.946771869451));
#34174=CARTESIAN_POINT('Ctrl Pts',(-1.19763387775233,2.21438012655007,106.941535309059));
#34175=CARTESIAN_POINT('Ctrl Pts',(-1.12338190495366,2.25453884954772,106.936213040288));
#34176=CARTESIAN_POINT('Ctrl Pts',(-1.04713474113545,2.29094427560626,106.930890771518));
#34177=CARTESIAN_POINT('Ctrl Pts',(-0.969311467327336,2.32341161426634,
106.925568502747));
#34178=CARTESIAN_POINT('Ctrl Pts',(-0.892631474319646,2.3554019839798,106.920324421997));
#34179=CARTESIAN_POINT('Ctrl Pts',(-0.814421833478372,2.38356910416829,
106.915080341247));
#34180=CARTESIAN_POINT('Ctrl Pts',(-0.7351004171564,2.40778604254956,106.909836260496));
#34181=CARTESIAN_POINT('Ctrl Pts',(-0.654005005126036,2.43254458428023,
106.904474897716));
#34182=CARTESIAN_POINT('Ctrl Pts',(-0.571747985255809,2.45317399867903,
106.899113534935));
#34183=CARTESIAN_POINT('Ctrl Pts',(-0.48878675866748,2.46959384404629,106.893752172155));
#34184=CARTESIAN_POINT('Ctrl Pts',(-0.405825532079157,2.48601368941355,
106.888390809374));
#34185=CARTESIAN_POINT('Ctrl Pts',(-0.322160611199794,2.49822395846987,
106.883029446594));
#34186=CARTESIAN_POINT('Ctrl Pts',(-0.23825275748405,2.50620068501133,106.877668083813));
#34187=CARTESIAN_POINT('Ctrl Pts',(-0.156005628058678,2.51401953427505,
106.872412834406));
#34188=CARTESIAN_POINT('Ctrl Pts',(-0.0732213097316059,2.51779982116764,
106.867157584998));
#34189=CARTESIAN_POINT('Ctrl Pts',(0.00966987373682366,2.51748142863893,
106.861902335591));
#34190=CARTESIAN_POINT('Ctrl Pts',(0.0924435363376794,2.5171634875185,106.856654536934));
#34191=CARTESIAN_POINT('Ctrl Pts',(0.175323305567954,2.51275841106903,106.851406738276));
#34192=CARTESIAN_POINT('Ctrl Pts',(0.257873800693145,2.50425784473486,106.846158939619));
#34193=CARTESIAN_POINT('Ctrl Pts',(0.341022445322474,2.49569568446924,106.840873116136));
#34194=CARTESIAN_POINT('Ctrl Pts',(0.423836552202129,2.48297838833264,106.835587292653));
#34195=CARTESIAN_POINT('Ctrl Pts',(0.505871224990067,2.46615095923324,106.83030146917));
#34196=CARTESIAN_POINT('Ctrl Pts',(0.587170298529627,2.44947442052906,106.825063043301));
#34197=CARTESIAN_POINT('Ctrl Pts',(0.667703399917501,2.42876125862325,106.819824617433));
#34198=CARTESIAN_POINT('Ctrl Pts',(0.747044454435803,2.40410707604647,106.814586191564));
#34199=CARTESIAN_POINT('Ctrl Pts',(0.826359415001698,2.37946100182003,106.809349488527));
#34200=CARTESIAN_POINT('Ctrl Pts',(0.904482667029798,2.35087661793432,106.804112785489));
#34201=CARTESIAN_POINT('Ctrl Pts',(0.981002283185595,2.31849968091105,106.798876082452));
#34202=CARTESIAN_POINT('Ctrl Pts',(1.0575198149853,2.28612362581937,106.793639522059));
#34203=CARTESIAN_POINT('Ctrl Pts',(1.13243337321914,2.24995540374435,106.788402961667));
#34204=CARTESIAN_POINT('Ctrl Pts',(1.20535133231732,2.21018877376591,106.783166401275));
#34205=CARTESIAN_POINT('Ctrl Pts',(1.27946276185102,2.16977127124816,106.777844132504));
#34206=CARTESIAN_POINT('Ctrl Pts',(1.35151223973336,2.1256367295182,106.772521863734));
#34207=CARTESIAN_POINT('Ctrl Pts',(1.42111659583186,2.07803606105651,106.767199594963));
#34208=CARTESIAN_POINT('Ctrl Pts',(1.48969841304111,2.0311346812225,106.761955514213));
#34209=CARTESIAN_POINT('Ctrl Pts',(1.55590613719532,1.98086867041453,106.756711433463));
#34210=CARTESIAN_POINT('Ctrl Pts',(1.61940578722056,1.92751942825917,106.751467352712));
#34211=CARTESIAN_POINT('Ctrl Pts',(1.6843255846897,1.87297704897863,106.746105989932));
#34212=CARTESIAN_POINT('Ctrl Pts',(1.74641434121004,1.81521221218204,106.740744627151));
#34213=CARTESIAN_POINT('Ctrl Pts',(1.80535555014975,1.75456478579261,106.735383264371));
#34214=CARTESIAN_POINT('Ctrl Pts',(1.86429675908946,1.69391735940319,106.73002190159));
#34215=CARTESIAN_POINT('Ctrl Pts',(1.9200901353509,1.6303877692775,106.72466053881));
#34216=CARTESIAN_POINT('Ctrl Pts',(1.97246471397388,1.56434945013189,106.719299176029));
#34217=CARTESIAN_POINT('Ctrl Pts',(2.02380268242187,1.49961817717862,106.714043926622));
#34218=CARTESIAN_POINT('Ctrl Pts',(2.07204560924584,1.43223751273161,106.708788677214));
#34219=CARTESIAN_POINT('Ctrl Pts',(2.11690877828482,1.36253567821935,106.703533427807));
#34220=CARTESIAN_POINT('Ctrl Pts',(2.16170834154179,1.29293266507408,106.69828562915));
#34221=CARTESIAN_POINT('Ctrl Pts',(2.20313741713628,1.22101540329658,106.693037830492));
#34222=CARTESIAN_POINT('Ctrl Pts',(2.24095195361092,1.14714453823719,106.687790031835));
#34223=CARTESIAN_POINT('Ctrl Pts',(2.27904048900231,1.07273841507621,106.682504208352));
#34224=CARTESIAN_POINT('Ctrl Pts',(2.3134615888812,0.996350629387463,106.677218384869));
#34225=CARTESIAN_POINT('Ctrl Pts',(2.34401077683186,0.918378858693995,106.671932561386));
#34226=CARTESIAN_POINT('Ctrl Pts',(2.37428603232284,0.841106255486301,106.666694135517));
#34227=CARTESIAN_POINT('Ctrl Pts',(2.40075836468042,0.76227839800666,106.661455709649));
#34228=CARTESIAN_POINT('Ctrl Pts',(2.42327598752447,0.682304725388393,106.65621728378));
#34229=CARTESIAN_POINT('Ctrl Pts',(2.4457862046971,0.602357354780098,106.650980580743));
#34230=CARTESIAN_POINT('Ctrl Pts',(2.46434417053718,0.521265361257645,106.645743877705));
#34231=CARTESIAN_POINT('Ctrl Pts',(2.47884787001032,0.43945362365706,106.640507174668));
#34232=CARTESIAN_POINT('Ctrl Pts',(2.49335117440993,0.357644114567297,106.635270614275));
#34233=CARTESIAN_POINT('Ctrl Pts',(2.50380035248801,0.275115354896424,106.630034053883));
#34234=CARTESIAN_POINT('Ctrl Pts',(2.51014470671314,0.192301329584582,106.624797493491));
#34235=CARTESIAN_POINT('Ctrl Pts',(2.51659290091533,0.108131861908733,106.61947522472));
#34236=CARTESIAN_POINT('Ctrl Pts',(2.51880063850722,0.0236681955689467,
106.61415295595));
#34237=CARTESIAN_POINT('Ctrl Pts',(2.51676976536494,-0.0606316595920765,
106.608830687179));
#34238=CARTESIAN_POINT('Ctrl Pts',(2.5147687272342,-0.14369308823651,106.603586606429));
#34239=CARTESIAN_POINT('Ctrl Pts',(2.50865288393013,-0.226595024528162,
106.598342525679));
#34240=CARTESIAN_POINT('Ctrl Pts',(2.49847643477152,-0.308904119252864,
106.593098444928));
#34241=CARTESIAN_POINT('Ctrl Pts',(2.48807239288988,-0.393054028067697,
106.587737082148));
#34242=CARTESIAN_POINT('Ctrl Pts',(2.4734240138405,-0.476583753600645,106.582375719367));
#34243=CARTESIAN_POINT('Ctrl Pts',(2.45464405368558,-0.559042770909367,
106.577014356587));
#34244=CARTESIAN_POINT('Ctrl Pts',(2.43586409353066,-0.64150178821809,106.571652993806));
#34245=CARTESIAN_POINT('Ctrl Pts',(2.41295275425355,-0.722889626306614,
106.566291631026));
#34246=CARTESIAN_POINT('Ctrl Pts',(2.38607574271778,-0.802775684742503,
106.560930268245));
#34247=CARTESIAN_POINT('Ctrl Pts',(2.35973068741657,-0.88108061922109,106.555675018838));
#34248=CARTESIAN_POINT('Ctrl Pts',(2.3294782427263,-0.958231921997691,106.55041976943));
#34249=CARTESIAN_POINT('Ctrl Pts',(2.29543870409073,-1.03381207468392,106.545164520023));
#34250=CARTESIAN_POINT('Ctrl Pts',(2.26144742578811,-1.10928507188334,106.539916721366));
#34251=CARTESIAN_POINT('Ctrl Pts',(2.22367990631748,-1.18319092631463,106.534668922708));
#34252=CARTESIAN_POINT('Ctrl Pts',(2.18230577801946,-1.25512857557418,106.529421124051));
#34253=CARTESIAN_POINT('Ctrl Pts',(2.14063185849318,-1.32758747512024,106.524135300568));
#34254=CARTESIAN_POINT('Ctrl Pts',(2.09529899473699,-1.39804907730869,106.518849477085));
#34255=CARTESIAN_POINT('Ctrl Pts',(2.04652942808546,-1.46612535275133,106.513563653602));
#34256=CARTESIAN_POINT('Ctrl Pts',(1.99819717477175,-1.53359119293106,106.508325227733));
#34257=CARTESIAN_POINT('Ctrl Pts',(1.94648987873675,-1.59871393114153,106.503086801865));
#34258=CARTESIAN_POINT('Ctrl Pts',(1.89166833403513,-1.66114333036279,106.497848375996));
#34259=CARTESIAN_POINT('Ctrl Pts',(1.83686481922718,-1.72355219759363,106.492611672959));
#34260=CARTESIAN_POINT('Ctrl Pts',(1.77894939414177,-1.78326913863002,106.487374969921));
#34261=CARTESIAN_POINT('Ctrl Pts',(1.71822290162397,-1.83997725810264,106.482138266884));
#34262=CARTESIAN_POINT('Ctrl Pts',(1.65749806326547,-1.89668383287443,106.476901706491));
#34263=CARTESIAN_POINT('Ctrl Pts',(1.593962647664,-1.95038143486623,106.471665146099));
#34264=CARTESIAN_POINT('Ctrl Pts',(1.52795307568914,-2.00079125560167,106.466428585707));
#34265=CARTESIAN_POINT('Ctrl Pts',(1.46086310495394,-2.05202614921975,106.461106316936));
#34266=CARTESIAN_POINT('Ctrl Pts',(1.39121763942812,-2.09986435746929,106.455784048166));
#34267=CARTESIAN_POINT('Ctrl Pts',(1.31940185922442,-2.14405806448313,106.450461779395));
#34268=CARTESIAN_POINT('Ctrl Pts',(1.24864110534721,-2.18760253362428,106.445217698645));
#34269=CARTESIAN_POINT('Ctrl Pts',(1.17577382032506,-2.22760870007057,106.439973617895));
#34270=CARTESIAN_POINT('Ctrl Pts',(1.10119300303935,-2.26388608813632,106.434729537144));
#34271=CARTESIAN_POINT('Ctrl Pts',(1.02494421188303,-2.30097480728679,106.429368174364));
#34272=CARTESIAN_POINT('Ctrl Pts',(0.946904789682408,-2.3341657494093,106.424006811583));
#34273=CARTESIAN_POINT('Ctrl Pts',(0.867514023497477,-2.36330820441076,
106.418645448802));
#34274=CARTESIAN_POINT('Ctrl Pts',(0.788123257312551,-2.39245065941223,
106.413284086022));
#34275=CARTESIAN_POINT('Ctrl Pts',(0.707381652181258,-2.41754454028025,
106.407922723241));
#34276=CARTESIAN_POINT('Ctrl Pts',(0.625740611784842,-2.43849439957592,
106.402561360461));
#34277=CARTESIAN_POINT('Ctrl Pts',(0.545715430368026,-2.45902961425046,
106.397306111053));
#34278=CARTESIAN_POINT('Ctrl Pts',(0.464530522070312,-2.47565924426923,
106.392050861646));
#34279=CARTESIAN_POINT('Ctrl Pts',(0.382601593136953,-2.48825687398409,
106.386795612239));
#34280=CARTESIAN_POINT('Ctrl Pts',(0.30078882081284,-2.50083664312184,106.381547813581));
#34281=CARTESIAN_POINT('Ctrl Pts',(0.218234575353637,-2.5093956969744,106.376300014924));
#34282=CARTESIAN_POINT('Ctrl Pts',(0.135367621402023,-2.51385796278866,
106.371052216266));
#34283=CARTESIAN_POINT('Ctrl Pts',(0.0519002249292542,-2.51835256156568,
106.365766392783));
#34284=CARTESIAN_POINT('Ctrl Pts',(-0.0318839718264673,-2.51869063448652,
106.3604805693));
#34285=CARTESIAN_POINT('Ctrl Pts',(-0.115538493166347,-2.51484733266193,
106.355194745817));
#34286=CARTESIAN_POINT('Ctrl Pts',(-0.198442890187689,-2.51103849345953,
106.349956319949));
#34287=CARTESIAN_POINT('Ctrl Pts',(-0.281219458631995,-2.50312298893549,
106.34471789408));
#34288=CARTESIAN_POINT('Ctrl Pts',(-0.36343243265878,-2.49112888403866,
106.339479468212));
#34289=CARTESIAN_POINT('Ctrl Pts',(-0.445618368206609,-2.47913872380333,
106.334242765174));
#34290=CARTESIAN_POINT('Ctrl Pts',(-0.527240621238637,-2.46307269381631,
106.329006062136));
#34291=CARTESIAN_POINT('Ctrl Pts',(-0.607869588007225,-2.44301060455658,
106.323769359099));
#34292=CARTESIAN_POINT('Ctrl Pts',(-0.688496358483101,-2.42294906177813,
106.318532798707));
#34293=CARTESIAN_POINT('Ctrl Pts',(-0.768129448972136,-2.39889178856418,
106.313296238314));
#34294=CARTESIAN_POINT('Ctrl Pts',(-0.846351832207721,-2.3709691744345,
106.308059677922));
#34295=CARTESIAN_POINT('Ctrl Pts',(-0.925854505003531,-2.34258954237868,
106.302737409151));
#34296=CARTESIAN_POINT('Ctrl Pts',(-1.00389940744499,-2.31021705035641,
106.297415140381));
#34297=CARTESIAN_POINT('Ctrl Pts',(-1.08006896158092,-2.27403986073892,
106.29209287161));
#34298=CARTESIAN_POINT('Ctrl Pts',(-1.15511952926764,-2.23839414049147,
106.28684879086));
#34299=CARTESIAN_POINT('Ctrl Pts',(-1.2283491001215,-2.19905504374551,106.28160471011));
#34300=CARTESIAN_POINT('Ctrl Pts',(-1.2993839357524,-2.15624851014641,106.276360629359));
#34301=CARTESIAN_POINT('Ctrl Pts',(-1.37200744061546,-2.11248462340838,
106.270999266579));
#34302=CARTESIAN_POINT('Ctrl Pts',(-1.44233643204541,-2.06509661837732,
106.265637903798));
#34303=CARTESIAN_POINT('Ctrl Pts',(-1.51000532505333,-2.01437091130471,
106.260276541018));
#34304=CARTESIAN_POINT('Ctrl Pts',(-1.57767421806126,-1.9636452042321,106.254915178237));
#34305=CARTESIAN_POINT('Ctrl Pts',(-1.64268266469312,-1.90958217136583,
106.249553815457));
#34306=CARTESIAN_POINT('Ctrl Pts',(-1.70470483693462,-1.8525084801241,106.244192452676));
#34307=CARTESIAN_POINT('Ctrl Pts',(-1.76459909663839,-1.79739292447774,
106.239015032358));
#34308=CARTESIAN_POINT('Ctrl Pts',(-1.82194411214334,-1.73925298659691,
106.23383761204));
#34309=CARTESIAN_POINT('Ctrl Pts',(-1.87641220836556,-1.67835737383214,
106.228660191721));
#34310=CARTESIAN_POINT('Ctrl Pts',(-1.9307897580279,-1.61756299258873,106.223491378232));
#34311=CARTESIAN_POINT('Ctrl Pts',(-1.98229957592409,-1.55402238995337,
106.218322564743));
#34312=CARTESIAN_POINT('Ctrl Pts',(-2.0306488285422,-1.4880428707333,106.213153751254));
#34313=CARTESIAN_POINT('Ctrl Pts',(-2.07895290625897,-1.42212499917289,
106.207989767222));
#34314=CARTESIAN_POINT('Ctrl Pts',(-2.12410199614056,-1.35377311300338,
106.20282578319));
#34315=CARTESIAN_POINT('Ctrl Pts',(-2.16584248281613,-1.2833287145657,106.197661799158));
#34316=CARTESIAN_POINT('Ctrl Pts',(-2.2075574479352,-1.2129273882347,106.192500972562));
#34317=CARTESIAN_POINT('Ctrl Pts',(-2.24586770342721,-1.14043649738507,
106.187340145966));
#34318=CARTESIAN_POINT('Ctrl Pts',(-2.2805629687953,-1.06622642780958,106.18217931937));
#34319=CARTESIAN_POINT('Ctrl Pts',(-2.31524822027081,-0.992037777054693,
106.177019982313));
#34320=CARTESIAN_POINT('Ctrl Pts',(-2.34632035285064,-0.916131364617167,
106.171860645256));
#34321=CARTESIAN_POINT('Ctrl Pts',(-2.37361579836201,-0.83890064475256,
106.166701308199));
#34322=CARTESIAN_POINT('Ctrl Pts',(-2.40092462170781,-0.761632073159825,
106.161539442488));
#34323=CARTESIAN_POINT('Ctrl Pts',(-2.42445289854654,-0.68303834630904,
106.156377576776));
#34324=CARTESIAN_POINT('Ctrl Pts',(-2.44408620525115,-0.603530340000433,
106.151215711065));
#34325=CARTESIAN_POINT('Ctrl Pts',(-2.46372478256864,-0.524000989558178,
106.146052459637));
#34326=CARTESIAN_POINT('Ctrl Pts',(-2.47946621212706,-0.443557337996501,
106.140889208209));
#34327=CARTESIAN_POINT('Ctrl Pts',(-2.49124719851246,-0.36262052603765,
106.135725956781));
#34328=CARTESIAN_POINT('Ctrl Pts',(-2.50304227978819,-0.281586880464768,
106.130556527987));
#34329=CARTESIAN_POINT('Ctrl Pts',(-2.51086741194788,-0.200059370820398,
106.125387099194));
#34330=CARTESIAN_POINT('Ctrl Pts',(-2.51471124598382,-0.118463493627845,
106.1202176704));
#34331=CARTESIAN_POINT('Ctrl Pts',(-2.5166034758707,-0.0782957454818718,
106.117672881117));
#34332=CARTESIAN_POINT('Ctrl Pts',(-2.51753169311315,-0.0381114278951565,
106.115128091833));
#34333=CARTESIAN_POINT('Ctrl Pts',(-2.51749917428736,0.00203898565078367,
106.11258330255));
#34334=CARTESIAN_POINT('Ctrl Pts',(-2.51749917428662,0.00203898656446618,
106.112583302492));
#34335=CARTESIAN_POINT('Ctrl Pts',(-2.51739410665396,0.131764058349367,
106.104361146272));
#34336=CARTESIAN_POINT('Ctrl Pts',(-2.50725905023951,0.261092140164354,
106.096138990052));
#34337=CARTESIAN_POINT('Ctrl Pts',(-2.4872941057706,0.388811369945391,106.087916833832));
#34338=CARTESIAN_POINT('Ctrl Pts',(-2.48559980578692,0.399650102268016,
106.087219070852));
#34339=CARTESIAN_POINT('Ctrl Pts',(-2.48383473575133,0.410477266841117,
106.086521307872));
#34340=CARTESIAN_POINT('Ctrl Pts',(-2.48199903094348,0.421292131893801,
106.085823544892));
#34341=CARTESIAN_POINT('Ctrl Pts',(-2.46817693389102,0.502723587391459,
106.08056967859));
#34342=CARTESIAN_POINT('Ctrl Pts',(-2.45031756944332,0.58362443547189,106.075315812289));
#34343=CARTESIAN_POINT('Ctrl Pts',(-2.42847467758016,0.663563855519524,
106.070061945987));
#34344=CARTESIAN_POINT('Ctrl Pts',(-2.40920337579527,0.734091910957334,
106.065426623719));
#34345=CARTESIAN_POINT('Ctrl Pts',(-2.38683207102609,0.803871386774122,
106.060791301452));
#34346=CARTESIAN_POINT('Ctrl Pts',(-2.36143112101026,0.872610629504504,
106.056155979185));
#34347=CARTESIAN_POINT('',(-2.51749974387929,-0.00113559134422,106.385343084406));
#34348=CARTESIAN_POINT('Ctrl Pts',(-2.36143111532954,0.872610644877486,
106.333142274553));
#34349=CARTESIAN_POINT('Ctrl Pts',(-2.37840222838592,0.826683959627441,
106.336110606514));
#34350=CARTESIAN_POINT('Ctrl Pts',(-2.39403264494922,0.780264573325589,
106.339038531095));
#34351=CARTESIAN_POINT('Ctrl Pts',(-2.48082626973949,0.495260363424947,
106.356658330302));
#34352=CARTESIAN_POINT('Ctrl Pts',(-2.51761199924472,0.247724049190195,
106.370316362223));
#34353=CARTESIAN_POINT('Ctrl Pts',(-2.51749974387929,-0.00113559134422,
106.385343084406));
#34354=CARTESIAN_POINT('Ctrl Pts',(-2.51749974245381,-0.00113874712773204,
106.38534327496));
#34355=CARTESIAN_POINT('Ctrl Pts',(-2.5174886769077,-0.0256020443719995,
106.386820426755));
#34356=CARTESIAN_POINT('Ctrl Pts',(-2.51712103637506,-0.0500631483503205,
106.38831115182));
#34357=CARTESIAN_POINT('Ctrl Pts',(-2.51590148255077,-0.0912483122380716,
106.390849931066));
#34358=CARTESIAN_POINT('Ctrl Pts',(-2.51523906686123,-0.107976511726821,
106.391889134037));
#34359=CARTESIAN_POINT('Ctrl Pts',(-2.5140400509716,-0.132153782305922,
106.393404299523));
#34360=CARTESIAN_POINT('Ctrl Pts',(-2.51363704738602,-0.139609422307697,
106.393873354727));
#34361=CARTESIAN_POINT('Ctrl Pts',(-2.51284220378002,-0.153192723263485,
106.394731410201));
#34362=CARTESIAN_POINT('Ctrl Pts',(-2.51246109876711,-0.15932098678088,
106.395119828112));
#34363=CARTESIAN_POINT('Ctrl Pts',(-2.51164734611005,-0.17167651256996,
106.395905663239));
#34364=CARTESIAN_POINT('Ctrl Pts',(-2.51121395728993,-0.177903552065781,
106.396303126556));
#34365=CARTESIAN_POINT('Ctrl Pts',(-2.51014024441833,-0.192544560959587,
106.397240925798));
#34366=CARTESIAN_POINT('Ctrl Pts',(-2.50948077436851,-0.200956942598961,
106.397782301401));
#34367=CARTESIAN_POINT('Ctrl Pts',(-2.5076297546577,-0.223137268022371,
106.399216124558));
#34368=CARTESIAN_POINT('Ctrl Pts',(-2.50636712718199,-0.23689877699717,
106.400112249799));
#34369=CARTESIAN_POINT('Ctrl Pts',(-2.49983804137136,-0.302150641058131,
106.404390150203));
#34370=CARTESIAN_POINT('Ctrl Pts',(-2.49309808721478,-0.353477521822113,
106.407840193943));
#34371=CARTESIAN_POINT('Ctrl Pts',(-2.45039581229338,-0.615754713508913,
106.425791061583));
#34372=CARTESIAN_POINT('Ctrl Pts',(-2.38922456477507,-0.821714523814122,
106.440867787194));
#34373=CARTESIAN_POINT('Ctrl Pts',(-2.2673384725194,-1.09756545525668,106.461138692496));
#34374=CARTESIAN_POINT('Ctrl Pts',(-2.22779112997989,-1.17576500379407,
106.466909277117));
#34375=CARTESIAN_POINT('Ctrl Pts',(-2.17348812189932,-1.27052099109105,
106.473930898796));
#34376=CARTESIAN_POINT('Ctrl Pts',(-2.16249039112194,-1.28915071300985,
106.475313064241));
#34377=CARTESIAN_POINT('Ctrl Pts',(-2.14451449585696,-1.31872368623372,
106.47751037029));
#34378=CARTESIAN_POINT('Ctrl Pts',(-2.13768967215345,-1.32975842143583,
106.478331002013));
#34379=CARTESIAN_POINT('Ctrl Pts',(-2.12457174787982,-1.35060616654113,
106.479883008618));
#34380=CARTESIAN_POINT('Ctrl Pts',(-2.1182952230244,-1.36042915451066,106.480614963194));
#34381=CARTESIAN_POINT('Ctrl Pts',(-2.10384015801193,-1.38270925803018,
106.482276915269));
#34382=CARTESIAN_POINT('Ctrl Pts',(-2.09561873828371,-1.39513813707365,
106.483205298159));
#34383=CARTESIAN_POINT('Ctrl Pts',(-2.06996941460449,-1.43317561839316,
106.486051105667));
#34384=CARTESIAN_POINT('Ctrl Pts',(-2.05217846194298,-1.45853673915997,
106.487954939507));
#34385=CARTESIAN_POINT('Ctrl Pts',(-1.91340326130433,-1.64879353647585,
106.502304452549));
#34386=CARTESIAN_POINT('Ctrl Pts',(-1.77320115967382,-1.79872133068051,
106.513920857825));
#34387=CARTESIAN_POINT('Ctrl Pts',(-1.54528393003118,-1.98959975225619,
106.531045769329));
#34388=CARTESIAN_POINT('Ctrl Pts',(-1.4709417104943,-2.0451742212175,106.536423246696));
#34389=CARTESIAN_POINT('Ctrl Pts',(-1.36805384530418,-2.11357138570874,
106.543831345724));
#34390=CARTESIAN_POINT('Ctrl Pts',(-1.34208865201766,-2.13015332933239,
106.545698345049));
#34391=CARTESIAN_POINT('Ctrl Pts',(-1.30316267420755,-2.1540180966544,106.548503645364));
#34392=CARTESIAN_POINT('Ctrl Pts',(-1.29043027905398,-2.16166986104699,
106.549422228113));
#34393=CARTESIAN_POINT('Ctrl Pts',(-1.26989609879762,-2.17376418612735,
106.550906490124));
#34394=CARTESIAN_POINT('Ctrl Pts',(-1.26213676920833,-2.17827858845475,
106.551467991951));
#34395=CARTESIAN_POINT('Ctrl Pts',(-1.24734474990491,-2.18677906326363,
106.552539945485));
#34396=CARTESIAN_POINT('Ctrl Pts',(-1.24031666126126,-2.19077296225725,
106.553049911725));
#34397=CARTESIAN_POINT('Ctrl Pts',(-1.22769644399515,-2.19786454508185,
106.553967036993));
#34398=CARTESIAN_POINT('Ctrl Pts',(-1.22211160398293,-2.2009748619724,106.554373387341));
#34399=CARTESIAN_POINT('Ctrl Pts',(-1.20977891756267,-2.20778178638898,
106.555271844535));
#34400=CARTESIAN_POINT('Ctrl Pts',(-1.20302605189916,-2.21146868853847,
106.555764525401));
#34401=CARTESIAN_POINT('Ctrl Pts',(-1.18408705283165,-2.22169651118994,
106.557148083931));
#34402=CARTESIAN_POINT('Ctrl Pts',(-1.17186397637098,-2.22816793285224,
106.558043085935));
#34403=CARTESIAN_POINT('Ctrl Pts',(-1.10031765231315,-2.26529609607387,
106.56329115958));
#34404=CARTESIAN_POINT('Ctrl Pts',(-1.03985169351275,-2.29368091646447,
106.567762891552));
#34405=CARTESIAN_POINT('Ctrl Pts',(-0.774096630116817,-2.40576687398546,
106.587362643806));
#34406=CARTESIAN_POINT('Ctrl Pts',(-0.559332233676539,-2.46457119808922,
106.602955951201));
#34407=CARTESIAN_POINT('Ctrl Pts',(-0.293643990155972,-2.5007468333505,
106.620816114834));
#34408=CARTESIAN_POINT('Ctrl Pts',(-0.247476936706913,-2.50573684319135,
106.623874056116));
#34409=CARTESIAN_POINT('Ctrl Pts',(-0.167108753650601,-2.51218038975102,
106.62911825787));
#34410=CARTESIAN_POINT('Ctrl Pts',(-0.132968270019118,-2.51421862076372,
106.631321415561));
#34411=CARTESIAN_POINT('Ctrl Pts',(-0.0833105800665508,-2.51616886314197,
106.634491718405));
#34412=CARTESIAN_POINT('Ctrl Pts',(-0.0678201651223361,-2.51663403046701,
106.63547585784));
#34413=CARTESIAN_POINT('Ctrl Pts',(-0.0405936575150107,-2.51720005481548,
106.637197427096));
#34414=CARTESIAN_POINT('Ctrl Pts',(-0.0288594408697667,-2.51736193289732,
106.637936726786));
#34415=CARTESIAN_POINT('Ctrl Pts',(-0.00599425838749794,-2.51751746840598,
106.639372275662));
#34416=CARTESIAN_POINT('Ctrl Pts',(0.00513636111921546,-2.51751936616252,
106.640068763188));
#34417=CARTESIAN_POINT('Ctrl Pts',(0.0350926329951424,-2.5173258003219,
106.641937198091));
#34418=CARTESIAN_POINT('Ctrl Pts',(0.0539169212550774,-2.51699298239075,
106.643104873476));
#34419=CARTESIAN_POINT('Ctrl Pts',(0.125040839673735,-2.51493719775465,
106.647494107486));
#34420=CARTESIAN_POINT('Ctrl Pts',(0.177288196806846,-2.51179493474101,
106.650671867291));
#34421=CARTESIAN_POINT('Ctrl Pts',(0.419181729845457,-2.48966074300661,
106.665228510676));
#34422=CARTESIAN_POINT('Ctrl Pts',(0.606371057255961,-2.45080421165191,
106.675992382609));
#34423=CARTESIAN_POINT('Ctrl Pts',(0.898128086010245,-2.35473242022073,
106.693750428235));
#34424=CARTESIAN_POINT('Ctrl Pts',(1.00618565585988,-2.31062377853236,106.700580180374));
#34425=CARTESIAN_POINT('Ctrl Pts',(1.12422216626366,-2.25258851585288,106.708734677337));
#34426=CARTESIAN_POINT('Ctrl Pts',(1.13760108703273,-2.24586158130117,106.709669493805));
#34427=CARTESIAN_POINT('Ctrl Pts',(1.15790223958993,-2.23542620265445,106.711105325391));
#34428=CARTESIAN_POINT('Ctrl Pts',(1.16486871567246,-2.23180392849727,106.711601183228));
#34429=CARTESIAN_POINT('Ctrl Pts',(1.17757722062226,-2.22512032973606,106.71251171493));
#34430=CARTESIAN_POINT('Ctrl Pts',(1.18332444369557,-2.22206927222134,106.712925751572));
#34431=CARTESIAN_POINT('Ctrl Pts',(1.19625390988776,-2.21514095472807,106.713862315884));
#34432=CARTESIAN_POINT('Ctrl Pts',(1.20342911054679,-2.2112510571332,106.714385615959));
#34433=CARTESIAN_POINT('Ctrl Pts',(1.22189132611882,-2.20112564752323,106.715741042883));
#34434=CARTESIAN_POINT('Ctrl Pts',(1.23314941870801,-2.19483826824055,106.716576247476));
#34435=CARTESIAN_POINT('Ctrl Pts',(1.30711216556026,-2.15278314078093,106.722118352285));
#34436=CARTESIAN_POINT('Ctrl Pts',(1.36829633275082,-2.11442204870785,106.726964688546));
#34437=CARTESIAN_POINT('Ctrl Pts',(1.55428769103191,-1.98635408150379,106.742347306281));
#34438=CARTESIAN_POINT('Ctrl Pts',(1.67259169940009,-1.88781673830012,106.753079315354));
#34439=CARTESIAN_POINT('Ctrl Pts',(1.84009812473606,-1.72011532924929,106.769253029855));
#34440=CARTESIAN_POINT('Ctrl Pts',(1.89605714629313,-1.65823019504619,106.774865064157));
#34441=CARTESIAN_POINT('Ctrl Pts',(1.97113171652223,-1.56642438114409,106.782681640062));
#34442=CARTESIAN_POINT('Ctrl Pts',(1.99284411990497,-1.53870663191259,106.78498086224));
#34443=CARTESIAN_POINT('Ctrl Pts',(2.0305234632661,-1.48846966088346,106.789042226085));
#34444=CARTESIAN_POINT('Ctrl Pts',(2.04671456062163,-1.46612655403242,106.790812688018));
#34445=CARTESIAN_POINT('Ctrl Pts',(2.07069829632754,-1.43185804823379,106.793475373802));
#34446=CARTESIAN_POINT('Ctrl Pts',(2.07876202172337,-1.42012583079747,106.794377827601));
#34447=CARTESIAN_POINT('Ctrl Pts',(2.09321413239448,-1.39871203760131,106.796008723936));
#34448=CARTESIAN_POINT('Ctrl Pts',(2.09963590355781,-1.38905357993688,106.796738404468));
#34449=CARTESIAN_POINT('Ctrl Pts',(2.11334116573075,-1.36812840804141,106.798306739406));
#34450=CARTESIAN_POINT('Ctrl Pts',(2.12060183297364,-1.35684711766214,106.799144532376));
#34451=CARTESIAN_POINT('Ctrl Pts',(2.1400893987707,-1.32602969115209,106.80141263594));
#34452=CARTESIAN_POINT('Ctrl Pts',(2.15213895821762,-1.30638253785931,106.802836452287));
#34453=CARTESIAN_POINT('Ctrl Pts',(2.21572749191487,-1.19943142137683,106.81047321577));
#34454=CARTESIAN_POINT('Ctrl Pts',(2.26223011997917,-1.10923505101745,106.816503531559));
#34455=CARTESIAN_POINT('Ctrl Pts',(2.37075433132497,-0.863335526133497,
106.832202296985));
#34456=CARTESIAN_POINT('Ctrl Pts',(2.42289426067117,-0.703849578767558,
106.841625986407));
#34457=CARTESIAN_POINT('Ctrl Pts',(2.47091192097962,-0.485359139711029,
106.854721856653));
#34458=CARTESIAN_POINT('Ctrl Pts',(2.48115219321345,-0.429956056647078,
106.858061058317));
#34459=CARTESIAN_POINT('Ctrl Pts',(2.49286405119169,-0.352050398636419,
106.862838924928));
#34460=CARTESIAN_POINT('Ctrl Pts',(2.49590542355734,-0.32979797667032,106.864212986107));
#34461=CARTESIAN_POINT('Ctrl Pts',(2.5007115231282,-0.290746217752555,106.866645372895));
#34462=CARTESIAN_POINT('Ctrl Pts',(2.50260568054328,-0.273963970336145,
106.86769743983));
#34463=CARTESIAN_POINT('Ctrl Pts',(2.50517245796069,-0.248968060895189,
106.869276154933));
#34464=CARTESIAN_POINT('Ctrl Pts',(2.50597387153135,-0.240767709911513,
106.869795956693));
#34465=CARTESIAN_POINT('Ctrl Pts',(2.50727865814311,-0.226703803424934,
106.87069087688));
#34466=CARTESIAN_POINT('Ctrl Pts',(2.50780174795306,-0.220842197136975,
106.87106489574));
#34467=CARTESIAN_POINT('Ctrl Pts',(2.50894693872986,-0.20748046942414,106.871919883087));
#34468=CARTESIAN_POINT('Ctrl Pts',(2.50955595289047,-0.199979504802744,
106.872401553832));
#34469=CARTESIAN_POINT('Ctrl Pts',(2.51113205142319,-0.179425183925563,
106.873725889042));
#34470=CARTESIAN_POINT('Ctrl Pts',(2.51203096385962,-0.166367050592956,
106.874572149448));
#34471=CARTESIAN_POINT('Ctrl Pts',(2.5161666262377,-0.0985782977269599,
106.878988780419));
#34472=CARTESIAN_POINT('Ctrl Pts',(2.51771641335306,-0.0437635962055014,
106.882639088061));
#34473=CARTESIAN_POINT('Ctrl Pts',(2.51645126434022,0.244386296747995,106.902099691672));
#34474=CARTESIAN_POINT('Ctrl Pts',(2.48299555575205,0.476456519781788,106.918572983341));
#34475=CARTESIAN_POINT('Ctrl Pts',(2.40487006445882,0.746087354917213,106.937285614347));
#34476=CARTESIAN_POINT('Ctrl Pts',(2.39041801702914,0.791169097729831,106.940405141234));
#34477=CARTESIAN_POINT('Ctrl Pts',(2.36318048929641,0.868555503862495,106.945743498774));
#34478=CARTESIAN_POINT('Ctrl Pts',(2.35098215947258,0.901051480322453,106.947980057709));
#34479=CARTESIAN_POINT('Ctrl Pts',(2.33233670789758,0.94776299795592,106.951189047578));
#34480=CARTESIAN_POINT('Ctrl Pts',(2.32642369775259,0.962186060828268,106.952179060037));
#34481=CARTESIAN_POINT('Ctrl Pts',(2.31581967285404,0.987382155442238,106.953907370227));
#34482=CARTESIAN_POINT('Ctrl Pts',(2.31118653816699,0.998178877466677,106.954647583877));
#34483=CARTESIAN_POINT('Ctrl Pts',(2.3020283553739,1.01911479569419,106.956082349339));
#34484=CARTESIAN_POINT('Ctrl Pts',(2.29751148651414,1.02925725228618,106.956777156834));
#34485=CARTESIAN_POINT('Ctrl Pts',(2.28521533274418,1.05638349278913,106.958634928802));
#34486=CARTESIAN_POINT('Ctrl Pts',(2.27731376972384,1.07331133616501,106.959793710683));
#34487=CARTESIAN_POINT('Ctrl Pts',(2.24700895384686,1.13639295301249,106.964111538885));
#34488=CARTESIAN_POINT('Ctrl Pts',(2.22338418791763,1.18194817248927,106.967228639571));
#34489=CARTESIAN_POINT('Ctrl Pts',(2.09333387098665,1.41500286422539,106.983233410034));
#34490=CARTESIAN_POINT('Ctrl Pts',(1.96454871445951,1.58897034589151,106.995291075475));
#34491=CARTESIAN_POINT('Ctrl Pts',(1.77097214112476,1.79040036688358,107.011567665163));
#34492=CARTESIAN_POINT('Ctrl Pts',(1.72503973352877,1.8346968791506,107.01532959863));
#34493=CARTESIAN_POINT('Ctrl Pts',(1.65043719390017,1.90136225680395,107.021380176019));
#34494=CARTESIAN_POINT('Ctrl Pts',(1.6228788549393,1.92493773219777,107.023603522261));
#34495=CARTESIAN_POINT('Ctrl Pts',(1.58624914291547,1.95492779508859,107.026558273332));
#34496=CARTESIAN_POINT('Ctrl Pts',(1.57762957652766,1.96189039858094,107.027253543476));
#34497=CARTESIAN_POINT('Ctrl Pts',(1.56348542193121,1.97316209955616,107.028394910984));
#34498=CARTESIAN_POINT('Ctrl Pts',(1.55798820457407,1.97750552142392,107.028838626335));
#34499=CARTESIAN_POINT('Ctrl Pts',(1.54723073535155,1.9859324376366,107.029707312746));
#34500=CARTESIAN_POINT('Ctrl Pts',(1.5419723026253,1.99001809277611,107.030132126949));
#34501=CARTESIAN_POINT('Ctrl Pts',(1.5301998914087,1.99909025320383,107.031083489174));
#34502=CARTESIAN_POINT('Ctrl Pts',(1.52367762884071,2.00406587392741,107.031610775091));
#34503=CARTESIAN_POINT('Ctrl Pts',(1.50107238146822,2.02113653917867,107.033438637201));
#34504=CARTESIAN_POINT('Ctrl Pts',(1.48486924715709,2.03307020620374,107.034749451249));
#34505=CARTESIAN_POINT('Ctrl Pts',(1.33188109177482,2.1429421376612,107.04711864875));
#34506=CARTESIAN_POINT('Ctrl Pts',(1.18575540582497,2.22712462742915,107.058847785858));
#34507=CARTESIAN_POINT('Ctrl Pts',(0.894088247691019,2.35825995116277,107.080897556558));
#34508=CARTESIAN_POINT('Ctrl Pts',(0.750485771436709,2.4078139260615,107.091199139716));
#34509=CARTESIAN_POINT('Ctrl Pts',(0.566954225203103,2.45311412334179,107.103526365418));
#34510=CARTESIAN_POINT('Ctrl Pts',(0.530434314292028,2.4612691195923,107.105940994534));
#34511=CARTESIAN_POINT('Ctrl Pts',(0.478000741989728,2.47175632357832,107.109355088195));
#34512=CARTESIAN_POINT('Ctrl Pts',(0.462226900996958,2.47475460277658,107.110375421833));
#34513=CARTESIAN_POINT('Ctrl Pts',(0.434789115058307,2.4796984632526,107.11213884487));
#34514=CARTESIAN_POINT('Ctrl Pts',(0.423138294957362,2.48171312489638,107.112884090315));
#34515=CARTESIAN_POINT('Ctrl Pts',(0.399174030091159,2.48568336160188,107.114409849717));
#34516=CARTESIAN_POINT('Ctrl Pts',(0.38685936972341,2.48762969861274,107.115190054142));
#34517=CARTESIAN_POINT('Ctrl Pts',(0.355446806058426,2.4923555628087,107.11717071872));
#34518=CARTESIAN_POINT('Ctrl Pts',(0.336330252339824,2.49500714968275,107.118367150429));
#34519=CARTESIAN_POINT('Ctrl Pts',(0.261661547090632,2.50449037300758,107.123007537263));
#34520=CARTESIAN_POINT('Ctrl Pts',(0.205915947458594,2.50968884843986,107.126400750155));
#34521=CARTESIAN_POINT('Ctrl Pts',(-0.0368404706516668,2.52418261208097,
107.140940069409));
#34522=CARTESIAN_POINT('Ctrl Pts',(-0.224377970224939,2.51446063642063,
107.151513092457));
#34523=CARTESIAN_POINT('Ctrl Pts',(-0.513036974492457,2.4669197658741,107.168431695489));
#34524=CARTESIAN_POINT('Ctrl Pts',(-0.615776510393933,2.44329991054807,
107.174599657339));
#34525=CARTESIAN_POINT('Ctrl Pts',(-0.737337379113756,2.40719801554209,
107.182390887225));
#34526=CARTESIAN_POINT('Ctrl Pts',(-0.757871962789267,2.4008120945672,107.183724497829));
#34527=CARTESIAN_POINT('Ctrl Pts',(-0.786957265933539,2.39135672184425,
107.185641718282));
#34528=CARTESIAN_POINT('Ctrl Pts',(-0.795577700844144,2.38850263249566,
107.186213514532));
#34529=CARTESIAN_POINT('Ctrl Pts',(-0.810441489727181,2.38349207475983,
107.187205902519));
#34530=CARTESIAN_POINT('Ctrl Pts',(-0.816692227877049,2.38135752939939,
107.187625225523));
#34531=CARTESIAN_POINT('Ctrl Pts',(-0.829809872755465,2.37682030264468,
107.188509503655));
#34532=CARTESIAN_POINT('Ctrl Pts',(-0.836674792114363,2.37441244627528,
107.18897474171));
#34533=CARTESIAN_POINT('Ctrl Pts',(-0.85511522574752,2.36785460206178,107.190230912942));
#34534=CARTESIAN_POINT('Ctrl Pts',(-0.866670756161856,2.36364956194156,
107.19102494862));
#34535=CARTESIAN_POINT('Ctrl Pts',(-0.919285349757061,2.34406549830082,
107.194670294172));
#34536=CARTESIAN_POINT('Ctrl Pts',(-0.959966617936126,2.32770104847975,
107.197572379141));
#34537=CARTESIAN_POINT('Ctrl Pts',(-1.167547076091,2.23783273385408,107.212743041166));
#34538=CARTESIAN_POINT('Ctrl Pts',(-1.32652653616748,2.1474146382059,107.225543998172));
#34539=CARTESIAN_POINT('Ctrl Pts',(-1.5693600164499,1.9719675435252,107.246005999776));
#34540=CARTESIAN_POINT('Ctrl Pts',(-1.65947508724273,1.89675931944158,107.253856652104));
#34541=CARTESIAN_POINT('Ctrl Pts',(-1.76603399516982,1.79439713634079,107.263437784845));
#34542=CARTESIAN_POINT('Ctrl Pts',(-1.78765196214386,1.77286145842605,107.265399266362));
#34543=CARTESIAN_POINT('Ctrl Pts',(-1.81917607289125,1.74029424969281,107.268287543781));
#34544=CARTESIAN_POINT('Ctrl Pts',(-1.82938429156376,1.72956028768908,107.269227362632));
#34545=CARTESIAN_POINT('Ctrl Pts',(-1.84744883653704,1.71022650405974,107.270898888472));
#34546=CARTESIAN_POINT('Ctrl Pts',(-1.8553412677625,1.70166115496169,107.271632121366));
#34547=CARTESIAN_POINT('Ctrl Pts',(-1.87193369860679,1.68340135913011,107.273180061547));
#34548=CARTESIAN_POINT('Ctrl Pts',(-1.88061849757676,1.67369351573479,107.273994119252));
#34549=CARTESIAN_POINT('Ctrl Pts',(-1.90367977858585,1.64750953545306,107.276166455543));
#34550=CARTESIAN_POINT('Ctrl Pts',(-1.91791780425728,1.63091253946289,107.277519022239));
#34551=CARTESIAN_POINT('Ctrl Pts',(-1.98321983997168,1.55275318554288,107.28377972546));
#34552=CARTESIAN_POINT('Ctrl Pts',(-2.03155053152866,1.48896195220122,107.288578251208));
#34553=CARTESIAN_POINT('Ctrl Pts',(-2.17073612603328,1.28582671935263,107.303099701702));
#34554=CARTESIAN_POINT('Ctrl Pts',(-2.25088842806099,1.13971363888592,107.312491585597));
#34555=CARTESIAN_POINT('Ctrl Pts',(-2.33210770891705,0.949082516362216,
107.324503685888));
#34556=CARTESIAN_POINT('Ctrl Pts',(-2.34723801617531,0.911019557884368,
107.32689269747));
#34557=CARTESIAN_POINT('Ctrl Pts',(-2.36143111856514,0.872610636121403,
107.329309102664));
#34558=CARTESIAN_POINT('Origin',(0.,0.,104.));
#34559=CARTESIAN_POINT('',(-2.36143103931299,0.872610850591009,108.330801621721));
#34560=CARTESIAN_POINT('',(-2.36143112101026,0.872610629504501,108.056228667503));
#34561=CARTESIAN_POINT('',(-2.36143112101026,0.872610629504505,104.));
#34562=CARTESIAN_POINT('',(-2.51749998978759,0.000226758633992978,107.11258330245));
#34563=CARTESIAN_POINT('Ctrl Pts',(-2.36143112101026,0.8726106295045,108.056228667503));
#34564=CARTESIAN_POINT('Ctrl Pts',(-2.3330193732305,0.949497597346625,108.051065788408));
#34565=CARTESIAN_POINT('Ctrl Pts',(-2.30085130969319,1.0249877363886,108.045902909314));
#34566=CARTESIAN_POINT('Ctrl Pts',(-2.26510104568141,1.09869172330229,108.04074003022));
#34567=CARTESIAN_POINT('Ctrl Pts',(-2.22931537254852,1.17246871089086,108.035572037513));
#34568=CARTESIAN_POINT('Ctrl Pts',(-2.1899406263118,1.24445558689348,108.030404044806));
#34569=CARTESIAN_POINT('Ctrl Pts',(-2.1471972905072,1.31428689624395,108.025236052099));
#34570=CARTESIAN_POINT('Ctrl Pts',(-2.10443039782417,1.38415669130532,108.020065211187));
#34571=CARTESIAN_POINT('Ctrl Pts',(-2.05829149119642,1.4518681640573,108.014894370275));
#34572=CARTESIAN_POINT('Ctrl Pts',(-2.00904340845741,1.51708629712809,108.009723529363));
#34573=CARTESIAN_POINT('Ctrl Pts',(-1.95971494943521,1.5824108707107,108.00454424928));
#34574=CARTESIAN_POINT('Ctrl Pts',(-1.90726749368202,1.64523362034305,107.999364969198));
#34575=CARTESIAN_POINT('Ctrl Pts',(-1.85200258460678,1.7052544316347,107.994185689115));
#34576=CARTESIAN_POINT('Ctrl Pts',(-1.82377852594175,1.7359073527625,107.991540605511));
#34577=CARTESIAN_POINT('Ctrl Pts',(-1.79482019034814,1.76583009294109,107.988895521906));
#34578=CARTESIAN_POINT('Ctrl Pts',(-1.76517104191664,1.79498675281433,107.986250438302));
#34579=CARTESIAN_POINT('Ctrl Pts',(-1.70626414405387,1.85291517491186,107.980995188895));
#34580=CARTESIAN_POINT('Ctrl Pts',(-1.64439384420539,1.90804774175334,107.975739939487));
#34581=CARTESIAN_POINT('Ctrl Pts',(-1.57985623667132,1.96006645842705,107.97048469008));
#34582=CARTESIAN_POINT('Ctrl Pts',(-1.51541012880355,2.01201142437774,107.965236891423));
#34583=CARTESIAN_POINT('Ctrl Pts',(-1.44830458093796,2.06085102195854,107.959989092765));
#34584=CARTESIAN_POINT('Ctrl Pts',(-1.37887225049189,2.10630424365129,107.954741294108));
#34585=CARTESIAN_POINT('Ctrl Pts',(-1.30893682295402,2.1520868131205,107.949455470625));
#34586=CARTESIAN_POINT('Ctrl Pts',(-1.23664108935141,2.19443339293706,107.944169647142));
#34587=CARTESIAN_POINT('Ctrl Pts',(-1.162358736518,2.23309838960138,107.938883823659));
#34588=CARTESIAN_POINT('Ctrl Pts',(-1.08874246841506,2.27141667990948,107.93364539779));
#34589=CARTESIAN_POINT('Ctrl Pts',(-1.01317548297708,2.30611893065921,107.928406971922));
#34590=CARTESIAN_POINT('Ctrl Pts',(-0.93604876330185,2.33701068947514,107.923168546053));
#34591=CARTESIAN_POINT('Ctrl Pts',(-0.858947409321192,2.3678922885057,107.917931843016));
#34592=CARTESIAN_POINT('Ctrl Pts',(-0.780287767892922,2.39496571311247,
107.912695139978));
#34593=CARTESIAN_POINT('Ctrl Pts',(-0.700481465352659,2.41808435888771,
107.907458436941));
#34594=CARTESIAN_POINT('Ctrl Pts',(-0.620677336696214,2.44120237492259,
107.902221876548));
#34595=CARTESIAN_POINT('Ctrl Pts',(-0.539727052516102,2.46036569891574,
107.896985316156));
#34596=CARTESIAN_POINT('Ctrl Pts',(-0.458056749043987,2.47547778512659,
107.891748755764));
#34597=CARTESIAN_POINT('Ctrl Pts',(-0.375049722851323,2.49083721545316,
107.886426486993));
#34598=CARTESIAN_POINT('Ctrl Pts',(-0.291299376297351,2.50201149345775,
107.881104218223));
#34599=CARTESIAN_POINT('Ctrl Pts',(-0.20726132009106,2.50895376505708,107.875781949452));
#34600=CARTESIAN_POINT('Ctrl Pts',(-0.124457844383297,2.51579404961009,
107.870537868702));
#34601=CARTESIAN_POINT('Ctrl Pts',(-0.0413755260267815,2.51852589088099,
107.865293787952));
#34602=CARTESIAN_POINT('Ctrl Pts',(0.0415489796359196,2.5171571131519,107.860049707201));
#34603=CARTESIAN_POINT('Ctrl Pts',(0.126328062838983,2.51575772318806,107.854688344421));
#34604=CARTESIAN_POINT('Ctrl Pts',(0.210941678431518,2.51007211743795,107.84932698164));
#34605=CARTESIAN_POINT('Ctrl Pts',(0.294929867698741,2.50016451921453,107.84396561886));
#34606=CARTESIAN_POINT('Ctrl Pts',(0.378918056965965,2.4902569209911,107.838604256079));
#34607=CARTESIAN_POINT('Ctrl Pts',(0.462280330108677,2.47612748106315,107.833242893299));
#34608=CARTESIAN_POINT('Ctrl Pts',(0.544570910994421,2.45789519160169,107.827881530518));
#34609=CARTESIAN_POINT('Ctrl Pts',(0.625232777039974,2.44002375996985,107.822626281111));
#34610=CARTESIAN_POINT('Ctrl Pts',(0.705162930103362,2.41814444185591,107.817371031703));
#34611=CARTESIAN_POINT('Ctrl Pts',(0.783933429502005,2.3923324660484,107.812115782296));
#34612=CARTESIAN_POINT('Ctrl Pts',(0.8625922502269,2.36655708575884,107.806867983639));
#34613=CARTESIAN_POINT('Ctrl Pts',(0.940094248178786,2.33686026505963,107.801620184981));
#34614=CARTESIAN_POINT('Ctrl Pts',(1.01602260056919,2.30336803944411,107.796372386324));
#34615=CARTESIAN_POINT('Ctrl Pts',(1.09250111933074,2.26963313378026,107.791086562841));
#34616=CARTESIAN_POINT('Ctrl Pts',(1.16738262880117,2.23204769166853,107.785800739358));
#34617=CARTESIAN_POINT('Ctrl Pts',(1.24025767266762,2.19079144497807,107.780514915875));
#34618=CARTESIAN_POINT('Ctrl Pts',(1.31247925104597,2.14990514020395,107.775276490006));
#34619=CARTESIAN_POINT('Ctrl Pts',(1.38272979443805,2.10541383039628,107.770038064138));
#34620=CARTESIAN_POINT('Ctrl Pts',(1.45063332633357,2.0575395992618,107.764799638269));
#34621=CARTESIAN_POINT('Ctrl Pts',(1.51851452588748,2.00968111316523,107.759562935232));
#34622=CARTESIAN_POINT('Ctrl Pts',(1.58404987014748,1.95844218106979,107.754326232194));
#34623=CARTESIAN_POINT('Ctrl Pts',(1.6468922778664,1.90408825297149,107.749089529157));
#34624=CARTESIAN_POINT('Ctrl Pts',(1.70973297378955,1.84973580544703,107.743852968764));
#34625=CARTESIAN_POINT('Ctrl Pts',(1.76988053070187,1.79226883325615,107.738616408372));
#34626=CARTESIAN_POINT('Ctrl Pts',(1.82702195624446,1.73199221170323,107.73337984798));
#34627=CARTESIAN_POINT('Ctrl Pts',(1.885098632895,1.6707290243348,107.728057579209));
#34628=CARTESIAN_POINT('Ctrl Pts',(1.94006953799661,1.60656373286699,107.722735310439));
#34629=CARTESIAN_POINT('Ctrl Pts',(1.99164731274398,1.53985299026877,107.717413041668));
#34630=CARTESIAN_POINT('Ctrl Pts',(2.04246737226403,1.4741222772616,107.712168960918));
#34631=CARTESIAN_POINT('Ctrl Pts',(2.08999311757033,1.4059208248335,107.706924880168));
#34632=CARTESIAN_POINT('Ctrl Pts',(2.13399337392747,1.33561915605971,107.701680799417));
#34633=CARTESIAN_POINT('Ctrl Pts',(2.17897768061521,1.26374521507374,107.696319436637));
#34634=CARTESIAN_POINT('Ctrl Pts',(2.22027665346995,1.18967643016715,107.690958073856));
#34635=CARTESIAN_POINT('Ctrl Pts',(2.25769373727083,1.11383357764438,107.685596711076));
#34636=CARTESIAN_POINT('Ctrl Pts',(2.29511082107171,1.03799072512162,107.680235348295));
#34637=CARTESIAN_POINT('Ctrl Pts',(2.32864587561049,0.960374297908778,107.674873985515));
#34638=CARTESIAN_POINT('Ctrl Pts',(2.35815600709104,0.881422995059944,107.669512622734));
#34639=CARTESIAN_POINT('Ctrl Pts',(2.38708206699787,0.804034315262545,107.664257373327));
#34640=CARTESIAN_POINT('Ctrl Pts',(2.41224796036825,0.725077290617908,107.659002123919));
#34641=CARTESIAN_POINT('Ctrl Pts',(2.43348379555697,0.644951832900452,107.653746874512));
#34642=CARTESIAN_POINT('Ctrl Pts',(2.45468952315555,0.56493997487986,107.648499075855));
#34643=CARTESIAN_POINT('Ctrl Pts',(2.47197614282711,0.483763416524039,107.643251277197));
#34644=CARTESIAN_POINT('Ctrl Pts',(2.48522243235326,0.401840405793344,107.63800347854));
#34645=CARTESIAN_POINT('Ctrl Pts',(2.49856470266671,0.31932379222374,107.632717655057));
#34646=CARTESIAN_POINT('Ctrl Pts',(2.50780767851231,0.236050307147021,107.627431831574));
#34647=CARTESIAN_POINT('Ctrl Pts',(2.51287918846662,0.15246125465624,107.622146008091));
#34648=CARTESIAN_POINT('Ctrl Pts',(2.51790522254122,0.0696217394294053,
107.616907582222));
#34649=CARTESIAN_POINT('Ctrl Pts',(2.51883427313051,-0.0135272374751904,
107.611669156354));
#34650=CARTESIAN_POINT('Ctrl Pts',(2.51564792133641,-0.096549396040497,
107.606430730485));
#34651=CARTESIAN_POINT('Ctrl Pts',(2.51246261748039,-0.179544249999562,
107.601194027448));
#34652=CARTESIAN_POINT('Ctrl Pts',(2.50516461702329,-0.262411907737051,
107.59595732441));
#34653=CARTESIAN_POINT('Ctrl Pts',(2.49378760844704,-0.344716715515772,
107.590720621373));
#34654=CARTESIAN_POINT('Ctrl Pts',(2.48241090977482,-0.427019281352698,
107.58548406098));
#34655=CARTESIAN_POINT('Ctrl Pts',(2.46695548810185,-0.508758570780944,
107.580247500588));
#34656=CARTESIAN_POINT('Ctrl Pts',(2.44750666130299,-0.589506058389143,
107.575010940196));
#34657=CARTESIAN_POINT('Ctrl Pts',(2.42773950963495,-0.671575164709622,
107.569688671425));
#34658=CARTESIAN_POINT('Ctrl Pts',(2.40384715326952,-0.752619228922522,
107.564366402655));
#34659=CARTESIAN_POINT('Ctrl Pts',(2.37597229701542,-0.832203036413159,
107.559044133884));
#34660=CARTESIAN_POINT('Ctrl Pts',(2.34850694278321,-0.910617699576022,
107.553800053134));
#34661=CARTESIAN_POINT('Ctrl Pts',(2.3171755568698,-0.987614315326077,107.548555972384));
#34662=CARTESIAN_POINT('Ctrl Pts',(2.28216306772662,-1.06279724421201,107.543311891633));
#34663=CARTESIAN_POINT('Ctrl Pts',(2.24636753652028,-1.13966161298381,107.537950528853));
#34664=CARTESIAN_POINT('Ctrl Pts',(2.2067245014078,-1.21462973836698,107.532589166072));
#34665=CARTESIAN_POINT('Ctrl Pts',(2.16347989151034,-1.28730765904285,107.527227803292));
#34666=CARTESIAN_POINT('Ctrl Pts',(2.12023528161289,-1.35998557971873,107.521866440511));
#34667=CARTESIAN_POINT('Ctrl Pts',(2.07338943405645,-1.43037290970733,107.516505077731));
#34668=CARTESIAN_POINT('Ctrl Pts',(2.02323252747275,-1.49811094041004,107.51114371495));
#34669=CARTESIAN_POINT('Ctrl Pts',(1.97406833836912,-1.56450828382311,107.505888465543));
#34670=CARTESIAN_POINT('Ctrl Pts',(1.92154140516658,-1.62860551635473,107.500633216135));
#34671=CARTESIAN_POINT('Ctrl Pts',(1.86589467300482,-1.69004240161371,107.495377966728));
#34672=CARTESIAN_POINT('Ctrl Pts',(1.81032683526791,-1.75139218332611,107.490130168071));
#34673=CARTESIAN_POINT('Ctrl Pts',(1.7516482914465,-1.81008877046016,107.484882369413));
#34674=CARTESIAN_POINT('Ctrl Pts',(1.69014386507701,-1.86580276699938,107.479634570756));
#34675=CARTESIAN_POINT('Ctrl Pts',(1.62819378611536,-1.9219204594747,107.474348747273));
#34676=CARTESIAN_POINT('Ctrl Pts',(1.56337698190051,-1.97501177524924,107.46906292379));
#34677=CARTESIAN_POINT('Ctrl Pts',(1.49602432105695,-2.02477590878746,107.463777100307));
#34678=CARTESIAN_POINT('Ctrl Pts',(1.42927560687408,-2.07409381077527,107.458538674438));
#34679=CARTESIAN_POINT('Ctrl Pts',(1.3600367095692,-2.12014368151661,107.45330024857));
#34680=CARTESIAN_POINT('Ctrl Pts',(1.28866354925701,-2.16267253804554,107.448061822701));
#34681=CARTESIAN_POINT('Ctrl Pts',(1.2173138623895,-2.20518740754129,107.442825119664));
#34682=CARTESIAN_POINT('Ctrl Pts',(1.14383170264682,-2.24418332667537,107.437588416626));
#34683=CARTESIAN_POINT('Ctrl Pts',(1.06860083476931,-2.27945136072923,107.432351713589));
#34684=CARTESIAN_POINT('Ctrl Pts',(0.993372016143048,-2.31471843409947,
107.427115153196));
#34685=CARTESIAN_POINT('Ctrl Pts',(0.916395002318008,-2.34625762936329,
107.421878592804));
#34686=CARTESIAN_POINT('Ctrl Pts',(0.838075688553412,-2.37390719916675,
107.416642032412));
#34687=CARTESIAN_POINT('Ctrl Pts',(0.758474498737001,-2.40200931789678,
107.411319763641));
#34688=CARTESIAN_POINT('Ctrl Pts',(0.677487132195316,-2.42609316097623,
107.405997494871));
#34689=CARTESIAN_POINT('Ctrl Pts',(0.595556339445428,-2.44604147482138,
107.4006752261));
#34690=CARTESIAN_POINT('Ctrl Pts',(0.514829169952915,-2.46569673334894,
107.39543114535));
#34691=CARTESIAN_POINT('Ctrl Pts',(0.433186580706433,-2.48133713620051,
107.3901870646));
#34692=CARTESIAN_POINT('Ctrl Pts',(0.351061115609519,-2.49290239341756,
107.384942983849));
#34693=CARTESIAN_POINT('Ctrl Pts',(0.267098943234842,-2.50472630356369,
107.379581621069));
#34694=CARTESIAN_POINT('Ctrl Pts',(0.182632545677586,-2.51229054444311,
107.374220258288));
#34695=CARTESIAN_POINT('Ctrl Pts',(0.0981262711464113,-2.51558690665039,
107.368858895508));
#34696=CARTESIAN_POINT('Ctrl Pts',(0.0136199966152368,-2.51888326885768,
107.363497532727));
#34697=CARTESIAN_POINT('Ctrl Pts',(-0.0709256475840465,-2.51791182502412,
107.358136169947));
#34698=CARTESIAN_POINT('Ctrl Pts',(-0.155051791237268,-2.51272067529085,
107.352774807166));
#34699=CARTESIAN_POINT('Ctrl Pts',(-0.237512890153433,-2.50763227003352,
107.347519557759));
#34700=CARTESIAN_POINT('Ctrl Pts',(-0.319875525081196,-2.49847092200903,
107.342264308351));
#34701=CARTESIAN_POINT('Ctrl Pts',(-0.401705260654237,-2.48524428046072,
107.337009058944));
#34702=CARTESIAN_POINT('Ctrl Pts',(-0.483418980251928,-2.47203639128536,
107.331761260287));
#34703=CARTESIAN_POINT('Ctrl Pts',(-0.564600849489855,-2.4547747299149,
107.326513461629));
#34704=CARTESIAN_POINT('Ctrl Pts',(-0.644819500911588,-2.43351886395896,
107.321265662972));
#34705=CARTESIAN_POINT('Ctrl Pts',(-0.725619405619257,-2.41210898092952,
107.315979839489));
#34706=CARTESIAN_POINT('Ctrl Pts',(-0.805441601937452,-2.38664679535493,
107.310694016006));
#34707=CARTESIAN_POINT('Ctrl Pts',(-0.883853634564483,-2.35724606324142,
107.305408192523));
#34708=CARTESIAN_POINT('Ctrl Pts',(-0.961562551907393,-2.32810896546336,
107.300169766654));
#34709=CARTESIAN_POINT('Ctrl Pts',(-1.03788605394107,-2.29510383658022,
107.294931340786));
#34710=CARTESIAN_POINT('Ctrl Pts',(-1.11241815924337,-2.25839148266761,
107.289692914917));
#34711=CARTESIAN_POINT('Ctrl Pts',(-1.18692575217654,-2.22169120283726,
107.28445621188));
#34712=CARTESIAN_POINT('Ctrl Pts',(-1.25964270488015,-2.18128632319323,
107.279219508842));
#34713=CARTESIAN_POINT('Ctrl Pts',(-1.33018482321224,-2.13738498780538,
107.273982805805));
#34714=CARTESIAN_POINT('Ctrl Pts',(-1.40072502001217,-2.09348484826804,
107.268746245412));
#34715=CARTESIAN_POINT('Ctrl Pts',(-1.46909010902132,-2.04608868703059,
107.26350968502));
#34716=CARTESIAN_POINT('Ctrl Pts',(-1.53492342749955,-1.9954489023057,107.258273124628));
#34717=CARTESIAN_POINT('Ctrl Pts',(-1.60183425994372,-1.94398028080736,
107.252950855857));
#34718=CARTESIAN_POINT('Ctrl Pts',(-1.6661292998544,-1.88916118851532,107.247628587087));
#34719=CARTESIAN_POINT('Ctrl Pts',(-1.72746913961996,-1.83129916225085,
107.242306318316));
#34720=CARTESIAN_POINT('Ctrl Pts',(-1.78790785228463,-1.7742871714638,107.237062237566));
#34721=CARTESIAN_POINT('Ctrl Pts',(-1.8454773366962,-1.71432143920929,107.231818156815));
#34722=CARTESIAN_POINT('Ctrl Pts',(-1.89989152289909,-1.65173195501455,
107.226574076065));
#34723=CARTESIAN_POINT('Ctrl Pts',(-1.95552266332799,-1.58774267891609,
107.221212713285));
#34724=CARTESIAN_POINT('Ctrl Pts',(-2.0078553522263,-1.52101127904271,107.215851350504));
#34725=CARTESIAN_POINT('Ctrl Pts',(-2.05662988850103,-1.45192277746588,
107.210489987723));
#34726=CARTESIAN_POINT('Ctrl Pts',(-2.10540442477575,-1.38283427588906,
107.205128624943));
#34727=CARTESIAN_POINT('Ctrl Pts',(-2.15062059314602,-1.31138913767721,
107.199767262162));
#34728=CARTESIAN_POINT('Ctrl Pts',(-2.19206890703471,-1.2379984478228,107.194405899382));
#34729=CARTESIAN_POINT('Ctrl Pts',(-2.23446890777379,-1.16292264829992,
107.18892143537));
#34730=CARTESIAN_POINT('Ctrl Pts',(-2.27307163741358,-1.08555429773656,
107.183436971359));
#34731=CARTESIAN_POINT('Ctrl Pts',(-2.30763425924455,-1.00629537192658,
107.177952507347));
#34732=CARTESIAN_POINT('Ctrl Pts',(-2.34210712091703,-0.927242283907992,
107.172482286652));
#34733=CARTESIAN_POINT('Ctrl Pts',(-2.37256061323769,-0.846308768249363,
107.167012065957));
#34734=CARTESIAN_POINT('Ctrl Pts',(-2.39879783154439,-0.763920947073663,
107.161541845262));
#34735=CARTESIAN_POINT('Ctrl Pts',(-2.42499481295695,-0.681659474278365,
107.156080013592));
#34736=CARTESIAN_POINT('Ctrl Pts',(-2.4469882590584,-0.597948514163733,
107.150618181923));
#34737=CARTESIAN_POINT('Ctrl Pts',(-2.4646291608708,-0.513234205198073,
107.145156350253));
#34738=CARTESIAN_POINT('Ctrl Pts',(-2.48223686891322,-0.428679297793389,
107.139704795767));
#34739=CARTESIAN_POINT('Ctrl Pts',(-2.49550826265296,-0.343125195358922,
107.134253241281));
#34740=CARTESIAN_POINT('Ctrl Pts',(-2.50434439920526,-0.257031866058002,
107.128801686795));
#34741=CARTESIAN_POINT('Ctrl Pts',(-2.51310690653038,-0.171655930072997,
107.123395558694));
#34742=CARTESIAN_POINT('Ctrl Pts',(-2.51750773395471,-0.0857501128067695,
107.117989430593));
#34743=CARTESIAN_POINT('Ctrl Pts',(-2.51749998978765,0.000226757967744173,
107.112583302492));
#34744=CARTESIAN_POINT('Ctrl Pts',(-2.51749998978759,0.000226758633996389,
107.11258330245));
#34745=CARTESIAN_POINT('Ctrl Pts',(-2.51749207334436,0.0881160063818547,
107.107056926255));
#34746=CARTESIAN_POINT('Ctrl Pts',(-2.51287737051979,0.175904335234615,
107.101530550059));
#34747=CARTESIAN_POINT('Ctrl Pts',(-2.5037131461786,0.263109733100915,107.096004173863));
#34748=CARTESIAN_POINT('Ctrl Pts',(-2.49453499866111,0.350447621845197,
107.090469401462));
#34749=CARTESIAN_POINT('Ctrl Pts',(-2.48079360116063,0.437200436864105,
107.084934629061));
#34750=CARTESIAN_POINT('Ctrl Pts',(-2.46259737508519,0.522896183026359,
107.07939985666));
#34751=CARTESIAN_POINT('Ctrl Pts',(-2.44435528551196,0.608807924892799,
107.073851133893));
#34752=CARTESIAN_POINT('Ctrl Pts',(-2.42163602170516,0.693656903619571,
107.068302411125));
#34753=CARTESIAN_POINT('Ctrl Pts',(-2.39459810500259,0.776985305857198,
107.062753688358));
#34754=CARTESIAN_POINT('Ctrl Pts',(-2.38417952725892,0.809094415686877,
107.060615587255));
#34755=CARTESIAN_POINT('Ctrl Pts',(-2.37312021907302,0.840977964248501,
107.058477486152));
#34756=CARTESIAN_POINT('Ctrl Pts',(-2.36143112101026,0.872610629504506,
107.056339385048));
#34757=CARTESIAN_POINT('Ctrl Pts',(-2.36143111856514,0.872610636121403,
107.329309102664));
#34758=CARTESIAN_POINT('Ctrl Pts',(-2.37273689814697,0.84201529540582,107.331233935146));
#34759=CARTESIAN_POINT('Ctrl Pts',(-2.38344800047675,0.811200434712442,
107.33317617158));
#34760=CARTESIAN_POINT('Ctrl Pts',(-2.40590495362348,0.742303791526028,
107.337544213279));
#34761=CARTESIAN_POINT('Ctrl Pts',(-2.41735015134349,0.704138768383658,
107.339980917275));
#34762=CARTESIAN_POINT('Ctrl Pts',(-2.43091236365006,0.654677368318164,
107.343179686073));
#34763=CARTESIAN_POINT('Ctrl Pts',(-2.43386499499604,0.64361366578133,107.343897802894));
#34764=CARTESIAN_POINT('Ctrl Pts',(-2.43852283196717,0.625669949665931,
107.345067266237));
#34765=CARTESIAN_POINT('Ctrl Pts',(-2.44027467697771,0.618802057110833,
107.345516003933));
#34766=CARTESIAN_POINT('Ctrl Pts',(-2.44360454133335,0.605513673250652,
107.346386590374));
#34767=CARTESIAN_POINT('Ctrl Pts',(-2.44518630160325,0.599094240915663,
107.346808224389));
#34768=CARTESIAN_POINT('Ctrl Pts',(-2.44862974977171,0.584878489911253,
107.347744182174));
#34769=CARTESIAN_POINT('Ctrl Pts',(-2.45047952588004,0.577079360666258,
107.348259166738));
#34770=CARTESIAN_POINT('Ctrl Pts',(-2.45691366547512,0.549362560083878,
107.35009430998));
#34771=CARTESIAN_POINT('Ctrl Pts',(-2.46129254261949,0.529398657675405,
107.351425227625));
#34772=CARTESIAN_POINT('Ctrl Pts',(-2.49990059893568,0.342535127648288,
107.363953619616));
#34773=CARTESIAN_POINT('Ctrl Pts',(-2.51734456373288,0.172630788688992,
107.375839042506));
#34774=CARTESIAN_POINT('Ctrl Pts',(-2.5176397475312,-0.153039840341469,
107.39828852783));
#34775=CARTESIAN_POINT('Ctrl Pts',(-2.50340621560271,-0.308062823131997,
107.408829194306));
#34776=CARTESIAN_POINT('Ctrl Pts',(-2.46882862719299,-0.493777574152181,
107.421109713271));
#34777=CARTESIAN_POINT('Ctrl Pts',(-2.46203120364396,-0.526624735993077,
107.423269681965));
#34778=CARTESIAN_POINT('Ctrl Pts',(-2.45119930196303,-0.574159955287971,
107.426379296072));
#34779=CARTESIAN_POINT('Ctrl Pts',(-2.44768500646156,-0.588961626850756,
107.42734528467));
#34780=CARTESIAN_POINT('Ctrl Pts',(-2.44122323026002,-0.615120335428029,
107.429048648769));
#34781=CARTESIAN_POINT('Ctrl Pts',(-2.43833014717352,-0.626490213755297,
107.42978773469));
#34782=CARTESIAN_POINT('Ctrl Pts',(-2.43214223862213,-0.650116483086283,
107.431321032895));
#34783=CARTESIAN_POINT('Ctrl Pts',(-2.42883399453497,-0.662369041288485,
107.432114791536));
#34784=CARTESIAN_POINT('Ctrl Pts',(-2.41998475919982,-0.694185449099741,
107.434172598875));
#34785=CARTESIAN_POINT('Ctrl Pts',(-2.41429908822412,-0.713708359657247,
107.435431967996));
#34786=CARTESIAN_POINT('Ctrl Pts',(-2.3875395192746,-0.801611517651557,
107.441089933652));
#34787=CARTESIAN_POINT('Ctrl Pts',(-2.36379169565279,-0.86914681868696,
107.445401461449));
#34788=CARTESIAN_POINT('Ctrl Pts',(-2.24976858893047,-1.15398984590854,
107.463588057807));
#34789=CARTESIAN_POINT('Ctrl Pts',(-2.13217136208571,-1.35903578456481,
107.476574377692));
#34790=CARTESIAN_POINT('Ctrl Pts',(-1.95534159602503,-1.58658455450562,
107.493749563226));
#34791=CARTESIAN_POINT('Ctrl Pts',(-1.92153396896601,-1.62736524213994,
107.496959424955));
#34792=CARTESIAN_POINT('Ctrl Pts',(-1.87789067353578,-1.67675301318114,
107.50105789196));
#34793=CARTESIAN_POINT('Ctrl Pts',(-1.86923835645084,-1.6863931923179,107.501868323682));
#34794=CARTESIAN_POINT('Ctrl Pts',(-1.85546325871562,-1.70150478009377,
107.503156122928));
#34795=CARTESIAN_POINT('Ctrl Pts',(-1.85038964103753,-1.70702097058127,
107.503629924334));
#34796=CARTESIAN_POINT('Ctrl Pts',(-1.84128479801558,-1.71683174382802,
107.504479439222));
#34797=CARTESIAN_POINT('Ctrl Pts',(-1.83726303814441,-1.7211349366474,107.504854440493));
#34798=CARTESIAN_POINT('Ctrl Pts',(-1.82754816163319,-1.73145678619184,
107.505759672488));
#34799=CARTESIAN_POINT('Ctrl Pts',(-1.82184044073542,-1.73746144975727,
107.506291002147));
#34800=CARTESIAN_POINT('Ctrl Pts',(-1.80424748488139,-1.75578767062189,
107.507926842971));
#34801=CARTESIAN_POINT('Ctrl Pts',(-1.79226639939556,-1.76801596338372,
107.509038269328));
#34802=CARTESIAN_POINT('Ctrl Pts',(-1.76400093125974,-1.79628208595371,
107.511652258178));
#34803=CARTESIAN_POINT('Ctrl Pts',(-1.74762118959818,-1.81222203874087,
107.513160962257));
#34804=CARTESIAN_POINT('Ctrl Pts',(-1.68903451856967,-1.86770271170236,
107.518528955032));
#34805=CARTESIAN_POINT('Ctrl Pts',(-1.64568636780856,-1.90600801817147,
107.522449708055));
#34806=CARTESIAN_POINT('Ctrl Pts',(-1.47041986490487,-2.05044624877503,
107.537992097549));
#34807=CARTESIAN_POINT('Ctrl Pts',(-1.32923894108942,-2.14466679944575,
107.549817972916));
#34808=CARTESIAN_POINT('Ctrl Pts',(-1.09345534932311,-2.26973247681531,
107.56785046946));
#34809=CARTESIAN_POINT('Ctrl Pts',(-1.00464834151209,-2.31041465803188,
107.574309502234));
#34810=CARTESIAN_POINT('Ctrl Pts',(-0.892417811418203,-2.35412786357626,
107.582065204711));
#34811=CARTESIAN_POINT('Ctrl Pts',(-0.871030385627863,-2.36212482134271,
107.583525828777));
#34812=CARTESIAN_POINT('Ctrl Pts',(-0.836953763574405,-2.37434060741084,
107.585826297673));
#34813=CARTESIAN_POINT('Ctrl Pts',(-0.824335072346266,-2.37875106349208,
107.586672419832));
#34814=CARTESIAN_POINT('Ctrl Pts',(-0.800699199987404,-2.38680155187183,
107.588246770937));
#34815=CARTESIAN_POINT('Ctrl Pts',(-0.789690876675213,-2.39046631087393,
107.588975793924));
#34816=CARTESIAN_POINT('Ctrl Pts',(-0.765059694475698,-2.39847751141546,
107.590597762841));
#34817=CARTESIAN_POINT('Ctrl Pts',(-0.751424278540976,-2.40278427575851,
107.591489395961));
#34818=CARTESIAN_POINT('Ctrl Pts',(-0.711074736937883,-2.41515166064484,
107.594109997489));
#34819=CARTESIAN_POINT('Ctrl Pts',(-0.68426192011347,-2.42288475684472,
107.595828372961));
#34820=CARTESIAN_POINT('Ctrl Pts',(-0.515246274224209,-2.46860098913525,
107.606526678152));
#34821=CARTESIAN_POINT('Ctrl Pts',(-0.370063688639742,-2.49449995921898,
107.615104390183));
#34822=CARTESIAN_POINT('Ctrl Pts',(-0.0679157977862989,-2.521422548848,
107.632575484822));
#34823=CARTESIAN_POINT('Ctrl Pts',(0.0885398498160474,-2.52078086286033,
107.641422385245));
#34824=CARTESIAN_POINT('Ctrl Pts',(0.287894343465228,-2.5013747994269,107.653443049762));
#34825=CARTESIAN_POINT('Ctrl Pts',(0.331753499104943,-2.49593632124955,
107.656136061144));
#34826=CARTESIAN_POINT('Ctrl Pts',(0.387635271294029,-2.4875082234345,107.659655108473));
#34827=CARTESIAN_POINT('Ctrl Pts',(0.399812874536767,-2.48557999591668,
107.660427339813));
#34828=CARTESIAN_POINT('Ctrl Pts',(0.419159555203438,-2.48237075144017,
107.661663445374));
#34829=CARTESIAN_POINT('Ctrl Pts',(0.426338266092768,-2.4811479117533,107.662124142499));
#34830=CARTESIAN_POINT('Ctrl Pts',(0.440015683495928,-2.47875695580567,
107.663005948195));
#34831=CARTESIAN_POINT('Ctrl Pts',(0.446515207308212,-2.47759440047486,
107.66342674747));
#34832=CARTESIAN_POINT('Ctrl Pts',(0.461926892671691,-2.47477513481603,
107.664428651862));
#34833=CARTESIAN_POINT('Ctrl Pts',(0.470834768384566,-2.47309584062801,
107.665011001159));
#34834=CARTESIAN_POINT('Ctrl Pts',(0.50075171350041,-2.46728847023686,107.666977318281));
#34835=CARTESIAN_POINT('Ctrl Pts',(0.521716494107387,-2.46294062085169,
107.668372697634));
#34836=CARTESIAN_POINT('Ctrl Pts',(0.644520579454797,-2.43583426928961,
107.67663911985));
#34837=CARTESIAN_POINT('Ctrl Pts',(0.744912145804099,-2.40703073883812,
107.683769243345));
#34838=CARTESIAN_POINT('Ctrl Pts',(1.01690754978523,-2.31034328907831,107.703663216678));
#34839=CARTESIAN_POINT('Ctrl Pts',(1.18331889751004,-2.229699782988,107.716452910183));
#34840=CARTESIAN_POINT('Ctrl Pts',(1.38948780979697,-2.10014844737259,107.732579459345));
#34841=CARTESIAN_POINT('Ctrl Pts',(1.43841432564662,-2.06694582650521,107.736435458679));
#34842=CARTESIAN_POINT('Ctrl Pts',(1.50202424560496,-2.02042499510938,107.741491039627));
#34843=CARTESIAN_POINT('Ctrl Pts',(1.5177818467596,-2.00861452172274,107.742747102242));
#34844=CARTESIAN_POINT('Ctrl Pts',(1.54335440051805,-1.9889748594715,107.744792071503));
#34845=CARTESIAN_POINT('Ctrl Pts',(1.55325199953916,-1.98125516589704,107.74558519594));
#34846=CARTESIAN_POINT('Ctrl Pts',(1.57232955797509,-1.9661446765782,107.74711731818));
#34847=CARTESIAN_POINT('Ctrl Pts',(1.58151615113009,-1.95876282367395,107.747856641001));
#34848=CARTESIAN_POINT('Ctrl Pts',(1.60291250815966,-1.94132120007636,107.749582441287));
#34849=CARTESIAN_POINT('Ctrl Pts',(1.61508004419543,-1.93121023699515,107.750566838334));
#34850=CARTESIAN_POINT('Ctrl Pts',(1.65464479149441,-1.89769730325464,107.753778452495));
#34851=CARTESIAN_POINT('Ctrl Pts',(1.68163577053573,-1.87382116955119,107.755986379395));
#34852=CARTESIAN_POINT('Ctrl Pts',(1.74462897033323,-1.8156397926821,107.761189604843));
#34853=CARTESIAN_POINT('Ctrl Pts',(1.78014612075191,-1.78083079818497,107.764164142176));
#34854=CARTESIAN_POINT('Ctrl Pts',(1.91777692789404,-1.63770895711041,107.775911732827));
#34855=CARTESIAN_POINT('Ctrl Pts',(2.01122624469881,-1.52148947275829,107.784380158775));
#34856=CARTESIAN_POINT('Ctrl Pts',(2.12439767532785,-1.35194876269409,107.796125722356));
#34857=CARTESIAN_POINT('Ctrl Pts',(2.153423502941,-1.30521943538464,107.799308739364));
#34858=CARTESIAN_POINT('Ctrl Pts',(2.19219183319685,-1.23798734341174,107.80386313478));
#34859=CARTESIAN_POINT('Ctrl Pts',(2.20322414981745,-1.21824504784661,107.805197583276));
#34860=CARTESIAN_POINT('Ctrl Pts',(2.24106598413371,-1.14833150984222,107.80992221766));
#34861=CARTESIAN_POINT('Ctrl Pts',(2.2664377331786,-1.09740645814627,107.813361653027));
#34862=CARTESIAN_POINT('Ctrl Pts',(2.29555642396273,-1.03363533027569,107.817719004292));
#34863=CARTESIAN_POINT('Ctrl Pts',(2.30095668485284,-1.021557442505,107.818546441299));
#34864=CARTESIAN_POINT('Ctrl Pts',(2.30929185406096,-1.00251409226718,107.819855341307));
#34865=CARTESIAN_POINT('Ctrl Pts',(2.31229110630431,-0.99557682204169,107.820333042218));
#34866=CARTESIAN_POINT('Ctrl Pts',(2.31756825163488,-0.983218301060807,
107.821185800388));
#34867=CARTESIAN_POINT('Ctrl Pts',(2.31985844539506,-0.977802443984049,
107.821560110185));
#34868=CARTESIAN_POINT('Ctrl Pts',(2.32529465394902,-0.964820277694676,
107.822458784537));
#34869=CARTESIAN_POINT('Ctrl Pts',(2.32842269464495,-0.957246648724728,
107.822984202635));
#34870=CARTESIAN_POINT('Ctrl Pts',(2.3377979674255,-0.934229334897529,107.824584186073));
#34871=CARTESIAN_POINT('Ctrl Pts',(2.34392878405485,-0.918739139793101,
107.825665246166));
#34872=CARTESIAN_POINT('Ctrl Pts',(2.39868530283107,-0.776274468189472,
107.835639745301));
#34873=CARTESIAN_POINT('Ctrl Pts',(2.43709837862244,-0.64562907928827,107.845005744956));
#34874=CARTESIAN_POINT('Ctrl Pts',(2.50516842552434,-0.318283069590887,
107.86810138086));
#34875=CARTESIAN_POINT('Ctrl Pts',(2.52246433399614,-0.119895850838917,
107.881728559255));
#34876=CARTESIAN_POINT('Ctrl Pts',(2.51529125392845,0.110063913837987,107.896660858092));
#34877=CARTESIAN_POINT('Ctrl Pts',(2.51371212515731,0.141617997356326,107.89869301647));
#34878=CARTESIAN_POINT('Ctrl Pts',(2.51050664270669,0.188117467548634,107.901664158685));
#34879=CARTESIAN_POINT('Ctrl Pts',(2.50933976865435,0.203090438096633,107.902617276328));
#34880=CARTESIAN_POINT('Ctrl Pts',(2.50702813035546,0.229678911893988,107.904303644521));
#34881=CARTESIAN_POINT('Ctrl Pts',(2.50593645270978,0.241298469426901,107.90503852366));
#34882=CARTESIAN_POINT('Ctrl Pts',(2.50346696871456,0.265755668878032,107.906581089356));
#34883=CARTESIAN_POINT('Ctrl Pts',(2.50207112271808,0.278591180274351,107.907388191469));
#34884=CARTESIAN_POINT('Ctrl Pts',(2.49810622332229,0.312613158775157,107.90952131565));
#34885=CARTESIAN_POINT('Ctrl Pts',(2.49536637464797,0.333778953187105,107.910841988435));
#34886=CARTESIAN_POINT('Ctrl Pts',(2.48057161178308,0.43767589124299,107.917296716172));
#34887=CARTESIAN_POINT('Ctrl Pts',(2.46466929813009,0.519810615605896,107.922309250048));
#34888=CARTESIAN_POINT('Ctrl Pts',(2.42145986710482,0.695572546135234,107.932970764743));
#34889=CARTESIAN_POINT('Ctrl Pts',(2.39274418269861,0.7887114204011,107.938578592326));
#34890=CARTESIAN_POINT('Ctrl Pts',(2.3012189893111,1.03404301987399,107.953626784182));
#34891=CARTESIAN_POINT('Ctrl Pts',(2.22878086077839,1.18210609476309,107.962998935097));
#34892=CARTESIAN_POINT('Ctrl Pts',(2.13178222107162,1.33929934022117,107.974358420027));
#34893=CARTESIAN_POINT('Ctrl Pts',(2.12091621140433,1.35644112473726,107.975617653109));
#34894=CARTESIAN_POINT('Ctrl Pts',(2.1053526965474,1.38034925396387,107.977405725032));
#34895=CARTESIAN_POINT('Ctrl Pts',(2.10082709740946,1.38722728567323,107.977923879195));
#34896=CARTESIAN_POINT('Ctrl Pts',(2.09257601745881,1.39963434870028,107.978865609198));
#34897=CARTESIAN_POINT('Ctrl Pts',(2.0888621151652,1.40517107902617,107.979288425012));
#34898=CARTESIAN_POINT('Ctrl Pts',(2.0812070926189,1.41648586492994,107.98015788932));
#34899=CARTESIAN_POINT('Ctrl Pts',(2.07726382989551,1.4222623337698,107.980604672529));
#34900=CARTESIAN_POINT('Ctrl Pts',(2.06704224577365,1.43710270214981,107.981759844823));
#34901=CARTESIAN_POINT('Ctrl Pts',(2.06072843375132,1.44614180979949,107.982470546693));
#34902=CARTESIAN_POINT('Ctrl Pts',(2.03368248268498,1.48432510538756,107.98550197938));
#34903=CARTESIAN_POINT('Ctrl Pts',(2.01239096355288,1.5130656831663,107.987856599212));
#34904=CARTESIAN_POINT('Ctrl Pts',(1.95223488177878,1.59075155172447,107.994403082894));
#34905=CARTESIAN_POINT('Ctrl Pts',(1.91214975774352,1.63871713307986,107.99865021433));
#34906=CARTESIAN_POINT('Ctrl Pts',(1.73528554908213,1.83501760207041,108.016769321747));
#34907=CARTESIAN_POINT('Ctrl Pts',(1.58269507948169,1.96814698947047,108.030859084748));
#34908=CARTESIAN_POINT('Ctrl Pts',(1.36313489513516,2.11748256622686,108.048494486417));
#34909=CARTESIAN_POINT('Ctrl Pts',(1.30908380261991,2.15131818668927,108.052660770032));
#34910=CARTESIAN_POINT('Ctrl Pts',(1.23625364841554,2.19314675845504,108.058052147831));
#34911=CARTESIAN_POINT('Ctrl Pts',(1.21858367241051,2.20301376748668,108.059343649117));
#34912=CARTESIAN_POINT('Ctrl Pts',(1.18966024886055,2.21871027277269,108.061431425591));
#34913=CARTESIAN_POINT('Ctrl Pts',(1.17847866304134,2.22466960075153,108.06223226367));
#34914=CARTESIAN_POINT('Ctrl Pts',(1.15685145289476,2.23598720260113,108.063769362043));
#34915=CARTESIAN_POINT('Ctrl Pts',(1.14641242940057,2.24135731276086,108.064506022363));
#34916=CARTESIAN_POINT('Ctrl Pts',(1.12208247172748,2.25365883907981,108.066210957893));
#34917=CARTESIAN_POINT('Ctrl Pts',(1.10816413229903,2.26053522626595,108.067177304173));
#34918=CARTESIAN_POINT('Ctrl Pts',(1.06324954787257,2.28221085152783,108.070267736891));
#34919=CARTESIAN_POINT('Ctrl Pts',(1.0320129367722,2.29650504981211,108.072374537644));
#34920=CARTESIAN_POINT('Ctrl Pts',(0.957645544975907,2.32871240160955,108.077298755507));
#34921=CARTESIAN_POINT('Ctrl Pts',(0.914289070389287,2.34607380723462,108.080098387069));
#34922=CARTESIAN_POINT('Ctrl Pts',(0.659359741120222,2.44001469863309,108.096213240708));
#34923=CARTESIAN_POINT('Ctrl Pts',(0.438793948486696,2.48915137675487,108.10868681219));
#34924=CARTESIAN_POINT('Ctrl Pts',(0.151521070688895,2.51373468206869,108.125747685716));
#34925=CARTESIAN_POINT('Ctrl Pts',(0.0882162564628579,2.51675130863097,
108.129564269507));
#34926=CARTESIAN_POINT('Ctrl Pts',(0.0112339803149129,2.51751187393382,
108.134346057575));
#34927=CARTESIAN_POINT('Ctrl Pts',(-0.00240360133929631,2.51753578745429,
108.135198528975));
#34928=CARTESIAN_POINT('Ctrl Pts',(-0.0236905794401699,2.51740015390106,
108.136538466333));
#34929=CARTESIAN_POINT('Ctrl Pts',(-0.0313404288354343,2.51731653795564,
108.137021873519));
#34930=CARTESIAN_POINT('Ctrl Pts',(-0.0455117849561255,2.51709703344466,
108.137921059261));
#34931=CARTESIAN_POINT('Ctrl Pts',(-0.0520332607158115,2.51697066626515,
108.138336311306));
#34932=CARTESIAN_POINT('Ctrl Pts',(-0.0669700053182231,2.51662316076199,
108.139290713749));
#34933=CARTESIAN_POINT('Ctrl Pts',(-0.0753846782449455,2.51638515738663,
108.139830771532));
#34934=CARTESIAN_POINT('Ctrl Pts',(-0.101599905143106,2.51551206990412,
108.141520401152));
#34935=CARTESIAN_POINT('Ctrl Pts',(-0.119394575348378,2.51473028524736,
108.142677543281));
#34936=CARTESIAN_POINT('Ctrl Pts',(-0.161199968462996,2.5124489154723,108.145417803337));
#34937=CARTESIAN_POINT('Ctrl Pts',(-0.185200156337948,2.51079385758992,
108.1470078621));
#34938=CARTESIAN_POINT('Ctrl Pts',(-0.271473199747342,2.50360080182631,
108.152776066349));
#34939=CARTESIAN_POINT('Ctrl Pts',(-0.333555510673574,2.49608781873919,
108.1570249602));
#34940=CARTESIAN_POINT('Ctrl Pts',(-0.594944163996494,2.45452994704682,
108.175174886114));
#34941=CARTESIAN_POINT('Ctrl Pts',(-0.790083902045263,2.3988464338153,108.18929401947));
#34942=CARTESIAN_POINT('Ctrl Pts',(-1.03487448804734,2.29583460928733,108.206928798769));
#34943=CARTESIAN_POINT('Ctrl Pts',(-1.09233663048296,2.26905786766917,108.211070080065));
#34944=CARTESIAN_POINT('Ctrl Pts',(-1.16670129227178,2.23092406339511,108.216434544981));
#34945=CARTESIAN_POINT('Ctrl Pts',(-1.18456009379324,2.22149308012234,108.217723307061));
#34946=CARTESIAN_POINT('Ctrl Pts',(-1.21342769651984,2.20580139071252,108.219807774026));
#34947=CARTESIAN_POINT('Ctrl Pts',(-1.22450586771664,2.19967087069475,108.220608014776));
#34948=CARTESIAN_POINT('Ctrl Pts',(-1.24556470046214,2.18780878363184,108.222129994019));
#34949=CARTESIAN_POINT('Ctrl Pts',(-1.25555319814988,2.18209185655596,108.222852227994));
#34950=CARTESIAN_POINT('Ctrl Pts',(-1.27838095320674,2.16881772664195,108.224503796395));
#34951=CARTESIAN_POINT('Ctrl Pts',(-1.29119311329453,2.16121460112651,108.225431456564));
#34952=CARTESIAN_POINT('Ctrl Pts',(-1.31813272050178,2.14490274187768,108.227383968589));
#34953=CARTESIAN_POINT('Ctrl Pts',(-1.33224310921159,2.13616711870962,108.228407807582));
#34954=CARTESIAN_POINT('Ctrl Pts',(-1.36974994519367,2.11243075313723,108.231133290806));
#34955=CARTESIAN_POINT('Ctrl Pts',(-1.39298647640837,2.09718081348469,108.232826020154));
#34956=CARTESIAN_POINT('Ctrl Pts',(-1.46447572565446,2.0485504970995,108.238053027727));
#34957=CARTESIAN_POINT('Ctrl Pts',(-1.51181881173821,2.01386515197023,108.241541868679));
#34958=CARTESIAN_POINT('Ctrl Pts',(-1.73135137361525,1.84091839519729,108.25796442526));
#34959=CARTESIAN_POINT('Ctrl Pts',(-1.88604367990163,1.68207600870287,108.270198713614));
#34960=CARTESIAN_POINT('Ctrl Pts',(-2.04690585806332,1.46639557031896,108.28629234842));
#34961=CARTESIAN_POINT('Ctrl Pts',(-2.07466267311769,1.42685446636724,108.289228390637));
#34962=CARTESIAN_POINT('Ctrl Pts',(-2.1082589665769,1.37594030815489,108.29302426831));
#34963=CARTESIAN_POINT('Ctrl Pts',(-2.11517446530262,1.36528552593771,108.293819457996));
#34964=CARTESIAN_POINT('Ctrl Pts',(-2.12597137066416,1.34837169016418,108.295083839822));
#34965=CARTESIAN_POINT('Ctrl Pts',(-2.12990655673148,1.34214698897622,108.295549600311));
#34966=CARTESIAN_POINT('Ctrl Pts',(-2.13730464089937,1.33033017905094,108.296434791846));
#34967=CARTESIAN_POINT('Ctrl Pts',(-2.14077299234516,1.32474167466878,108.296853862742));
#34968=CARTESIAN_POINT('Ctrl Pts',(-2.14887966770191,1.31156453353929,108.297842948205));
#34969=CARTESIAN_POINT('Ctrl Pts',(-2.15349971822447,1.30396484224259,108.298414118023));
#34970=CARTESIAN_POINT('Ctrl Pts',(-2.16859273918081,1.27883878576177,108.300304510656));
#34971=CARTESIAN_POINT('Ctrl Pts',(-2.17889246462463,1.26121000363504,108.301634011481));
#34972=CARTESIAN_POINT('Ctrl Pts',(-2.23561321498277,1.16135917054091,108.309173865764));
#34973=CARTESIAN_POINT('Ctrl Pts',(-2.27759005986772,1.07670868388783,108.31559905276));
#34974=CARTESIAN_POINT('Ctrl Pts',(-2.33127140486613,0.951185466908145,
108.324987841862));
#34975=CARTESIAN_POINT('Ctrl Pts',(-2.34684876526915,0.912072925269062,
108.327895159897));
#34976=CARTESIAN_POINT('Ctrl Pts',(-2.36143103931297,0.872610850591077,
108.330801621721));
#34977=CARTESIAN_POINT('Origin',(0.,0.,104.));
#34978=CARTESIAN_POINT('',(-2.36143112100138,0.872610629528524,109.333394523839));
#34979=CARTESIAN_POINT('',(-2.36143112101026,0.8726106295045,109.056156733688));
#34980=CARTESIAN_POINT('',(-2.36143112101026,0.872610629504505,104.));
#34981=CARTESIAN_POINT('',(-2.5174990352485,-0.00220397887332777,108.112583302432));
#34982=CARTESIAN_POINT('Ctrl Pts',(-2.36143112101026,0.8726106295045,109.056156733688));
#34983=CARTESIAN_POINT('Ctrl Pts',(-2.33268216378951,0.950410142806583,
109.050916676707));
#34984=CARTESIAN_POINT('Ctrl Pts',(-2.30005751129571,1.02686009642425,109.045676619726));
#34985=CARTESIAN_POINT('Ctrl Pts',(-2.26371131250978,1.10155224279888,109.040436562745));
#34986=CARTESIAN_POINT('Ctrl Pts',(-2.22738312760807,1.17620737029062,109.035199102838));
#34987=CARTESIAN_POINT('Ctrl Pts',(-2.18733726025505,1.24910600616275,109.029961642932));
#34988=CARTESIAN_POINT('Ctrl Pts',(-2.14377559608639,1.31986076675703,109.024724183025));
#34989=CARTESIAN_POINT('Ctrl Pts',(-2.10022238166327,1.39060180290497,109.01948773904));
#34990=CARTESIAN_POINT('Ctrl Pts',(-2.05315496725343,1.45919939721905,109.014251295054));
#34991=CARTESIAN_POINT('Ctrl Pts',(-2.00282001409352,1.52529283783359,109.009014851069));
#34992=CARTESIAN_POINT('Ctrl Pts',(-1.95247964142512,1.59139339465545,109.003777843281));
#34993=CARTESIAN_POINT('Ctrl Pts',(-1.89887131212628,1.65498889619735,108.998540835493));
#34994=CARTESIAN_POINT('Ctrl Pts',(-1.84228278095399,1.71575068264606,108.993303827705));
#34995=CARTESIAN_POINT('Ctrl Pts',(-1.78563437319289,1.77657676142447,108.988061278615));
#34996=CARTESIAN_POINT('Ctrl Pts',(-1.72599978335873,1.83456280099905,108.982818729525));
#34997=CARTESIAN_POINT('Ctrl Pts',(-1.66370416107772,1.88941650104276,108.977576180435));
#34998=CARTESIAN_POINT('Ctrl Pts',(-1.6013728793718,1.94430160058657,108.972330630391));
#34999=CARTESIAN_POINT('Ctrl Pts',(-1.53637789353067,1.99605050335782,108.967085080347));
#35000=CARTESIAN_POINT('Ctrl Pts',(-1.4690761065609,2.04441229773543,108.961839530303));
#35001=CARTESIAN_POINT('Ctrl Pts',(-1.4016609880652,2.09285553000942,108.956585147118));
#35002=CARTESIAN_POINT('Ctrl Pts',(-1.33193169961201,2.13790001469722,108.951330763933));
#35003=CARTESIAN_POINT('Ctrl Pts',(-1.26027236462642,2.17933930744135,108.946076380748));
#35004=CARTESIAN_POINT('Ctrl Pts',(-1.21657392417061,2.20460932239298,108.942872215501));
#35005=CARTESIAN_POINT('Ctrl Pts',(-1.17215823529164,2.22853959777458,108.939668050255));
#35006=CARTESIAN_POINT('Ctrl Pts',(-1.12711601958332,2.25109211903881,108.936463885008));
#35007=CARTESIAN_POINT('Ctrl Pts',(-1.05324090416649,2.28808119884174,108.931208635601));
#35008=CARTESIAN_POINT('Ctrl Pts',(-0.977406600329775,2.32149814501377,
108.925953386194));
#35009=CARTESIAN_POINT('Ctrl Pts',(-0.899992693089532,2.3511315153316,108.920698136786));
#35010=CARTESIAN_POINT('Ctrl Pts',(-0.822688541183468,2.38072287226219,
108.915450338129));
#35011=CARTESIAN_POINT('Ctrl Pts',(-0.743809661544561,2.40654114472751,
108.910202539471));
#35012=CARTESIAN_POINT('Ctrl Pts',(-0.663759045355638,2.42842133488169,
108.904954740814));
#35013=CARTESIAN_POINT('Ctrl Pts',(-0.583128393440582,2.45046006587651,
108.899668917331));
#35014=CARTESIAN_POINT('Ctrl Pts',(-0.501309376583863,2.46850319198874,
108.894383093848));
#35015=CARTESIAN_POINT('Ctrl Pts',(-0.418733125877407,2.48243203719516,
108.889097270365));
#35016=CARTESIAN_POINT('Ctrl Pts',(-0.336897330711175,2.49623598340806,
108.883858844496));
#35017=CARTESIAN_POINT('Ctrl Pts',(-0.254318290808967,2.505999059978,108.878620418628));
#35018=CARTESIAN_POINT('Ctrl Pts',(-0.171427855907963,2.51165657290538,
108.873381992759));
#35019=CARTESIAN_POINT('Ctrl Pts',(-0.0885646822915049,2.51731222517092,
108.868145289722));
#35020=CARTESIAN_POINT('Ctrl Pts',(-0.00539077705992319,2.51886496407218,
108.862908586684));
#35021=CARTESIAN_POINT('Ctrl Pts',(0.0776570934187217,2.51630197429517,
108.857671883646));
#35022=CARTESIAN_POINT('Ctrl Pts',(0.160702701714922,2.51373905433272,108.852435323254));
#35023=CARTESIAN_POINT('Ctrl Pts',(0.243621820914811,2.50706064386026,108.847198762862));
#35024=CARTESIAN_POINT('Ctrl Pts',(0.325979284034066,2.4963060221817,108.841962202469));
#35025=CARTESIAN_POINT('Ctrl Pts',(0.40968471682491,2.48537537633602,108.836639933699));
#35026=CARTESIAN_POINT('Ctrl Pts',(0.492809452780374,2.47023393290518,108.831317664928));
#35027=CARTESIAN_POINT('Ctrl Pts',(0.574905573004285,2.45097732183075,108.825995396157));
#35028=CARTESIAN_POINT('Ctrl Pts',(0.655795641189291,2.4320036044544,108.820751315407));
#35029=CARTESIAN_POINT('Ctrl Pts',(0.735686682421675,2.40903501479311,108.815507234657));
#35030=CARTESIAN_POINT('Ctrl Pts',(0.814165640056965,2.38221337426995,108.810263153906));
#35031=CARTESIAN_POINT('Ctrl Pts',(0.894399752107213,2.35479187714574,108.804901791126));
#35032=CARTESIAN_POINT('Ctrl Pts',(0.973157381352583,2.32334309510195,108.799540428345));
#35033=CARTESIAN_POINT('Ctrl Pts',(1.05002065499409,2.28806968296112,108.794179065564));
#35034=CARTESIAN_POINT('Ctrl Pts',(1.12688392863559,2.25279627082028,108.788817702784));
#35035=CARTESIAN_POINT('Ctrl Pts',(1.2018524270417,2.2136985227658,108.783456340003));
#35036=CARTESIAN_POINT('Ctrl Pts',(1.27453862635215,2.17102683998526,108.778094977223));
#35037=CARTESIAN_POINT('Ctrl Pts',(1.34578620303758,2.12919972534665,108.772839727815));
#35038=CARTESIAN_POINT('Ctrl Pts',(1.41510418478533,2.08378440484462,108.767584478408));
#35039=CARTESIAN_POINT('Ctrl Pts',(1.48210854983503,2.03498415141394,108.762329229001));
#35040=CARTESIAN_POINT('Ctrl Pts',(1.54901791791665,1.98625308565653,108.757081430343));
#35041=CARTESIAN_POINT('Ctrl Pts',(1.6136198148298,1.9341468886985,108.751833631686));
#35042=CARTESIAN_POINT('Ctrl Pts',(1.67555643247572,1.87891375310024,108.746585833028));
#35043=CARTESIAN_POINT('Ctrl Pts',(1.73794183431208,1.82328040581805,108.741300009545));
#35044=CARTESIAN_POINT('Ctrl Pts',(1.79762276074586,1.76447485387521,108.736014186062));
#35045=CARTESIAN_POINT('Ctrl Pts',(1.85426493724833,1.70279411335941,108.730728362579));
#35046=CARTESIAN_POINT('Ctrl Pts',(1.91039920726393,1.64166645978618,108.725489936711));
#35047=CARTESIAN_POINT('Ctrl Pts',(1.96354868775432,1.57771532047734,108.720251510842));
#35048=CARTESIAN_POINT('Ctrl Pts',(2.01342399262818,1.51126770491174,108.715013084974));
#35049=CARTESIAN_POINT('Ctrl Pts',(2.06328289434433,1.44484194286104,108.709776381936));
#35050=CARTESIAN_POINT('Ctrl Pts',(2.10986948229665,1.37592170394282,108.704539678899));
#35051=CARTESIAN_POINT('Ctrl Pts',(2.15293520896774,1.30486636709934,108.699302975861));
#35052=CARTESIAN_POINT('Ctrl Pts',(2.19599976254997,1.2338129657677,108.694066415469));
#35053=CARTESIAN_POINT('Ctrl Pts',(2.23554340725672,1.1606249772816,108.688829855077));
#35054=CARTESIAN_POINT('Ctrl Pts',(2.27136216292113,1.08568880202857,108.683593294684));
#35055=CARTESIAN_POINT('Ctrl Pts',(2.307767175064,1.00952612358196,108.678271025914));
#35056=CARTESIAN_POINT('Ctrl Pts',(2.34032404137947,0.93155795384246,108.672948757144));
#35057=CARTESIAN_POINT('Ctrl Pts',(2.36886910538251,0.852212069595514,108.667626488373));
#35058=CARTESIAN_POINT('Ctrl Pts',(2.39699482152184,0.774031834409633,108.662382407623));
#35059=CARTESIAN_POINT('Ctrl Pts',(2.4212257478244,0.694514560872618,108.657138326873));
#35060=CARTESIAN_POINT('Ctrl Pts',(2.44145595367082,0.614083932606366,108.651894246122));
#35061=CARTESIAN_POINT('Ctrl Pts',(2.46213860098907,0.531854501495064,108.646532883342));
#35062=CARTESIAN_POINT('Ctrl Pts',(2.4786393194186,0.448670871208492,108.641171520561));
#35063=CARTESIAN_POINT('Ctrl Pts',(2.49090058276339,0.364993885961109,108.635810157781));
#35064=CARTESIAN_POINT('Ctrl Pts',(2.50316184610818,0.281316900713732,108.630448795));
#35065=CARTESIAN_POINT('Ctrl Pts',(2.51118367265796,0.197147072657835,108.62508743222));
#35066=CARTESIAN_POINT('Ctrl Pts',(2.5149651090264,0.112945785135207,108.619726069439));
#35067=CARTESIAN_POINT('Ctrl Pts',(2.51867170230268,0.0304110296148989,
108.614470820032));
#35068=CARTESIAN_POINT('Ctrl Pts',(2.5183179652071,-0.0524588008418233,
108.609215570625));
#35069=CARTESIAN_POINT('Ctrl Pts',(2.51386532026221,-0.135230919478382,
108.603960321217));
#35070=CARTESIAN_POINT('Ctrl Pts',(2.50941898815634,-0.217885686054263,
108.59871252256));
#35071=CARTESIAN_POINT('Ctrl Pts',(2.50088531575818,-0.300442559066649,
108.593464723902));
#35072=CARTESIAN_POINT('Ctrl Pts',(2.48827767589473,-0.382466283015776,
108.588216925245));
#35073=CARTESIAN_POINT('Ctrl Pts',(2.4755786828114,-0.465084339557793,108.582931101762));
#35074=CARTESIAN_POINT('Ctrl Pts',(2.45874641307694,-0.547161014776089,
108.577645278279));
#35075=CARTESIAN_POINT('Ctrl Pts',(2.43784800520533,-0.628254210902234,
108.572359454796));
#35076=CARTESIAN_POINT('Ctrl Pts',(2.4171369919146,-0.70862024993616,108.567121028928));
#35077=CARTESIAN_POINT('Ctrl Pts',(2.39243258725514,-0.788019921759766,
108.561882603059));
#35078=CARTESIAN_POINT('Ctrl Pts',(2.36385152754585,-0.866032450731004,
108.55664417719));
#35079=CARTESIAN_POINT('Ctrl Pts',(2.33527986767144,-0.944019322679784,
108.551407474153));
#35080=CARTESIAN_POINT('Ctrl Pts',(2.30283424350808,-1.02061952491328,108.546170771115));
#35081=CARTESIAN_POINT('Ctrl Pts',(2.26668077725614,-1.09542891326526,108.540934068078));
#35082=CARTESIAN_POINT('Ctrl Pts',(2.23052829580655,-1.1702362638469,108.535697507686));
#35083=CARTESIAN_POINT('Ctrl Pts',(2.19066837478622,-1.24325248253537,108.530460947293));
#35084=CARTESIAN_POINT('Ctrl Pts',(2.14731406653896,-1.31409609604623,108.525224386901));
#35085=CARTESIAN_POINT('Ctrl Pts',(2.10325016512985,-1.38609922854699,108.51990211813));
#35086=CARTESIAN_POINT('Ctrl Pts',(2.05557670255045,-1.45585756856834,108.51457984936));
#35087=CARTESIAN_POINT('Ctrl Pts',(2.00456339163943,-1.52300093857457,108.509257580589));
#35088=CARTESIAN_POINT('Ctrl Pts',(1.95429950356922,-1.58915792337676,108.504013499839));
#35089=CARTESIAN_POINT('Ctrl Pts',(1.90079359363855,-1.65277594112891,108.498769419089));
#35090=CARTESIAN_POINT('Ctrl Pts',(1.84434337030973,-1.7135354628354,108.493525338338));
#35091=CARTESIAN_POINT('Ctrl Pts',(1.78663065749725,-1.77565384997527,108.488163975558));
#35092=CARTESIAN_POINT('Ctrl Pts',(1.72584071206637,-1.8347839826566,108.482802612777));
#35093=CARTESIAN_POINT('Ctrl Pts',(1.66232876636165,-1.89062670099799,108.477441249997));
#35094=CARTESIAN_POINT('Ctrl Pts',(1.59881682065693,-1.94646941933939,108.472079887216));
#35095=CARTESIAN_POINT('Ctrl Pts',(1.53258331422562,-1.99902445984004,108.466718524435));
#35096=CARTESIAN_POINT('Ctrl Pts',(1.46401473278267,-2.04803982192615,108.461357161655));
#35097=CARTESIAN_POINT('Ctrl Pts',(1.39680327708815,-2.0960850602536,108.456101912248));
#35098=CARTESIAN_POINT('Ctrl Pts',(1.32710010991272,-2.14090695686203,108.45084666284));
#35099=CARTESIAN_POINT('Ctrl Pts',(1.2552472458811,-2.18223752183577,108.445591413433));
#35100=CARTESIAN_POINT('Ctrl Pts',(1.18349625288767,-2.22350948945755,108.440343614775));
#35101=CARTESIAN_POINT('Ctrl Pts',(1.10960201345743,-2.26129972927178,108.435095816118));
#35102=CARTESIAN_POINT('Ctrl Pts',(1.03393689740221,-2.29538248276628,108.42984801746));
#35103=CARTESIAN_POINT('Ctrl Pts',(0.957723522350116,-2.32971219519266,
108.424562193978));
#35104=CARTESIAN_POINT('Ctrl Pts',(0.879713884850795,-2.36028019114474,
108.419276370495));
#35105=CARTESIAN_POINT('Ctrl Pts',(0.800315366770437,-2.38690208506991,
108.413990547012));
#35106=CARTESIAN_POINT('Ctrl Pts',(0.721628809721186,-2.41328526230985,
108.408752121143));
#35107=CARTESIAN_POINT('Ctrl Pts',(0.641578625868065,-2.43579267354179,
108.403513695275));
#35108=CARTESIAN_POINT('Ctrl Pts',(0.560581315844466,-2.45429314433425,
108.398275269406));
#35109=CARTESIAN_POINT('Ctrl Pts',(0.47961064448814,-2.47278753062976,108.393038566369));
#35110=CARTESIAN_POINT('Ctrl Pts',(0.397693915086567,-2.48727749107548,
108.387801863331));
#35111=CARTESIAN_POINT('Ctrl Pts',(0.315260566139785,-2.49768233076931,
108.382565160294));
#35112=CARTESIAN_POINT('Ctrl Pts',(0.232829462636183,-2.50808688704051,
108.377328599901));
#35113=CARTESIAN_POINT('Ctrl Pts',(0.149882225484559,-2.51440648704673,
108.372092039509));
#35114=CARTESIAN_POINT('Ctrl Pts',(0.0668548282140929,-2.51661214372506,
108.366855479117));
#35115=CARTESIAN_POINT('Ctrl Pts',(-0.0175315037441317,-2.51885390105774,
108.361533210346));
#35116=CARTESIAN_POINT('Ctrl Pts',(-0.102000152302608,-2.51684580555824,
108.356210941576));
#35117=CARTESIAN_POINT('Ctrl Pts',(-0.186093769824212,-2.51061254653772,
108.350888672805));
#35118=CARTESIAN_POINT('Ctrl Pts',(-0.268951990610984,-2.50447085865027,
108.345644592055));
#35119=CARTESIAN_POINT('Ctrl Pts',(-0.351445669286695,-2.49422744326405,
108.340400511305));
#35120=CARTESIAN_POINT('Ctrl Pts',(-0.433144699557888,-2.47995804788003,
108.335156430554));
#35121=CARTESIAN_POINT('Ctrl Pts',(-0.516670900041242,-2.46536952246344,
108.329795067774));
#35122=CARTESIAN_POINT('Ctrl Pts',(-0.599365979841367,-2.44657287826211,
108.324433704993));
#35123=CARTESIAN_POINT('Ctrl Pts',(-0.680785599153208,-2.42370320336167,
108.319072342213));
#35124=CARTESIAN_POINT('Ctrl Pts',(-0.762205218465049,-2.40083352846123,
108.313710979432));
#35125=CARTESIAN_POINT('Ctrl Pts',(-0.842348916953951,-2.37389104808709,
108.308349616652));
#35126=CARTESIAN_POINT('Ctrl Pts',(-0.920794895731956,-2.3430627413695,
108.302988253871));
#35127=CARTESIAN_POINT('Ctrl Pts',(-0.997688252953404,-2.31284459586487,
108.297733004464));
#35128=CARTESIAN_POINT('Ctrl Pts',(-1.07323451221387,-2.27878146856245,
108.292477755056));
#35129=CARTESIAN_POINT('Ctrl Pts',(-1.14702267524325,-2.24101433116297,
108.287222505649));
#35130=CARTESIAN_POINT('Ctrl Pts',(-1.22070622342013,-2.20330073898465,
108.281974706992));
#35131=CARTESIAN_POINT('Ctrl Pts',(-1.29263621904113,-2.16189377608995,
108.276726908334));
#35132=CARTESIAN_POINT('Ctrl Pts',(-1.3624205602826,-2.1169828688299,108.271479109677));
#35133=CARTESIAN_POINT('Ctrl Pts',(-1.43271054923752,-2.07174654332899,
108.266193286194));
#35134=CARTESIAN_POINT('Ctrl Pts',(-1.50082321732818,-2.02295545433858,
108.260907462711));
#35135=CARTESIAN_POINT('Ctrl Pts',(-1.56638210368257,-1.97085092162319,
108.255621639228));
#35136=CARTESIAN_POINT('Ctrl Pts',(-1.63135312802827,-1.9192136066561,108.250383213359));
#35137=CARTESIAN_POINT('Ctrl Pts',(-1.69381561848933,-1.86432232519278,
108.245144787491));
#35138=CARTESIAN_POINT('Ctrl Pts',(-1.75343278254459,-1.8064550166273,108.239906361622));
#35139=CARTESIAN_POINT('Ctrl Pts',(-1.81303033950678,-1.74860673965654,
108.234669658585));
#35140=CARTESIAN_POINT('Ctrl Pts',(-1.86978409773914,-1.68778470059112,
108.229432955547));
#35141=CARTESIAN_POINT('Ctrl Pts',(-1.92339256251863,-1.6243051746664,108.22419625251));
#35142=CARTESIAN_POINT('Ctrl Pts',(-1.97699956703033,-1.56082737789222,
108.218959692117));
#35143=CARTESIAN_POINT('Ctrl Pts',(-2.02746115151203,-1.49469259138072,
108.213723131725));
#35144=CARTESIAN_POINT('Ctrl Pts',(-2.07451563537045,-1.42625072431307,
108.208486571333));
#35145=CARTESIAN_POINT('Ctrl Pts',(-2.1223402742913,-1.35668864837088,108.203164302562));
#35146=CARTESIAN_POINT('Ctrl Pts',(-2.16664498684489,-1.28474368689081,
108.197842033792));
#35147=CARTESIAN_POINT('Ctrl Pts',(-2.20720147859993,-1.2108129016765,108.192519765021));
#35148=CARTESIAN_POINT('Ctrl Pts',(-2.2471621658342,-1.13796821375881,108.187275684271));
#35149=CARTESIAN_POINT('Ctrl Pts',(-2.28348388016513,-1.06319610901183,
108.18203160352));
#35150=CARTESIAN_POINT('Ctrl Pts',(-2.31599598596929,-0.986898598121488,
108.17678752277));
#35151=CARTESIAN_POINT('Ctrl Pts',(-2.34923521363841,-0.908894720109143,
108.171426159989));
#35152=CARTESIAN_POINT('Ctrl Pts',(-2.37849219878238,-0.829296862872565,
108.166064797209));
#35153=CARTESIAN_POINT('Ctrl Pts',(-2.40363833074474,-0.748551284131325,
108.160703434428));
#35154=CARTESIAN_POINT('Ctrl Pts',(-2.42878446270709,-0.667805705390085,
108.155342071648));
#35155=CARTESIAN_POINT('Ctrl Pts',(-2.44981967977525,-0.585912913893669,
108.149980708867));
#35156=CARTESIAN_POINT('Ctrl Pts',(-2.46667116953818,-0.503328512374544,
108.144619346087));
#35157=CARTESIAN_POINT('Ctrl Pts',(-2.4901232042434,-0.388396700541625,
108.137157995917));
#35158=CARTESIAN_POINT('Ctrl Pts',(-2.50554871649174,-0.271776010995007,
108.129696645748));
#35159=CARTESIAN_POINT('Ctrl Pts',(-2.51276111767346,-0.154394998327111,
108.122235295578));
#35160=CARTESIAN_POINT('Ctrl Pts',(-2.51587110200439,-0.103780355443597,
108.11901796455));
#35161=CARTESIAN_POINT('Ctrl Pts',(-2.5174545435931,-0.0530246346749353,
108.115800633521));
#35162=CARTESIAN_POINT('Ctrl Pts',(-2.51749903524768,-0.00220397981460282,
108.112583302492));
#35163=CARTESIAN_POINT('Ctrl Pts',(-2.5174990352485,-0.00220397887333112,
108.112583302432));
#35164=CARTESIAN_POINT('Ctrl Pts',(-2.51757053067579,0.0794618081286696,
108.107413241731));
#35165=CARTESIAN_POINT('Ctrl Pts',(-2.51366404211222,0.161254080773151,
108.10224318103));
#35166=CARTESIAN_POINT('Ctrl Pts',(-2.50576929896393,0.242747750493866,
108.097073120328));
#35167=CARTESIAN_POINT('Ctrl Pts',(-2.49788117529288,0.3241730905068,108.091907394549));
#35168=CARTESIAN_POINT('Ctrl Pts',(-2.48601147691956,0.405299852895239,
108.08674166877));
#35169=CARTESIAN_POINT('Ctrl Pts',(-2.47020197011635,0.48570410419649,108.081575942991));
#35170=CARTESIAN_POINT('Ctrl Pts',(-2.45439918980559,0.56607414579113,108.076412415081));
#35171=CARTESIAN_POINT('Ctrl Pts',(-2.43466001448788,0.645721819316943,
108.07124888717));
#35172=CARTESIAN_POINT('Ctrl Pts',(-2.41107772898596,0.724230926423269,
108.06608535926));
#35173=CARTESIAN_POINT('Ctrl Pts',(-2.39607226998297,0.77418644019011,108.062799795341));
#35174=CARTESIAN_POINT('Ctrl Pts',(-2.3795118491617,0.823681138270154,108.059514231422));
#35175=CARTESIAN_POINT('Ctrl Pts',(-2.36143112101026,0.8726106295045,108.056228667503));
#35176=CARTESIAN_POINT('',(-2.51749991139346,-0.000667932580992832,108.389610494019));
#35177=CARTESIAN_POINT('Ctrl Pts',(-2.36143103931297,0.872610850591077,
108.330801621721));
#35178=CARTESIAN_POINT('Ctrl Pts',(-2.41699789040957,0.722237649469957,
108.341876912921));
#35179=CARTESIAN_POINT('Ctrl Pts',(-2.45811556380063,0.566786644106253,
108.35290722707));
#35180=CARTESIAN_POINT('Ctrl Pts',(-2.49286589157802,0.355398459208296,
108.367046773783));
#35181=CARTESIAN_POINT('Ctrl Pts',(-2.49987821345447,0.302155671775727,
108.370540950515));
#35182=CARTESIAN_POINT('Ctrl Pts',(-2.50705947385862,0.229825560448704,
108.375200002371));
#35183=CARTESIAN_POINT('Ctrl Pts',(-2.50872207453657,0.210904193218192,
108.376410764129));
#35184=CARTESIAN_POINT('Ctrl Pts',(-2.51111609185144,0.179599636397731,
108.378401073442));
#35185=CARTESIAN_POINT('Ctrl Pts',(-2.5119703885151,0.167226888682806,108.379184411809));
#35186=CARTESIAN_POINT('Ctrl Pts',(-2.51341356707306,0.143808315729925,
108.380660998116));
#35187=CARTESIAN_POINT('Ctrl Pts',(-2.51402114612365,0.132763978260241,
108.381354809862));
#35188=CARTESIAN_POINT('Ctrl Pts',(-2.51511445898997,0.110176975016777,
108.382768670918));
#35189=CARTESIAN_POINT('Ctrl Pts',(-2.51559356833387,0.0986342416272372,
108.383488499357));
#35190=CARTESIAN_POINT('Ctrl Pts',(-2.5164777214697,0.0730909819278779,
108.385075666263));
#35191=CARTESIAN_POINT('Ctrl Pts',(-2.51684541818914,0.0590894867524746,
108.385941840848));
#35192=CARTESIAN_POINT('Ctrl Pts',(-2.5173693966288,0.0298360417485043,
108.387743962294));
#35193=CARTESIAN_POINT('Ctrl Pts',(-2.5175039580511,0.0145842957774581,
108.388679221811));
#35194=CARTESIAN_POINT('Ctrl Pts',(-2.51749991139346,-0.000667932580992832,
108.389610494019));
#35195=CARTESIAN_POINT('Ctrl Pts',(-2.51749991190576,-0.000665998854557162,
108.389610375949));
#35196=CARTESIAN_POINT('Ctrl Pts',(-2.51746333858691,-0.138914475365931,
108.398051569454));
#35197=CARTESIAN_POINT('Ctrl Pts',(-2.50603947464677,-0.276938265112995,
108.406130853442));
#35198=CARTESIAN_POINT('Ctrl Pts',(-2.46726158300713,-0.509911691712988,
108.419750920604));
#35199=CARTESIAN_POINT('Ctrl Pts',(-2.44556977785967,-0.605456467028899,
108.425337009676));
#35200=CARTESIAN_POINT('Ctrl Pts',(-2.39826491729595,-0.769004275891744,
108.435212037579));
#35201=CARTESIAN_POINT('Ctrl Pts',(-2.37517335532977,-0.837611053587795,
108.439455650568));
#35202=CARTESIAN_POINT('Ctrl Pts',(-2.33499235898631,-0.941897032090542,
108.446194928368));
#35203=CARTESIAN_POINT('Ctrl Pts',(-2.31996281270867,-0.978330971549724,
108.448605911819));
#35204=CARTESIAN_POINT('Ctrl Pts',(-2.29948862147339,-1.02483582835349,
108.451775331619));
#35205=CARTESIAN_POINT('Ctrl Pts',(-2.29482104528161,-1.03524526269562,
108.452490803074));
#35206=CARTESIAN_POINT('Ctrl Pts',(-2.28714303859006,-1.05206134544333,
108.453657011255));
#35207=CARTESIAN_POINT('Ctrl Pts',(-2.28417599065181,-1.05848778657624,
108.454105165809));
#35208=CARTESIAN_POINT('Ctrl Pts',(-2.27838309933927,-1.07089704557172,
108.454975499619));
#35209=CARTESIAN_POINT('Ctrl Pts',(-2.2755607178232,-1.07688135150353,108.455397470688));
#35210=CARTESIAN_POINT('Ctrl Pts',(-2.26925827442145,-1.09010903689316,
108.456335098059));
#35211=CARTESIAN_POINT('Ctrl Pts',(-2.26576705434302,-1.09734701877104,
108.456851423583));
#35212=CARTESIAN_POINT('Ctrl Pts',(-2.2532166134995,-1.12305129815746,108.458696394838));
#35213=CARTESIAN_POINT('Ctrl Pts',(-2.24396608378319,-1.14142256697539,
108.460035947309));
#35214=CARTESIAN_POINT('Ctrl Pts',(-2.15687780182908,-1.30922613306967,
108.472451063908));
#35215=CARTESIAN_POINT('Ctrl Pts',(-2.06445305756935,-1.45059306180974,
108.48419898562));
#35216=CARTESIAN_POINT('Ctrl Pts',(-1.86535522708747,-1.69714152118424,
108.506048822544));
#35217=CARTESIAN_POINT('Ctrl Pts',(-1.76205530324812,-1.80416536657462,
108.516140092782));
#35218=CARTESIAN_POINT('Ctrl Pts',(-1.62955327403261,-1.91913751840924,
108.527597786545));
#35219=CARTESIAN_POINT('Ctrl Pts',(-1.60891302327847,-1.93647402825981,
108.529345254292));
#35220=CARTESIAN_POINT('Ctrl Pts',(-1.57538320841784,-1.96373070313886,
108.532125507894));
#35221=CARTESIAN_POINT('Ctrl Pts',(-1.56266947363193,-1.97386287878403,
108.533166627106));
#35222=CARTESIAN_POINT('Ctrl Pts',(-1.53867115513765,-1.99261106568585,
108.535107762159));
#35223=CARTESIAN_POINT('Ctrl Pts',(-1.52741016601901,-2.00125610078862,
108.536008898644));
#35224=CARTESIAN_POINT('Ctrl Pts',(-1.51592641023422,-2.00991875559233,
108.536918196063));
#35225=CARTESIAN_POINT('Ctrl Pts',(-1.5157763459574,-2.01003192869255,108.536930076669));
#35226=CARTESIAN_POINT('Ctrl Pts',(-1.51546785880682,-2.01026452445519,
108.536954496221));
#35227=CARTESIAN_POINT('Ctrl Pts',(-1.51530943447976,-2.01038394520456,
108.536967035091));
#35228=CARTESIAN_POINT('Ctrl Pts',(-1.51498324303016,-2.01062976886877,
108.536992848482));
#35229=CARTESIAN_POINT('Ctrl Pts',(-1.51481547419925,-2.01075616951684,
108.537006122914));
#35230=CARTESIAN_POINT('Ctrl Pts',(-1.51446944965376,-2.01101680397236,
108.537033497261));
#35231=CARTESIAN_POINT('Ctrl Pts',(-1.5142911918994,-2.01115103508656,108.537047597072));
#35232=CARTESIAN_POINT('Ctrl Pts',(-1.51392285031801,-2.011428325813,108.537076727281));
#35233=CARTESIAN_POINT('Ctrl Pts',(-1.5137327640548,-2.01157138218482,108.537091757552));
#35234=CARTESIAN_POINT('Ctrl Pts',(-1.51333918605269,-2.01186749633094,
108.537122872578));
#35235=CARTESIAN_POINT('Ctrl Pts',(-1.51313569135498,-2.01202055018911,
108.53713895718));
#35236=CARTESIAN_POINT('Ctrl Pts',(-1.51271341830748,-2.01233805285787,
108.537172328122));
#35237=CARTESIAN_POINT('Ctrl Pts',(-1.5124946363424,-2.01250249687868,108.537189614276));
#35238=CARTESIAN_POINT('Ctrl Pts',(-1.51203953482206,-2.01284445064483,
108.537225564941));
#35239=CARTESIAN_POINT('Ctrl Pts',(-1.51180321080559,-2.01302195446414,
108.537244229221));
#35240=CARTESIAN_POINT('Ctrl Pts',(-1.51131029278324,-2.01339205120609,
108.537283150117));
#35241=CARTESIAN_POINT('Ctrl Pts',(-1.51105369319284,-2.01358463671654,
108.537303406445));
#35242=CARTESIAN_POINT('Ctrl Pts',(-1.51051687384625,-2.01398737496365,
108.537345773628));
#35243=CARTESIAN_POINT('Ctrl Pts',(-1.51023664701592,-2.01419751829296,
108.537367884117));
#35244=CARTESIAN_POINT('Ctrl Pts',(-1.50964841276359,-2.01463844596748,
108.537414284993));
#35245=CARTESIAN_POINT('Ctrl Pts',(-1.50934039623226,-2.01486921819546,
108.537438574908));
#35246=CARTESIAN_POINT('Ctrl Pts',(-1.50017571663267,-2.02173230108417,
108.538161087501));
#35247=CARTESIAN_POINT('Ctrl Pts',(-1.49127536609841,-2.02830630497187,
108.538857036846));
#35248=CARTESIAN_POINT('Ctrl Pts',(-1.47144444523328,-2.04275278370774,
108.540395212104));
#35249=CARTESIAN_POINT('Ctrl Pts',(-1.46049339993789,-2.05059667674585,
108.54123632755));
#35250=CARTESIAN_POINT('Ctrl Pts',(-1.43043967229383,-2.07176033625264,
108.543522555112));
#35251=CARTESIAN_POINT('Ctrl Pts',(-1.41121399978581,-2.0849037506754,108.544960994706));
#35252=CARTESIAN_POINT('Ctrl Pts',(-1.30596207449112,-2.15473498859743,
108.552711416484));
#35253=CARTESIAN_POINT('Ctrl Pts',(-1.21669521133149,-2.20637172091286,
108.558834577188));
#35254=CARTESIAN_POINT('Ctrl Pts',(-0.998250752172163,-2.3154298165149,
108.573084285152));
#35255=CARTESIAN_POINT('Ctrl Pts',(-0.866921960984713,-2.36773428392264,
108.581082679637));
#35256=CARTESIAN_POINT('Ctrl Pts',(-0.662212604872423,-2.42993537835929,
108.593489635586));
#35257=CARTESIAN_POINT('Ctrl Pts',(-0.591640190933045,-2.44807514075426,
108.597759977346));
#35258=CARTESIAN_POINT('Ctrl Pts',(-0.481663310697931,-2.47130999478101,
108.604537157694));
#35259=CARTESIAN_POINT('Ctrl Pts',(-0.442755389331779,-2.47857618449848,
108.606958169524));
#35260=CARTESIAN_POINT('Ctrl Pts',(-0.392417861308584,-2.48675390836866,
108.610139034492));
#35261=CARTESIAN_POINT('Ctrl Pts',(-0.381128703346094,-2.48850912767786,
108.61085554078));
#35262=CARTESIAN_POINT('Ctrl Pts',(-0.362822979665856,-2.49122778796279,
108.612023022286));
#35263=CARTESIAN_POINT('Ctrl Pts',(-0.355813461566265,-2.4922385888413,
108.612471404918));
#35264=CARTESIAN_POINT('Ctrl Pts',(-0.34224904229243,-2.49413624254058,
108.613341836605));
#35265=CARTESIAN_POINT('Ctrl Pts',(-0.335694785065585,-2.49502685571191,
108.61376367491));
#35266=CARTESIAN_POINT('Ctrl Pts',(-0.321178115962958,-2.49694119209988,
108.614700645817));
#35267=CARTESIAN_POINT('Ctrl Pts',(-0.313214164012915,-2.49795267814626,
108.615216444332));
#35268=CARTESIAN_POINT('Ctrl Pts',(-0.284879494293792,-2.50141377874519,
108.617057548712));
#35269=CARTESIAN_POINT('Ctrl Pts',(-0.264484455369829,-2.50365235765994,
108.618393703052));
#35270=CARTESIAN_POINT('Ctrl Pts',(-0.0755845507974478,-2.52205238877293,
108.630856500826));
#35271=CARTESIAN_POINT('Ctrl Pts',(0.0941080406935608,-2.5214275092692,
108.642661974447));
#35272=CARTESIAN_POINT('Ctrl Pts',(0.426934503078466,-2.48654159468299,
108.665733434406));
#35273=CARTESIAN_POINT('Ctrl Pts',(0.589355177573529,-2.45312868676567,
108.676944953262));
#35274=CARTESIAN_POINT('Ctrl Pts',(0.773808198014051,-2.39578692895605,
108.689438858101));
#35275=CARTESIAN_POINT('Ctrl Pts',(0.80013297455786,-2.38712409804105,108.691217200007));
#35276=CARTESIAN_POINT('Ctrl Pts',(0.839780322442438,-2.37334755370228,
108.693889238942));
#35277=CARTESIAN_POINT('Ctrl Pts',(0.853210612960806,-2.3685525673245,108.694793275094));
#35278=CARTESIAN_POINT('Ctrl Pts',(0.877490380605397,-2.35965070152689,
108.696425853453));
#35279=CARTESIAN_POINT('Ctrl Pts',(0.888353513293747,-2.35558248506623,
108.697155645875));
#35280=CARTESIAN_POINT('Ctrl Pts',(0.911701088606557,-2.3466543930261,108.698722928328));
#35281=CARTESIAN_POINT('Ctrl Pts',(0.924175683487847,-2.34176963690626,
108.699559566943));
#35282=CARTESIAN_POINT('Ctrl Pts',(0.957925098484118,-2.32824247746864,
108.701821380599));
#35283=CARTESIAN_POINT('Ctrl Pts',(0.979121947515239,-2.31940806967414,
108.70324012276));
#35284=CARTESIAN_POINT('Ctrl Pts',(1.09184924120375,-2.27060484844487,108.710780038984));
#35285=CARTESIAN_POINT('Ctrl Pts',(1.18106650315315,-2.22550362656058,108.716724356643));
#35286=CARTESIAN_POINT('Ctrl Pts',(1.41254605896588,-2.09063347878695,108.732381286424));
#35287=CARTESIAN_POINT('Ctrl Pts',(1.54887690997742,-1.99173584295994,108.741839705979));
#35288=CARTESIAN_POINT('Ctrl Pts',(1.73728240666024,-1.82394101861242,108.756602160552));
#35289=CARTESIAN_POINT('Ctrl Pts',(1.79736592419613,-1.76476164604931,108.761624645243));
#35290=CARTESIAN_POINT('Ctrl Pts',(1.86394491425296,-1.69225185866636,108.767735328594));
#35291=CARTESIAN_POINT('Ctrl Pts',(1.87343912186556,-1.68173506582467,108.76862064406));
#35292=CARTESIAN_POINT('Ctrl Pts',(1.88794318951693,-1.66539358008089,108.769995829921));
#35293=CARTESIAN_POINT('Ctrl Pts',(1.89301617777139,-1.65962496076666,108.77048119004));
#35294=CARTESIAN_POINT('Ctrl Pts',(1.90234542403943,-1.6489180210646,108.771382088526));
#35295=CARTESIAN_POINT('Ctrl Pts',(1.90660898007681,-1.6439862975236,108.771797082733));
#35296=CARTESIAN_POINT('Ctrl Pts',(1.91630551108093,-1.63268171053714,108.772748387447));
#35297=CARTESIAN_POINT('Ctrl Pts',(1.92172585364824,-1.62629828701506,108.773285582395));
#35298=CARTESIAN_POINT('Ctrl Pts',(1.93586748090133,-1.60947457499884,108.774701147161));
#35299=CARTESIAN_POINT('Ctrl Pts',(1.94453603364752,-1.598990589669,108.775583050609));
#35300=CARTESIAN_POINT('Ctrl Pts',(2.01516647525875,-1.51214443660754,108.782882983432));
#35301=CARTESIAN_POINT('Ctrl Pts',(2.07268396817956,-1.43228965011507,108.789557663786));
#35302=CARTESIAN_POINT('Ctrl Pts',(2.18935272312382,-1.24851455922901,108.804513568481));
#35303=CARTESIAN_POINT('Ctrl Pts',(2.24608159076478,-1.1433165920949,108.812810456099));
#35304=CARTESIAN_POINT('Ctrl Pts',(2.34450257311796,-0.924958688047079,
108.829185953278));
#35305=CARTESIAN_POINT('Ctrl Pts',(2.38597350632561,-0.812021187139037,
108.837241374193));
#35306=CARTESIAN_POINT('Ctrl Pts',(2.42776742182877,-0.666862274751989,
108.8470393948));
#35307=CARTESIAN_POINT('Ctrl Pts',(2.43576532750426,-0.637030105837842,
108.849025189864));
#35308=CARTESIAN_POINT('Ctrl Pts',(2.44680155591433,-0.592612789132666,
108.851942010241));
#35309=CARTESIAN_POINT('Ctrl Pts',(2.45026241064343,-0.578136581056765,
108.85288643593));
#35310=CARTESIAN_POINT('Ctrl Pts',(2.45620405288014,-0.552271430060218,
108.854563084024));
#35311=CARTESIAN_POINT('Ctrl Pts',(2.45873448767691,-0.54089445211354,108.855296867868));
#35312=CARTESIAN_POINT('Ctrl Pts',(2.46391683492136,-0.516806225463399,
108.856842850126));
#35313=CARTESIAN_POINT('Ctrl Pts',(2.46654960292947,-0.504091172727498,
108.857654422037));
#35314=CARTESIAN_POINT('Ctrl Pts',(2.47331500824227,-0.470094744218063,
108.85981274229));
#35315=CARTESIAN_POINT('Ctrl Pts',(2.47727139383357,-0.448779105049962,
108.861153909465));
#35316=CARTESIAN_POINT('Ctrl Pts',(2.49412221726988,-0.350967529750927,
108.867256245764));
#35317=CARTESIAN_POINT('Ctrl Pts',(2.50375278175546,-0.27394811607055,108.871914795089));
#35318=CARTESIAN_POINT('Ctrl Pts',(2.52442382519882,-0.0100610028700596,
108.887543249065));
#35319=CARTESIAN_POINT('Ctrl Pts',(2.51819422098116,0.177516684600116,108.898046085373));
#35320=CARTESIAN_POINT('Ctrl Pts',(2.48243448512861,0.423156610254938,108.912531765076));
#35321=CARTESIAN_POINT('Ctrl Pts',(2.47142941830604,0.483299230818696,108.916142924413));
#35322=CARTESIAN_POINT('Ctrl Pts',(2.45064801600347,0.577383837320642,108.921975621837));
#35323=CARTESIAN_POINT('Ctrl Pts',(2.44232730426858,0.611624758267027,108.924137432778));
#35324=CARTESIAN_POINT('Ctrl Pts',(2.4304784776155,0.656278064802941,108.927021548435));
#35325=CARTESIAN_POINT('Ctrl Pts',(2.42759649009636,0.666859654983338,108.927709828053));
#35326=CARTESIAN_POINT('Ctrl Pts',(2.42276697668829,0.684145572261141,108.928842608653));
#35327=CARTESIAN_POINT('Ctrl Pts',(2.42086050256178,0.690861354888463,108.929284795501));
#35328=CARTESIAN_POINT('Ctrl Pts',(2.41707635562121,0.703983457042877,108.930153039899));
#35329=CARTESIAN_POINT('Ctrl Pts',(2.41520109472548,0.710390375221268,108.930578958957));
#35330=CARTESIAN_POINT('Ctrl Pts',(2.41094676380002,0.724713934070805,108.931535517147));
#35331=CARTESIAN_POINT('Ctrl Pts',(2.40855414147304,0.73262645813286,108.932066919892));
#35332=CARTESIAN_POINT('Ctrl Pts',(2.40009642940454,0.760107285400779,108.933922583181));
#35333=CARTESIAN_POINT('Ctrl Pts',(2.39383166342938,0.779612634500628,108.935257483357));
#35334=CARTESIAN_POINT('Ctrl Pts',(2.3362658198685,0.951605141823017,108.947173152212));
#35335=CARTESIAN_POINT('Ctrl Pts',(2.27069886475129,1.09891258036199,108.958366828552));
#35336=CARTESIAN_POINT('Ctrl Pts',(2.13220371766402,1.34389279173709,108.97778587728));
#35337=CARTESIAN_POINT('Ctrl Pts',(2.06540573043216,1.44445325698215,108.986033146747));
#35338=CARTESIAN_POINT('Ctrl Pts',(1.9645685702433,1.57487685459164,108.996993444172));
#35339=CARTESIAN_POINT('Ctrl Pts',(1.936565054912,1.60918704634741,108.999905506404));
#35340=CARTESIAN_POINT('Ctrl Pts',(1.88615183195814,1.66773047365585,109.004925615677));
#35341=CARTESIAN_POINT('Ctrl Pts',(1.86414436128791,1.69229419268715,109.00704867235));
#35342=CARTESIAN_POINT('Ctrl Pts',(1.83124496865168,1.72759412376548,109.010125913908));
#35343=CARTESIAN_POINT('Ctrl Pts',(1.82072851487356,1.7386740015226,109.011095722724));
#35344=CARTESIAN_POINT('Ctrl Pts',(1.80197762972351,1.75807276537668,109.012800940214));
#35345=CARTESIAN_POINT('Ctrl Pts',(1.79378489550945,1.76643114286886,109.013538106927));
#35346=CARTESIAN_POINT('Ctrl Pts',(1.77652361843944,1.78379748022837,109.015075034738));
#35347=CARTESIAN_POINT('Ctrl Pts',(1.76744414296857,1.79279414000099,109.015874287265));
#35348=CARTESIAN_POINT('Ctrl Pts',(1.74344715693463,1.81621275203769,109.017963141571));
#35349=CARTESIAN_POINT('Ctrl Pts',(1.72841899227392,1.83052030217492,109.019247791894));
#35350=CARTESIAN_POINT('Ctrl Pts',(1.66307518755323,1.89120854487413,109.024736454857));
#35351=CARTESIAN_POINT('Ctrl Pts',(1.61105444541873,1.93571527797469,109.028862064715));
#35352=CARTESIAN_POINT('Ctrl Pts',(1.40282363979073,2.09965141435771,109.044587988333));
#35353=CARTESIAN_POINT('Ctrl Pts',(1.23466418538949,2.20273746325408,109.055607880864));
#35354=CARTESIAN_POINT('Ctrl Pts',(0.999823223430909,2.31128120473676,109.070695919608));
#35355=CARTESIAN_POINT('Ctrl Pts',(0.942477087573467,2.33525228024153,109.074364333308));
#35356=CARTESIAN_POINT('Ctrl Pts',(0.850948628480963,2.36959112447785,109.080279902329));
#35357=CARTESIAN_POINT('Ctrl Pts',(0.81733017887474,2.38139596608829,109.082465243418));
#35358=CARTESIAN_POINT('Ctrl Pts',(0.773010520174252,2.39590947755397,109.085376383704));
#35359=CARTESIAN_POINT('Ctrl Pts',(0.762524312630417,2.39926741968057,109.086067358711));
#35360=CARTESIAN_POINT('Ctrl Pts',(0.74534501647702,2.40464465729226,109.087203449577));
#35361=CARTESIAN_POINT('Ctrl Pts',(0.738664819041111,2.40670509279752,109.087646225212));
#35362=CARTESIAN_POINT('Ctrl Pts',(0.725595049539507,2.41067678333594,109.088514631593));
#35363=CARTESIAN_POINT('Ctrl Pts',(0.719206329340282,2.41259051268546,109.088940116727));
#35364=CARTESIAN_POINT('Ctrl Pts',(0.704905608604688,2.41681241749096,109.089894642457));
#35365=CARTESIAN_POINT('Ctrl Pts',(0.696989733440576,2.41910716698275,109.09042443662));
#35366=CARTESIAN_POINT('Ctrl Pts',(0.669495559641228,2.42693136122433,109.092269198296));
#35367=CARTESIAN_POINT('Ctrl Pts',(0.649862194865251,2.43226215740726,109.093594646919));
#35368=CARTESIAN_POINT('Ctrl Pts',(0.472145256735906,2.47821008405001,109.105652198853));
#35369=CARTESIAN_POINT('Ctrl Pts',(0.3105379007965,2.50359828578337,109.117015584906));
#35370=CARTESIAN_POINT('Ctrl Pts',(-0.0250773544836534,2.52331264180319,
109.140209223901));
#35371=CARTESIAN_POINT('Ctrl Pts',(-0.198394193695286,2.51563024589888,
109.151952980096));
#35372=CARTESIAN_POINT('Ctrl Pts',(-0.395812286315085,2.48633108232782,
109.164847881198));
#35373=CARTESIAN_POINT('Ctrl Pts',(-0.421983631928079,2.48202327127825,
109.166548530343));
#35374=CARTESIAN_POINT('Ctrl Pts',(-0.461876063855393,2.4748077154357,109.169128178034));
#35375=CARTESIAN_POINT('Ctrl Pts',(-0.475648411716759,2.47219767172996,
109.170016462));
#35376=CARTESIAN_POINT('Ctrl Pts',(-0.49965905895639,2.46743925746936,109.171561271319));
#35377=CARTESIAN_POINT('Ctrl Pts',(-0.509906994914169,2.46534186805006,
109.17221938842));
#35378=CARTESIAN_POINT('Ctrl Pts',(-0.533035750388499,2.46045784546207,
109.173702080205));
#35379=CARTESIAN_POINT('Ctrl Pts',(-0.545908425246748,2.45763380555895,
109.174525449243));
#35380=CARTESIAN_POINT('Ctrl Pts',(-0.580765552836482,2.44969937457842,
109.17675035579));
#35381=CARTESIAN_POINT('Ctrl Pts',(-0.602704743495286,2.44439413686139,
109.178145679838));
#35382=CARTESIAN_POINT('Ctrl Pts',(-0.711301645720829,2.41658269598789,
109.185031397582));
#35383=CARTESIAN_POINT('Ctrl Pts',(-0.796791996511805,2.38975877237735,
109.19038211359));
#35384=CARTESIAN_POINT('Ctrl Pts',(-1.0457741304706,2.29678467592964,109.205984010064));
#35385=CARTESIAN_POINT('Ctrl Pts',(-1.20393176061232,2.21797401137319,109.215891885325));
#35386=CARTESIAN_POINT('Ctrl Pts',(-1.40253973374737,2.09145886075199,109.229649947858));
#35387=CARTESIAN_POINT('Ctrl Pts',(-1.45137675709278,2.05786843024439,109.233155447749));
#35388=CARTESIAN_POINT('Ctrl Pts',(-1.51763988347758,2.00875953646937,109.238151730462));
#35389=CARTESIAN_POINT('Ctrl Pts',(-1.53610687086798,1.99467322974401,109.23957135806));
#35390=CARTESIAN_POINT('Ctrl Pts',(-1.56801122628479,1.96963131584228,109.242077084624));
#35391=CARTESIAN_POINT('Ctrl Pts',(-1.58153547696412,1.95878845788043,109.243156390919));
#35392=CARTESIAN_POINT('Ctrl Pts',(-1.60138840778976,1.94253204495766,109.244768137679));
#35393=CARTESIAN_POINT('Ctrl Pts',(-1.60780425245238,1.93722509260327,109.245293307571));
#35394=CARTESIAN_POINT('Ctrl Pts',(-1.61919371185878,1.92770859572735,109.246233538929));
#35395=CARTESIAN_POINT('Ctrl Pts',(-1.62417745930115,1.92351144672044,109.246647713261));
#35396=CARTESIAN_POINT('Ctrl Pts',(-1.63502895684537,1.91430042754033,109.247555611739));
#35397=CARTESIAN_POINT('Ctrl Pts',(-1.64088987842461,1.90927897901221,109.248049867951));
#35398=CARTESIAN_POINT('Ctrl Pts',(-1.65727001709763,1.89511387568682,109.249441969225));
#35399=CARTESIAN_POINT('Ctrl Pts',(-1.66773633683908,1.88590986033912,109.250344017501));
#35400=CARTESIAN_POINT('Ctrl Pts',(-1.72949579221855,1.83068284061257,109.255739106464));
#35401=CARTESIAN_POINT('Ctrl Pts',(-1.77895368377705,1.78266019255683,109.260358508032));
#35402=CARTESIAN_POINT('Ctrl Pts',(-1.94400044518552,1.60868797362264,109.276670219196));
#35403=CARTESIAN_POINT('Ctrl Pts',(-2.0486967105319,1.47304489841446,109.288634065611));
#35404=CARTESIAN_POINT('Ctrl Pts',(-2.19828907335813,1.23208470389072,109.307902200272));
#35405=CARTESIAN_POINT('Ctrl Pts',(-2.25124153304283,1.13244217619082,109.315393695307));
#35406=CARTESIAN_POINT('Ctrl Pts',(-2.30679254905932,1.00848809634885,109.324140394719));
#35407=CARTESIAN_POINT('Ctrl Pts',(-2.31595136907461,0.987273730573168,
109.325618389642));
#35408=CARTESIAN_POINT('Ctrl Pts',(-2.32991797368891,0.95365886216644,109.327931256745));
#35409=CARTESIAN_POINT('Ctrl Pts',(-2.33492160985876,0.941341636358608,
109.328772673544));
#35410=CARTESIAN_POINT('Ctrl Pts',(-2.34411129147988,0.91819565842027,109.330342696065));
#35411=CARTESIAN_POINT('Ctrl Pts',(-2.34832043804173,0.907376515852697,
109.331072057258));
#35412=CARTESIAN_POINT('Ctrl Pts',(-2.35548722762594,0.888571148750481,
109.332332140506));
#35413=CARTESIAN_POINT('Ctrl Pts',(-2.35847942165005,0.880598424396253,
109.332863994183));
#35414=CARTESIAN_POINT('Ctrl Pts',(-2.36143112100139,0.87261062952849,109.333394523839));
#35415=CARTESIAN_POINT('Origin',(0.,0.,104.));
#35416=CARTESIAN_POINT('',(-2.36143112015948,0.872610631806858,110.330000354267));
#35417=CARTESIAN_POINT('',(-2.36143112101026,0.872610629504504,110.0563084973));
#35418=CARTESIAN_POINT('',(-2.36143112101026,0.872610629504505,104.));
#35419=CARTESIAN_POINT('',(-2.51749952702257,0.00154319186397671,109.112583302534));
#35420=CARTESIAN_POINT('Ctrl Pts',(-2.36143112101026,0.872610629504504,
110.0563084973));
#35421=CARTESIAN_POINT('Ctrl Pts',(-2.34094181790185,0.928058129651828,
110.052554411366));
#35422=CARTESIAN_POINT('Ctrl Pts',(-2.31851575568189,0.982738051259023,
110.048800325432));
#35423=CARTESIAN_POINT('Ctrl Pts',(-2.29421643253635,1.03652168847553,110.045046239498));
#35424=CARTESIAN_POINT('Ctrl Pts',(-2.26020042816479,1.11181203412497,110.039790990091));
#35425=CARTESIAN_POINT('Ctrl Pts',(-2.22241142208431,1.18556516930059,110.034535740684));
#35426=CARTESIAN_POINT('Ctrl Pts',(-2.18101071128821,1.2573776390751,110.029280491277));
#35427=CARTESIAN_POINT('Ctrl Pts',(-2.13966869729493,1.32908829508128,110.02403269262));
#35428=CARTESIAN_POINT('Ctrl Pts',(-2.09472537808228,1.39886335440258,110.018784893963));
#35429=CARTESIAN_POINT('Ctrl Pts',(-2.04638950241424,1.46632065197514,110.013537095306));
#35430=CARTESIAN_POINT('Ctrl Pts',(-1.99770339165185,1.53426673583022,110.008251271823));
#35431=CARTESIAN_POINT('Ctrl Pts',(-1.94557554810732,1.59986089598963,110.00296544834));
#35432=CARTESIAN_POINT('Ctrl Pts',(-1.89026576918357,1.66273917733746,109.997679624857));
#35433=CARTESIAN_POINT('Ctrl Pts',(-1.83545194923493,1.72505363347063,109.992441198989));
#35434=CARTESIAN_POINT('Ctrl Pts',(-1.77751334011617,1.78470036907002,109.98720277312));
#35435=CARTESIAN_POINT('Ctrl Pts',(-1.71674433460059,1.8413568745946,109.981964347252));
#35436=CARTESIAN_POINT('Ctrl Pts',(-1.65599531499959,1.8979947467374,109.976727644215));
#35437=CARTESIAN_POINT('Ctrl Pts',(-1.59241808498862,1.95164402755928,109.971490941178));
#35438=CARTESIAN_POINT('Ctrl Pts',(-1.52634356479197,2.00201937358712,109.966254238141));
#35439=CARTESIAN_POINT('Ctrl Pts',(-1.46027084443221,2.05239334741571,109.961017677749));
#35440=CARTESIAN_POINT('Ctrl Pts',(-1.39170133670365,2.09949328482736,109.955781117357));
#35441=CARTESIAN_POINT('Ctrl Pts',(-1.32099756796234,2.14307528459398,109.950544556965));
#35442=CARTESIAN_POINT('Ctrl Pts',(-1.24913656910106,2.18737060422625,109.945222288194));
#35443=CARTESIAN_POINT('Ctrl Pts',(-1.17507122640473,2.22803151972832,109.939900019423));
#35444=CARTESIAN_POINT('Ctrl Pts',(-1.09920949483988,2.26484982646838,109.934577750652));
#35445=CARTESIAN_POINT('Ctrl Pts',(-1.02446222759804,2.30112724535301,109.929333669902));
#35446=CARTESIAN_POINT('Ctrl Pts',(-0.94797145635493,2.33367408074203,109.924089589152));
#35447=CARTESIAN_POINT('Ctrl Pts',(-0.870147202752004,2.36233996189009,
109.918845508402));
#35448=CARTESIAN_POINT('Ctrl Pts',(-0.790582436940955,2.39164694544241,
109.91348414562));
#35449=CARTESIAN_POINT('Ctrl Pts',(-0.70962431210848,2.41689713519337,109.908122782839));
#35450=CARTESIAN_POINT('Ctrl Pts',(-0.627724945627277,2.43798434011321,
109.902761420057));
#35451=CARTESIAN_POINT('Ctrl Pts',(-0.545825579146075,2.45907154503304,
109.897400057275));
#35452=CARTESIAN_POINT('Ctrl Pts',(-0.46298548221059,2.47599572886265,109.892038694494));
#35453=CARTESIAN_POINT('Ctrl Pts',(-0.379663322332631,2.48870689549319,
109.886677331712));
#35454=CARTESIAN_POINT('Ctrl Pts',(-0.297990294570631,2.50116647967373,
109.881422082305));
#35455=CARTESIAN_POINT('Ctrl Pts',(-0.215552450424524,2.50962436248652,
109.876166832898));
#35456=CARTESIAN_POINT('Ctrl Pts',(-0.132776023174533,2.5139961769402,109.870911583491));
#35457=CARTESIAN_POINT('Ctrl Pts',(-0.0501169540939206,2.51836179315414,
109.865663784834));
#35458=CARTESIAN_POINT('Ctrl Pts',(0.0328792876686863,2.51865282369666,
109.860415986177));
#35459=CARTESIAN_POINT('Ctrl Pts',(0.115778491415589,2.51483629505492,109.855168187519));
#35460=CARTESIAN_POINT('Ctrl Pts',(0.199278371366194,2.5109921123727,109.849882364036));
#35461=CARTESIAN_POINT('Ctrl Pts',(0.282679332651454,2.5029805222577,109.844596540553));
#35462=CARTESIAN_POINT('Ctrl Pts',(0.365534645426433,2.49082128483618,109.83931071707));
#35463=CARTESIAN_POINT('Ctrl Pts',(0.447647000325784,2.47877107845807,109.834072291202));
#35464=CARTESIAN_POINT('Ctrl Pts',(0.529222988163966,2.462647378422,109.828833865334));
#35465=CARTESIAN_POINT('Ctrl Pts',(0.609831807821048,2.44252152829196,109.823595439465));
#35466=CARTESIAN_POINT('Ctrl Pts',(0.69041411657882,2.4224022972191,109.818358736428));
#35467=CARTESIAN_POINT('Ctrl Pts',(0.77002944156567,2.3982836418633,109.813122033391));
#35468=CARTESIAN_POINT('Ctrl Pts',(0.848258268845002,2.37028777985629,109.807885330354));
#35469=CARTESIAN_POINT('Ctrl Pts',(0.926484965210141,2.34229268044259,109.802648769961));
#35470=CARTESIAN_POINT('Ctrl Pts',(1.00332480486783,2.31042074080787,109.797412209569));
#35471=CARTESIAN_POINT('Ctrl Pts',(1.07837582730909,2.27484325285841,109.792175649177));
#35472=CARTESIAN_POINT('Ctrl Pts',(1.15465523269139,2.23868345732858,109.786853380407));
#35473=CARTESIAN_POINT('Ctrl Pts',(1.22908628637025,2.19869591819411,109.781531111636));
#35474=CARTESIAN_POINT('Ctrl Pts',(1.30127223618843,2.15510946759676,109.776208842865));
#35475=CARTESIAN_POINT('Ctrl Pts',(1.37239772160992,2.11216333383603,109.770964762115));
#35476=CARTESIAN_POINT('Ctrl Pts',(1.44134327585117,2.06572364036187,109.765720681365));
#35477=CARTESIAN_POINT('Ctrl Pts',(1.50775953216826,2.01605244057682,109.760476600615));
#35478=CARTESIAN_POINT('Ctrl Pts',(1.57566116481919,1.96527036178826,109.755115237834));
#35479=CARTESIAN_POINT('Ctrl Pts',(1.6409186066216,1.9111108164844,109.749753875053));
#35480=CARTESIAN_POINT('Ctrl Pts',(1.70319662934966,1.85389522135744,109.744392512272));
#35481=CARTESIAN_POINT('Ctrl Pts',(1.76547465207773,1.79667962623047,109.73903114949));
#35482=CARTESIAN_POINT('Ctrl Pts',(1.82477294699697,1.73640839032503,109.733669786709));
#35483=CARTESIAN_POINT('Ctrl Pts',(1.88079985551424,1.67343901995191,109.728308423928));
#35484=CARTESIAN_POINT('Ctrl Pts',(1.93571786606685,1.61171595440785,109.723053174521));
#35485=CARTESIAN_POINT('Ctrl Pts',(1.98769568585796,1.54717263422441,109.717797925113));
#35486=CARTESIAN_POINT('Ctrl Pts',(2.03643048513133,1.48012064684868,109.712542675705));
#35487=CARTESIAN_POINT('Ctrl Pts',(2.08509618953059,1.41316372395862,109.707294877048));
#35488=CARTESIAN_POINT('Ctrl Pts',(2.13052773709554,1.34370556869451,109.70204707839));
#35489=CARTESIAN_POINT('Ctrl Pts',(2.17246106320583,1.27209244115928,109.696799279732));
#35490=CARTESIAN_POINT('Ctrl Pts',(2.21469823241219,1.19996041478137,109.691513456249));
#35491=CARTESIAN_POINT('Ctrl Pts',(2.25338595599294,1.12564240913494,109.686227632767));
#35492=CARTESIAN_POINT('Ctrl Pts',(2.28829758582821,1.04952389619903,109.680941809284));
#35493=CARTESIAN_POINT('Ctrl Pts',(2.32289616549057,0.974087932710064,109.675703383415));
#35494=CARTESIAN_POINT('Ctrl Pts',(2.35378590421434,0.896884049792989,109.670464957546));
#35495=CARTESIAN_POINT('Ctrl Pts',(2.38079209408838,0.818312443218525,109.665226531677));
#35496=CARTESIAN_POINT('Ctrl Pts',(2.40778940207603,0.739766677537807,109.659989828639));
#35497=CARTESIAN_POINT('Ctrl Pts',(2.4309055480056,0.659854517589931,109.654753125602));
#35498=CARTESIAN_POINT('Ctrl Pts',(2.45001464206608,0.578994390008915,109.649516422564));
#35499=CARTESIAN_POINT('Ctrl Pts',(2.46912321560441,0.498136465017324,109.644279862171));
#35500=CARTESIAN_POINT('Ctrl Pts',(2.48422484917438,0.416331073022448,109.639043301779));
#35501=CARTESIAN_POINT('Ctrl Pts',(2.49524437307892,0.334008635544001,109.633806741386));
#35502=CARTESIAN_POINT('Ctrl Pts',(2.50644425688482,0.250338801677915,109.628484472616));
#35503=CARTESIAN_POINT('Ctrl Pts',(2.51342712091624,0.166135329980568,109.623162203846));
#35504=CARTESIAN_POINT('Ctrl Pts',(2.51616889547696,0.0818556011171571,
109.617839935076));
#35505=CARTESIAN_POINT('Ctrl Pts',(2.51887039136475,-0.00118599690829541,
109.612595854325));
#35506=CARTESIAN_POINT('Ctrl Pts',(2.5174546493823,-0.084301159516965,109.607351773574));
#35507=CARTESIAN_POINT('Ctrl Pts',(2.51195126463292,-0.16705416519519,109.602107692824));
#35508=CARTESIAN_POINT('Ctrl Pts',(2.50632479861102,-0.25165791286358,109.596746330044));
#35509=CARTESIAN_POINT('Ctrl Pts',(2.49642570589944,-0.335882600564322,
109.591384967264));
#35510=CARTESIAN_POINT('Ctrl Pts',(2.48234107280901,-0.419272045628374,
109.586023604484));
#35511=CARTESIAN_POINT('Ctrl Pts',(2.46825643971858,-0.502661490692423,
109.580662241704));
#35512=CARTESIAN_POINT('Ctrl Pts',(2.44998644126181,-0.585215211450702,
109.575300878924));
#35513=CARTESIAN_POINT('Ctrl Pts',(2.42767215699761,-0.666493922056721,
109.569939516144));
#35514=CARTESIAN_POINT('Ctrl Pts',(2.40579952237753,-0.746163945008328,
109.564684266737));
#35515=CARTESIAN_POINT('Ctrl Pts',(2.37996048847428,-0.824903250673477,
109.55942901733));
#35516=CARTESIAN_POINT('Ctrl Pts',(2.3502515363011,-0.902288183516956,109.554173767922));
#35517=CARTESIAN_POINT('Ctrl Pts',(2.32058470467304,-0.979563402105383,
109.548925969265));
#35518=CARTESIAN_POINT('Ctrl Pts',(2.2870590168895,-1.05548763476304,109.543678170607));
#35519=CARTESIAN_POINT('Ctrl Pts',(2.24982114285869,-1.12965086427003,109.53843037195));
#35520=CARTESIAN_POINT('Ctrl Pts',(2.21231344832706,-1.20435147031229,109.533144548467));
#35521=CARTESIAN_POINT('Ctrl Pts',(2.17103967003756,-1.27726498857237,109.527858724984));
#35522=CARTESIAN_POINT('Ctrl Pts',(2.12619973998966,-1.34799143753508,109.522572901501));
#35523=CARTESIAN_POINT('Ctrl Pts',(2.08176188650013,-1.41808368731073,109.517334475633));
#35524=CARTESIAN_POINT('Ctrl Pts',(2.03382183159514,-1.48602753641291,109.512096049764));
#35525=CARTESIAN_POINT('Ctrl Pts',(1.98262013640475,-1.55145855398152,109.506857623896));
#35526=CARTESIAN_POINT('Ctrl Pts',(1.93143528059979,-1.61686805237737,109.501620920858));
#35527=CARTESIAN_POINT('Ctrl Pts',(1.87699119908413,-1.67976599747351,109.496384217821));
#35528=CARTESIAN_POINT('Ctrl Pts',(1.81957032398615,-1.73981898083362,109.491147514783));
#35529=CARTESIAN_POINT('Ctrl Pts',(1.76215101300411,-1.79987032838048,109.485910954391));
#35530=CARTESIAN_POINT('Ctrl Pts',(1.70175538928872,-1.85707653548407,109.480674393999));
#35531=CARTESIAN_POINT('Ctrl Pts',(1.63870356083115,-1.91114020671413,109.475437833607));
#35532=CARTESIAN_POINT('Ctrl Pts',(1.57461974390001,-1.96608875451181,109.470115564836));
#35533=CARTESIAN_POINT('Ctrl Pts',(1.50779235267326,-2.01779063860604,109.464793296066));
#35534=CARTESIAN_POINT('Ctrl Pts',(1.43859192974068,-2.06597664790408,109.459471027295));
#35535=CARTESIAN_POINT('Ctrl Pts',(1.37040811162573,-2.11345476948817,109.454226946545));
#35536=CARTESIAN_POINT('Ctrl Pts',(1.2999209515205,-2.15751943606303,109.448982865794));
#35537=CARTESIAN_POINT('Ctrl Pts',(1.22751204236929,-2.19795824251472,109.443738785044));
#35538=CARTESIAN_POINT('Ctrl Pts',(1.15348373330948,-2.2393014487183,109.438377422264));
#35539=CARTESIAN_POINT('Ctrl Pts',(1.0774471385546,-2.27685442882497,109.433016059483));
#35540=CARTESIAN_POINT('Ctrl Pts',(0.999832314886172,-2.31044186079403,
109.427654696702));
#35541=CARTESIAN_POINT('Ctrl Pts',(0.922217491217744,-2.34402929276309,
109.422293333921));
#35542=CARTESIAN_POINT('Ctrl Pts',(0.843024937941911,-2.3736510611482,109.416931971141));
#35543=CARTESIAN_POINT('Ctrl Pts',(0.762699935624001,-2.39918633253008,
109.41157060836));
#35544=CARTESIAN_POINT('Ctrl Pts',(0.683964744948231,-2.4242162037183,109.406315358953));
#35545=CARTESIAN_POINT('Ctrl Pts',(0.603850720470603,-2.44541235930828,
109.401060109545));
#35546=CARTESIAN_POINT('Ctrl Pts',(0.522765750423893,-2.46262506691208,
109.395804860138));
#35547=CARTESIAN_POINT('Ctrl Pts',(0.441795740444478,-2.47981337080675,
109.390557061481));
#35548=CARTESIAN_POINT('Ctrl Pts',(0.359857966783513,-2.49302934952956,
109.385309262823));
#35549=CARTESIAN_POINT('Ctrl Pts',(0.277376203382308,-2.50217279415256,
109.380061464166));
#35550=CARTESIAN_POINT('Ctrl Pts',(0.194296788497055,-2.51138249091449,
109.374775640683));
#35551=CARTESIAN_POINT('Ctrl Pts',(0.110665918875473,-2.51646024294225,
109.3694898172));
#35552=CARTESIAN_POINT('Ctrl Pts',(0.0269279492159412,-2.51735598109426,
109.364203993717));
#35553=CARTESIAN_POINT('Ctrl Pts',(-0.0560591478492334,-2.51824368722407,
109.358965567848));
#35554=CARTESIAN_POINT('Ctrl Pts',(-0.139150962031731,-2.51502407372498,
109.35372714198));
#35555=CARTESIAN_POINT('Ctrl Pts',(-0.221910837654832,-2.5077005064663,
109.348488716111));
#35556=CARTESIAN_POINT('Ctrl Pts',(-0.304643494932171,-2.50037934780701,
109.343252013074));
#35557=CARTESIAN_POINT('Ctrl Pts',(-0.38704397120383,-2.48895695665119,
109.338015310036));
#35558=CARTESIAN_POINT('Ctrl Pts',(-0.468678835432439,-2.47348871014559,
109.332778606999));
#35559=CARTESIAN_POINT('Ctrl Pts',(-0.550311475968167,-2.45802088498729,
109.327542046607));
#35560=CARTESIAN_POINT('Ctrl Pts',(-0.631178092763609,-2.43850751051419,
109.322305486214));
#35561=CARTESIAN_POINT('Ctrl Pts',(-0.710854949530708,-2.41505517343345,
109.317068925822));
#35562=CARTESIAN_POINT('Ctrl Pts',(-0.791835901669957,-2.3912189848117,
109.311746657051));
#35563=CARTESIAN_POINT('Ctrl Pts',(-0.871587320650252,-2.36331385611554,
109.306424388281));
#35564=CARTESIAN_POINT('Ctrl Pts',(-0.949681651792507,-2.33150402321091,
109.30110211951));
#35565=CARTESIAN_POINT('Ctrl Pts',(-1.02662872010301,-2.30016150001291,
109.29585803876));
#35566=CARTESIAN_POINT('Ctrl Pts',(-1.10196666682814,-2.26502849041496,
109.29061395801));
#35567=CARTESIAN_POINT('Ctrl Pts',(-1.17530956932278,-2.22630942733895,
109.28536987726));
#35568=CARTESIAN_POINT('Ctrl Pts',(-1.2502927601582,-2.18672442597076,109.280008514479));
#35569=CARTESIAN_POINT('Ctrl Pts',(-1.3231901528662,-2.14339129554009,109.274647151698));
#35570=CARTESIAN_POINT('Ctrl Pts',(-1.39362054358561,-2.0965753099987,109.269285788918));
#35571=CARTESIAN_POINT('Ctrl Pts',(-1.46405093430502,-2.04975932445731,
109.263924426137));
#35572=CARTESIAN_POINT('Ctrl Pts',(-1.53201395435234,-1.99946083976441,
109.258563063356));
#35573=CARTESIAN_POINT('Ctrl Pts',(-1.5971658158888,-1.94598756587915,109.253201700576));
#35574=CARTESIAN_POINT('Ctrl Pts',(-1.66018580041137,-1.89426402624193,
109.248015770481));
#35575=CARTESIAN_POINT('Ctrl Pts',(-1.7208219529501,-1.83936794722398,109.242829840387));
#35576=CARTESIAN_POINT('Ctrl Pts',(-1.77873133380123,-1.78155019355439,
109.237643910292));
#35577=CARTESIAN_POINT('Ctrl Pts',(-1.8369190827697,-1.72345451221573,109.232433051636));
#35578=CARTESIAN_POINT('Ctrl Pts',(-1.89235335502134,-1.66240923774307,
109.227222192979));
#35579=CARTESIAN_POINT('Ctrl Pts',(-1.94471789917081,-1.59871152577464,
109.222011334322));
#35580=CARTESIAN_POINT('Ctrl Pts',(-1.99669805314474,-1.53548139688332,
109.216838726794));
#35581=CARTESIAN_POINT('Ctrl Pts',(-2.04565307367539,-1.4696379988631,109.211666119265));
#35582=CARTESIAN_POINT('Ctrl Pts',(-2.09131013992786,-1.40150923958243,
109.206493511736));
#35583=CARTESIAN_POINT('Ctrl Pts',(-2.1369397234866,-1.33342148954696,109.201324017793));
#35584=CARTESIAN_POINT('Ctrl Pts',(-2.179275028083,-1.26305150124533,109.19615452385));
#35585=CARTESIAN_POINT('Ctrl Pts',(-2.21808489358349,-1.19075843681946,
109.190985029907));
#35586=CARTESIAN_POINT('Ctrl Pts',(-2.25688384819613,-1.1184856966464,109.1858169893));
#35587=CARTESIAN_POINT('Ctrl Pts',(-2.29215910763426,-1.04429137214069,
109.180648948693));
#35588=CARTESIAN_POINT('Ctrl Pts',(-2.323724860714,-0.968560282945616,109.175480908086));
#35589=CARTESIAN_POINT('Ctrl Pts',(-2.35573909391273,-0.891753221071957,
109.170239440956));
#35590=CARTESIAN_POINT('Ctrl Pts',(-2.38393735988397,-0.813365831117959,
109.164997973827));
#35591=CARTESIAN_POINT('Ctrl Pts',(-2.40817655178005,-0.733820104287649,
109.159756506698));
#35592=CARTESIAN_POINT('Ctrl Pts',(-2.43209781731412,-0.655317716016403,
109.154583787759));
#35593=CARTESIAN_POINT('Ctrl Pts',(-2.45216318475308,-0.575687678742618,
109.14941106882));
#35594=CARTESIAN_POINT('Ctrl Pts',(-2.46828607654817,-0.495348457470522,
109.14423834988));
#35595=CARTESIAN_POINT('Ctrl Pts',(-2.48473039107442,-0.413407609626218,
109.138962508656));
#35596=CARTESIAN_POINT('Ctrl Pts',(-2.49707324762341,-0.33072950682054,
109.133686667432));
#35597=CARTESIAN_POINT('Ctrl Pts',(-2.50527825607931,-0.247764221824343,
109.128410826207));
#35598=CARTESIAN_POINT('Ctrl Pts',(-2.51348326453521,-0.16479893682814,
109.123134984983));
#35599=CARTESIAN_POINT('Ctrl Pts',(-2.51755046013732,-0.0815469897811725,
109.117859143758));
#35600=CARTESIAN_POINT('Ctrl Pts',(-2.51749952702257,0.00154319186397808,
109.112583302534));
#35601=CARTESIAN_POINT('Ctrl Pts',(-2.51749952702217,0.00154319252614217,
109.112583302492));
#35602=CARTESIAN_POINT('Ctrl Pts',(-2.51744240569643,0.0947285262351732,
109.106666465925));
#35603=CARTESIAN_POINT('Ctrl Pts',(-2.51221164500478,0.18775354483245,109.100749629358));
#35604=CARTESIAN_POINT('Ctrl Pts',(-2.50185877901989,0.280194396519821,
109.094832792791));
#35605=CARTESIAN_POINT('Ctrl Pts',(-2.49266337038751,0.362300299062281,
109.089577462516));
#35606=CARTESIAN_POINT('Ctrl Pts',(-2.47940487525419,0.44410469072322,109.084322132241));
#35607=CARTESIAN_POINT('Ctrl Pts',(-2.46211260492313,0.525174038465942,
109.079066801966));
#35608=CARTESIAN_POINT('Ctrl Pts',(-2.44484692813231,0.606118710794753,
109.07381955379));
#35609=CARTESIAN_POINT('Ctrl Pts',(-2.42355989977268,0.686330138217152,
109.068572305614));
#35610=CARTESIAN_POINT('Ctrl Pts',(-2.39833250270469,0.76538059582816,109.063325057437));
#35611=CARTESIAN_POINT('Ctrl Pts',(-2.38684469401716,0.801377830550768,
109.060935616187));
#35612=CARTESIAN_POINT('Ctrl Pts',(-2.37454050980643,0.837134418656268,
109.058546174938));
#35613=CARTESIAN_POINT('Ctrl Pts',(-2.36143112101026,0.8726106295045,109.056156733688));
#35614=CARTESIAN_POINT('Ctrl Pts',(-2.36143112100139,0.87261062952849,109.333394523839));
#35615=CARTESIAN_POINT('Ctrl Pts',(-2.36346984958465,0.867093487104515,
109.333760958848));
#35616=CARTESIAN_POINT('Ctrl Pts',(-2.36548925970523,0.861569155118568,
109.334126762288));
#35617=CARTESIAN_POINT('Ctrl Pts',(-2.37506141720324,0.835096045723733,
109.335874488354));
#35618=CARTESIAN_POINT('Ctrl Pts',(-2.38235550549763,0.814054319465642,
109.337247961307));
#35619=CARTESIAN_POINT('Ctrl Pts',(-2.438745542544,0.644129267194206,109.348220758002));
#35620=CARTESIAN_POINT('Ctrl Pts',(-2.47411894835068,0.491046575985721,
109.357347000226));
#35621=CARTESIAN_POINT('Ctrl Pts',(-2.51007103693908,0.223800113368748,
109.372868433239));
#35622=CARTESIAN_POINT('Ctrl Pts',(-2.51757913315039,0.111069461290839,
109.37930321569));
#35623=CARTESIAN_POINT('Ctrl Pts',(-2.51748053141364,-0.0284342513975516,
109.387482928585));
#35624=CARTESIAN_POINT('Ctrl Pts',(-2.5170383666155,-0.0550864820178238,
109.38905572446));
#35625=CARTESIAN_POINT('Ctrl Pts',(-2.51439311537659,-0.136528308785591,
109.393905511809));
#35626=CARTESIAN_POINT('Ctrl Pts',(-2.51082333543405,-0.191253570963997,
109.397224888042));
#35627=CARTESIAN_POINT('Ctrl Pts',(-2.50419226738626,-0.258841019621582,
109.401446971244));
#35628=CARTESIAN_POINT('Ctrl Pts',(-2.50281263159588,-0.271857498427805,
109.40226575223));
#35629=CARTESIAN_POINT('Ctrl Pts',(-2.5004800230266,-0.29233977185561,109.403563913153));
#35630=CARTESIAN_POINT('Ctrl Pts',(-2.49959494432716,-0.299813272812452,
109.404039631313));
#35631=CARTESIAN_POINT('Ctrl Pts',(-2.49795805589807,-0.31312367426411,
109.404890724882));
#35632=CARTESIAN_POINT('Ctrl Pts',(-2.49721927243702,-0.318962046818765,
109.40526537069));
#35633=CARTESIAN_POINT('Ctrl Pts',(-2.49539701410415,-0.332968286145085,
109.406167309786));
#35634=CARTESIAN_POINT('Ctrl Pts',(-2.4942939136824,-0.341133412569161,
109.406695679288));
#35635=CARTESIAN_POINT('Ctrl Pts',(-2.49080758458314,-0.366017816506546,
109.408313508455));
#35636=CARTESIAN_POINT('Ctrl Pts',(-2.48829623603564,-0.382718265534257,
109.409409670501));
#35637=CARTESIAN_POINT('Ctrl Pts',(-2.48205424858673,-0.421565325297277,
109.411981780215));
#35638=CARTESIAN_POINT('Ctrl Pts',(-2.47819493482364,-0.443689539333963,
109.413463615741));
#35639=CARTESIAN_POINT('Ctrl Pts',(-2.46361967436347,-0.521111197328586,
109.418702116494));
#35640=CARTESIAN_POINT('Ctrl Pts',(-2.45134493936348,-0.57609546026345,
109.422517357224));
#35641=CARTESIAN_POINT('Ctrl Pts',(-2.39532394427507,-0.792607583981021,
109.437811005721));
#35642=CARTESIAN_POINT('Ctrl Pts',(-2.33736025802409,-0.950030092836987,
109.449502067731));
#35643=CARTESIAN_POINT('Ctrl Pts',(-2.21986824165573,-1.19175400172207,
109.467689887044));
#35644=CARTESIAN_POINT('Ctrl Pts',(-2.17005539982266,-1.28021744699912,
109.474411240295));
#35645=CARTESIAN_POINT('Ctrl Pts',(-2.10253295841837,-1.38480780114625,
109.482429521941));
#35646=CARTESIAN_POINT('Ctrl Pts',(-2.08976618527293,-1.40399958544812,
109.483904251773));
#35647=CARTESIAN_POINT('Ctrl Pts',(-2.06915392804172,-1.43408098113171,
109.4862218571));
#35648=CARTESIAN_POINT('Ctrl Pts',(-2.06148210285805,-1.44508746769828,
109.487071167814));
#35649=CARTESIAN_POINT('Ctrl Pts',(-2.04701457617386,-1.46549380489623,
109.488648496492));
#35650=CARTESIAN_POINT('Ctrl Pts',(-2.04024122290779,-1.47490898934411,
109.489377334437));
#35651=CARTESIAN_POINT('Ctrl Pts',(-2.02501023821994,-1.49577485600221,
109.490995187945));
#35652=CARTESIAN_POINT('Ctrl Pts',(-2.01652002237354,-1.50720134596288,
109.49188292278));
#35653=CARTESIAN_POINT('Ctrl Pts',(-1.99129290285451,-1.54055829234207,
109.494480221376));
#35654=CARTESIAN_POINT('Ctrl Pts',(-1.97429158922705,-1.56228681409909,
109.496179480908));
#35655=CARTESIAN_POINT('Ctrl Pts',(-1.93479290357716,-1.61109329947915,
109.50001702054));
#35656=CARTESIAN_POINT('Ctrl Pts',(-1.9120776619221,-1.6379879079882,109.502146631196));
#35657=CARTESIAN_POINT('Ctrl Pts',(-1.83369471278203,-1.72693903970804,
109.509255455459));
#35658=CARTESIAN_POINT('Ctrl Pts',(-1.77550937380536,-1.78670724155929,
109.514140886404));
#35659=CARTESIAN_POINT('Ctrl Pts',(-1.64411754920209,-1.90890338974462,
109.524539441658));
#35660=CARTESIAN_POINT('Ctrl Pts',(-1.57008586047114,-1.9702449534474,109.530025511459));
#35661=CARTESIAN_POINT('Ctrl Pts',(-1.47237922826388,-2.04219106653644,
109.537021166083));
#35662=CARTESIAN_POINT('Ctrl Pts',(-1.45180447133898,-2.05686866191258,
109.538481671739));
#35663=CARTESIAN_POINT('Ctrl Pts',(-1.34625820570126,-2.12979042484566,
109.545927628196));
#35664=CARTESIAN_POINT('Ctrl Pts',(-1.25799940137787,-2.18308287036585,
109.552002056204));
#35665=CARTESIAN_POINT('Ctrl Pts',(-1.1546145115725,-2.23715415990781,109.559232998796));
#35666=CARTESIAN_POINT('Ctrl Pts',(-1.1424407580423,-2.24339530639306,109.560086225954));
#35667=CARTESIAN_POINT('Ctrl Pts',(-1.12271371071132,-2.25330661156631,
109.561472663653));
#35668=CARTESIAN_POINT('Ctrl Pts',(-1.11519167762764,-2.25703882981834,
109.562002208242));
#35669=CARTESIAN_POINT('Ctrl Pts',(-1.10179520818773,-2.26360245946967,
109.562947130089));
#35670=CARTESIAN_POINT('Ctrl Pts',(-1.09592825977956,-2.26644876916602,
109.563361583586));
#35671=CARTESIAN_POINT('Ctrl Pts',(-1.08314060552501,-2.27259134851176,
109.564266352561));
#35672=CARTESIAN_POINT('Ctrl Pts',(-1.07621598820648,-2.27587876471487,
109.564757170805));
#35673=CARTESIAN_POINT('Ctrl Pts',(-1.05652005003723,-2.28511929253639,
109.566155484484));
#35674=CARTESIAN_POINT('Ctrl Pts',(-1.04371384608329,-2.29099676629381,
109.567067347726));
#35675=CARTESIAN_POINT('Ctrl Pts',(-0.95590180266367,-2.33040951181688,
109.573334927669));
#35676=CARTESIAN_POINT('Ctrl Pts',(-0.879349628913439,-2.36035975501343,
109.578871567652));
#35677=CARTESIAN_POINT('Ctrl Pts',(-0.644383220125851,-2.43927021755126,
109.595814669249));
#35678=CARTESIAN_POINT('Ctrl Pts',(-0.482447046194343,-2.47639249119478,
109.607394073785));
#35679=CARTESIAN_POINT('Ctrl Pts',(-0.214874691263757,-2.51046816798263,
109.625666546562));
#35680=CARTESIAN_POINT('Ctrl Pts',(-0.110986203589693,-2.5172025135603,
109.63256452816));
#35681=CARTESIAN_POINT('Ctrl Pts',(0.0162200407558962,-2.51755452374944,
109.640758791927));
#35682=CARTESIAN_POINT('Ctrl Pts',(0.0394069677846057,-2.51729835724784,
109.642242511613));
#35683=CARTESIAN_POINT('Ctrl Pts',(0.0760307746945406,-2.51638756939638,
109.644571033584));
#35684=CARTESIAN_POINT('Ctrl Pts',(0.0894711651940837,-2.5159455479244,
109.645422372565));
#35685=CARTESIAN_POINT('Ctrl Pts',(0.114493880676477,-2.51492184137784,
109.647001612961));
#35686=CARTESIAN_POINT('Ctrl Pts',(0.126076916518214,-2.51436778043953,
109.647730350782));
#35687=CARTESIAN_POINT('Ctrl Pts',(0.151830052040208,-2.51295749969201,
109.649345671937));
#35688=CARTESIAN_POINT('Ctrl Pts',(0.165997640259432,-2.5120614157388,109.650230994418));
#35689=CARTESIAN_POINT('Ctrl Pts',(0.207478766265878,-2.50908531662416,
109.652813924134));
#35690=CARTESIAN_POINT('Ctrl Pts',(0.234767371536839,-2.50667926461903,
109.654501403183));
#35691=CARTESIAN_POINT('Ctrl Pts',(0.409372627539705,-2.48840776669711,
109.665233473326));
#35692=CARTESIAN_POINT('Ctrl Pts',(0.555091765975768,-2.46000814296342,
109.673868613575));
#35693=CARTESIAN_POINT('Ctrl Pts',(0.847737503890756,-2.37562646291455,
109.691409784299));
#35694=CARTESIAN_POINT('Ctrl Pts',(0.993615204999481,-2.3184002987068,109.700270387116));
#35695=CARTESIAN_POINT('Ctrl Pts',(1.17239575523607,-2.22827700514637,109.712289230991));
#35696=CARTESIAN_POINT('Ctrl Pts',(1.21103827733235,-2.2075135297388,109.714962857984));
#35697=CARTESIAN_POINT('Ctrl Pts',(1.25979404845179,-2.17965053703283,109.718459806681));
#35698=CARTESIAN_POINT('Ctrl Pts',(1.27042695876615,-2.17347022896262,109.719230145277));
#35699=CARTESIAN_POINT('Ctrl Pts',(1.28727700254527,-2.16351036517836,109.720463919338));
#35700=CARTESIAN_POINT('Ctrl Pts',(1.29352392836076,-2.15978124473093,109.720924198332));
#35701=CARTESIAN_POINT('Ctrl Pts',(1.30541129630678,-2.15261497394746,109.721805740327));
#35702=CARTESIAN_POINT('Ctrl Pts',(1.31105446944537,-2.14918264758338,109.722226698313));
#35703=CARTESIAN_POINT('Ctrl Pts',(1.3244229870632,-2.14097931926834,109.723229734364));
#35704=CARTESIAN_POINT('Ctrl Pts',(1.33213610497564,-2.1361886822006,109.723813064418));
#35705=CARTESIAN_POINT('Ctrl Pts',(1.35802489082578,-2.11991435625366,109.725786145086));
#35706=CARTESIAN_POINT('Ctrl Pts',(1.3760787582864,-2.10823994370133,109.727187411152));
#35707=CARTESIAN_POINT('Ctrl Pts',(1.48164213695745,-2.03804449734193,109.735521148586));
#35708=CARTESIAN_POINT('Ctrl Pts',(1.56555319278055,-1.97431700619429,109.742716984641));
#35709=CARTESIAN_POINT('Ctrl Pts',(1.78678930491417,-1.78330363322121,109.762863477234));
#35710=CARTESIAN_POINT('Ctrl Pts',(1.91431841023979,-1.64565848939293,109.775834612889));
#35711=CARTESIAN_POINT('Ctrl Pts',(2.05876710896484,-1.44997777030523,109.791913260181));
#35712=CARTESIAN_POINT('Ctrl Pts',(2.09058847857081,-1.40370872004539,109.795570851985));
#35713=CARTESIAN_POINT('Ctrl Pts',(2.13124773119218,-1.34013529890697,109.800409868807));
#35714=CARTESIAN_POINT('Ctrl Pts',(2.14146971785509,-1.32373977525013,109.801641831734));
#35715=CARTESIAN_POINT('Ctrl Pts',(2.15797823903794,-1.29656920952478,109.803657710542));
#35716=CARTESIAN_POINT('Ctrl Pts',(2.16437508709541,-1.28586246803049,109.804445615109));
#35717=CARTESIAN_POINT('Ctrl Pts',(2.17667959459117,-1.26491578073643,109.805974714704));
#35718=CARTESIAN_POINT('Ctrl Pts',(2.18259520292458,-1.25468090671586,109.806716181823));
#35719=CARTESIAN_POINT('Ctrl Pts',(2.19636825885272,-1.23045929348502,109.808457816894));
#35720=CARTESIAN_POINT('Ctrl Pts',(2.20416459824456,-1.21643826147093,109.809455789388));
#35721=CARTESIAN_POINT('Ctrl Pts',(2.22965681919375,-1.16954286512847,109.81276079625));
#35722=CARTESIAN_POINT('Ctrl Pts',(2.24675593487772,-1.1363485534053,109.815046915215));
#35723=CARTESIAN_POINT('Ctrl Pts',(2.34240742133841,-0.940054646262984,
109.828282878177));
#35724=CARTESIAN_POINT('Ctrl Pts',(2.40392278574608,-0.76924523925228,109.838626697978));
#35725=CARTESIAN_POINT('Ctrl Pts',(2.47888245101036,-0.46013491701283,109.856916111287));
#35726=CARTESIAN_POINT('Ctrl Pts',(2.5002453912599,-0.324570399740312,109.864820011941));
#35727=CARTESIAN_POINT('Ctrl Pts',(2.51207333564027,-0.166592293806112,
109.8745484853));
#35728=CARTESIAN_POINT('Ctrl Pts',(2.51340027666628,-0.145204734981214,
109.875876613134));
#35729=CARTESIAN_POINT('Ctrl Pts',(2.51486834015722,-0.115388348748911,
109.877746770805));
#35730=CARTESIAN_POINT('Ctrl Pts',(2.51524042787282,-0.106971139050084,
109.87827678384));
#35731=CARTESIAN_POINT('Ctrl Pts',(2.51580952623664,-0.0924447807835918,
109.879195281467));
#35732=CARTESIAN_POINT('Ctrl Pts',(2.51602655575973,-0.0863364268397177,
109.879582671416));
#35733=CARTESIAN_POINT('Ctrl Pts',(2.51643757768587,-0.0734452965639899,
109.880402784831));
#35734=CARTESIAN_POINT('Ctrl Pts',(2.51662639417135,-0.0666624536343644,
109.880835800592));
#35735=CARTESIAN_POINT('Ctrl Pts',(2.51702696808261,-0.0498258560599105,
109.881914238328));
#35736=CARTESIAN_POINT('Ctrl Pts',(2.51720590979569,-0.0397715167232285,
109.882561428108));
#35737=CARTESIAN_POINT('Ctrl Pts',(2.51765389437049,-0.00182224345531749,
109.885015506109));
#35738=CARTESIAN_POINT('Ctrl Pts',(2.51751949958342,0.0260742971917743,
109.886842557029));
#35739=CARTESIAN_POINT('Ctrl Pts',(2.515983127897,0.0977352401847407,109.891585589694));
#35740=CARTESIAN_POINT('Ctrl Pts',(2.51390289075263,0.141474738151433,109.894528157572));
#35741=CARTESIAN_POINT('Ctrl Pts',(2.5015626962541,0.308824500872177,109.905917914244));
#35742=CARTESIAN_POINT('Ctrl Pts',(2.48331440821473,0.431667625630043,109.914544530062));
#35743=CARTESIAN_POINT('Ctrl Pts',(2.42057821092703,0.710473413325409,109.934220995561));
#35744=CARTESIAN_POINT('Ctrl Pts',(2.36993616672713,0.864517724247111,109.945146938457));
#35745=CARTESIAN_POINT('Ctrl Pts',(2.29590555748541,1.03301415870238,109.95701699396));
#35746=CARTESIAN_POINT('Ctrl Pts',(2.28669267099375,1.0532508063944,109.958441908611));
#35747=CARTESIAN_POINT('Ctrl Pts',(2.27107873114421,1.08637683344634,109.960773813584));
#35748=CARTESIAN_POINT('Ctrl Pts',(2.26483326338453,1.09933776900559,109.9616860519));
#35749=CARTESIAN_POINT('Ctrl Pts',(2.2533484462779,1.12265835212401,109.963327409729));
#35750=CARTESIAN_POINT('Ctrl Pts',(2.24814793446607,1.13303656956481,109.964057842713));
#35751=CARTESIAN_POINT('Ctrl Pts',(2.23683435812628,1.15522952153017,109.965619965314));
#35752=CARTESIAN_POINT('Ctrl Pts',(2.2306990387499,1.16703256270518,109.966450853798));
#35753=CARTESIAN_POINT('Ctrl Pts',(2.21363500498472,1.19923384260389,109.96871834599));
#35754=CARTESIAN_POINT('Ctrl Pts',(2.20251797246947,1.21953121335917,109.970148316695));
#35755=CARTESIAN_POINT('Ctrl Pts',(2.13525389273553,1.33842049743581,109.978533689033));
#35756=CARTESIAN_POINT('Ctrl Pts',(2.0727704661541,1.43328497146815,109.985255357299));
#35757=CARTESIAN_POINT('Ctrl Pts',(1.89641154450373,1.66525865298754,110.002207016496));
#35758=CARTESIAN_POINT('Ctrl Pts',(1.77402711162415,1.79507187028435,110.012193334975));
#35759=CARTESIAN_POINT('Ctrl Pts',(1.59207714147863,1.95113219459781,110.026391986564));
#35760=CARTESIAN_POINT('Ctrl Pts',(1.54370027120321,1.98962674905459,110.030118445536));
#35761=CARTESIAN_POINT('Ctrl Pts',(1.48306078753487,2.03433535628456,110.034798695307));
#35762=CARTESIAN_POINT('Ctrl Pts',(1.47209647748619,2.04228342387063,110.035645298137));
#35763=CARTESIAN_POINT('Ctrl Pts',(1.45485631443609,2.05456991914629,110.036977962798));
#35764=CARTESIAN_POINT('Ctrl Pts',(1.44862377075494,2.05896906617798,110.037460036284));
#35765=CARTESIAN_POINT('Ctrl Pts',(1.43702309065858,2.06707848660173,110.038358068399));
#35766=CARTESIAN_POINT('Ctrl Pts',(1.43166042965011,2.0707962825175,110.038773512639));
#35767=CARTESIAN_POINT('Ctrl Pts',(1.4193212636266,2.07927987157974,110.039730102644));
#35768=CARTESIAN_POINT('Ctrl Pts',(1.41233519957301,2.08403140880092,110.040272171893));
#35769=CARTESIAN_POINT('Ctrl Pts',(1.39041282617187,2.09878095040168,110.041974346044));
#35770=CARTESIAN_POINT('Ctrl Pts',(1.37539365486613,2.10865396772303,110.043142178256));
#35771=CARTESIAN_POINT('Ctrl Pts',(1.33978923477499,2.1315167157797,110.045912148842));
#35772=CARTESIAN_POINT('Ctrl Pts',(1.31911901981497,2.14437021581,110.047521423599));
#35773=CARTESIAN_POINT('Ctrl Pts',(1.24373340008868,2.18974536147545,110.053385993537));
#35774=CARTESIAN_POINT('Ctrl Pts',(1.18797839541248,2.22048729241579,110.057714350784));
#35775=CARTESIAN_POINT('Ctrl Pts',(0.938813812376638,2.34579873148568,110.076848734929));
#35776=CARTESIAN_POINT('Ctrl Pts',(0.73485300110441,2.41747031016112,110.091875517807));
#35777=CARTESIAN_POINT('Ctrl Pts',(0.473733481223952,2.47306492985238,110.109473561756));
#35778=CARTESIAN_POINT('Ctrl Pts',(0.422897961496968,2.48226338438602,110.112832051939));
#35779=CARTESIAN_POINT('Ctrl Pts',(0.353272504175593,2.49266046113153,110.117343059449));
#35780=CARTESIAN_POINT('Ctrl Pts',(0.334702023936276,2.4952218784915,110.118537734943));
#35781=CARTESIAN_POINT('Ctrl Pts',(0.305077306451513,2.49897131401624,110.120430429919));
#35782=CARTESIAN_POINT('Ctrl Pts',(0.294041102889617,2.50029390820895,110.121132632443));
#35783=CARTESIAN_POINT('Ctrl Pts',(0.271328371682351,2.50286337001245,110.122571975704));
#35784=CARTESIAN_POINT('Ctrl Pts',(0.259651139208311,2.50410172070423,110.123308833754));
#35785=CARTESIAN_POINT('Ctrl Pts',(0.232494453781475,2.50678963564373,110.125015376843));
#35786=CARTESIAN_POINT('Ctrl Pts',(0.217009280925179,2.50817761282148,110.125983121273));
#35787=CARTESIAN_POINT('Ctrl Pts',(0.167147064172982,2.51218165558898,110.129082822464));
#35788=CARTESIAN_POINT('Ctrl Pts',(0.132727917554875,2.51423512964181,110.131197344345));
#35789=CARTESIAN_POINT('Ctrl Pts',(0.0513909479018113,2.5174127185878,110.136142727679));
#35790=CARTESIAN_POINT('Ctrl Pts',(0.00446189482594016,2.51793333820691,
110.138955587364));
#35791=CARTESIAN_POINT('Ctrl Pts',(-0.270322207029544,2.5132985785105,110.15525326836));
#35792=CARTESIAN_POINT('Ctrl Pts',(-0.496585165582177,2.47853447527572,
110.167872582218));
#35793=CARTESIAN_POINT('Ctrl Pts',(-0.77294120111929,2.39666673196435,110.184961338577));
#35794=CARTESIAN_POINT('Ctrl Pts',(-0.830174527957854,2.37744790123484,
110.188603487654));
#35795=CARTESIAN_POINT('Ctrl Pts',(-0.899256002207809,2.35145191526845,
110.19318940675));
#35796=CARTESIAN_POINT('Ctrl Pts',(-0.911816598428019,2.34660988226944,
110.194031062936));
#35797=CARTESIAN_POINT('Ctrl Pts',(-0.931416421807931,2.33887315164513,
110.195357595893));
#35798=CARTESIAN_POINT('Ctrl Pts',(-0.938482591291469,2.33604678731531,
110.195838543262));
#35799=CARTESIAN_POINT('Ctrl Pts',(-0.951528148091245,2.33076001336847,
110.196731668242));
#35800=CARTESIAN_POINT('Ctrl Pts',(-0.957510980919255,2.32830856517606,
110.197143314625));
#35801=CARTESIAN_POINT('Ctrl Pts',(-0.971124928183119,2.32266894361101,
110.198084663355));
#35802=CARTESIAN_POINT('Ctrl Pts',(-0.978749804297957,2.31946620232442,
110.198615217839));
#35803=CARTESIAN_POINT('Ctrl Pts',(-1.00207311581661,2.30953403266787,110.200248008988));
#35804=CARTESIAN_POINT('Ctrl Pts',(-1.01771859107161,2.30268252466107,110.201357113242));
#35805=CARTESIAN_POINT('Ctrl Pts',(-1.05436616772552,2.28618728436905,110.203985658807));
#35806=CARTESIAN_POINT('Ctrl Pts',(-1.07530732243676,2.27641261571774,110.205511582211));
#35807=CARTESIAN_POINT('Ctrl Pts',(-1.14905385211283,2.24074545575631,110.210963253567));
#35808=CARTESIAN_POINT('Ctrl Pts',(-1.20108085237109,2.21329366978944,110.214952362949));
#35809=CARTESIAN_POINT('Ctrl Pts',(-1.4063694961024,2.09560346987792,110.231153431149));
#35810=CARTESIAN_POINT('Ctrl Pts',(-1.55085631513265,1.99105094290367,110.243579060927));
#35811=CARTESIAN_POINT('Ctrl Pts',(-1.74906870344958,1.81285123428931,110.261515451035));
#35812=CARTESIAN_POINT('Ctrl Pts',(-1.81184466034434,1.75011226518961,110.267366783505));
#35813=CARTESIAN_POINT('Ctrl Pts',(-1.88624639705353,1.66744945425621,110.274523852778));
#35814=CARTESIAN_POINT('Ctrl Pts',(-1.90108360634812,1.65051335298086,110.275963399404));
#35815=CARTESIAN_POINT('Ctrl Pts',(-1.92423450504423,1.62336107290992,110.278229941457));
#35816=CARTESIAN_POINT('Ctrl Pts',(-1.93269838498003,1.6132751057523,110.279063049797));
#35817=CARTESIAN_POINT('Ctrl Pts',(-1.94774475117345,1.5950567637726,110.280552362701));
#35818=CARTESIAN_POINT('Ctrl Pts',(-1.95435635505879,1.58694893999044,110.281209731729));
#35819=CARTESIAN_POINT('Ctrl Pts',(-1.96971792895204,1.5678694014886,110.282744165839));
#35820=CARTESIAN_POINT('Ctrl Pts',(-1.97842713849519,1.55686519970285,110.283619595965));
#35821=CARTESIAN_POINT('Ctrl Pts',(-2.00337651649327,1.52479385868837,110.286143999506));
#35822=CARTESIAN_POINT('Ctrl Pts',(-2.01937569930384,1.50354103564462,110.287783546316));
#35823=CARTESIAN_POINT('Ctrl Pts',(-2.09140652708025,1.40463311715435,110.295268923289));
#35824=CARTESIAN_POINT('Ctrl Pts',(-2.14331893088709,1.32407035491419,110.300958584952));
#35825=CARTESIAN_POINT('Ctrl Pts',(-2.2573087540372,1.12282171676607,110.314467186735));
#35826=CARTESIAN_POINT('Ctrl Pts',(-2.31446337576209,0.999713246903394,
110.322160480437));
#35827=CARTESIAN_POINT('Ctrl Pts',(-2.36143112015948,0.872610631806857,
110.330000354267));
#35828=CARTESIAN_POINT('Origin',(0.,0.,104.));
#35829=CARTESIAN_POINT('',(-2.36143104183299,0.872610843771477,111.329984892853));
#35830=CARTESIAN_POINT('',(-2.36143112101025,0.872610629504508,111.056268151607));
#35831=CARTESIAN_POINT('',(-2.36143112101026,0.872610629504505,104.));
#35832=CARTESIAN_POINT('',(-2.51749981257983,0.000971421916385074,110.112583302448));
#35833=CARTESIAN_POINT('Ctrl Pts',(-2.36143112101026,0.872610629504506,
111.056268151607));
#35834=CARTESIAN_POINT('Ctrl Pts',(-2.33290162629547,0.94981624035577,111.051081932139));
#35835=CARTESIAN_POINT('Ctrl Pts',(-2.30059282193492,1.02559131211717,111.04589571267));
#35836=CARTESIAN_POINT('Ctrl Pts',(-2.26468631750998,1.09954633066692,111.040709493202));
#35837=CARTESIAN_POINT('Ctrl Pts',(-2.22876338451224,1.17353518641205,111.035520900843));
#35838=CARTESIAN_POINT('Ctrl Pts',(-2.18923970143173,1.24570191647689,111.030332308485));
#35839=CARTESIAN_POINT('Ctrl Pts',(-2.14634234083047,1.31568263876908,111.025143716127));
#35840=CARTESIAN_POINT('Ctrl Pts',(-2.10336877650249,1.38578767621173,111.019945906649));
#35841=CARTESIAN_POINT('Ctrl Pts',(-2.05700982965078,1.4536985579788,111.014748097172));
#35842=CARTESIAN_POINT('Ctrl Pts',(-2.0075351419556,1.51908159880018,111.009550287694));
#35843=CARTESIAN_POINT('Ctrl Pts',(-1.96219405170571,1.57900190335994,111.004786753863));
#35844=CARTESIAN_POINT('Ctrl Pts',(-1.91423677985947,1.6367993045682,111.000023220032));
#35845=CARTESIAN_POINT('Ctrl Pts',(-1.86389785842549,1.69224437459749,110.995259686201));
#35846=CARTESIAN_POINT('Ctrl Pts',(-1.80836270405406,1.75341275952704,110.990004436801));
#35847=CARTESIAN_POINT('Ctrl Pts',(-1.74971071445244,1.81195742648223,110.984749187401));
#35848=CARTESIAN_POINT('Ctrl Pts',(-1.68821951860107,1.8675441379026,110.979493938002));
#35849=CARTESIAN_POINT('Ctrl Pts',(-1.62681550329481,1.92305203999531,110.974246139351));
#35850=CARTESIAN_POINT('Ctrl Pts',(-1.56258061669531,1.97561000963871,110.968998340701));
#35851=CARTESIAN_POINT('Ctrl Pts',(-1.49583108495485,2.02491866880692,110.963750542051));
#35852=CARTESIAN_POINT('Ctrl Pts',(-1.42859789519625,2.07458461180543,110.958464718566));
#35853=CARTESIAN_POINT('Ctrl Pts',(-1.35881378352396,2.12095360666406,110.953178895081));
#35854=CARTESIAN_POINT('Ctrl Pts',(-1.28683794339329,2.16375931134757,110.947893071597));
#35855=CARTESIAN_POINT('Ctrl Pts',(-1.21550750577025,2.20618118016209,110.942654645735));
#35856=CARTESIAN_POINT('Ctrl Pts',(-1.14202489231661,2.24510316621814,110.937416219873));
#35857=CARTESIAN_POINT('Ctrl Pts',(-1.06676945843396,2.28030900812861,110.932177794011));
#35858=CARTESIAN_POINT('Ctrl Pts',(-0.991538774808701,2.31550327142471,
110.926941090981));
#35859=CARTESIAN_POINT('Ctrl Pts',(-0.914536846343273,2.3469836225186,110.92170438795));
#35860=CARTESIAN_POINT('Ctrl Pts',(-0.836166345684795,2.37458040342797,
110.916467684919));
#35861=CARTESIAN_POINT('Ctrl Pts',(-0.757797979796856,2.40217643261578,
110.911231124533));
#35862=CARTESIAN_POINT('Ctrl Pts',(-0.678061551404548,2.42588894966515,
110.905994564147));
#35863=CARTESIAN_POINT('Ctrl Pts',(-0.597377051956488,2.44559745416039,
110.900758003761));
#35864=CARTESIAN_POINT('Ctrl Pts',(-0.515371964515496,2.46562853380418,
110.895435734983));
#35865=CARTESIAN_POINT('Ctrl Pts',(-0.432387965843948,2.48152321912133,
110.890113466204));
#35866=CARTESIAN_POINT('Ctrl Pts',(-0.348877286043428,2.49320895419597,
110.884791197426));
#35867=CARTESIAN_POINT('Ctrl Pts',(-0.266593439415926,2.50472301724645,
110.879547116681));
#35868=CARTESIAN_POINT('Ctrl Pts',(-0.183798755238067,2.51215099361981,
110.874303035937));
#35869=CARTESIAN_POINT('Ctrl Pts',(-0.100929632115851,2.51547599061509,
110.869058955193));
#35870=CARTESIAN_POINT('Ctrl Pts',(-0.0162071697278075,2.51887535001771,
110.863697592397));
#35871=CARTESIAN_POINT('Ctrl Pts',(0.0685925893749563,2.51798599741062,
110.858336229601));
#35872=CARTESIAN_POINT('Ctrl Pts',(0.153006789672422,2.51284603036361,110.852974866805));
#35873=CARTESIAN_POINT('Ctrl Pts',(0.237420989969885,2.5077060633166,110.847613504009));
#35874=CARTESIAN_POINT('Ctrl Pts',(0.321449133917394,2.49831560464582,110.842252141214));
#35875=CARTESIAN_POINT('Ctrl Pts',(0.40463942722808,2.48476823545628,110.836890778418));
#35876=CARTESIAN_POINT('Ctrl Pts',(0.486183197812372,2.47148899912655,110.831635529032));
#35877=CARTESIAN_POINT('Ctrl Pts',(0.567223179826133,2.4541668981303,110.826380279646));
#35878=CARTESIAN_POINT('Ctrl Pts',(0.647327861852357,2.43285282934863,110.82112503026));
#35879=CARTESIAN_POINT('Ctrl Pts',(0.727318973630284,2.41156897907633,110.815877231624));
#35880=CARTESIAN_POINT('Ctrl Pts',(0.806376977142961,2.38630452049806,110.810629432989));
#35881=CARTESIAN_POINT('Ctrl Pts',(0.884078586591063,2.35716170483299,110.805381634353));
#35882=CARTESIAN_POINT('Ctrl Pts',(0.962343211590781,2.32780772419264,110.800095810864));
#35883=CARTESIAN_POINT('Ctrl Pts',(1.03923123535665,2.29451902136058,110.794809987376));
#35884=CARTESIAN_POINT('Ctrl Pts',(1.11432368880329,2.25745187469674,110.789524163888));
#35885=CARTESIAN_POINT('Ctrl Pts',(1.18874279300605,2.22071710677448,110.784285738042));
#35886=CARTESIAN_POINT('Ctrl Pts',(1.26139797806441,2.18027159375407,110.779047312196));
#35887=CARTESIAN_POINT('Ctrl Pts',(1.33190130495525,2.13631579216616,110.77380888635));
#35888=CARTESIAN_POINT('Ctrl Pts',(1.40238144447153,2.09237444691215,110.768572183335));
#35889=CARTESIAN_POINT('Ctrl Pts',(1.47071074012569,2.04492534986803,110.76333548032));
#35890=CARTESIAN_POINT('Ctrl Pts',(1.53652764835991,1.9942138891868,110.758098777306));
#35891=CARTESIAN_POINT('Ctrl Pts',(1.60234276377146,1.94350380986272,110.752862216936));
#35892=CARTESIAN_POINT('Ctrl Pts',(1.66564526295127,1.88953182602826,110.747625656567));
#35893=CARTESIAN_POINT('Ctrl Pts',(1.72610540608032,1.83258461662764,110.742389096198));
#35894=CARTESIAN_POINT('Ctrl Pts',(1.7875551193565,1.7747053343693,110.737066827401));
#35895=CARTESIAN_POINT('Ctrl Pts',(1.84606822671548,1.71375288254076,110.731744558604));
#35896=CARTESIAN_POINT('Ctrl Pts',(1.90133765142355,1.65006708508447,110.726422289807));
#35897=CARTESIAN_POINT('Ctrl Pts',(1.95579512735124,1.58731687915724,110.72117820908));
#35898=CARTESIAN_POINT('Ctrl Pts',(2.00710335162121,1.52191351037076,110.715934128353));
#35899=CARTESIAN_POINT('Ctrl Pts',(2.05501055686366,1.45421382924896,110.710690047626));
#35900=CARTESIAN_POINT('Ctrl Pts',(2.10398919067139,1.38500006748214,110.705328684794));
#35901=CARTESIAN_POINT('Ctrl Pts',(2.1494125701995,1.31338647383459,110.699967321962));
#35902=CARTESIAN_POINT('Ctrl Pts',(2.19106064897833,1.23978203023703,110.694605959129));
#35903=CARTESIAN_POINT('Ctrl Pts',(2.23270872775716,1.16617758663948,110.689244596297));
#35904=CARTESIAN_POINT('Ctrl Pts',(2.27058133791497,1.09058277729602,110.683883233465));
#35905=CARTESIAN_POINT('Ctrl Pts',(2.30451099445111,1.01342751415874,110.678521870633));
#35906=CARTESIAN_POINT('Ctrl Pts',(2.33776910688383,0.93779932695729,110.673266621212));
#35907=CARTESIAN_POINT('Ctrl Pts',(2.36736180708549,0.860392569738316,110.668011371791));
#35908=CARTESIAN_POINT('Ctrl Pts',(2.39309684990577,0.781596901843338,110.66275612237));
#35909=CARTESIAN_POINT('Ctrl Pts',(2.41879540628265,0.70291294830205,110.657508323699));
#35910=CARTESIAN_POINT('Ctrl Pts',(2.44064702680772,0.622844430370973,110.652260525027));
#35911=CARTESIAN_POINT('Ctrl Pts',(2.45850702040397,0.541802067755736,110.647012726356));
#35912=CARTESIAN_POINT('Ctrl Pts',(2.47649642499183,0.460172483624873,110.641726902876));
#35913=CARTESIAN_POINT('Ctrl Pts',(2.49043592227857,0.377555316375038,110.636441079397));
#35914=CARTESIAN_POINT('Ctrl Pts',(2.50022848898027,0.294387080034804,110.631155255918));
#35915=CARTESIAN_POINT('Ctrl Pts',(2.50993324644491,0.211964607252194,110.625916830035));
#35916=CARTESIAN_POINT('Ctrl Pts',(2.51556509096039,0.129001375289329,110.620678404152));
#35917=CARTESIAN_POINT('Ctrl Pts',(2.51708094991472,0.0459319232824279,
110.615439978269));
#35918=CARTESIAN_POINT('Ctrl Pts',(2.51859631032829,-0.0371102085658783,
110.610203275217));
#35919=CARTESIAN_POINT('Ctrl Pts',(2.51599836524963,-0.120258030097391,
110.604966572166));
#35920=CARTESIAN_POINT('Ctrl Pts',(2.50929610141724,-0.203074679397106,
110.599729869114));
#35921=CARTESIAN_POINT('Ctrl Pts',(2.50259402015106,-0.285889072814097,
110.594493308707));
#35922=CARTESIAN_POINT('Ctrl Pts',(2.49178788066565,-0.368371852101413,
110.5892567483));
#35923=CARTESIAN_POINT('Ctrl Pts',(2.47693861969188,-0.450090351239497,
110.584020187894));
#35924=CARTESIAN_POINT('Ctrl Pts',(2.46184631643197,-0.533146361441927,
110.57869791914));
#35925=CARTESIAN_POINT('Ctrl Pts',(2.44257742264818,-0.615412361223516,
110.573375650386));
#35926=CARTESIAN_POINT('Ctrl Pts',(2.41924979163227,-0.696445759328899,
110.568053381633));
#35927=CARTESIAN_POINT('Ctrl Pts',(2.39626486043877,-0.776288718031306,
110.562809300868));
#35928=CARTESIAN_POINT('Ctrl Pts',(2.36933986167899,-0.854934627375409,
110.557565220103));
#35929=CARTESIAN_POINT('Ctrl Pts',(2.33863704368428,-0.931978019004564,
110.552321139338));
#35930=CARTESIAN_POINT('Ctrl Pts',(2.30724756818869,-1.01074445842575,110.54695977659));
#35931=CARTESIAN_POINT('Ctrl Pts',(2.27190946861718,-1.08783537024603,110.541598413842));
#35932=CARTESIAN_POINT('Ctrl Pts',(2.2328459912008,-1.16284351035662,110.536237051094));
#35933=CARTESIAN_POINT('Ctrl Pts',(2.19378251378443,-1.2378516504672,110.530875688346));
#35934=CARTESIAN_POINT('Ctrl Pts',(2.15099397327178,-1.31077661443296,110.525514325597));
#35935=CARTESIAN_POINT('Ctrl Pts',(2.10474978900411,-1.38124385091379,110.520152962849));
#35936=CARTESIAN_POINT('Ctrl Pts',(2.05942088042597,-1.45031638340145,110.514897713444));
#35937=CARTESIAN_POINT('Ctrl Pts',(2.01060448164522,-1.51728274163174,110.509642464039));
#35938=CARTESIAN_POINT('Ctrl Pts',(1.95852276773595,-1.5817695212198,110.504387214633));
#35939=CARTESIAN_POINT('Ctrl Pts',(1.90651489386549,-1.646164873204,110.499139415978));
#35940=CARTESIAN_POINT('Ctrl Pts',(1.85125118785159,-1.70808727334008,110.493891617323));
#35941=CARTESIAN_POINT('Ctrl Pts',(1.79299738092891,-1.76719173888463,110.488643818667));
#35942=CARTESIAN_POINT('Ctrl Pts',(1.73432147492567,-1.82672446726521,110.483357995184));
#35943=CARTESIAN_POINT('Ctrl Pts',(1.67261221345808,-1.8833978558186,110.4780721717));
#35944=CARTESIAN_POINT('Ctrl Pts',(1.60818291664799,-1.9368928614153,110.472786348217));
#35945=CARTESIAN_POINT('Ctrl Pts',(1.5443313529261,-1.98990818096363,110.46754792235));
#35946=CARTESIAN_POINT('Ctrl Pts',(1.47780870077296,-2.03980158975459,110.462309496484));
#35947=CARTESIAN_POINT('Ctrl Pts',(1.4089559973102,-2.08630037330285,110.457071070617));
#35948=CARTESIAN_POINT('Ctrl Pts',(1.34012593835553,-2.1327838641752,110.451834367582));
#35949=CARTESIAN_POINT('Ctrl Pts',(1.26896773212161,-2.17587468907029,110.446597664546));
#35950=CARTESIAN_POINT('Ctrl Pts',(1.19585270785378,-2.21534253584379,110.441360961511));
#35951=CARTESIAN_POINT('Ctrl Pts',(1.12273967520259,-2.2548093075329,110.43612440112));
#35952=CARTESIAN_POINT('Ctrl Pts',(1.04767033702651,-2.29065307904286,110.43088784073));
#35953=CARTESIAN_POINT('Ctrl Pts',(0.971040787340695,-2.32268939794385,
110.42565128034));
#35954=CARTESIAN_POINT('Ctrl Pts',(0.893157018421006,-2.35525006505663,
110.420329011567));
#35955=CARTESIAN_POINT('Ctrl Pts',(0.813661952898577,-2.38387731782439,
110.415006742794));
#35956=CARTESIAN_POINT('Ctrl Pts',(0.732990998319023,-2.40842904117669,
110.409684474021));
#35957=CARTESIAN_POINT('Ctrl Pts',(0.653505159118581,-2.4326200817395,110.404440393273));
#35958=CARTESIAN_POINT('Ctrl Pts',(0.572878219751572,-2.45285448865618,
110.399196312524));
#35959=CARTESIAN_POINT('Ctrl Pts',(0.49153862030256,-2.46904759669615,110.393952231776));
#35960=CARTESIAN_POINT('Ctrl Pts',(0.408379889083523,-2.4856028579492,110.388590868991));
#35961=CARTESIAN_POINT('Ctrl Pts',(0.324476742934424,-2.49793380011266,
110.383229506206));
#35962=CARTESIAN_POINT('Ctrl Pts',(0.240292321842426,-2.50600595571191,
110.37786814342));
#35963=CARTESIAN_POINT('Ctrl Pts',(0.156107900750426,-2.51407811131116,
110.372506780635));
#35964=CARTESIAN_POINT('Ctrl Pts',(0.0716427153179948,-2.51789152415955,
110.36714541785));
#35965=CARTESIAN_POINT('Ctrl Pts',(-0.0126423778882081,-2.51746825606229,
110.361784055065));
#35966=CARTESIAN_POINT('Ctrl Pts',(-0.095259280281888,-2.5170533653889,
110.35652880566));
#35967=CARTESIAN_POINT('Ctrl Pts',(-0.178008309443103,-2.51256648497769,
110.351273556255));
#35968=CARTESIAN_POINT('Ctrl Pts',(-0.260455293088755,-2.50399067296627,
110.34601830685));
#35969=CARTESIAN_POINT('Ctrl Pts',(-0.342785385640271,-2.49542701950819,
110.340770508195));
#35970=CARTESIAN_POINT('Ctrl Pts',(-0.424813828153972,-2.48278599667312,
110.33552270954));
#35971=CARTESIAN_POINT('Ctrl Pts',(-0.506106573980688,-2.46610267137715,
110.330274910885));
#35972=CARTESIAN_POINT('Ctrl Pts',(-0.587988355880546,-2.44929846099704,
110.324989087401));
#35973=CARTESIAN_POINT('Ctrl Pts',(-0.669123260711364,-2.42839312342264,
110.319703263918));
#35974=CARTESIAN_POINT('Ctrl Pts',(-0.749073089927936,-2.40347576562482,
110.314417440434));
#35975=CARTESIAN_POINT('Ctrl Pts',(-0.828306014497535,-2.37878184006907,
110.309179014568));
#35976=CARTESIAN_POINT('Ctrl Pts',(-0.906374582676004,-2.35014769695937,
110.303940588702));
#35977=CARTESIAN_POINT('Ctrl Pts',(-0.982864365463725,-2.31771091577478,
110.298702162836));
#35978=CARTESIAN_POINT('Ctrl Pts',(-1.05932899203433,-2.28528480250793,
110.293465459801));
#35979=CARTESIAN_POINT('Ctrl Pts',(-1.13421543997866,-2.24905871497737,
110.288228756766));
#35980=CARTESIAN_POINT('Ctrl Pts',(-1.20712835445952,-2.20921872748261,
110.282992053731));
#35981=CARTESIAN_POINT('Ctrl Pts',(-1.28003928282855,-2.16937982520944,
110.277755493342));
#35982=CARTESIAN_POINT('Ctrl Pts',(-1.35097638019609,-2.12592744085146,
110.272518932952));
#35983=CARTESIAN_POINT('Ctrl Pts',(-1.41956927528209,-2.0790933895992,110.267282372562));
#35984=CARTESIAN_POINT('Ctrl Pts',(-1.48928485123735,-2.03149279112211,
110.261960103789));
#35985=CARTESIAN_POINT('Ctrl Pts',(-1.55657838253628,-1.98039909590352,
110.256637835015));
#35986=CARTESIAN_POINT('Ctrl Pts',(-1.62109360583593,-1.92610014566166,
110.251315566242));
#35987=CARTESIAN_POINT('Ctrl Pts',(-1.6846610532615,-1.87259888676139,110.246071485494));
#35988=CARTESIAN_POINT('Ctrl Pts',(-1.74553098067731,-1.81598628647952,
110.240827404746));
#35989=CARTESIAN_POINT('Ctrl Pts',(-1.80339910666816,-1.75657562093651,
110.235583323999));
#35990=CARTESIAN_POINT('Ctrl Pts',(-1.86256143313221,-1.69583625656073,
110.230221961212));
#35991=CARTESIAN_POINT('Ctrl Pts',(-1.91858573120319,-1.63217254555964,
110.224860598426));
#35992=CARTESIAN_POINT('Ctrl Pts',(-1.97119093253988,-1.56595420031129,
110.21949923564));
#35993=CARTESIAN_POINT('Ctrl Pts',(-2.02379613387657,-1.49973585506294,
110.214137872853));
#35994=CARTESIAN_POINT('Ctrl Pts',(-2.07298199723095,-1.43096332771099,
110.208776510067));
#35995=CARTESIAN_POINT('Ctrl Pts',(-2.11851611379751,-1.36003519277271,
110.203415147281));
#35996=CARTESIAN_POINT('Ctrl Pts',(-2.16415197863569,-1.28894856535267,
110.19804180426));
#35997=CARTESIAN_POINT('Ctrl Pts',(-2.20628267264359,-1.21544362347196,
110.192668461239));
#35998=CARTESIAN_POINT('Ctrl Pts',(-2.24465002135591,-1.13989145607242,
110.187295118218));
#35999=CARTESIAN_POINT('Ctrl Pts',(-2.28295541755198,-1.0644612842508,110.18193045164));
#36000=CARTESIAN_POINT('Ctrl Pts',(-2.317509353925,-0.986990841980724,110.176565785063));
#36001=CARTESIAN_POINT('Ctrl Pts',(-2.34809743268924,-0.907879230183296,
110.171201118485));
#36002=CARTESIAN_POINT('Ctrl Pts',(-2.37863368161104,-0.828901668726391,
110.165845542044));
#36003=CARTESIAN_POINT('Ctrl Pts',(-2.40521729335624,-0.74828887520221,
110.160489965604));
#36004=CARTESIAN_POINT('Ctrl Pts',(-2.42768086911504,-0.666462187774268,
110.155134389163));
#36005=CARTESIAN_POINT('Ctrl Pts',(-2.45012200377272,-0.584717245166741,
110.14978416294));
#36006=CARTESIAN_POINT('Ctrl Pts',(-2.46845116952332,-0.501761235536918,
110.144433936718));
#36007=CARTESIAN_POINT('Ctrl Pts',(-2.48255009884958,-0.418032602439035,
110.139083710495));
#36008=CARTESIAN_POINT('Ctrl Pts',(-2.49663704236547,-0.334375148896358,
110.133738032618));
#36009=CARTESIAN_POINT('Ctrl Pts',(-2.50650083249334,-0.249946805333563,
110.12839235474));
#36010=CARTESIAN_POINT('Ctrl Pts',(-2.51207407896376,-0.165197069581622,
110.123046676863));
#36011=CARTESIAN_POINT('Ctrl Pts',(-2.5157103477164,-0.10990204224983,110.119558885406));
#36012=CARTESIAN_POINT('Ctrl Pts',(-2.51752120578779,-0.0544704357890657,
110.116071093949));
#36013=CARTESIAN_POINT('Ctrl Pts',(-2.5174998125801,0.000971421219968912,
110.112583302492));
#36014=CARTESIAN_POINT('Ctrl Pts',(-2.51749981257983,0.000971421916383455,
110.112583302448));
#36015=CARTESIAN_POINT('Ctrl Pts',(-2.5174649075931,0.0914298479257806,
110.106892653857));
#36016=CARTESIAN_POINT('Ctrl Pts',(-2.51255029658571,0.181738101408035,
110.101202005267));
#36017=CARTESIAN_POINT('Ctrl Pts',(-2.50282943169604,0.27138733543788,110.095511356676));
#36018=CARTESIAN_POINT('Ctrl Pts',(-2.49308231405315,0.361278681588806,
110.089805339577));
#36019=CARTESIAN_POINT('Ctrl Pts',(-2.47850306961473,0.450507135567614,
110.084099322478));
#36020=CARTESIAN_POINT('Ctrl Pts',(-2.45921603044753,0.538574753947772,
110.07839330538));
#36021=CARTESIAN_POINT('Ctrl Pts',(-2.43985726985429,0.626969863505942,
110.072666069695));
#36022=CARTESIAN_POINT('Ctrl Pts',(-2.41575577495363,0.71419518908884,110.066938834011));
#36023=CARTESIAN_POINT('Ctrl Pts',(-2.38708590651013,0.799766919133763,
110.061211598327));
#36024=CARTESIAN_POINT('Ctrl Pts',(-2.37890445742615,0.824186311004028,
110.059577231318));
#36025=CARTESIAN_POINT('Ctrl Pts',(-2.37035127937335,0.848471180762149,
110.057942864309));
#36026=CARTESIAN_POINT('Ctrl Pts',(-2.36143112101026,0.872610629504504,
110.0563084973));
#36027=CARTESIAN_POINT('',(-2.51749930920945,0.00210565722249706,110.386763667368));
#36028=CARTESIAN_POINT('Ctrl Pts',(-2.36143112015948,0.872610631806858,
110.330000354267));
#36029=CARTESIAN_POINT('Ctrl Pts',(-2.36296399590596,0.868462412246907,
110.330256222472));
#36030=CARTESIAN_POINT('Ctrl Pts',(-2.36448602047482,0.86430993896747,110.330512261035));
#36031=CARTESIAN_POINT('Ctrl Pts',(-2.40316528250013,0.757916079188607,
110.337070542764));
#36032=CARTESIAN_POINT('Ctrl Pts',(-2.4336632123791,0.653389373353525,110.343466229615));
#36033=CARTESIAN_POINT('Ctrl Pts',(-2.46029282490902,0.533811334540226,
110.351057984404));
#36034=CARTESIAN_POINT('Ctrl Pts',(-2.46317169506485,0.520365742903747,
110.351915497782));
#36035=CARTESIAN_POINT('Ctrl Pts',(-2.46763513881816,0.498652115547464,
110.353307551631));
#36036=CARTESIAN_POINT('Ctrl Pts',(-2.46928867943535,0.490398331419059,
110.353838378079));
#36037=CARTESIAN_POINT('Ctrl Pts',(-2.47214998174644,0.475734448201513,
110.354784684309));
#36038=CARTESIAN_POINT('Ctrl Pts',(-2.47337426686735,0.469327744784659,
110.355199229615));
#36039=CARTESIAN_POINT('Ctrl Pts',(-2.47598044322707,0.455396119768616,
110.356103126194));
#36040=CARTESIAN_POINT('Ctrl Pts',(-2.47735291470224,0.447869750556951,
110.356592971902));
#36041=CARTESIAN_POINT('Ctrl Pts',(-2.48011967607558,0.432295449558692,
110.357609601127));
#36042=CARTESIAN_POINT('Ctrl Pts',(-2.48150914672819,0.42424676048847,110.358136636322));
#36043=CARTESIAN_POINT('Ctrl Pts',(-2.48498571496911,0.403506720311722,
110.359498706434));
#36044=CARTESIAN_POINT('Ctrl Pts',(-2.48701473576366,0.390806045783101,
110.360336647044));
#36045=CARTESIAN_POINT('Ctrl Pts',(-2.50785197421962,0.253635865350339,
110.369424037005));
#36046=CARTESIAN_POINT('Ctrl Pts',(-2.51739394917129,0.127954017128451,
110.378073632483));
#36047=CARTESIAN_POINT('Ctrl Pts',(-2.51749912091712,0.0021038492205399,
110.386763463131));
#36048=CARTESIAN_POINT('Ctrl Pts',(-2.51749911942459,0.0021056344473654,
110.386763339863));
#36049=CARTESIAN_POINT('Ctrl Pts',(-2.51764329833865,-0.170274851464046,
110.398666042829));
#36050=CARTESIAN_POINT('Ctrl Pts',(-2.50008177033433,-0.342246676778853,
110.410566416665));
#36051=CARTESIAN_POINT('Ctrl Pts',(-2.45545670408571,-0.557478736267895,
110.42508713168));
#36052=CARTESIAN_POINT('Ctrl Pts',(-2.44453208447062,-0.603583914935035,
110.428178433417));
#36053=CARTESIAN_POINT('Ctrl Pts',(-2.42634831314994,-0.671695416985644,
110.432718035789));
#36054=CARTESIAN_POINT('Ctrl Pts',(-2.42007670117976,-0.693952223558913,
110.434197108021));
#36055=CARTESIAN_POINT('Ctrl Pts',(-2.40971649144246,-0.728868654455705,
110.436511272229));
#36056=CARTESIAN_POINT('Ctrl Pts',(-2.40583279957737,-0.741587241047874,
110.437352921095));
#36057=CARTESIAN_POINT('Ctrl Pts',(-2.39837042256289,-0.7653498034775,110.438923155181));
#36058=CARTESIAN_POINT('Ctrl Pts',(-2.39481578578661,-0.776400904761422,
110.439652497783));
#36059=CARTESIAN_POINT('Ctrl Pts',(-2.3866831242604,-0.801097406431204,
110.441280532335));
#36060=CARTESIAN_POINT('Ctrl Pts',(-2.38206424300593,-0.814729001574641,
110.442177864633));
#36061=CARTESIAN_POINT('Ctrl Pts',(-2.3700071018441,-0.849333708582673,
110.444452994953));
#36062=CARTESIAN_POINT('Ctrl Pts',(-2.36240711075495,-0.87024944861862,
110.445825475878));
#36063=CARTESIAN_POINT('Ctrl Pts',(-2.29794020685439,-1.04059591718973,
110.456988449925));
#36064=CARTESIAN_POINT('Ctrl Pts',(-2.22723159648514,-1.18440607317206,
110.466284810636));
#36065=CARTESIAN_POINT('Ctrl Pts',(-2.07236844857468,-1.43575982673904,
110.483272012167));
#36066=CARTESIAN_POINT('Ctrl Pts',(-1.99221931021569,-1.54504835624853,
110.490972141341));
#36067=CARTESIAN_POINT('Ctrl Pts',(-1.87882400547249,-1.67608769707031,
110.501278484627));
#36068=CARTESIAN_POINT('Ctrl Pts',(-1.85331782356258,-1.70424832738821,
110.503564715586));
#36069=CARTESIAN_POINT('Ctrl Pts',(-1.81009660686039,-1.74984960487127,
110.507408245809));
#36070=CARTESIAN_POINT('Ctrl Pts',(-1.79274241516079,-1.76762492956887,
110.508943793693));
#36071=CARTESIAN_POINT('Ctrl Pts',(-1.76842553870494,-1.79180543838547,
110.51108992227));
#36072=CARTESIAN_POINT('Ctrl Pts',(-1.76168490739144,-1.79843317789301,
110.51168426053));
#36073=CARTESIAN_POINT('Ctrl Pts',(-1.75003919197618,-1.80975555658372,
110.512710464341));
#36074=CARTESIAN_POINT('Ctrl Pts',(-1.74515207398136,-1.81446867838519,
110.513140922979));
#36075=CARTESIAN_POINT('Ctrl Pts',(-1.73583180624045,-1.82338462940491,
110.513961639012));
#36076=CARTESIAN_POINT('Ctrl Pts',(-1.73140231587304,-1.82759119744597,
110.514351591185));
#36077=CARTESIAN_POINT('Ctrl Pts',(-1.71965051990675,-1.83867049539541,
110.51538580572));
#36078=CARTESIAN_POINT('Ctrl Pts',(-1.71230241387873,-1.84551552054584,
110.516032107405));
#36079=CARTESIAN_POINT('Ctrl Pts',(-1.68598309736712,-1.86974041359636,
110.518345084864));
#36080=CARTESIAN_POINT('Ctrl Pts',(-1.66678734393684,-1.88687255747639,
110.520028479651));
#36081=CARTESIAN_POINT('Ctrl Pts',(-1.46354085495847,-2.06274771198428,
110.537785324103));
#36082=CARTESIAN_POINT('Ctrl Pts',(-1.25768649220713,-2.19433807223394,
110.555052539306));
#36083=CARTESIAN_POINT('Ctrl Pts',(-0.950715499486211,-2.33296668823648,
110.577757280399));
#36084=CARTESIAN_POINT('Ctrl Pts',(-0.863186945362496,-2.36674997844094,
110.583948379089));
#36085=CARTESIAN_POINT('Ctrl Pts',(-0.752984734023684,-2.40235436498814,
110.591397561033));
#36086=CARTESIAN_POINT('Ctrl Pts',(-0.731912822413238,-2.40885785707047,
110.592806967996));
#36087=CARTESIAN_POINT('Ctrl Pts',(-0.698223518727957,-2.41877259755477,
110.595037156421));
#36088=CARTESIAN_POINT('Ctrl Pts',(-0.685660703036756,-2.4223637983495,
110.59586372085));
#36089=CARTESIAN_POINT('Ctrl Pts',(-0.661854342247283,-2.42896903266096,
110.597420663598));
#36090=CARTESIAN_POINT('Ctrl Pts',(-0.65061678576954,-2.43200319435752,
110.598151672839));
#36091=CARTESIAN_POINT('Ctrl Pts',(-0.625097279860039,-2.43870396798316,
110.59980303306));
#36092=CARTESIAN_POINT('Ctrl Pts',(-0.610803268316554,-2.44232328629008,
110.600721848056));
#36093=CARTESIAN_POINT('Ctrl Pts',(-0.567178033251368,-2.45296246985002,
110.603508004502));
#36094=CARTESIAN_POINT('Ctrl Pts',(-0.537751086756829,-2.45958120165861,
110.60536258629));
#36095=CARTESIAN_POINT('Ctrl Pts',(-0.301082449323961,-2.50836213760925,
110.620097502664));
#36096=CARTESIAN_POINT('Ctrl Pts',(-0.0894038025816362,-2.52478641643537,
110.632078951845));
#36097=CARTESIAN_POINT('Ctrl Pts',(0.244908168020617,-2.50858624571339,
110.651378927812));
#36098=CARTESIAN_POINT('Ctrl Pts',(0.367347059302306,-2.49359848791987,
110.658553452984));
#36099=CARTESIAN_POINT('Ctrl Pts',(0.505768845967032,-2.46623713093697,
110.667263469902));
#36100=CARTESIAN_POINT('Ctrl Pts',(0.523319645846156,-2.46257268267309,
110.668379150227));
#36101=CARTESIAN_POINT('Ctrl Pts',(0.54907262591235,-2.45690796388606,110.670034909156));
#36102=CARTESIAN_POINT('Ctrl Pts',(0.557306715375849,-2.45505330118695,
110.670567132018));
#36103=CARTESIAN_POINT('Ctrl Pts',(0.571889187600747,-2.45169157515576,
110.671514951305));
#36104=CARTESIAN_POINT('Ctrl Pts',(0.57824124413233,-2.45020119271443,110.671929601588));
#36105=CARTESIAN_POINT('Ctrl Pts',(0.592013518152153,-2.44691326617059,
110.672832569946));
#36106=CARTESIAN_POINT('Ctrl Pts',(0.599431258679526,-2.44510668484646,
110.673321373505));
#36107=CARTESIAN_POINT('Ctrl Pts',(0.620008583542812,-2.43999584019113,
110.674683982924));
#36108=CARTESIAN_POINT('Ctrl Pts',(0.633149619978672,-2.4366189450218,110.675561722554));
#36109=CARTESIAN_POINT('Ctrl Pts',(0.706331848654608,-2.41718110067154,
110.680489642497));
#36110=CARTESIAN_POINT('Ctrl Pts',(0.765784781830726,-2.39900843149059,
110.684642638261));
#36111=CARTESIAN_POINT('Ctrl Pts',(0.992271495586989,-2.32050276135613,
110.700895299131));
#36112=CARTESIAN_POINT('Ctrl Pts',(1.153422131308,-2.24476232836648,110.713342448533));
#36113=CARTESIAN_POINT('Ctrl Pts',(1.40224111491262,-2.0938928176765,110.733116221043));
#36114=CARTESIAN_POINT('Ctrl Pts',(1.49514037930865,-2.02860266874869,110.740656443378));
#36115=CARTESIAN_POINT('Ctrl Pts',(1.60132042408556,-1.94270804358123,110.749451090932));
#36116=CARTESIAN_POINT('Ctrl Pts',(1.61910876371784,-1.9279078071364,110.750931251268));
#36117=CARTESIAN_POINT('Ctrl Pts',(1.64679788193825,-1.9042163523838,110.753246725604));
#36118=CARTESIAN_POINT('Ctrl Pts',(1.65683619805588,-1.89548859255138,110.754088608896));
#36119=CARTESIAN_POINT('Ctrl Pts',(1.67550441776598,-1.8789959933731,110.755659057023));
#36120=CARTESIAN_POINT('Ctrl Pts',(1.68415066144695,-1.8712502648957,110.756388381168));
#36121=CARTESIAN_POINT('Ctrl Pts',(1.70339261395467,-1.85377098068766,110.758016089393));
#36122=CARTESIAN_POINT('Ctrl Pts',(1.71395913390444,-1.8440057882232,110.758913116331));
#36123=CARTESIAN_POINT('Ctrl Pts',(1.74064159773811,-1.81891932352864,110.761186931874));
#36124=CARTESIAN_POINT('Ctrl Pts',(1.75663953666859,-1.80347394320802,110.76255841418));
#36125=CARTESIAN_POINT('Ctrl Pts',(1.87205792432113,-1.68904891988188,110.772519591715));
#36126=CARTESIAN_POINT('Ctrl Pts',(1.96326066391103,-1.58211946020137,110.780738609599));
#36127=CARTESIAN_POINT('Ctrl Pts',(2.15574901970139,-1.31398633388733,110.799790462211));
#36128=CARTESIAN_POINT('Ctrl Pts',(2.24861184733092,-1.14784146530307,110.810451683602));
#36129=CARTESIAN_POINT('Ctrl Pts',(2.33259982649779,-0.947389891033239,
110.823710363112));
#36130=CARTESIAN_POINT('Ctrl Pts',(2.3428557902465,-0.921735405158754,110.825414972068));
#36131=CARTESIAN_POINT('Ctrl Pts',(2.35625249026904,-0.886555599091831,
110.827769685938));
#36132=CARTESIAN_POINT('Ctrl Pts',(2.35976198099206,-0.877171598542212,
110.828399441413));
#36133=CARTESIAN_POINT('Ctrl Pts',(2.36555159457127,-0.861404575828846,
110.829460715437));
#36134=CARTESIAN_POINT('Ctrl Pts',(2.3678621656094,-0.855032720284201,110.82989046374));
#36135=CARTESIAN_POINT('Ctrl Pts',(2.37220971985199,-0.842890703919863,
110.830711151496));
#36136=CARTESIAN_POINT('Ctrl Pts',(2.37425144596497,-0.837122310732061,
110.831101794246));
#36137=CARTESIAN_POINT('Ctrl Pts',(2.37960687987857,-0.821814654359174,
110.83214033244));
#36138=CARTESIAN_POINT('Ctrl Pts',(2.38288421396437,-0.812262915249904,
110.832790298342));
#36139=CARTESIAN_POINT('Ctrl Pts',(2.39441755864728,-0.777978579479148,
110.835129504385));
#36140=CARTESIAN_POINT('Ctrl Pts',(2.40234637176346,-0.753138698998407,
110.836835946197));
#36141=CARTESIAN_POINT('Ctrl Pts',(2.48090624281213,-0.493147885579695,
110.854785551936));
#36142=CARTESIAN_POINT('Ctrl Pts',(2.51716358381374,-0.248987751820035,
110.872236167635));
#36143=CARTESIAN_POINT('Ctrl Pts',(2.5176216474378,0.0877017228365608,110.894904945598));
#36144=CARTESIAN_POINT('Ctrl Pts',(2.51279781121409,0.178776008820882,110.900917916456));
#36145=CARTESIAN_POINT('Ctrl Pts',(2.50070308824772,0.291151166824925,110.908186495869));
#36146=CARTESIAN_POINT('Ctrl Pts',(2.49807828607229,0.312873558370864,110.90958470036));
#36147=CARTESIAN_POINT('Ctrl Pts',(2.49343921493223,0.347472104184843,110.911801369078));
#36148=CARTESIAN_POINT('Ctrl Pts',(2.49160762867454,0.36037122088898,110.91262549553));
#36149=CARTESIAN_POINT('Ctrl Pts',(2.487949229522,0.384773333181392,110.914180387578));
#36150=CARTESIAN_POINT('Ctrl Pts',(2.48614257036175,0.396278959529849,110.914911763166));
#36151=CARTESIAN_POINT('Ctrl Pts',(2.48185764350168,0.422383893568352,110.916567367625));
#36152=CARTESIAN_POINT('Ctrl Pts',(2.47933026533961,0.436974789095167,110.917490028922));
#36153=CARTESIAN_POINT('Ctrl Pts',(2.47120631175511,0.481533992124443,110.920300074781));
#36154=CARTESIAN_POINT('Ctrl Pts',(2.46519388526105,0.511424336201167,110.922174370069));
#36155=CARTESIAN_POINT('Ctrl Pts',(2.41374593185286,0.745149747006543,110.936763458479));
#36156=CARTESIAN_POINT('Ctrl Pts',(2.34365232581276,0.94271933301619,110.948606305652));
#36157=CARTESIAN_POINT('Ctrl Pts',(2.19375913317683,1.24133829274307,110.967865195147));
#36158=CARTESIAN_POINT('Ctrl Pts',(2.12928795658594,1.348934648664,110.97515283595));
#36159=CARTESIAN_POINT('Ctrl Pts',(2.04673092243822,1.46595417215013,110.983992650407));
#36160=CARTESIAN_POINT('Ctrl Pts',(2.03621622391404,1.48052441740371,110.985110700126));
#36161=CARTESIAN_POINT('Ctrl Pts',(2.02053020003841,1.50177738913931,110.986769322118));
#36162=CARTESIAN_POINT('Ctrl Pts',(2.01547948648121,1.50854898843145,110.987301999782));
#36163=CARTESIAN_POINT('Ctrl Pts',(2.00646719936282,1.5205059055601,110.988250312824));
#36164=CARTESIAN_POINT('Ctrl Pts',(2.00251942084914,1.52570141204202,110.988664998259));
#36165=CARTESIAN_POINT('Ctrl Pts',(1.99391193254135,1.53693840630447,110.989567668675));
#36166=CARTESIAN_POINT('Ctrl Pts',(1.9892450181865,1.54297398340292,110.990056136251));
#36167=CARTESIAN_POINT('Ctrl Pts',(1.97621645630644,1.5596660691145,110.991416935954));
#36168=CARTESIAN_POINT('Ctrl Pts',(1.96779627073543,1.57027626454492,110.992293185582));
#36169=CARTESIAN_POINT('Ctrl Pts',(1.92044609161951,1.62896284405293,110.997200557076));
#36170=CARTESIAN_POINT('Ctrl Pts',(1.8798429750062,1.67565574524605,111.001333546881));
#36171=CARTESIAN_POINT('Ctrl Pts',(1.71599060106809,1.85062621329894,111.017584161762));
#36172=CARTESIAN_POINT('Ctrl Pts',(1.5809995624089,1.96720264391738,111.030052847615));
#36173=CARTESIAN_POINT('Ctrl Pts',(1.34163221489586,2.13323642262933,111.049849200214));
#36174=CARTESIAN_POINT('Ctrl Pts',(1.24414846610622,2.19152355668126,111.057391660969));
#36175=CARTESIAN_POINT('Ctrl Pts',(1.12243469940877,2.25354877002397,111.066188509777));
#36176=CARTESIAN_POINT('Ctrl Pts',(1.10167293224502,2.26377086341799,111.06766876876));
#36177=CARTESIAN_POINT('Ctrl Pts',(1.06875889310635,2.27941606945674,111.069984361724));
#36178=CARTESIAN_POINT('Ctrl Pts',(1.05669993667899,2.28503138800181,111.070826266126));
#36179=CARTESIAN_POINT('Ctrl Pts',(1.03403527199155,2.29536752013784,111.072396733316));
#36180=CARTESIAN_POINT('Ctrl Pts',(1.02344036850641,2.30011104418824,111.073126055589));
#36181=CARTESIAN_POINT('Ctrl Pts',(0.999641626306764,2.31056916188519,111.074753733701));
#36182=CARTESIAN_POINT('Ctrl Pts',(0.986420778775437,2.31624422151011,111.075650732627));
#36183=CARTESIAN_POINT('Ctrl Pts',(0.952645918878369,2.33040047278099,111.077924427997));
#36184=CARTESIAN_POINT('Ctrl Pts',(0.93202660782502,2.33872338272945,111.079295819125));
#36185=CARTESIAN_POINT('Ctrl Pts',(0.760783654652436,2.4052204919798,111.090554863484));
#36186=CARTESIAN_POINT('Ctrl Pts',(0.604987457403047,2.44905634527811,111.099937467251));
#36187=CARTESIAN_POINT('Ctrl Pts',(0.323164559339578,2.49979211058615,111.116410999687));
#36188=CARTESIAN_POINT('Ctrl Pts',(0.198813172750137,2.51274066839984,111.123526272158));
#36189=CARTESIAN_POINT('Ctrl Pts',(0.0305860775248409,2.51768924404162,
111.133481900247));
#36190=CARTESIAN_POINT('Ctrl Pts',(-0.0128741655536576,2.51784202757347,
111.136084261461));
#36191=CARTESIAN_POINT('Ctrl Pts',(-0.0840523629938136,2.51624944081131,
111.140427058072));
#36192=CARTESIAN_POINT('Ctrl Pts',(-0.111777184821294,2.51517032467341,
111.142138743466));
#36193=CARTESIAN_POINT('Ctrl Pts',(-0.149496912776967,2.51307732224715,
111.144501723648));
#36194=CARTESIAN_POINT('Ctrl Pts',(-0.159513051122024,2.51246144906779,
111.145132484003));
#36195=CARTESIAN_POINT('Ctrl Pts',(-0.176290874480291,2.511329082898,111.146194974938));
#36196=CARTESIAN_POINT('Ctrl Pts',(-0.183054766898247,2.51084511381333,
111.146624926254));
#36197=CARTESIAN_POINT('Ctrl Pts',(-0.195915258578477,2.50987267968945,
111.147445619513));
#36198=CARTESIAN_POINT('Ctrl Pts',(-0.202012179560194,2.50938931498974,
111.147836062298));
#36199=CARTESIAN_POINT('Ctrl Pts',(-0.216518914339997,2.5081860085542,111.148768222285));
#36200=CARTESIAN_POINT('Ctrl Pts',(-0.224926924535857,2.50744598497346,
111.149311024371));
#36201=CARTESIAN_POINT('Ctrl Pts',(-0.254757061301248,2.50466926907201,
111.15124539124));
#36202=CARTESIAN_POINT('Ctrl Pts',(-0.276155932536117,2.50240027495241,
111.152648777436));
#36203=CARTESIAN_POINT('Ctrl Pts',(-0.424750308401898,2.48471521378279,
111.162491659274));
#36204=CARTESIAN_POINT('Ctrl Pts',(-0.550624975280106,2.45988382505115,
111.171318960531));
#36205=CARTESIAN_POINT('Ctrl Pts',(-0.81232890958307,2.38715851098287,111.190081669048));
#36206=CARTESIAN_POINT('Ctrl Pts',(-0.947083159303446,2.33697358364249,
111.199981762439));
#36207=CARTESIAN_POINT('Ctrl Pts',(-1.14334995170638,2.24409714444885,111.214473325633));
#36208=CARTESIAN_POINT('Ctrl Pts',(-1.20845710557636,2.20971815671582,111.219297945602));
#36209=CARTESIAN_POINT('Ctrl Pts',(-1.28967573089423,2.16216643855821,111.225341380822));
#36210=CARTESIAN_POINT('Ctrl Pts',(-1.30725439326156,2.15158387958411,111.22665106952));
#36211=CARTESIAN_POINT('Ctrl Pts',(-1.33552819121489,2.13408827863243,111.228760821941));
#36212=CARTESIAN_POINT('Ctrl Pts',(-1.34630341301713,2.12730709120473,111.22956562949));
#36213=CARTESIAN_POINT('Ctrl Pts',(-1.36689747730258,2.11412744844487,111.231105494151));
#36214=CARTESIAN_POINT('Ctrl Pts',(-1.37672396433045,2.10774161490821,111.231840988625));
#36215=CARTESIAN_POINT('Ctrl Pts',(-1.39913027009237,2.0929571210878,111.233519978948));
#36216=CARTESIAN_POINT('Ctrl Pts',(-1.4116797841383,2.08451318685592,111.234461763272));
#36217=CARTESIAN_POINT('Ctrl Pts',(-1.45140864262269,2.05725830032516,111.237448430081));
#36218=CARTESIAN_POINT('Ctrl Pts',(-1.47829465102032,2.03802449499353,111.239477405331));
#36219=CARTESIAN_POINT('Ctrl Pts',(-1.64314642487512,1.91511298206485,111.251985100253));
#36220=CARTESIAN_POINT('Ctrl Pts',(-1.7705287216286,1.7980057007078,111.261906290343));
#36221=CARTESIAN_POINT('Ctrl Pts',(-1.94989840103383,1.59540149108219,111.277454413042));
#36222=CARTESIAN_POINT('Ctrl Pts',(-2.01051478956918,1.51830102061003,111.283080421963));
#36223=CARTESIAN_POINT('Ctrl Pts',(-2.09212920244327,1.40100620191224,111.29152201836));
#36224=CARTESIAN_POINT('Ctrl Pts',(-2.11678601996941,1.36346597643312,111.294208050461));
#36225=CARTESIAN_POINT('Ctrl Pts',(-2.1553800283297,1.3011342341153,111.298676752008));
#36226=CARTESIAN_POINT('Ctrl Pts',(-2.16992510023507,1.2767295187199,111.300428526105));
#36227=CARTESIAN_POINT('Ctrl Pts',(-2.18908971810314,1.24330004359021,111.302838287168));
#36228=CARTESIAN_POINT('Ctrl Pts',(-2.19407291621182,1.23448484091084,111.303474675938));
#36229=CARTESIAN_POINT('Ctrl Pts',(-2.20231328604422,1.21970024216596,111.304543992961));
#36230=CARTESIAN_POINT('Ctrl Pts',(-2.20559975925482,1.21374716914736,111.304975091204));
#36231=CARTESIAN_POINT('Ctrl Pts',(-2.21178839982244,1.20242901282071,111.305795857677));
#36232=CARTESIAN_POINT('Ctrl Pts',(-2.21469526273643,1.19706655945658,111.306185213192));
#36233=CARTESIAN_POINT('Ctrl Pts',(-2.22154739615755,1.18431565533583,111.307112075069));
#36234=CARTESIAN_POINT('Ctrl Pts',(-2.22547530924003,1.17691802946674,111.307650638592));
#36235=CARTESIAN_POINT('Ctrl Pts',(-2.23918245250679,1.15078873182618,111.309555463624));
#36236=CARTESIAN_POINT('Ctrl Pts',(-2.24876238074172,1.13195426011333,111.310933095378));
#36237=CARTESIAN_POINT('Ctrl Pts',(-2.29670992164692,1.03467635481964,111.318063501898));
#36238=CARTESIAN_POINT('Ctrl Pts',(-2.33119449209657,0.954436009772043,
111.323993087481));
#36239=CARTESIAN_POINT('Ctrl Pts',(-2.36143104183299,0.872610843771477,
111.329984892853));
#36240=CARTESIAN_POINT('Origin',(0.,0.,104.));
#36241=CARTESIAN_POINT('',(-2.36143112095426,0.872610629656035,112.333400434891));
#36242=CARTESIAN_POINT('',(-2.36143112101026,0.872610629504506,112.056167113269));
#36243=CARTESIAN_POINT('',(-2.36143112101026,0.872610629504505,104.));
#36244=CARTESIAN_POINT('',(-2.51749898697117,-0.00225845060319292,111.11258330253));
#36245=CARTESIAN_POINT('Ctrl Pts',(-2.36143112101026,0.872610629504506,
112.056167113269));
#36246=CARTESIAN_POINT('Ctrl Pts',(-2.33266408168154,0.950459076031816,
112.050928731472));
#36247=CARTESIAN_POINT('Ctrl Pts',(-2.30002250408097,1.02693994154336,112.045690349676));
#36248=CARTESIAN_POINT('Ctrl Pts',(-2.26366542465182,1.10164653824895,112.040451967879));
#36249=CARTESIAN_POINT('Ctrl Pts',(-2.22732008720791,1.1763290075007,112.035215277885));
#36250=CARTESIAN_POINT('Ctrl Pts',(-2.18726183293021,1.249237931436,112.029978587892));
#36251=CARTESIAN_POINT('Ctrl Pts',(-2.14369712875725,1.31998820834049,112.024741897898));
#36252=CARTESIAN_POINT('Ctrl Pts',(-2.10013335341261,1.39073697680224,112.019505319554));
#36253=CARTESIAN_POINT('Ctrl Pts',(-2.05306351968801,1.45932679740954,112.014268741209));
#36254=CARTESIAN_POINT('Ctrl Pts',(-2.00273846521359,1.52539991148351,112.009032162865));
#36255=CARTESIAN_POINT('Ctrl Pts',(-1.95183672119319,1.59223017673308,112.003735577035));
#36256=CARTESIAN_POINT('Ctrl Pts',(-1.89760495238244,1.6564852927305,111.998438991206));
#36257=CARTESIAN_POINT('Ctrl Pts',(-1.84034469218861,1.71782934656886,111.993142405376));
#36258=CARTESIAN_POINT('Ctrl Pts',(-1.78365150597444,1.77856588279169,111.987898274005));
#36259=CARTESIAN_POINT('Ctrl Pts',(-1.72398992664513,1.83644848078674,111.982654142635));
#36260=CARTESIAN_POINT('Ctrl Pts',(-1.66168851342568,1.89118944961872,111.977410011265));
#36261=CARTESIAN_POINT('Ctrl Pts',(-1.59845234474376,1.94675173881877,111.972087198205));
#36262=CARTESIAN_POINT('Ctrl Pts',(-1.53249686008921,1.99907704075062,111.966764385146));
#36263=CARTESIAN_POINT('Ctrl Pts',(-1.46419743944608,2.04790920412003,111.961441572086));
#36264=CARTESIAN_POINT('Ctrl Pts',(-1.39589801880295,2.09674136748945,111.956118759026));
#36265=CARTESIAN_POINT('Ctrl Pts',(-1.32525510956176,2.14208018212246,111.950795945967));
#36266=CARTESIAN_POINT('Ctrl Pts',(-1.25266969144954,2.18371813522801,111.945473132907));
#36267=CARTESIAN_POINT('Ctrl Pts',(-1.18100560812644,2.22482757316149,111.940217882906));
#36268=CARTESIAN_POINT('Ctrl Pts',(-1.10718337541876,2.26248144184893,111.934962632905));
#36269=CARTESIAN_POINT('Ctrl Pts',(-1.03157000785796,2.29644716222428,111.929707382903));
#36270=CARTESIAN_POINT('Ctrl Pts',(-0.956063842513632,2.33036472708657,
111.924459583628));
#36271=CARTESIAN_POINT('Ctrl Pts',(-0.87877200372657,2.3606043423413,111.919211784352));
#36272=CARTESIAN_POINT('Ctrl Pts',(-0.800087502345774,2.38697847468093,
111.913963985076));
#36273=CARTESIAN_POINT('Ctrl Pts',(-0.720832875525854,2.41354370645587,
111.908678161745));
#36274=CARTESIAN_POINT('Ctrl Pts',(-0.640165730344157,2.43618696679044,
111.903392338414));
#36275=CARTESIAN_POINT('Ctrl Pts',(-0.558509793004058,2.45476537801855,
111.898106515082));
#36276=CARTESIAN_POINT('Ctrl Pts',(-0.477586046098783,2.4731772008094,111.892868088541));
#36277=CARTESIAN_POINT('Ctrl Pts',(-0.395691626781038,2.48759667545717,
111.887629661999));
#36278=CARTESIAN_POINT('Ctrl Pts',(-0.313254033035,2.49793477913001,111.882391235457));
#36279=CARTESIAN_POINT('Ctrl Pts',(-0.230843551335432,2.508269482811,111.877154531727));
#36280=CARTESIAN_POINT('Ctrl Pts',(-0.147890707467881,2.51452542398895,
111.871917827997));
#36281=CARTESIAN_POINT('Ctrl Pts',(-0.0648308432706447,2.51666509725883,
111.866681124267));
#36282=CARTESIAN_POINT('Ctrl Pts',(0.0182267587089307,2.5188047122526,111.861444563164));
#36283=CARTESIAN_POINT('Ctrl Pts',(0.101390913928715,2.51682827139128,111.856208002061));
#36284=CARTESIAN_POINT('Ctrl Pts',(0.184224930055796,2.51075037093414,111.850971440958));
#36285=CARTESIAN_POINT('Ctrl Pts',(0.268414691909898,2.5045729933786,111.845649172972));
#36286=CARTESIAN_POINT('Ctrl Pts',(0.352262919021846,2.49415871053369,111.840326904985));
#36287=CARTESIAN_POINT('Ctrl Pts',(0.435316999847022,2.47957765751432,111.835004636999));
#36288=CARTESIAN_POINT('Ctrl Pts',(0.517150979240378,2.46521080665683,111.8297605555));
#36289=CARTESIAN_POINT('Ctrl Pts',(0.59821354739173,2.44679895993656,111.824516474));
#36290=CARTESIAN_POINT('Ctrl Pts',(0.678084285437258,2.42446034239437,111.819272392501));
#36291=CARTESIAN_POINT('Ctrl Pts',(0.759741269292391,2.40162213936001,111.813911031271));
#36292=CARTESIAN_POINT('Ctrl Pts',(0.840151985597406,2.37467957055689,111.808549670041));
#36293=CARTESIAN_POINT('Ctrl Pts',(0.918887765864556,2.34381132426321,111.803188308812));
#36294=CARTESIAN_POINT('Ctrl Pts',(0.997623546131707,2.31294307796952,111.797826947582));
#36295=CARTESIAN_POINT('Ctrl Pts',(1.07468395475887,2.27814942415562,111.792465586352));
#36296=CARTESIAN_POINT('Ctrl Pts',(1.14966792222199,2.23965843793507,111.787104225123));
#36297=CARTESIAN_POINT('Ctrl Pts',(1.22316778867983,2.20192927471852,111.781848977265));
#36298=CARTESIAN_POINT('Ctrl Pts',(1.29494416129683,2.1605084851675,111.776593729406));
#36299=CARTESIAN_POINT('Ctrl Pts',(1.36460213303968,2.1155772896549,111.771338481548));
#36300=CARTESIAN_POINT('Ctrl Pts',(1.43416134522127,2.0707097966166,111.766090684466));
#36301=CARTESIAN_POINT('Ctrl Pts',(1.50160773768334,2.02234203137133,111.760842887384));
#36302=CARTESIAN_POINT('Ctrl Pts',(1.56657003363604,1.97070154506297,111.755595090303));
#36303=CARTESIAN_POINT('Ctrl Pts',(1.63200306190929,1.91868685945026,111.750309266429));
#36304=CARTESIAN_POINT('Ctrl Pts',(1.6949154194594,1.8633520392084,111.745023442556));
#36305=CARTESIAN_POINT('Ctrl Pts',(1.75495656268644,1.80497471258846,111.739737618682));
#36306=CARTESIAN_POINT('Ctrl Pts',(1.81445929822488,1.74712087369383,111.734499194443));
#36307=CARTESIAN_POINT('Ctrl Pts',(1.87114177041857,1.68627920366057,111.729260770203));
#36308=CARTESIAN_POINT('Ctrl Pts',(1.92469655566788,1.62275981543795,111.724022345963));
#36309=CARTESIAN_POINT('Ctrl Pts',(1.97823372746608,1.5592613178908,111.718785644571));
#36310=CARTESIAN_POINT('Ctrl Pts',(2.0286449580902,1.49308720369504,111.713548943179));
#36311=CARTESIAN_POINT('Ctrl Pts',(2.07566176573437,1.42458221393799,111.708312241787));
#36312=CARTESIAN_POINT('Ctrl Pts',(2.12267729253595,1.35607909040949,111.703075683055));
#36313=CARTESIAN_POINT('Ctrl Pts',(2.16629831995995,1.2852455985925,111.697839124322));
#36314=CARTESIAN_POINT('Ctrl Pts',(2.20629933337562,1.21245597921999,111.69260256559));
#36315=CARTESIAN_POINT('Ctrl Pts',(2.24695508308651,1.1384749398896,111.687280294902));
#36316=CARTESIAN_POINT('Ctrl Pts',(2.28387099652829,1.06247358409721,111.681958024214));
#36317=CARTESIAN_POINT('Ctrl Pts',(2.31685947685962,0.984869744933706,111.676635753527));
#36318=CARTESIAN_POINT('Ctrl Pts',(2.34936331018264,0.908406014926671,111.671391674454));
#36319=CARTESIAN_POINT('Ctrl Pts',(2.37805423941063,0.830387034882338,111.666147595382));
#36320=CARTESIAN_POINT('Ctrl Pts',(2.40280253307926,0.751229816386359,111.66090351631));
#36321=CARTESIAN_POINT('Ctrl Pts',(2.42810433929985,0.670302192439338,111.655542149815));
#36322=CARTESIAN_POINT('Ctrl Pts',(2.44928489436196,0.588185296471621,111.650180783319));
#36323=CARTESIAN_POINT('Ctrl Pts',(2.46626069105269,0.505335981074263,111.644819416824));
#36324=CARTESIAN_POINT('Ctrl Pts',(2.48323648774343,0.422486665676905,111.639458050329));
#36325=CARTESIAN_POINT('Ctrl Pts',(2.49600751534742,0.338905443219578,111.634096683833));
#36326=CARTESIAN_POINT('Ctrl Pts',(2.50454671857413,0.255052905256035,111.628735317338));
#36327=CARTESIAN_POINT('Ctrl Pts',(2.51291690716762,0.172860042741429,111.623480067229));
#36328=CARTESIAN_POINT('Ctrl Pts',(2.51725222512239,0.0901029227652949,
111.618224817121));
#36329=CARTESIAN_POINT('Ctrl Pts',(2.51748967125913,0.00721145641435616,
111.612969567012));
#36330=CARTESIAN_POINT('Ctrl Pts',(2.51772678075161,-0.0755624888167714,
111.607721767645));
#36331=CARTESIAN_POINT('Ctrl Pts',(2.5138775571612,-0.158469944519678,111.602473968278));
#36332=CARTESIAN_POINT('Ctrl Pts',(2.50593072673114,-0.24107559566393,111.59722616891));
#36333=CARTESIAN_POINT('Ctrl Pts',(2.4979263160133,-0.324279781935754,111.591940345604));
#36334=CARTESIAN_POINT('Ctrl Pts',(2.48576461990296,-0.407177300180112,
111.586654522297));
#36335=CARTESIAN_POINT('Ctrl Pts',(2.46948765707609,-0.489322962417326,
111.581368698991));
#36336=CARTESIAN_POINT('Ctrl Pts',(2.45335664588034,-0.570732044156025,
111.576130272397));
#36337=CARTESIAN_POINT('Ctrl Pts',(2.43318396494953,-0.651402238350493,
111.570891845803));
#36338=CARTESIAN_POINT('Ctrl Pts',(2.40906235766797,-0.730906838706032,
111.56565341921));
#36339=CARTESIAN_POINT('Ctrl Pts',(2.38494868356147,-0.810385291388008,
111.560416715443));
#36340=CARTESIAN_POINT('Ctrl Pts',(2.35688879631775,-0.888698470374929,
111.555180011676));
#36341=CARTESIAN_POINT('Ctrl Pts',(2.32502568704904,-0.965433480133231,
111.54994330791));
#36342=CARTESIAN_POINT('Ctrl Pts',(2.29316344569622,-1.04216639971462,111.544706746785));
#36343=CARTESIAN_POINT('Ctrl Pts',(2.25749836619498,-1.11732080979032,111.53947018566));
#36344=CARTESIAN_POINT('Ctrl Pts',(2.21822157726942,-1.19050379425535,111.534233624536));
#36345=CARTESIAN_POINT('Ctrl Pts',(2.17830194518036,-1.26488456455099,111.528911356621));
#36346=CARTESIAN_POINT('Ctrl Pts',(2.13465153231263,-1.33722835490508,111.523589088705));
#36347=CARTESIAN_POINT('Ctrl Pts',(2.08751867597528,-1.40715032155574,111.51826682079));
#36348=CARTESIAN_POINT('Ctrl Pts',(2.04107822181224,-1.47604510408256,111.513022739307));
#36349=CARTESIAN_POINT('Ctrl Pts',(1.99125729187287,-1.54258840801495,111.507778657824));
#36350=CARTESIAN_POINT('Ctrl Pts',(1.93833503998196,-1.60644437276183,111.502534576342));
#36351=CARTESIAN_POINT('Ctrl Pts',(1.88422922465678,-1.67172842460315,111.49717321521));
#36352=CARTESIAN_POINT('Ctrl Pts',(1.82688204264785,-1.73420310927673,111.491811854079));
#36353=CARTESIAN_POINT('Ctrl Pts',(1.76663123148277,-1.79354964858787,111.486450492948));
#36354=CARTESIAN_POINT('Ctrl Pts',(1.70638042031768,-1.85289618789902,111.481089131817));
#36355=CARTESIAN_POINT('Ctrl Pts',(1.64322640393058,-1.90911429390156,111.475727770685));
#36356=CARTESIAN_POINT('Ctrl Pts',(1.57754079121682,-1.961930503878,111.470366409554));
#36357=CARTESIAN_POINT('Ctrl Pts',(1.51315522391518,-2.01370137883163,111.465111160137));
#36358=CARTESIAN_POINT('Ctrl Pts',(1.44609957065455,-2.06239504738502,111.459855910719));
#36359=CARTESIAN_POINT('Ctrl Pts',(1.37670013630848,-2.10772459887155,111.454600661302));
#36360=CARTESIAN_POINT('Ctrl Pts',(1.30739909456602,-2.1529898833704,111.449352862632));
#36361=CARTESIAN_POINT('Ctrl Pts',(1.23576125517507,-2.19490027430168,111.444105063962));
#36362=CARTESIAN_POINT('Ctrl Pts',(1.16214561888101,-2.23320930736814,111.438857265293));
#36363=CARTESIAN_POINT('Ctrl Pts',(1.08799657404998,-2.27179592229504,111.433571441813));
#36364=CARTESIAN_POINT('Ctrl Pts',(1.01184131901189,-2.30672847232742,111.428285618332));
#36365=CARTESIAN_POINT('Ctrl Pts',(0.934076151220512,-2.33779981900099,
111.422999794852));
#36366=CARTESIAN_POINT('Ctrl Pts',(0.857008298023256,-2.3685925511726,111.417761368966));
#36367=CARTESIAN_POINT('Ctrl Pts',(0.778359724756236,-2.39559287454398,
111.41252294308));
#36368=CARTESIAN_POINT('Ctrl Pts',(0.698538843538567,-2.41864626063172,
111.407284517194));
#36369=CARTESIAN_POINT('Ctrl Pts',(0.618744214050853,-2.44169206485295,
111.402047814137));
#36370=CARTESIAN_POINT('Ctrl Pts',(0.537778485292789,-2.46079338191883,
111.39681111108));
#36371=CARTESIAN_POINT('Ctrl Pts',(0.456065842483091,-2.47584535004111,
111.391574408024));
#36372=CARTESIAN_POINT('Ctrl Pts',(0.37435542545508,-2.49089690816081,111.38633784761));
#36373=CARTESIAN_POINT('Ctrl Pts',(0.2918985887999,-2.50189925406705,111.381101287196));
#36374=CARTESIAN_POINT('Ctrl Pts',(0.209128967747527,-2.50879878125944,
111.375864726783));
#36375=CARTESIAN_POINT('Ctrl Pts',(0.125004631758573,-2.51581123505973,
111.370542458032));
#36376=CARTESIAN_POINT('Ctrl Pts',(0.040557669060788,-2.51858530040419,
111.36522018928));
#36377=CARTESIAN_POINT('Ctrl Pts',(-0.0437539084321868,-2.51711975191823,
111.359897920529));
#36378=CARTESIAN_POINT('Ctrl Pts',(-0.126826887911599,-2.51567573339883,
111.354653839753));
#36379=CARTESIAN_POINT('Ctrl Pts',(-0.209767970726271,-2.51011593271426,
111.349409758977));
#36380=CARTESIAN_POINT('Ctrl Pts',(-0.292143453966913,-2.50049164211846,
111.344165678201));
#36381=CARTESIAN_POINT('Ctrl Pts',(-0.376361234977798,-2.49065210775829,
111.338804315462));
#36382=CARTESIAN_POINT('Ctrl Pts',(-0.459987307352202,-2.47656417307093,
111.333442952724));
#36383=CARTESIAN_POINT('Ctrl Pts',(-0.542570400201254,-2.45833757055972,
111.328081589985));
#36384=CARTESIAN_POINT('Ctrl Pts',(-0.625153493050303,-2.44011096804851,
111.322720227247));
#36385=CARTESIAN_POINT('Ctrl Pts',(-0.706693134034247,-2.41774589653397,
111.317358864508));
#36386=CARTESIAN_POINT('Ctrl Pts',(-0.786757621261283,-2.39140517173215,
111.31199750177));
#36387=CARTESIAN_POINT('Ctrl Pts',(-0.865237450878734,-2.36558578955607,
111.306742252548));
#36388=CARTESIAN_POINT('Ctrl Pts',(-0.94258987623988,-2.33585137034942,
111.301487003325));
#36389=CARTESIAN_POINT('Ctrl Pts',(-1.01839658171196,-2.30231940711045,
111.296231754103));
#36390=CARTESIAN_POINT('Ctrl Pts',(-1.09409581044478,-2.26883498460085,
111.290983955634));
#36391=CARTESIAN_POINT('Ctrl Pts',(-1.16825325374797,-2.23156389746811,
111.285736157165));
#36392=CARTESIAN_POINT('Ctrl Pts',(-1.2404667207669,-2.19067308484626,111.280488358696));
#36393=CARTESIAN_POINT('Ctrl Pts',(-1.31320343986261,-2.14948598119299,
111.275202535166));
#36394=CARTESIAN_POINT('Ctrl Pts',(-1.38396744190819,-2.10462662241895,
111.269916711637));
#36395=CARTESIAN_POINT('Ctrl Pts',(-1.45236921594197,-2.05631464289493,
111.264630888107));
#36396=CARTESIAN_POINT('Ctrl Pts',(-1.52015763286562,-2.0084358757629,111.259392462434));
#36397=CARTESIAN_POINT('Ctrl Pts',(-1.58562563235106,-1.95716643012531,
111.25415403676));
#36398=CARTESIAN_POINT('Ctrl Pts',(-1.64842123648773,-1.90276474559948,
111.248915611087));
#36399=CARTESIAN_POINT('Ctrl Pts',(-1.71119618816908,-1.84838095290501,
111.243678908246));
#36400=CARTESIAN_POINT('Ctrl Pts',(-1.77130014158641,-1.79086726913501,
111.238442205406));
#36401=CARTESIAN_POINT('Ctrl Pts',(-1.82841419117776,-1.73052240537353,
111.233205502566));
#36402=CARTESIAN_POINT('Ctrl Pts',(-1.88552668499061,-1.67017918539746,
111.227968942373));
#36403=CARTESIAN_POINT('Ctrl Pts',(-1.93964912047973,-1.60700527459635,
111.22273238218));
#36404=CARTESIAN_POINT('Ctrl Pts',(-1.99050043954715,-1.54133521667501,
111.217495821986));
#36405=CARTESIAN_POINT('Ctrl Pts',(-2.04218406182935,-1.47459031150634,
111.212173552986));
#36406=CARTESIAN_POINT('Ctrl Pts',(-2.09048821090684,-1.40526719194838,
111.206851283986));
#36407=CARTESIAN_POINT('Ctrl Pts',(-2.13516249357516,-1.33374936777114,
111.201529014986));
#36408=CARTESIAN_POINT('Ctrl Pts',(-2.17918047477147,-1.26328219847807,
111.196284934438));
#36409=CARTESIAN_POINT('Ctrl Pts',(-2.21967435859153,-1.19068481914261,
111.191040853889));
#36410=CARTESIAN_POINT('Ctrl Pts',(-2.25645103835623,-1.11634894253593,
111.18579677334));
#36411=CARTESIAN_POINT('Ctrl Pts',(-2.29405022025787,-1.04035056083767,
111.180435410114));
#36412=CARTESIAN_POINT('Ctrl Pts',(-2.32776371931494,-0.962535451149197,
111.175074046889));
#36413=CARTESIAN_POINT('Ctrl Pts',(-2.35743788310572,-0.883341880190247,
111.169712683663));
#36414=CARTESIAN_POINT('Ctrl Pts',(-2.38711204689649,-0.804148309231296,
111.164351320437));
#36415=CARTESIAN_POINT('Ctrl Pts',(-2.4127467850239,-0.723576781445333,
111.158989957212));
#36416=CARTESIAN_POINT('Ctrl Pts',(-2.43424362525605,-0.642078050473828,
111.153628593986));
#36417=CARTESIAN_POINT('Ctrl Pts',(-2.46167272104034,-0.538088977011254,
111.146787712076));
#36418=CARTESIAN_POINT('Ctrl Pts',(-2.48245069235363,-0.432277827512794,
111.139946830167));
#36419=CARTESIAN_POINT('Ctrl Pts',(-2.49638302038995,-0.325389098632332,
111.133105948258));
#36420=CARTESIAN_POINT('Ctrl Pts',(-2.51031534842627,-0.218500369751869,
111.126265066348));
#36421=CARTESIAN_POINT('Ctrl Pts',(-2.51740185313733,-0.110533711503309,
111.119424184439));
#36422=CARTESIAN_POINT('Ctrl Pts',(-2.51749898697117,-0.00225845060319963,
111.11258330253));
#36423=CARTESIAN_POINT('Ctrl Pts',(-2.51749898697171,-0.00225845000779732,
111.112583302492));
#36424=CARTESIAN_POINT('Ctrl Pts',(-2.51757261569501,0.0798156431506282,
111.107397822684));
#36425=CARTESIAN_POINT('Ctrl Pts',(-2.51362839019092,0.161986447060072,
111.102212342876));
#36426=CARTESIAN_POINT('Ctrl Pts',(-2.50566466251812,0.243825447826831,
111.097026863068));
#36427=CARTESIAN_POINT('Ctrl Pts',(-2.49770584547388,0.325613984671257,
111.091844580753));
#36428=CARTESIAN_POINT('Ctrl Pts',(-2.48573249308511,0.40707065575182,111.086662298438));
#36429=CARTESIAN_POINT('Ctrl Pts',(-2.46979497866708,0.487769426420808,
111.081480016123));
#36430=CARTESIAN_POINT('Ctrl Pts',(-2.45385906771586,0.568460078019457,
111.076298255196));
#36431=CARTESIAN_POINT('Ctrl Pts',(-2.43395986851913,0.648392515612904,
111.071116494268));
#36432=CARTESIAN_POINT('Ctrl Pts',(-2.41019911302312,0.727149562045231,
111.06593473334));
#36433=CARTESIAN_POINT('Ctrl Pts',(-2.39542387295519,0.776123352810164,
111.062712539429));
#36434=CARTESIAN_POINT('Ctrl Pts',(-2.37915647272574,0.82464284667384,111.059490345518));
#36435=CARTESIAN_POINT('Ctrl Pts',(-2.36143112101026,0.872610629504506,
111.056268151607));
#36436=CARTESIAN_POINT('Ctrl Pts',(-2.36143104183299,0.872610843771477,
111.329984892853));
#36437=CARTESIAN_POINT('Ctrl Pts',(-2.38229711288321,0.816143761966584,
111.334119803671));
#36438=CARTESIAN_POINT('Ctrl Pts',(-2.40114012091893,0.75892196203164,111.338284776278));
#36439=CARTESIAN_POINT('Ctrl Pts',(-2.45397655537651,0.57669045218432,111.351389496961));
#36440=CARTESIAN_POINT('Ctrl Pts',(-2.48038965065677,0.449718197749219,
111.36027728338));
#36441=CARTESIAN_POINT('Ctrl Pts',(-2.50280298128401,0.275519363787184,
111.371972880807));
#36442=CARTESIAN_POINT('Ctrl Pts',(-2.50743097882214,0.229617084015653,
111.375010368583));
#36443=CARTESIAN_POINT('Ctrl Pts',(-2.51327703119018,0.14967507360673,111.380223240681));
#36444=CARTESIAN_POINT('Ctrl Pts',(-2.51507054653771,0.115690941624686,
111.382415250734));
#36445=CARTESIAN_POINT('Ctrl Pts',(-2.51667641816118,0.066221318604821,
111.385572625589));
#36446=CARTESIAN_POINT('Ctrl Pts',(-2.51703576466368,0.0507585812687205,
111.386554790778));
#36447=CARTESIAN_POINT('Ctrl Pts',(-2.51741704981101,0.0235638166596553,
111.388274098202));
#36448=CARTESIAN_POINT('Ctrl Pts',(-2.51749952096065,0.0118332422881704,
111.389013094862));
#36449=CARTESIAN_POINT('Ctrl Pts',(-2.51750051406999,-0.0125924704623981,
111.390546540677));
#36450=CARTESIAN_POINT('Ctrl Pts',(-2.51740500723337,-0.025287301469883,
111.391340533799));
#36451=CARTESIAN_POINT('Ctrl Pts',(-2.51690645117222,-0.0583293546827333,
111.393399671163));
#36452=CARTESIAN_POINT('Ctrl Pts',(-2.51635269694493,-0.0786736282879076,
111.394660124281));
#36453=CARTESIAN_POINT('Ctrl Pts',(-2.51273062852249,-0.170700247685259,
111.400331018358));
#36454=CARTESIAN_POINT('Ctrl Pts',(-2.50684544331757,-0.242241844617296,
111.404653883072));
#36455=CARTESIAN_POINT('Ctrl Pts',(-2.46839587202294,-0.548660119344687,
111.422957309732));
#36456=CARTESIAN_POINT('Ctrl Pts',(-2.40581011773477,-0.778501324702915,
111.436033522515));
#36457=CARTESIAN_POINT('Ctrl Pts',(-2.29176568242305,-1.04318555947838,
111.45323335973));
#36458=CARTESIAN_POINT('Ctrl Pts',(-2.27008475429137,-1.08955975546668,
111.456338779605));
#36459=CARTESIAN_POINT('Ctrl Pts',(-2.24122796721196,-1.14667681291608,
111.460319083837));
#36460=CARTESIAN_POINT('Ctrl Pts',(-2.23536135591467,-1.15807171912494,
111.461121080619));
#36461=CARTESIAN_POINT('Ctrl Pts',(-2.2259413211573,-1.17603026546513,111.462398408591));
#36462=CARTESIAN_POINT('Ctrl Pts',(-2.22244518318594,-1.18262392789843,
111.462870269199));
#36463=CARTESIAN_POINT('Ctrl Pts',(-2.21613482111481,-1.19439836938347,
111.463718217072));
#36464=CARTESIAN_POINT('Ctrl Pts',(-2.2133316523582,-1.19958492996755,111.464093609856));
#36465=CARTESIAN_POINT('Ctrl Pts',(-2.20652289883753,-1.21207770885202,
111.465002317962));
#36466=CARTESIAN_POINT('Ctrl Pts',(-2.20249926041712,-1.21937388791465,
111.465536756066));
#36467=CARTESIAN_POINT('Ctrl Pts',(-2.18997874533529,-1.24181353999731,
111.467191638406));
#36468=CARTESIAN_POINT('Ctrl Pts',(-2.18136155740626,-1.256888813542,111.468319226414));
#36469=CARTESIAN_POINT('Ctrl Pts',(-2.16082899745834,-1.29196213747666,
111.470977710746));
#36470=CARTESIAN_POINT('Ctrl Pts',(-2.14879096499259,-1.31188620997376,
111.47251502445));
#36471=CARTESIAN_POINT('Ctrl Pts',(-2.10502673364014,-1.38210141427275,
111.47802234941));
#36472=CARTESIAN_POINT('Ctrl Pts',(-2.07179858577641,-1.43142991344348,
111.482056997129));
#36473=CARTESIAN_POINT('Ctrl Pts',(-1.93269916909471,-1.62292669528796,
111.498266504626));
#36474=CARTESIAN_POINT('Ctrl Pts',(-1.8136762573168,-1.75493751377668,111.510647824571));
#36475=CARTESIAN_POINT('Ctrl Pts',(-1.61602745460668,-1.93237347880955,
111.528518899809));
#36476=CARTESIAN_POINT('Ctrl Pts',(-1.54721634787599,-1.9878975381383,111.534347594578));
#36477=CARTESIAN_POINT('Ctrl Pts',(-1.45739679203625,-2.05287767866344,
111.541481669317));
#36478=CARTESIAN_POINT('Ctrl Pts',(-1.43899671046783,-2.06581719759917,
111.542919799444));
#36479=CARTESIAN_POINT('Ctrl Pts',(-1.40955861375282,-2.08593480081386,
111.54518463337));
#36480=CARTESIAN_POINT('Ctrl Pts',(-1.39863381125282,-2.09327565111773,
111.546017434415));
#36481=CARTESIAN_POINT('Ctrl Pts',(-1.37892240917232,-2.10629739046327,
111.547506473789));
#36482=CARTESIAN_POINT('Ctrl Pts',(-1.37015708031947,-2.11200977463559,
111.548163874056));
#36483=CARTESIAN_POINT('Ctrl Pts',(-1.34954652799984,-2.12525940237391,
111.549698730898));
#36484=CARTESIAN_POINT('Ctrl Pts',(-1.33767328192528,-2.13275257872918,
111.550574549437));
#36485=CARTESIAN_POINT('Ctrl Pts',(-1.30309911291886,-2.15416993933617,
111.553101240828));
#36486=CARTESIAN_POINT('Ctrl Pts',(-1.28023872677981,-2.16783401367335,
111.554742660105));
#36487=CARTESIAN_POINT('Ctrl Pts',(-1.22800821524524,-2.19793872198445,
111.558430601004));
#36488=CARTESIAN_POINT('Ctrl Pts',(-1.19851631910115,-2.21415843773837,
111.560469419978));
#36489=CARTESIAN_POINT('Ctrl Pts',(-1.09974253052201,-2.26592923685664,
111.567166984433));
#36490=CARTESIAN_POINT('Ctrl Pts',(-1.02913506058263,-2.29885869710453,
111.571744130763));
#36491=CARTESIAN_POINT('Ctrl Pts',(-0.863938634819748,-2.36676234934217,
111.582120812596));
#36492=CARTESIAN_POINT('Ctrl Pts',(-0.768552083639069,-2.39943368171147,
111.587873512919));
#36493=CARTESIAN_POINT('Ctrl Pts',(-0.615375170747078,-2.44182442556879,
111.597030208845));
#36494=CARTESIAN_POINT('Ctrl Pts',(-0.558766982987014,-2.45539653080876,
111.600398314467));
#36495=CARTESIAN_POINT('Ctrl Pts',(-0.428001626262012,-2.48199181126257,
111.608238753064));
#36496=CARTESIAN_POINT('Ctrl Pts',(-0.353633507436423,-2.49367396204227,
111.612741249147));
#36497=CARTESIAN_POINT('Ctrl Pts',(-0.265923136866028,-2.5034497453985,
111.618217208517));
#36498=CARTESIAN_POINT('Ctrl Pts',(-0.252973651521361,-2.50479141995599,
111.619029893264));
#36499=CARTESIAN_POINT('Ctrl Pts',(-0.231852694931628,-2.50681427445869,
111.620363120844));
#36500=CARTESIAN_POINT('Ctrl Pts',(-0.223687093462902,-2.50755609279657,
111.620880438663));
#36501=CARTESIAN_POINT('Ctrl Pts',(-0.209033393997464,-2.50881518903251,
111.621812397235));
#36502=CARTESIAN_POINT('Ctrl Pts',(-0.202546740222107,-2.50934721166434,
111.622226216904));
#36503=CARTESIAN_POINT('Ctrl Pts',(-0.188261769184757,-2.51046308643859,
111.623140382446));
#36504=CARTESIAN_POINT('Ctrl Pts',(-0.180462867634823,-2.51103575274764,
111.62364131666));
#36505=CARTESIAN_POINT('Ctrl Pts',(-0.157874957975957,-2.51258859033894,
111.625097261471));
#36506=CARTESIAN_POINT('Ctrl Pts',(-0.143080092410167,-2.51347448541747,
111.626057206997));
#36507=CARTESIAN_POINT('Ctrl Pts',(-0.0203654575983437,-2.51973551769987,
111.634067000898));
#36508=CARTESIAN_POINT('Ctrl Pts',(0.0877787246391703,-2.51828740509499,
111.641426483692));
#36509=CARTESIAN_POINT('Ctrl Pts',(0.362032782808291,-2.49692731611548,
111.660363496811));
#36510=CARTESIAN_POINT('Ctrl Pts',(0.526898845618981,-2.46740794424107,
111.671977547523));
#36511=CARTESIAN_POINT('Ctrl Pts',(0.763389533845402,-2.40025926108424,
111.688440367221));
#36512=CARTESIAN_POINT('Ctrl Pts',(0.838101609340371,-2.37520440864219,
111.693617737743));
#36513=CARTESIAN_POINT('Ctrl Pts',(0.931767489828273,-2.33882176946208,
111.700078724876));
#36514=CARTESIAN_POINT('Ctrl Pts',(0.951909859335047,-2.33069637499014,
111.701466469118));
#36515=CARTESIAN_POINT('Ctrl Pts',(0.98393080097929,-2.31729481284869,111.703670514166));
#36516=CARTESIAN_POINT('Ctrl Pts',(0.995877677547504,-2.31218570456943,
111.704492365309));
#36517=CARTESIAN_POINT('Ctrl Pts',(1.01846326482464,-2.30231940049616,111.706045377038));
#36518=CARTESIAN_POINT('Ctrl Pts',(1.02910950381845,-2.29758039689254,111.706777127885));
#36519=CARTESIAN_POINT('Ctrl Pts',(1.05326379797822,-2.2866269248687,111.708436849598));
#36520=CARTESIAN_POINT('Ctrl Pts',(1.06675055270763,-2.28036632910666,111.709363222423));
#36521=CARTESIAN_POINT('Ctrl Pts',(1.10800435606921,-2.26077008872686,111.712196416476));
#36522=CARTESIAN_POINT('Ctrl Pts',(1.13558339739316,-2.24704372926393,111.714089825076));
#36523=CARTESIAN_POINT('Ctrl Pts',(1.26890715327651,-2.17760543952424,111.72325101599));
#36524=CARTESIAN_POINT('Ctrl Pts',(1.37084998143279,-2.11491510187378,111.730271171286));
#36525=CARTESIAN_POINT('Ctrl Pts',(1.55269538046208,-1.98439456118379,111.74322271115));
#36526=CARTESIAN_POINT('Ctrl Pts',(1.63356601333388,-1.91837079876647,111.749168590198));
#36527=CARTESIAN_POINT('Ctrl Pts',(1.79366086666738,-1.77018341521113,111.761787913692));
#36528=CARTESIAN_POINT('Ctrl Pts',(1.87186117358412,-1.68727526079769,111.768464567702));
#36529=CARTESIAN_POINT('Ctrl Pts',(1.9529239624428,-1.58873659216649,111.776371431333));
#36530=CARTESIAN_POINT('Ctrl Pts',(1.96158670312308,-1.57802837394737,111.777230362504));
#36531=CARTESIAN_POINT('Ctrl Pts',(1.97540567417953,-1.56065680043112,111.778624274475));
#36532=CARTESIAN_POINT('Ctrl Pts',(1.98061721478924,-1.55403753814311,111.779155525308));
#36533=CARTESIAN_POINT('Ctrl Pts',(1.98980498109427,-1.54224671890582,111.780102289748));
#36534=CARTESIAN_POINT('Ctrl Pts',(1.9937944597679,-1.53708570208269,111.780516865322));
#36535=CARTESIAN_POINT('Ctrl Pts',(2.00241630724092,-1.52584194402355,111.781420471881));
#36536=CARTESIAN_POINT('Ctrl Pts',(2.00704096790004,-1.51975368238673,111.781909994538));
#36537=CARTESIAN_POINT('Ctrl Pts',(2.02005422863553,-1.50245902320068,111.783301008822));
#36538=CARTESIAN_POINT('Ctrl Pts',(2.02837704111314,-1.49120379591061,111.784206798787));
#36539=CARTESIAN_POINT('Ctrl Pts',(2.083492475056,-1.41535414432738,111.7903112832));
#36540=CARTESIAN_POINT('Ctrl Pts',(2.12728196775874,-1.34864267619319,111.795680620909));
#36541=CARTESIAN_POINT('Ctrl Pts',(2.2253461372201,-1.18255627346517,111.808853489364));
#36542=CARTESIAN_POINT('Ctrl Pts',(2.27623252583276,-1.08137411602237,111.816716347026));
#36543=CARTESIAN_POINT('Ctrl Pts',(2.38104602525567,-0.832496058697998,
111.835294276462));
#36544=CARTESIAN_POINT('Ctrl Pts',(2.42830522530029,-0.682480177323201,
111.845877998643));
#36545=CARTESIAN_POINT('Ctrl Pts',(2.46596634230732,-0.507258807512532,
111.857437486713));
#36546=CARTESIAN_POINT('Ctrl Pts',(2.47035415572538,-0.485439899886147,
111.858863748363));
#36547=CARTESIAN_POINT('Ctrl Pts',(2.47710245681933,-0.449418316911209,
111.861197387093));
#36548=CARTESIAN_POINT('Ctrl Pts',(2.47963139714493,-0.435248840845943,
111.862110025733));
#36549=CARTESIAN_POINT('Ctrl Pts',(2.483980249321,-0.409613384289519,111.863751806883));
#36550=CARTESIAN_POINT('Ctrl Pts',(2.4858426170471,-0.398155113187746,111.864482266014));
#36551=CARTESIAN_POINT('Ctrl Pts',(2.48966812999361,-0.373544736174674,
111.866044124285));
#36552=CARTESIAN_POINT('Ctrl Pts',(2.49160646643803,-0.360389087803307,
111.866874724751));
#36553=CARTESIAN_POINT('Ctrl Pts',(2.49662916817981,-0.324320133712944,
111.869140611059));
#36554=CARTESIAN_POINT('Ctrl Pts',(2.49950232713127,-0.301378373349695,
111.870569279755));
#36555=CARTESIAN_POINT('Ctrl Pts',(2.51455567263471,-0.166089569936953,
111.878925695353));
#36556=CARTESIAN_POINT('Ctrl Pts',(2.51947720137194,-0.0530581234540805,
111.885621709153));
#36557=CARTESIAN_POINT('Ctrl Pts',(2.51265170387703,0.233566240413223,111.902302873451));
#36558=CARTESIAN_POINT('Ctrl Pts',(2.49056046207414,0.406292574422091,111.912061708187));
#36559=CARTESIAN_POINT('Ctrl Pts',(2.43576554085955,0.639703725203097,111.926224330721));
#36560=CARTESIAN_POINT('Ctrl Pts',(2.41813351061093,0.703422597384991,111.93019941436));
#36561=CARTESIAN_POINT('Ctrl Pts',(2.39381942274178,0.77950303052444,111.935159157788));
#36562=CARTESIAN_POINT('Ctrl Pts',(2.3895139011996,0.792603115905413,111.93602095817));
#36563=CARTESIAN_POINT('Ctrl Pts',(2.38264182050799,0.812947266442638,111.937372449032));
#36564=CARTESIAN_POINT('Ctrl Pts',(2.38014926590214,0.820216295350178,111.937857967591));
#36565=CARTESIAN_POINT('Ctrl Pts',(2.37548077362315,0.833630518924669,111.938759000705));
#36566=CARTESIAN_POINT('Ctrl Pts',(2.37331420922904,0.839778785760929,111.939173969626));
#36567=CARTESIAN_POINT('Ctrl Pts',(2.36831113619256,0.853802482704644,111.940125007452));
#36568=CARTESIAN_POINT('Ctrl Pts',(2.36545922406888,0.861672195075561,111.940661958888));
#36569=CARTESIAN_POINT('Ctrl Pts',(2.35650168939696,0.886010457680317,111.942332343444));
#36570=CARTESIAN_POINT('Ctrl Pts',(2.35026307801699,0.902429036898991,111.943473109261));
#36571=CARTESIAN_POINT('Ctrl Pts',(2.33523147200849,0.940775391603699,111.946167993238));
#36572=CARTESIAN_POINT('Ctrl Pts',(2.32630069286313,0.962647062292938,111.947728759237));
#36573=CARTESIAN_POINT('Ctrl Pts',(2.29328563902398,1.04035820034957,111.953351435431));
#36574=CARTESIAN_POINT('Ctrl Pts',(2.26748879668205,1.0954441231953,111.957480658369));
#36575=CARTESIAN_POINT('Ctrl Pts',(2.15528270723519,1.31406298953152,111.974319816998));
#36576=CARTESIAN_POINT('Ctrl Pts',(2.05295671387077,1.46880457820489,111.987238051842));
#36577=CARTESIAN_POINT('Ctrl Pts',(1.88349774221641,1.67230969081851,112.004982769701));
#36578=CARTESIAN_POINT('Ctrl Pts',(1.82950223408957,1.73121555619502,112.010235200587));
#36579=CARTESIAN_POINT('Ctrl Pts',(1.75727395606073,1.80285112891874,112.016777166042));
#36580=CARTESIAN_POINT('Ctrl Pts',(1.74155549111149,1.81803973286882,112.018173902209));
#36581=CARTESIAN_POINT('Ctrl Pts',(1.716158463428,1.84194896288625,112.020388798612));
#36582=CARTESIAN_POINT('Ctrl Pts',(1.70660685462993,1.85080223350775,112.021212605329));
#36583=CARTESIAN_POINT('Ctrl Pts',(1.68838347405453,1.86743223496468,112.022767230626));
#36584=CARTESIAN_POINT('Ctrl Pts',(1.67972562537669,1.87522365024132,112.023498656438));
#36585=CARTESIAN_POINT('Ctrl Pts',(1.65993229419706,1.89278909120363,112.025154828225));
#36586=CARTESIAN_POINT('Ctrl Pts',(1.64876390939381,1.9025255191411,112.026078002413));
#36587=CARTESIAN_POINT('Ctrl Pts',(1.61432154261329,1.93202076745023,112.028891243156));
#36588=CARTESIAN_POINT('Ctrl Pts',(1.59077303389617,1.95145575576374,112.03076817607));
#36589=CARTESIAN_POINT('Ctrl Pts',(1.47501005172878,2.04350857684085,112.039783952679));
#36590=CARTESIAN_POINT('Ctrl Pts',(1.37814270631383,2.1100495741371,112.046684545069));
#36591=CARTESIAN_POINT('Ctrl Pts',(1.12002051686159,2.26197468025798,112.064026113519));
#36592=CARTESIAN_POINT('Ctrl Pts',(0.953520813800322,2.33704107421866,112.074250439112));
#36593=CARTESIAN_POINT('Ctrl Pts',(0.738654526577406,2.40709862065585,112.087816802761));
#36594=CARTESIAN_POINT('Ctrl Pts',(0.696562033847317,2.41961465635794,112.09049317055));
#36595=CARTESIAN_POINT('Ctrl Pts',(0.642286257365155,2.43421978905894,112.093993249389));
#36596=CARTESIAN_POINT('Ctrl Pts',(0.630382717951387,2.43732952888696,112.094763862593));
#36597=CARTESIAN_POINT('Ctrl Pts',(0.611403679682745,2.44213937711137,112.095997978751));
#36598=CARTESIAN_POINT('Ctrl Pts',(0.604342601114428,2.44389631818982,112.096458322325));
#36599=CARTESIAN_POINT('Ctrl Pts',(0.590857455825236,2.44718968331548,112.097339931052));
#36600=CARTESIAN_POINT('Ctrl Pts',(0.584434853091539,2.4487314629538,112.09776089071));
#36601=CARTESIAN_POINT('Ctrl Pts',(0.569170414552988,2.45233229962099,112.09876383604));
#36602=CARTESIAN_POINT('Ctrl Pts',(0.560323419139634,2.45436882486701,112.099347072797));
#36603=CARTESIAN_POINT('Ctrl Pts',(0.530498549867877,2.46106467225022,112.10131937713));
#36604=CARTESIAN_POINT('Ctrl Pts',(0.509472734492231,2.46550309117595,112.102719946813));
#36605=CARTESIAN_POINT('Ctrl Pts',(0.385231283500474,2.49007264101417,112.111045412677));
#36606=CARTESIAN_POINT('Ctrl Pts',(0.280901792470644,2.50398776696118,112.118233119482));
#36607=CARTESIAN_POINT('Ctrl Pts',(-0.0102396569414233,2.52439385968174,
112.138349353213));
#36608=CARTESIAN_POINT('Ctrl Pts',(-0.197403401790635,2.51668828409672,
112.151299005578));
#36609=CARTESIAN_POINT('Ctrl Pts',(-0.437825881043689,2.47977900007459,
112.167382242781));
#36610=CARTESIAN_POINT('Ctrl Pts',(-0.493343578136614,2.46933358089448,
112.171062260673));
#36611=CARTESIAN_POINT('Ctrl Pts',(-0.567364900802064,2.45281027721735,
112.175925861383));
#36612=CARTESIAN_POINT('Ctrl Pts',(-0.5862141870893,2.44837377615213,112.177160635127));
#36613=CARTESIAN_POINT('Ctrl Pts',(-0.617126518722295,2.44072056916095,
112.179179929749));
#36614=CARTESIAN_POINT('Ctrl Pts',(-0.629219884878387,2.43763089544132,
112.179968465449));
#36615=CARTESIAN_POINT('Ctrl Pts',(-0.65271740419986,2.43144111352305,112.181497964349));
#36616=CARTESIAN_POINT('Ctrl Pts',(-0.664123672032448,2.42835039772998,
112.182239205783));
#36617=CARTESIAN_POINT('Ctrl Pts',(-0.690937107355352,2.42088180079674,
112.183979039497));
#36618=CARTESIAN_POINT('Ctrl Pts',(-0.706325209677865,2.41643694238857,
112.184975449882));
#36619=CARTESIAN_POINT('Ctrl Pts',(-0.757289062893238,2.40118758611259,
112.188269447425));
#36620=CARTESIAN_POINT('Ctrl Pts',(-0.792668834338255,2.38974159395874,
112.190546315903));
#36621=CARTESIAN_POINT('Ctrl Pts',(-0.997083239671975,2.31857029305641,
112.203668196522));
#36622=CARTESIAN_POINT('Ctrl Pts',(-1.15960518299079,2.24171068333428,112.213920002746));
#36623=CARTESIAN_POINT('Ctrl Pts',(-1.43129821580121,2.07570281156209,112.232225164233));
#36624=CARTESIAN_POINT('Ctrl Pts',(-1.54377004544984,1.99346959907223,112.240241665327));
#36625=CARTESIAN_POINT('Ctrl Pts',(-1.66500051199955,1.88839500978216,112.250094379419));
#36626=CARTESIAN_POINT('Ctrl Pts',(-1.68096076346272,1.87420203289338,112.251418221307));
#36627=CARTESIAN_POINT('Ctrl Pts',(-1.70295360638334,1.85413755061158,112.253283284331));
#36628=CARTESIAN_POINT('Ctrl Pts',(-1.70914074916309,1.84843580816176,112.253812574051));
#36629=CARTESIAN_POINT('Ctrl Pts',(-1.71977086123151,1.83854066008376,112.254730164414));
#36630=CARTESIAN_POINT('Ctrl Pts',(-1.72422740800457,1.83436185566017,112.255117375558));
#36631=CARTESIAN_POINT('Ctrl Pts',(-1.73360359792454,1.82550565501097,112.255937490958));
#36632=CARTESIAN_POINT('Ctrl Pts',(-1.73851958622172,1.82082453194555,112.25637068992));
#36633=CARTESIAN_POINT('Ctrl Pts',(-1.7502330242428,1.80958003280287,112.257410454314));
#36634=CARTESIAN_POINT('Ctrl Pts',(-1.75701253213182,1.80299819451964,112.258018406027));
#36635=CARTESIAN_POINT('Ctrl Pts',(-1.78150075794305,1.77895469591384,112.260236326502));
#36636=CARTESIAN_POINT('Ctrl Pts',(-1.79898688021145,1.76126967146124,112.261862135518));
#36637=CARTESIAN_POINT('Ctrl Pts',(-1.84253758800642,1.71589837260386,112.266012638196));
#36638=CARTESIAN_POINT('Ctrl Pts',(-1.86824166146068,1.68787581911322,112.268557339162));
#36639=CARTESIAN_POINT('Ctrl Pts',(-1.9814001918855,1.5587580191167,112.280159426443));
#36640=CARTESIAN_POINT('Ctrl Pts',(-2.06135163454704,1.45137899828533,112.289465148528));
#36641=CARTESIAN_POINT('Ctrl Pts',(-2.21825237761731,1.20135364584752,112.309788295908));
#36642=CARTESIAN_POINT('Ctrl Pts',(-2.29075388481616,1.05657832094613,112.320697349063));
#36643=CARTESIAN_POINT('Ctrl Pts',(-2.35314765889223,0.894786252596313,
112.331881384402));
#36644=CARTESIAN_POINT('Ctrl Pts',(-2.35732850676449,0.883712993638031,
112.332642198402));
#36645=CARTESIAN_POINT('Ctrl Pts',(-2.36143112095427,0.872610629656001,
112.333400434891));
#36646=CARTESIAN_POINT('Origin',(0.,0.,104.));
#36647=CARTESIAN_POINT('',(-2.36143112101026,0.872610629504504,113.330979739671));
#36648=CARTESIAN_POINT('',(-2.36143112101026,0.872610629504504,113.056261826378));
#36649=CARTESIAN_POINT('',(-2.36143112101026,0.872610629504505,104.));
#36650=CARTESIAN_POINT('',(-2.51749943375649,0.00168850103947855,113.387416697547));
#36651=CARTESIAN_POINT('Ctrl Pts',(-2.36143112101026,0.872610629504504,
113.330979739671));
#36652=CARTESIAN_POINT('Ctrl Pts',(-2.390175081664,0.794824637753064,113.33622078171));
#36653=CARTESIAN_POINT('Ctrl Pts',(-2.41504172891221,0.715697691567379,
113.341461823748));
#36654=CARTESIAN_POINT('Ctrl Pts',(-2.43592936053144,0.635652735777082,
113.346702865786));
#36655=CARTESIAN_POINT('Ctrl Pts',(-2.45685043664356,0.555479615003627,
113.351952299585));
#36656=CARTESIAN_POINT('Ctrl Pts',(-2.47377969301068,0.474386003757832,
113.357201733383));
#36657=CARTESIAN_POINT('Ctrl Pts',(-2.48666679435607,0.392803390829163,
113.362451167182));
#36658=CARTESIAN_POINT('Ctrl Pts',(-2.48999996417262,0.371702547770623,
113.363808901076));
#36659=CARTESIAN_POINT('Ctrl Pts',(-2.49306299843523,0.350569005603976,
113.365166634969));
#36660=CARTESIAN_POINT('Ctrl Pts',(-2.49585559325281,0.329410242142917,
113.366524368863));
#36661=CARTESIAN_POINT('Ctrl Pts',(-2.51017941349532,0.220882387524782,
113.373488478412));
#36662=CARTESIAN_POINT('Ctrl Pts',(-2.51742584483449,0.111407119474494,
113.38045258796));
#36663=CARTESIAN_POINT('Ctrl Pts',(-2.51749943375607,0.00168850166091125,
113.387416697508));
#36664=CARTESIAN_POINT('',(1.91346599666509,1.63598720337492,114.));
#36665=CARTESIAN_POINT('Ctrl Pts',(-2.51749943375649,0.00168850103947504,
113.387416697547));
#36666=CARTESIAN_POINT('Ctrl Pts',(-2.51755421150463,-0.0799833171623861,
113.392600607993));
#36667=CARTESIAN_POINT('Ctrl Pts',(-2.51363042105735,-0.161806285473799,
113.397784518439));
#36668=CARTESIAN_POINT('Ctrl Pts',(-2.50571039821078,-0.243354988233973,
113.402968428884));
#36669=CARTESIAN_POINT('Ctrl Pts',(-2.49780084907216,-0.32479584821237,
113.40814548395));
#36670=CARTESIAN_POINT('Ctrl Pts',(-2.48590561137912,-0.405962694191178,
113.413322539016));
#36671=CARTESIAN_POINT('Ctrl Pts',(-2.47005904803184,-0.486430415615699,
113.418499594082));
#36672=CARTESIAN_POINT('Ctrl Pts',(-2.45422403262535,-0.566839497418313,
113.423672876448));
#36673=CARTESIAN_POINT('Ctrl Pts',(-2.43444349473638,-0.646550001534911,
113.428846158814));
#36674=CARTESIAN_POINT('Ctrl Pts',(-2.41080343797533,-0.72514345714924,
113.43401944118));
#36675=CARTESIAN_POINT('Ctrl Pts',(-2.38717303572815,-0.803704815479894,
113.439190610796));
#36676=CARTESIAN_POINT('Ctrl Pts',(-2.35968637923368,-0.881149576872663,
113.444361780413));
#36677=CARTESIAN_POINT('Ctrl Pts',(-2.32847986839699,-0.957072490707963,
113.449532950029));
#36678=CARTESIAN_POINT('Ctrl Pts',(-2.29727610643059,-1.03298871676443,
113.454703664135));
#36679=CARTESIAN_POINT('Ctrl Pts',(-2.2623533225281,-1.10738292322524,113.459874378242));
#36680=CARTESIAN_POINT('Ctrl Pts',(-2.22389621033664,-1.17986944008663,
113.465045092348));
#36681=CARTESIAN_POINT('Ctrl Pts',(-2.18540521498254,-1.25241982218125,
113.470220362183));
#36682=CARTESIAN_POINT('Ctrl Pts',(-2.14337389406924,-1.32305873727335,
113.475395632017));
#36683=CARTESIAN_POINT('Ctrl Pts',(-2.09803277362101,-1.39142543127979,
113.480570901852));
#36684=CARTESIAN_POINT('Ctrl Pts',(-2.05267206221442,-1.45982166511767,
113.485748407813));
#36685=CARTESIAN_POINT('Ctrl Pts',(-2.00399898569736,-1.52594334083173,
113.490925913774));
#36686=CARTESIAN_POINT('Ctrl Pts',(-1.95228575326899,-1.58946109973882,
113.496103419735));
#36687=CARTESIAN_POINT('Ctrl Pts',(-1.90048496764483,-1.65308639751981,
113.501289691484));
#36688=CARTESIAN_POINT('Ctrl Pts',(-1.84563406334905,-1.71409861995426,
113.506475963233));
#36689=CARTESIAN_POINT('Ctrl Pts',(-1.78804338289506,-1.77220402631446,
113.511662234981));
#36690=CARTESIAN_POINT('Ctrl Pts',(-1.73906891532323,-1.82161621101349,
113.516072582203));
#36691=CARTESIAN_POINT('Ctrl Pts',(-1.68811389733081,-1.86892683868316,
113.520482929426));
#36692=CARTESIAN_POINT('Ctrl Pts',(-1.63538707771097,-1.91397893302303,
113.524893276648));
#36693=CARTESIAN_POINT('Ctrl Pts',(-1.57250705357179,-1.9677063681317,113.530152891049));
#36694=CARTESIAN_POINT('Ctrl Pts',(-1.50686303370176,-2.01842883236994,
113.53541250545));
#36695=CARTESIAN_POINT('Ctrl Pts',(-1.4387738333564,-2.06584997191203,113.540672119851));
#36696=CARTESIAN_POINT('Ctrl Pts',(-1.37077968294609,-2.11320491334619,
113.545924392031));
#36697=CARTESIAN_POINT('Ctrl Pts',(-1.30034750725321,-2.15726742356124,
113.55117666421));
#36698=CARTESIAN_POINT('Ctrl Pts',(-1.22782991160256,-2.19778068928045,
113.556428936389));
#36699=CARTESIAN_POINT('Ctrl Pts',(-1.15486433052847,-2.23854423015475,
113.561713655058));
#36700=CARTESIAN_POINT('Ctrl Pts',(-1.0797878306465,-2.27571421165269,113.566998373726));
#36701=CARTESIAN_POINT('Ctrl Pts',(-1.00299011791318,-2.30907277351072,
113.572283092395));
#36702=CARTESIAN_POINT('Ctrl Pts',(-0.926796819238338,-2.34216879651128,
113.577526219222));
#36703=CARTESIAN_POINT('Ctrl Pts',(-0.848909733928286,-2.37151299596481,
113.58276934605));
#36704=CARTESIAN_POINT('Ctrl Pts',(-0.76973339418745,-2.39693903799673,
113.588012472877));
#36705=CARTESIAN_POINT('Ctrl Pts',(-0.690581954112356,-2.42235708395368,
113.593253950827));
#36706=CARTESIAN_POINT('Ctrl Pts',(-0.610142502947859,-2.44385927919593,
113.598495428776));
#36707=CARTESIAN_POINT('Ctrl Pts',(-0.528836740693188,-2.46132849325177,
113.603736906726));
#36708=CARTESIAN_POINT('Ctrl Pts',(-0.447532155743138,-2.47879745435398,
113.608978308779));
#36709=CARTESIAN_POINT('Ctrl Pts',(-0.365361735020498,-2.49223345476331,
113.614219710832));
#36710=CARTESIAN_POINT('Ctrl Pts',(-0.282758083655926,-2.50157033003816,
113.619461112886));
#36711=CARTESIAN_POINT('Ctrl Pts',(-0.198966866834742,-2.51104143848994,
113.624777868848));
#36712=CARTESIAN_POINT('Ctrl Pts',(-0.114730345459241,-2.51629454991259,
113.63009462481));
#36713=CARTESIAN_POINT('Ctrl Pts',(-0.0305043257572554,-2.51731518410192,
113.635411380772));
#36714=CARTESIAN_POINT('Ctrl Pts',(0.0526488683712037,-2.51832281800389,
113.640660414767));
#36715=CARTESIAN_POINT('Ctrl Pts',(0.135791363028913,-2.51520525956991,
113.645909448762));
#36716=CARTESIAN_POINT('Ctrl Pts',(0.218487445379377,-2.5080010937421,113.651158482757));
#36717=CARTESIAN_POINT('Ctrl Pts',(0.302783919745552,-2.50065750789411,
113.656509099702));
#36718=CARTESIAN_POINT('Ctrl Pts',(0.386616022731536,-2.48906754631549,
113.661859716648));
#36719=CARTESIAN_POINT('Ctrl Pts',(0.469532709508704,-2.47332676464341,
113.667210333594));
#36720=CARTESIAN_POINT('Ctrl Pts',(0.552449396285871,-2.45758598297132,
113.67256095054));
#36721=CARTESIAN_POINT('Ctrl Pts',(0.634450196834202,-2.43769456279067,
113.677911567486));
#36722=CARTESIAN_POINT('Ctrl Pts',(0.715101824085999,-2.41380107531438,
113.683262184432));
#36723=CARTESIAN_POINT('Ctrl Pts',(0.793554342076212,-2.39055908603338,
113.688466907344));
#36724=CARTESIAN_POINT('Ctrl Pts',(0.871033305088665,-2.36344058807609,
113.693671630255));
#36725=CARTESIAN_POINT('Ctrl Pts',(0.947122874109041,-2.33254464294672,
113.698876353167));
#36726=CARTESIAN_POINT('Ctrl Pts',(1.02310324455864,-2.30169303757501,113.704073606614));
#36727=CARTESIAN_POINT('Ctrl Pts',(1.09769774699205,-2.26707492238892,113.709270860061));
#36728=CARTESIAN_POINT('Ctrl Pts',(1.17050463881239,-2.22883941559698,113.714468113509));
#36729=CARTESIAN_POINT('Ctrl Pts',(1.2447292695713,-2.18985936436068,113.719766570955));
#36730=CARTESIAN_POINT('Ctrl Pts',(1.31709545147365,-2.14711967416191,113.725065028401));
#36731=CARTESIAN_POINT('Ctrl Pts',(1.38719800100625,-2.10083030157227,113.730363485847));
#36732=CARTESIAN_POINT('Ctrl Pts',(1.45584139845677,-2.055504420822,113.735551658357));
#36733=CARTESIAN_POINT('Ctrl Pts',(1.52231407870445,-2.00677548085572,113.740739830867));
#36734=CARTESIAN_POINT('Ctrl Pts',(1.58626141440623,-1.95488643536292,113.745928003376));
#36735=CARTESIAN_POINT('Ctrl Pts',(1.65019005547335,-1.9030125593332,113.751114659154));
#36736=CARTESIAN_POINT('Ctrl Pts',(1.71159445158167,-1.84798070796214,113.756301314931));
#36737=CARTESIAN_POINT('Ctrl Pts',(1.77015176078904,-1.79007513634916,113.761487970709));
#36738=CARTESIAN_POINT('Ctrl Pts',(1.82871044984529,-1.73216820024489,113.766674748705));
#36739=CARTESIAN_POINT('Ctrl Pts',(1.88442158455526,-1.67138774159439,113.771861526701));
#36740=CARTESIAN_POINT('Ctrl Pts',(1.9369991156543,-1.60805493561459,113.777048304698));
#36741=CARTESIAN_POINT('Ctrl Pts',(1.99155455645801,-1.54233961815218,113.782430203657));
#36742=CARTESIAN_POINT('Ctrl Pts',(2.04273558987152,-1.47387652273846,113.787812102617));
#36743=CARTESIAN_POINT('Ctrl Pts',(2.09026985344726,-1.40306029441701,113.793194001577));
#36744=CARTESIAN_POINT('Ctrl Pts',(2.13615726482396,-1.33469753549987,113.798389441518));
#36745=CARTESIAN_POINT('Ctrl Pts',(2.17864626181776,-1.26414246756954,113.80358488146));
#36746=CARTESIAN_POINT('Ctrl Pts',(2.21753822073832,-1.19177619105465,113.808780321401));
#36747=CARTESIAN_POINT('Ctrl Pts',(2.25646172605579,-1.11935121615208,113.813979975514));
#36748=CARTESIAN_POINT('Ctrl Pts',(2.29178219227516,-1.045112536375,113.819179629628));
#36749=CARTESIAN_POINT('Ctrl Pts',(2.32334910253939,-0.969461292537977,
113.824379283741));
#36750=CARTESIAN_POINT('Ctrl Pts',(2.35496983129941,-0.893681070726442,
113.829587802756));
#36751=CARTESIAN_POINT('Ctrl Pts',(2.38282409013507,-0.816483924998248,
113.834796321772));
#36752=CARTESIAN_POINT('Ctrl Pts',(2.40681135176588,-0.738285423810404,
113.840004840787));
#36753=CARTESIAN_POINT('Ctrl Pts',(2.40930785914718,-0.730146806804966,
113.840546924597));
#36754=CARTESIAN_POINT('Ctrl Pts',(2.41176252558664,-0.721997350558678,
113.841089008406));
#36755=CARTESIAN_POINT('Ctrl Pts',(2.4141752698409,-0.713837528075284,113.841631092216));
#36756=CARTESIAN_POINT('Ctrl Pts',(2.43819602524483,-0.632600115669368,
113.847027960358));
#36757=CARTESIAN_POINT('Ctrl Pts',(2.45814875987533,-0.550025254596369,
113.852424828499));
#36758=CARTESIAN_POINT('Ctrl Pts',(2.47389213394086,-0.466544702708686,
113.857821696641));
#36759=CARTESIAN_POINT('Ctrl Pts',(2.48961070129014,-0.38319569049949,113.863210060978));
#36760=CARTESIAN_POINT('Ctrl Pts',(2.50113302019914,-0.298944246618516,
113.868598425315));
#36761=CARTESIAN_POINT('Ctrl Pts',(2.50836781699562,-0.214236188961182,
113.873986789652));
#36762=CARTESIAN_POINT('Ctrl Pts',(2.51559120170127,-0.129661748885135,
113.879366654441));
#36763=CARTESIAN_POINT('Ctrl Pts',(2.51854049285268,-0.0446325564713008,
113.884746519229));
#36764=CARTESIAN_POINT('Ctrl Pts',(2.51717585105964,0.0403978321467932,
113.890126384018));
#36765=CARTESIAN_POINT('Ctrl Pts',(2.515812477245,0.125349213441812,113.895501250021));
#36766=CARTESIAN_POINT('Ctrl Pts',(2.51014314800948,0.210301359333818,113.900876116024));
#36767=CARTESIAN_POINT('Ctrl Pts',(2.50018000938136,0.29479852558964,113.906250982027));
#36768=CARTESIAN_POINT('Ctrl Pts',(2.49022373185465,0.379237502990729,113.911622146636));
#36769=CARTESIAN_POINT('Ctrl Pts',(2.47597957677018,0.463221696707422,113.916993311245));
#36770=CARTESIAN_POINT('Ctrl Pts',(2.45751161106588,0.546299305762291,113.922364475854));
#36771=CARTESIAN_POINT('Ctrl Pts',(2.43905192557554,0.629339666514449,113.927733232272));
#36772=CARTESIAN_POINT('Ctrl Pts',(2.41637229132917,0.711473830977599,113.933101988689));
#36773=CARTESIAN_POINT('Ctrl Pts',(2.3895878950694,0.792260021544572,113.938470745107));
#36774=CARTESIAN_POINT('Ctrl Pts',(2.36280113558813,0.873053339980342,113.943839975217));
#36775=CARTESIAN_POINT('Ctrl Pts',(2.3319090164842,0.952498034205536,113.949209205327));
#36776=CARTESIAN_POINT('Ctrl Pts',(2.2970764722723,1.03016791375632,113.954578435437));
#36777=CARTESIAN_POINT('Ctrl Pts',(2.26224447137888,1.10783658181131,113.959947581798));
#36778=CARTESIAN_POINT('Ctrl Pts',(2.22347234975331,1.18373009898536,113.965316728159));
#36779=CARTESIAN_POINT('Ctrl Pts',(2.18097243197872,1.2574440349172,113.97068587452));
#36780=CARTESIAN_POINT('Ctrl Pts',(2.13844113945146,1.33121238875449,113.97605898455));
#36781=CARTESIAN_POINT('Ctrl Pts',(2.09217677159438,1.40279757420296,113.98143209458));
#36782=CARTESIAN_POINT('Ctrl Pts',(2.0424365335209,1.47182174754252,113.986805204611));
#36783=CARTESIAN_POINT('Ctrl Pts',(2.00172068117099,1.52832284522758,113.991203469741));
#36784=CARTESIAN_POINT('Ctrl Pts',(1.95867669090703,1.58310835081476,113.99560173487));
#36785=CARTESIAN_POINT('Ctrl Pts',(1.91346599666509,1.63598720337492,114.));
#36786=CARTESIAN_POINT('',(-1.91365515010967,1.63576594183237,113.999998295674));
#36787=CARTESIAN_POINT('Origin',(0.,0.,114.));
#36788=CARTESIAN_POINT('',(-2.51749949088407,0.00160106165700581,113.112583302433));
#36789=CARTESIAN_POINT('Ctrl Pts',(-1.91365515010967,1.63576594183237,113.999998295674));
#36790=CARTESIAN_POINT('Ctrl Pts',(-1.86017206798978,1.69833490290746,113.994762825085));
#36791=CARTESIAN_POINT('Ctrl Pts',(-1.80351482559582,1.75839765718748,113.989527354496));
#36792=CARTESIAN_POINT('Ctrl Pts',(-1.74394816828049,1.81561312959318,113.984291883907));
#36793=CARTESIAN_POINT('Ctrl Pts',(-1.68446595189907,1.87274749407471,113.979063835054));
#36794=CARTESIAN_POINT('Ctrl Pts',(-1.62208284389702,1.92704227278225,113.973835786202));
#36795=CARTESIAN_POINT('Ctrl Pts',(-1.55710332208692,1.9781899540605,113.968607737349));
#36796=CARTESIAN_POINT('Ctrl Pts',(-1.49219790864146,2.02927930202221,113.963385651023));
#36797=CARTESIAN_POINT('Ctrl Pts',(-1.42470232982389,2.07722839907304,113.958163564698));
#36798=CARTESIAN_POINT('Ctrl Pts',(-1.35495624407953,2.12176808973787,113.952941478372));
#36799=CARTESIAN_POINT('Ctrl Pts',(-1.28525345971406,2.16628012824128,113.947722634143));
#36800=CARTESIAN_POINT('Ctrl Pts',(-1.21330333288295,2.20738671206429,113.942503789914));
#36801=CARTESIAN_POINT('Ctrl Pts',(-1.13947583620391,2.24486103550028,113.937284945685));
#36802=CARTESIAN_POINT('Ctrl Pts',(-1.06567145944788,2.28232362342428,113.932067735796));
#36803=CARTESIAN_POINT('Ctrl Pts',(-0.989991294991094,2.31615599939776,
113.926850525907));
#36804=CARTESIAN_POINT('Ctrl Pts',(-0.912830071039806,2.34617721227649,
113.921633316019));
#36805=CARTESIAN_POINT('Ctrl Pts',(-0.835669270168312,2.37619826054704,
113.916416134737));
#36806=CARTESIAN_POINT('Ctrl Pts',(-0.757027860163825,2.40240802003829,
113.911198953454));
#36807=CARTESIAN_POINT('Ctrl Pts',(-0.677319358495791,2.42467415060392,
113.905981772172));
#36808=CARTESIAN_POINT('Ctrl Pts',(-0.59753402159868,2.44696174466726,113.900759561773));
#36809=CARTESIAN_POINT('Ctrl Pts',(-0.516679987743237,2.46529799189702,
113.895537351375));
#36810=CARTESIAN_POINT('Ctrl Pts',(-0.435184140292947,2.47960097879427,
113.890315140976));
#36811=CARTESIAN_POINT('Ctrl Pts',(-0.353648944782196,2.49391087150096,
113.885090409175));
#36812=CARTESIAN_POINT('Ctrl Pts',(-0.271471780659217,2.50418356786419,
113.879865677374));
#36813=CARTESIAN_POINT('Ctrl Pts',(-0.189085423689017,2.5103890042279,113.874640945573));
#36814=CARTESIAN_POINT('Ctrl Pts',(-0.106557256956499,2.51660512186808,
113.869407220559));
#36815=CARTESIAN_POINT('Ctrl Pts',(-0.0238196439423053,2.51873998240891,
113.864173495546));
#36816=CARTESIAN_POINT('Ctrl Pts',(0.0586941218575013,2.51681569648224,
113.858939770533));
#36817=CARTESIAN_POINT('Ctrl Pts',(0.12722137524081,2.5152175870274,113.854593189128));
#36818=CARTESIAN_POINT('Ctrl Pts',(0.195594143011457,2.51082076482695,113.850246607722));
#36819=CARTESIAN_POINT('Ctrl Pts',(0.263568588429768,2.50366488356432,113.845900026317));
#36820=CARTESIAN_POINT('Ctrl Pts',(0.345886857750583,2.49499898335168,113.840636238483));
#36821=CARTESIAN_POINT('Ctrl Pts',(0.427923672364484,2.4822535576129,113.83537245065));
#36822=CARTESIAN_POINT('Ctrl Pts',(0.509244082206853,2.46545669496288,113.830108662817));
#36823=CARTESIAN_POINT('Ctrl Pts',(0.590452038900465,2.44868305969327,113.824852153962));
#36824=CARTESIAN_POINT('Ctrl Pts',(0.670945112211881,2.42786920923019,113.819595645108));
#36825=CARTESIAN_POINT('Ctrl Pts',(0.750293879482346,2.4030949511851,113.814339136253));
#36826=CARTESIAN_POINT('Ctrl Pts',(0.830052614195825,2.37819269317767,113.809055468848));
#36827=CARTESIAN_POINT('Ctrl Pts',(0.908654715917763,2.34928903312637,113.803771801443));
#36828=CARTESIAN_POINT('Ctrl Pts',(0.985674857527892,2.31651706776302,113.798488134038));
#36829=CARTESIAN_POINT('Ctrl Pts',(1.0621676390054,2.2839694934179,113.793240644125));
#36830=CARTESIAN_POINT('Ctrl Pts',(1.13709962859141,2.24760660554363,113.787993154212));
#36831=CARTESIAN_POINT('Ctrl Pts',(1.21007143981663,2.20760806316251,113.782745664299));
#36832=CARTESIAN_POINT('Ctrl Pts',(1.28302085789761,2.16762179529004,113.777499784703));
#36833=CARTESIAN_POINT('Ctrl Pts',(1.35401088964504,2.12400230977291,113.772253905108));
#36834=CARTESIAN_POINT('Ctrl Pts',(1.42266608394282,2.07697555681303,113.767008025512));
#36835=CARTESIAN_POINT('Ctrl Pts',(1.49132072010692,2.02994918615801,113.761762188563));
#36836=CARTESIAN_POINT('Ctrl Pts',(1.55764017800716,1.9795158638528,113.756516351614));
#36837=CARTESIAN_POINT('Ctrl Pts',(1.62127851820578,1.92594449982456,113.751270514665));
#36838=CARTESIAN_POINT('Ctrl Pts',(1.68571484194417,1.87170138561295,113.745958898321));
#36839=CARTESIAN_POINT('Ctrl Pts',(1.74740195992598,1.81424128057953,113.740647281976));
#36840=CARTESIAN_POINT('Ctrl Pts',(1.80601721206052,1.75388371328921,113.735335665632));
#36841=CARTESIAN_POINT('Ctrl Pts',(1.86399122970701,1.69418644092815,113.730082156887));
#36842=CARTESIAN_POINT('Ctrl Pts',(1.91896000322127,1.63165518174354,113.724828648142));
#36843=CARTESIAN_POINT('Ctrl Pts',(1.97065142286629,1.56663308389523,113.719575139397));
#36844=CARTESIAN_POINT('Ctrl Pts',(2.0232004591392,1.50053219903201,113.714234469253));
#36845=CARTESIAN_POINT('Ctrl Pts',(2.0723621148443,1.43185747623515,113.708893799109));
#36846=CARTESIAN_POINT('Ctrl Pts',(2.11789694190401,1.36099918937288,113.703553128965));
#36847=CARTESIAN_POINT('Ctrl Pts',(2.16343176896373,1.29014090251061,113.698212458821));
#36848=CARTESIAN_POINT('Ctrl Pts',(2.20533957838103,1.21709951046272,113.692871788677));
#36849=CARTESIAN_POINT('Ctrl Pts',(2.24343105055273,1.14228865503246,113.687531118533));
#36850=CARTESIAN_POINT('Ctrl Pts',(2.28087180004238,1.06875580535301,113.682281683907));
#36851=CARTESIAN_POINT('Ctrl Pts',(2.31476407192179,0.993241483549429,113.677032249281));
#36852=CARTESIAN_POINT('Ctrl Pts',(2.34489351657419,0.916122615116727,113.671782814655));
#36853=CARTESIAN_POINT('Ctrl Pts',(2.3749797309288,0.83911439829699,113.666540912018));
#36854=CARTESIAN_POINT('Ctrl Pts',(2.4013136743019,0.760506634589067,113.66129900938));
#36855=CARTESIAN_POINT('Ctrl Pts',(2.42372722344526,0.680700078103652,113.656057106742));
#36856=CARTESIAN_POINT('Ctrl Pts',(2.44633483038983,0.600202551849299,113.650769819409));
#36857=CARTESIAN_POINT('Ctrl Pts',(2.46495359977937,0.518485794368826,113.645482532076));
#36858=CARTESIAN_POINT('Ctrl Pts',(2.47946100625358,0.435980926725019,113.640195244743));
#36859=CARTESIAN_POINT('Ctrl Pts',(2.49381774094527,0.354332942459809,113.634962870396));
#36860=CARTESIAN_POINT('Ctrl Pts',(2.50414803386643,0.271913608038802,113.629730496049));
#36861=CARTESIAN_POINT('Ctrl Pts',(2.51038388229762,0.1891534126056,113.624498121702));
#36862=CARTESIAN_POINT('Ctrl Pts',(2.51661762373109,0.106421180575309,113.619267515294));
#36863=CARTESIAN_POINT('Ctrl Pts',(2.51875963333115,0.0233487771706928,
113.614036908886));
#36864=CARTESIAN_POINT('Ctrl Pts',(2.51679374497759,-0.0596279736504867,
113.608806302478));
#36865=CARTESIAN_POINT('Ctrl Pts',(2.51482792416235,-0.142601873795793,
113.603575875768));
#36866=CARTESIAN_POINT('Ctrl Pts',(2.50875449790617,-0.22547966543505,113.598345449058));
#36867=CARTESIAN_POINT('Ctrl Pts',(2.49860940534716,-0.307826719942721,
113.593115022348));
#36868=CARTESIAN_POINT('Ctrl Pts',(2.48827233935064,-0.391732010319809,
113.587785621381));
#36869=CARTESIAN_POINT('Ctrl Pts',(2.47370796649111,-0.475085773950252,
113.582456220415));
#36870=CARTESIAN_POINT('Ctrl Pts',(2.45500924246962,-0.557436874801747,
113.577126819448));
#36871=CARTESIAN_POINT('Ctrl Pts',(2.4366314972481,-0.638374352055361,113.571888901982));
#36872=CARTESIAN_POINT('Ctrl Pts',(2.41426041510205,-0.718342884315836,
113.566650984516));
#36873=CARTESIAN_POINT('Ctrl Pts',(2.38803476196017,-0.796929247593444,
113.56141306705));
#36874=CARTESIAN_POINT('Ctrl Pts',(2.36112203769729,-0.877574450756549,
113.556037924333));
#36875=CARTESIAN_POINT('Ctrl Pts',(2.33015013274271,-0.956763560776925,
113.550662781616));
#36876=CARTESIAN_POINT('Ctrl Pts',(2.29532093802874,-1.0340735183955,113.545287638899));
#36877=CARTESIAN_POINT('Ctrl Pts',(2.26049174331478,-1.11138347601407,113.539912496182));
#36878=CARTESIAN_POINT('Ctrl Pts',(2.22180555688258,-1.18681385088719,113.534537353466));
#36879=CARTESIAN_POINT('Ctrl Pts',(2.17951291006165,-1.25997211273686,113.529162210749));
#36880=CARTESIAN_POINT('Ctrl Pts',(2.13815552656625,-1.33151254632535,113.523905934412));
#36881=CARTESIAN_POINT('Ctrl Pts',(2.09319585109432,-1.40114634549873,113.518649658076));
#36882=CARTESIAN_POINT('Ctrl Pts',(2.04483473617717,-1.46848804956774,113.51339338174));
#36883=CARTESIAN_POINT('Ctrl Pts',(1.99654215127683,-1.53573432721573,113.508144553799));
#36884=CARTESIAN_POINT('Ctrl Pts',(1.94485796776963,-1.60069458982375,113.502895725858));
#36885=CARTESIAN_POINT('Ctrl Pts',(1.89002812601534,-1.66300930029599,113.497646897917));
#36886=CARTESIAN_POINT('Ctrl Pts',(1.83481450963244,-1.72576017480049,113.492361331461));
#36887=CARTESIAN_POINT('Ctrl Pts',(1.77641125714273,-1.78582790185507,113.487075765005));
#36888=CARTESIAN_POINT('Ctrl Pts',(1.71511306460385,-1.84287639998596,113.481790198548));
#36889=CARTESIAN_POINT('Ctrl Pts',(1.65434966255228,-1.8994271837006,113.476550745534));
#36890=CARTESIAN_POINT('Ctrl Pts',(1.59074198040323,-1.95301089524435,113.47131129252));
#36891=CARTESIAN_POINT('Ctrl Pts',(1.5246152113669,-2.00333589476869,113.466071839506));
#36892=CARTESIAN_POINT('Ctrl Pts',(1.45851022582843,-2.05364431621829,113.460834112474));
#36893=CARTESIAN_POINT('Ctrl Pts',(1.38988816825624,-2.10069587858728,113.455596385441));
#36894=CARTESIAN_POINT('Ctrl Pts',(1.31910687156902,-2.14423956482931,113.450358658409));
#36895=CARTESIAN_POINT('Ctrl Pts',(1.2483275644794,-2.18778202709809,113.445121078605));
#36896=CARTESIAN_POINT('Ctrl Pts',(1.17538953231913,-2.2278165685016,113.4398834988));
#36897=CARTESIAN_POINT('Ctrl Pts',(1.10067792697136,-2.26413655751547,113.434645918996));
#36898=CARTESIAN_POINT('Ctrl Pts',(1.02477563959907,-2.30103537973536,113.42932486766));
#36899=CARTESIAN_POINT('Ctrl Pts',(0.947043186099315,-2.33409998341538,
113.424003816324));
#36900=CARTESIAN_POINT('Ctrl Pts',(0.867906828277549,-2.36316397810842,
113.418682764988));
#36901=CARTESIAN_POINT('Ctrl Pts',(0.789900366584946,-2.39181300178175,
113.413437686763));
#36902=CARTESIAN_POINT('Ctrl Pts',(0.710530296499695,-2.41657483980014,
113.408192608538));
#36903=CARTESIAN_POINT('Ctrl Pts',(0.630219709544866,-2.43734063431872,
113.402947530313));
#36904=CARTESIAN_POINT('Ctrl Pts',(0.548164216731687,-2.4585576066693,113.397588492422));
#36905=CARTESIAN_POINT('Ctrl Pts',(0.46512735781871,-2.47560275032423,113.39222945453));
#36906=CARTESIAN_POINT('Ctrl Pts',(0.381568868438044,-2.4884154493651,113.386870416639));
#36907=CARTESIAN_POINT('Ctrl Pts',(0.298010379057378,-2.50122814840597,
113.381511378747));
#36908=CARTESIAN_POINT('Ctrl Pts',(0.213930769663557,-2.50980841740042,
113.376152340855));
#36909=CARTESIAN_POINT('Ctrl Pts',(0.129790714023531,-2.51415206790545,
113.370793302964));
#36910=CARTESIAN_POINT('Ctrl Pts',(0.0472656661578695,-2.51841234516714,
113.365537127945));
#36911=CARTESIAN_POINT('Ctrl Pts',(-0.0356211275015085,-2.51861292477043,
113.360280952927));
#36912=CARTESIAN_POINT('Ctrl Pts',(-0.118436984617641,-2.51471249463526,
113.355024777908));
#36913=CARTESIAN_POINT('Ctrl Pts',(-0.201135760636818,-2.51081757874162,
113.349776033818));
#36914=CARTESIAN_POINT('Ctrl Pts',(-0.283763342413377,-2.50283319092071,
113.344527289729));
#36915=CARTESIAN_POINT('Ctrl Pts',(-0.365884255560971,-2.49076995355504,
113.339278545639));
#36916=CARTESIAN_POINT('Ctrl Pts',(-0.448581647023647,-2.47862203380478,
113.333992956037));
#36917=CARTESIAN_POINT('Ctrl Pts',(-0.530764754398789,-2.46233774014118,
113.328707366434));
#36918=CARTESIAN_POINT('Ctrl Pts',(-0.611991222275894,-2.44198136640255,
113.323421776832));
#36919=CARTESIAN_POINT('Ctrl Pts',(-0.692508066750636,-2.4218028332074,
113.318182364026));
#36920=CARTESIAN_POINT('Ctrl Pts',(-0.77208446623163,-2.39762320674597,
113.31294295122));
#36921=CARTESIAN_POINT('Ctrl Pts',(-0.850298770475567,-2.36955655153612,
113.307703538414));
#36922=CARTESIAN_POINT('Ctrl Pts',(-0.928487556411774,-2.34149905339224,
113.302465835026));
#36923=CARTESIAN_POINT('Ctrl Pts',(-1.00531469593654,-2.30955720088386,
113.297228131638));
#36924=CARTESIAN_POINT('Ctrl Pts',(-1.08037485415755,-2.27389454999656,
113.29199042825));
#36925=CARTESIAN_POINT('Ctrl Pts',(-1.15543314141069,-2.23823278804522,
113.286752855419));
#36926=CARTESIAN_POINT('Ctrl Pts',(-1.22872411878293,-2.19885061099978,
113.281515282587));
#36927=CARTESIAN_POINT('Ctrl Pts',(-1.29986481932664,-2.15595865022429,
113.276277709755));
#36928=CARTESIAN_POINT('Ctrl Pts',(-1.37214017913248,-2.11238258372319,
113.270956600207));
#36929=CARTESIAN_POINT('Ctrl Pts',(-1.442195639441,-2.06518403122962,113.26563549066));
#36930=CARTESIAN_POINT('Ctrl Pts',(-1.50965960883331,-2.0146300194967,113.260314381112));
#36931=CARTESIAN_POINT('Ctrl Pts',(-1.57616004961209,-1.964798026306,113.255069268297));
#36932=CARTESIAN_POINT('Ctrl Pts',(-1.6401422257576,-1.91170614836506,113.249824155483));
#36933=CARTESIAN_POINT('Ctrl Pts',(-1.70128454596898,-1.85565005958751,
113.244579042668));
#36934=CARTESIAN_POINT('Ctrl Pts',(-1.76375570793684,-1.79837567109193,
113.239219934754));
#36935=CARTESIAN_POINT('Ctrl Pts',(-1.82326176568727,-1.73800707625495,
113.233860826839));
#36936=CARTESIAN_POINT('Ctrl Pts',(-1.87950165344929,-1.67489694748107,
113.228501718924));
#36937=CARTESIAN_POINT('Ctrl Pts',(-1.9357415412113,-1.61178681870719,113.223142611009));
#36938=CARTESIAN_POINT('Ctrl Pts',(-1.98871499347162,-1.54593559223706,
113.217783503095));
#36939=CARTESIAN_POINT('Ctrl Pts',(-2.03816777581588,-1.47772743346862,
113.21242439518));
#36940=CARTESIAN_POINT('Ctrl Pts',(-2.08698649321268,-1.41039381401942,
113.207133999728));
#36941=CARTESIAN_POINT('Ctrl Pts',(-2.13255478527078,-1.3405147003582,113.201843604277));
#36942=CARTESIAN_POINT('Ctrl Pts',(-2.17459904927782,-1.26843416261152,
113.196553208825));
#36943=CARTESIAN_POINT('Ctrl Pts',(-2.21658214617846,-1.19645848953606,
113.19127050998));
#36944=CARTESIAN_POINT('Ctrl Pts',(-2.25505117194463,-1.12228814139204,
113.185987811136));
#36945=CARTESIAN_POINT('Ctrl Pts',(-2.28977440510418,-1.04629796125663,
113.180705112291));
#36946=CARTESIAN_POINT('Ctrl Pts',(-2.32445711796564,-0.970396457908242,
113.175428578095));
#36947=CARTESIAN_POINT('Ctrl Pts',(-2.3554025359366,-0.892679751782247,
113.170152043899));
#36948=CARTESIAN_POINT('Ctrl Pts',(-2.38242433929953,-0.813548103994591,
113.164875509703));
#36949=CARTESIAN_POINT('Ctrl Pts',(-2.40942081620889,-0.734490623129741,
113.159603920991));
#36950=CARTESIAN_POINT('Ctrl Pts',(-2.43250084524009,-0.654021265133354,
113.154332332279));
#36951=CARTESIAN_POINT('Ctrl Pts',(-2.45152634821391,-0.572559878102677,
113.149060743568));
#36952=CARTESIAN_POINT('Ctrl Pts',(-2.47054157481037,-0.491142491378067,
113.143792002236));
#36953=CARTESIAN_POINT('Ctrl Pts',(-2.48550652623066,-0.408734581394225,
113.138523260904));
#36954=CARTESIAN_POINT('Ctrl Pts',(-2.49633338758601,-0.325769654853503,
113.133254519572));
#36955=CARTESIAN_POINT('Ctrl Pts',(-2.5071586393188,-0.242817062655348,
113.12798656154));
#36956=CARTESIAN_POINT('Ctrl Pts',(-2.51384696245808,-0.15930806729188,
113.122718603509));
#36957=CARTESIAN_POINT('Ctrl Pts',(-2.51636210187741,-0.0756836986086212,
113.117450645477));
#36958=CARTESIAN_POINT('Ctrl Pts',(-2.51713672499427,-0.0499287171486604,
113.115828197815));
#36959=CARTESIAN_POINT('Ctrl Pts',(-2.51751587600766,-0.0241628209646658,
113.114205750154));
#36960=CARTESIAN_POINT('Ctrl Pts',(-2.51749949088467,0.00160106071358734,
113.112583302492));
#36961=CARTESIAN_POINT('Ctrl Pts',(-2.51749949088407,0.00160106165700588,
113.112583302433));
#36962=CARTESIAN_POINT('Ctrl Pts',(-2.51743978923143,0.0954755726528559,
113.106671674567));
#36963=CARTESIAN_POINT('Ctrl Pts',(-2.51212532380063,0.18915115378945,113.100760046701));
#36964=CARTESIAN_POINT('Ctrl Pts',(-2.50164689230095,0.282079911090854,
113.094848418835));
#36965=CARTESIAN_POINT('Ctrl Pts',(-2.49111954918855,0.375442444705727,
113.088909196452));
#36966=CARTESIAN_POINT('Ctrl Pts',(-2.47538004733398,0.468050954361973,
113.08296997407));
#36967=CARTESIAN_POINT('Ctrl Pts',(-2.45457000539992,0.559367802604915,
113.077030751687));
#36968=CARTESIAN_POINT('Ctrl Pts',(-2.43364683981328,0.65118105039612,113.071059243616));
#36969=CARTESIAN_POINT('Ctrl Pts',(-2.40759797707336,0.74168835061026,113.065087735545));
#36970=CARTESIAN_POINT('Ctrl Pts',(-2.37661545553252,0.830364514248985,
113.059116227474));
#36971=CARTESIAN_POINT('Ctrl Pts',(-2.37167887209854,0.844493683168649,
113.058164760442));
#36972=CARTESIAN_POINT('Ctrl Pts',(-2.36661713203812,0.858576411468391,
113.05721329341));
#36973=CARTESIAN_POINT('Ctrl Pts',(-2.36143112101026,0.872610629504505,
113.056261826378));
#36974=CARTESIAN_POINT('Origin',(0.,0.,104.));
#36975=CARTESIAN_POINT('',(-2.51749986513132,0.000824053271277057,112.112583302525));
#36976=CARTESIAN_POINT('Ctrl Pts',(-2.36143112101026,0.872610629504505,
113.056261826378));
#36977=CARTESIAN_POINT('Ctrl Pts',(-2.35742253990996,0.883458524133866,
113.055526380051));
#36978=CARTESIAN_POINT('Ctrl Pts',(-2.35333971150685,0.894277435752685,
113.054790933724));
#36979=CARTESIAN_POINT('Ctrl Pts',(-2.34918305681532,0.90506641500601,113.054055487397));
#36980=CARTESIAN_POINT('Ctrl Pts',(-2.31947994965906,0.982163559380531,
113.048800049387));
#36981=CARTESIAN_POINT('Ctrl Pts',(-2.28592265483531,1.05793922995017,113.043544611376));
#36982=CARTESIAN_POINT('Ctrl Pts',(-2.24864941558701,1.13198147324953,113.038289173366));
#36983=CARTESIAN_POINT('Ctrl Pts',(-2.21142901042525,1.20591876311934,113.033041184837));
#36984=CARTESIAN_POINT('Ctrl Pts',(-2.17050332894378,1.27812709757133,113.027793196307));
#36985=CARTESIAN_POINT('Ctrl Pts',(-2.12605919360101,1.34821309714177,113.022545207777));
#36986=CARTESIAN_POINT('Ctrl Pts',(-2.08129504247615,1.41880374430617,113.017259431604));
#36987=CARTESIAN_POINT('Ctrl Pts',(-2.03296172678269,1.48724092295824,113.01197365543));
#36988=CARTESIAN_POINT('Ctrl Pts',(-1.98129803209388,1.55314659901147,113.006687879257));
#36989=CARTESIAN_POINT('Ctrl Pts',(-1.93009527182849,1.61846427618127,113.001449261851));
#36990=CARTESIAN_POINT('Ctrl Pts',(-1.87562161171082,1.68129507221643,112.996210644446));
#36991=CARTESIAN_POINT('Ctrl Pts',(-1.81815275188423,1.74130032470444,112.99097202704));
#36992=CARTESIAN_POINT('Ctrl Pts',(-1.76070278980934,1.801285845387,112.985735132273));
#36993=CARTESIAN_POINT('Ctrl Pts',(-1.70025990302305,1.85844733489328,112.980498237507));
#36994=CARTESIAN_POINT('Ctrl Pts',(-1.63713836248182,1.91248117169565,112.97526134274));
#36995=CARTESIAN_POINT('Ctrl Pts',(-1.57401854213981,1.96651353595848,112.97002459069));
#36996=CARTESIAN_POINT('Ctrl Pts',(-1.5082205643552,2.01741811773257,112.96478783864));
#36997=CARTESIAN_POINT('Ctrl Pts',(-1.44009259967277,2.06493088367812,112.95955108659));
#36998=CARTESIAN_POINT('Ctrl Pts',(-1.37085504500771,2.11321748294433,112.954229044342));
#36999=CARTESIAN_POINT('Ctrl Pts',(-1.29921132121754,2.15800049824826,112.948907002094));
#37000=CARTESIAN_POINT('Ctrl Pts',(-1.2255568803691,2.19904901786658,112.943584959845));
#37001=CARTESIAN_POINT('Ctrl Pts',(-1.15297876560743,2.23949768780877,112.938340689594));
#37002=CARTESIAN_POINT('Ctrl Pts',(-1.07844875856923,2.27632013507848,112.933096419342));
#37003=CARTESIAN_POINT('Ctrl Pts',(-1.00236773890926,2.30934301609656,112.92785214909));
#37004=CARTESIAN_POINT('Ctrl Pts',(-0.924594308532173,2.34310048608301,
112.922491220844));
#37005=CARTESIAN_POINT('Ctrl Pts',(-0.845200512098593,2.37288713906597,
112.917130292597));
#37006=CARTESIAN_POINT('Ctrl Pts',(-0.76463160291642,2.39857140019251,112.911769364351));
#37007=CARTESIAN_POINT('Ctrl Pts',(-0.684062693734246,2.42425566131905,
112.906408436104));
#37008=CARTESIAN_POINT('Ctrl Pts',(-0.602319179784995,2.4458374654769,112.901047507858));
#37009=CARTESIAN_POINT('Ctrl Pts',(-0.519856031971376,2.46324094558835,
112.895686579612));
#37010=CARTESIAN_POINT('Ctrl Pts',(-0.439017021013886,2.48030165884911,
112.890431236483));
#37011=CARTESIAN_POINT('Ctrl Pts',(-0.35718804757108,2.49341016839008,112.885175893354));
#37012=CARTESIAN_POINT('Ctrl Pts',(-0.274789908521613,2.50245814274179,
112.879920550225));
#37013=CARTESIAN_POINT('Ctrl Pts',(-0.192508554083284,2.51149329320963,
112.874672655604));
#37014=CARTESIAN_POINT('Ctrl Pts',(-0.109660091183823,2.51647928983228,
112.869424760983));
#37015=CARTESIAN_POINT('Ctrl Pts',(-0.02667618636761,2.51735866158974,112.864176866363));
#37016=CARTESIAN_POINT('Ctrl Pts',(0.0569071050046635,2.51824438498382,
112.85889106659));
#37017=CARTESIAN_POINT('Ctrl Pts',(0.140627339457404,2.51496381246618,112.853605266818));
#37018=CARTESIAN_POINT('Ctrl Pts',(0.224037401075276,2.50751141431489,112.848319467046));
#37019=CARTESIAN_POINT('Ctrl Pts',(0.306701490974546,2.50012566613541,112.843080940433));
#37020=CARTESIAN_POINT('Ctrl Pts',(0.389060465882272,2.48864245688889,112.83784241382));
#37021=CARTESIAN_POINT('Ctrl Pts',(0.470680165815713,2.47310865744061,112.832603887207));
#37022=CARTESIAN_POINT('Ctrl Pts',(0.552273047443024,2.45757996203203,112.82736708185));
#37023=CARTESIAN_POINT('Ctrl Pts',(0.633126683617536,2.43800340591899,112.822130276494));
#37024=CARTESIAN_POINT('Ctrl Pts',(0.712815306971328,2.41447729087423,112.816893471137));
#37025=CARTESIAN_POINT('Ctrl Pts',(0.792501781614026,2.39095181018382,112.811656806985));
#37026=CARTESIAN_POINT('Ctrl Pts',(0.871022863666545,2.3634771139357,112.806420142832));
#37027=CARTESIAN_POINT('Ctrl Pts',(0.947967536103355,2.33220149225879,112.80118347868));
#37028=CARTESIAN_POINT('Ctrl Pts',(1.02616829911449,2.30041530874115,112.795861328109));
#37029=CARTESIAN_POINT('Ctrl Pts',(1.10274026042232,2.26470315876107,112.790539177538));
#37030=CARTESIAN_POINT('Ctrl Pts',(1.17727439967341,2.22527104818124,112.785217026967));
#37031=CARTESIAN_POINT('Ctrl Pts',(1.25071669726387,2.18641657385681,112.779972839941));
#37032=CARTESIAN_POINT('Ctrl Pts',(1.32218011034016,2.14395069601214,112.774728652915));
#37033=CARTESIAN_POINT('Ctrl Pts',(1.39130099717206,2.09811529360711,112.769484465889));
#37034=CARTESIAN_POINT('Ctrl Pts',(1.46196327907883,2.0512577621936,112.764123333546));
#37035=CARTESIAN_POINT('Ctrl Pts',(1.53017688912916,2.00087892113285,112.758762201202));
#37036=CARTESIAN_POINT('Ctrl Pts',(1.59558900860551,1.94728065918021,112.753401068859));
#37037=CARTESIAN_POINT('Ctrl Pts',(1.66100112808185,1.89368239722757,112.748039936515));
#37038=CARTESIAN_POINT('Ctrl Pts',(1.72361142572262,1.83686510516709,112.742678804172));
#37039=CARTESIAN_POINT('Ctrl Pts',(1.78310853031011,1.77716915884092,112.737317671828));
#37040=CARTESIAN_POINT('Ctrl Pts',(1.84142945236355,1.71865332589856,112.732062522293));
#37041=CARTESIAN_POINT('Ctrl Pts',(1.89697461828024,1.6571554909892,112.726807372758));
#37042=CARTESIAN_POINT('Ctrl Pts',(1.94942405491907,1.59296958668484,112.721552223222));
#37043=CARTESIAN_POINT('Ctrl Pts',(2.0017991132017,1.52887470417901,112.716304525996));
#37044=CARTESIAN_POINT('Ctrl Pts',(2.05108687255724,1.46209967823052,112.711056828769));
#37045=CARTESIAN_POINT('Ctrl Pts',(2.09700409958307,1.39297525330919,112.705809131542));
#37046=CARTESIAN_POINT('Ctrl Pts',(2.1432551506256,1.32334828512306,112.700523282896));
#37047=CARTESIAN_POINT('Ctrl Pts',(2.18608611890685,1.25133794816154,112.695237434251));
#37048=CARTESIAN_POINT('Ctrl Pts',(2.22524889018405,1.1773162815211,112.689951585605));
#37049=CARTESIAN_POINT('Ctrl Pts',(2.26405953268012,1.10396017450275,112.684713264225));
#37050=CARTESIAN_POINT('Ctrl Pts',(2.29926745803909,1.02862917736508,112.679474942845));
#37051=CARTESIAN_POINT('Ctrl Pts',(2.33067559396206,0.951712942913775,112.674236621465));
#37052=CARTESIAN_POINT('Ctrl Pts',(2.36207339457172,0.874822018891059,112.669000023833));
#37053=CARTESIAN_POINT('Ctrl Pts',(2.38967371475449,0.796347320430814,112.6637634262));
#37054=CARTESIAN_POINT('Ctrl Pts',(2.41332719013228,0.716699465165306,112.658526828567));
#37055=CARTESIAN_POINT('Ctrl Pts',(2.4369800176874,0.637053791299605,112.653290374355));
#37056=CARTESIAN_POINT('Ctrl Pts',(2.45668608498179,0.556235467152466,112.648053920143));
#37057=CARTESIAN_POINT('Ctrl Pts',(2.47234598758015,0.474669956597551,112.64281746593));
#37058=CARTESIAN_POINT('Ctrl Pts',(2.48826289130412,0.391765840780482,112.637495074107));
#37059=CARTESIAN_POINT('Ctrl Pts',(2.49999951690567,0.30809027249351,112.632172682283));
#37060=CARTESIAN_POINT('Ctrl Pts',(2.50750594724184,0.224098582206117,112.626850290459));
#37061=CARTESIAN_POINT('Ctrl Pts',(2.5149017807015,0.141344393391824,112.621606316722));
#37062=CARTESIAN_POINT('Ctrl Pts',(2.51819128388743,0.0582838059104078,
112.616362342986));
#37063=CARTESIAN_POINT('Ctrl Pts',(2.51737935166998,-0.0246464964168013,
112.61111836925));
#37064=CARTESIAN_POINT('Ctrl Pts',(2.51654920706964,-0.109437001340971,
112.605756768382));
#37065=CARTESIAN_POINT('Ctrl Pts',(2.51143143353047,-0.194090794260034,
112.600395167514));
#37066=CARTESIAN_POINT('Ctrl Pts',(2.50208718104879,-0.278147422118786,
112.595033566647));
#37067=CARTESIAN_POINT('Ctrl Pts',(2.4927429285671,-0.362204049977539,112.589671965779));
#37068=CARTESIAN_POINT('Ctrl Pts',(2.47917234468489,-0.44566302179835,112.584310364911));
#37069=CARTESIAN_POINT('Ctrl Pts',(2.4614914561348,-0.528077703918061,112.578948764044));
#37070=CARTESIAN_POINT('Ctrl Pts',(2.4441611792165,-0.608858104700658,112.573693483603));
#37071=CARTESIAN_POINT('Ctrl Pts',(2.4228181518075,-0.688933658633213,112.568438203163));
#37072=CARTESIAN_POINT('Ctrl Pts',(2.39753473630544,-0.767875926311536,
112.563182922723));
#37073=CARTESIAN_POINT('Ctrl Pts',(2.37228716535847,-0.846706276734757,
112.557935092747));
#37074=CARTESIAN_POINT('Ctrl Pts',(2.34311044196548,-0.92440609646199,112.552687262772));
#37075=CARTESIAN_POINT('Ctrl Pts',(2.31012780853102,-1.00055772359804,112.547439432796));
#37076=CARTESIAN_POINT('Ctrl Pts',(2.27690643472855,-1.07726056407256,112.542153617107));
#37077=CARTESIAN_POINT('Ctrl Pts',(2.23982392090673,-1.15239224138215,112.536867801418));
#37078=CARTESIAN_POINT('Ctrl Pts',(2.19905724983395,-1.22554210941638,112.531581985729));
#37079=CARTESIAN_POINT('Ctrl Pts',(2.15865582601481,-1.29803659432266,112.52634352808));
#37080=CARTESIAN_POINT('Ctrl Pts',(2.1146362256131,-1.36858422924356,112.521105070432));
#37081=CARTESIAN_POINT('Ctrl Pts',(2.06721801032139,-1.43680755419885,112.515866612784));
#37082=CARTESIAN_POINT('Ctrl Pts',(2.01981538907437,-1.50500844310142,112.510629877864));
#37083=CARTESIAN_POINT('Ctrl Pts',(1.9690166358365,-1.57088616154709,112.505393142945));
#37084=CARTESIAN_POINT('Ctrl Pts',(1.91508487122922,-1.63409185359604,112.500156408026));
#37085=CARTESIAN_POINT('Ctrl Pts',(1.86115457508603,-1.69729582466869,112.494919815693));
#37086=CARTESIAN_POINT('Ctrl Pts',(1.80409173746947,-1.75782756366648,112.489683223361));
#37087=CARTESIAN_POINT('Ctrl Pts',(1.74419913189159,-1.81537203853883,112.484446631028));
#37088=CARTESIAN_POINT('Ctrl Pts',(1.68332704644748,-1.87385759209704,112.479124399797));
#37089=CARTESIAN_POINT('Ctrl Pts',(1.61953214840592,-1.92925694349847,112.473802168567));
#37090=CARTESIAN_POINT('Ctrl Pts',(1.55316914556331,-1.9812803575643,112.468479937336));
#37091=CARTESIAN_POINT('Ctrl Pts',(1.48778020658823,-2.03254018159147,112.46323582483));
#37092=CARTESIAN_POINT('Ctrl Pts',(1.41989846878913,-2.08052229379791,112.457991712323));
#37093=CARTESIAN_POINT('Ctrl Pts',(1.34989290014419,-2.12499303719807,112.452747599817));
#37094=CARTESIAN_POINT('Ctrl Pts',(1.27832307852287,-2.17045746573032,112.447386309224));
#37095=CARTESIAN_POINT('Ctrl Pts',(1.20453381450385,-2.21225146025582,112.442025018631));
#37096=CARTESIAN_POINT('Ctrl Pts',(1.1289445359492,-2.25017565642117,112.436663728038));
#37097=CARTESIAN_POINT('Ctrl Pts',(1.05335525739454,-2.28809985258653,112.431302437445));
#37098=CARTESIAN_POINT('Ctrl Pts',(0.975966456223256,-2.32215410689282,
112.425941146852));
#37099=CARTESIAN_POINT('Ctrl Pts',(0.897215841482083,-2.35219259071055,
112.420579856259));
#37100=CARTESIAN_POINT('Ctrl Pts',(0.820022714062956,-2.38163698954401,
112.415324598389));
#37101=CARTESIAN_POINT('Ctrl Pts',(0.741236063657785,-2.40733180564496,
112.410069340519));
#37102=CARTESIAN_POINT('Ctrl Pts',(0.66125465588879,-2.429104470801,112.404814082649));
#37103=CARTESIAN_POINT('Ctrl Pts',(0.581386639723933,-2.45084626831545,
112.399566275287));
#37104=CARTESIAN_POINT('Ctrl Pts',(0.50032767215338,-2.46867683953436,112.394318467926));
#37105=CARTESIAN_POINT('Ctrl Pts',(0.418495180676302,-2.48247216172724,
112.389070660564));
#37106=CARTESIAN_POINT('Ctrl Pts',(0.336069912429048,-2.49636741423369,
112.383784839227));
#37107=CARTESIAN_POINT('Ctrl Pts',(0.252860309293708,-2.50616854129163,
112.37849901789));
#37108=CARTESIAN_POINT('Ctrl Pts',(0.169307180293646,-2.5118004157777,112.373213196553));
#37109=CARTESIAN_POINT('Ctrl Pts',(0.0865030868762668,-2.51738180173703,
112.367974761451));
#37110=CARTESIAN_POINT('Ctrl Pts',(0.00336207105493,-2.518868357077,112.36273632635));
#37111=CARTESIAN_POINT('Ctrl Pts',(-0.0796797191176613,-2.51623873914248,
112.357497891249));
#37112=CARTESIAN_POINT('Ctrl Pts',(-0.162694201103312,-2.51360998595447,
112.3522611788));
#37113=CARTESIAN_POINT('Ctrl Pts',(-0.245609061421601,-2.50686776240543,
112.347024466351));
#37114=CARTESIAN_POINT('Ctrl Pts',(-0.327988429067703,-2.49604283625055,
112.341787753903));
#37115=CARTESIAN_POINT('Ctrl Pts',(-0.410365555359416,-2.48521820461718,
112.336551183933));
#37116=CARTESIAN_POINT('Ctrl Pts',(-0.492206760595113,-2.47031115237332,
112.331314613964));
#37117=CARTESIAN_POINT('Ctrl Pts',(-0.57308295589743,-2.45140412328524,
112.326078043994));
#37118=CARTESIAN_POINT('Ctrl Pts',(-0.655282559208771,-2.43218771127393,
112.320755786034));
#37119=CARTESIAN_POINT('Ctrl Pts',(-0.736484804272134,-2.4088393344905,
112.315433528074));
#37120=CARTESIAN_POINT('Ctrl Pts',(-0.816253533495705,-2.38149877578297,
112.310111270114));
#37121=CARTESIAN_POINT('Ctrl Pts',(-0.894850709663508,-2.35455976434104,
112.304867179472));
#37122=CARTESIAN_POINT('Ctrl Pts',(-0.972055786362678,-2.32374528861014,
112.299623088829));
#37123=CARTESIAN_POINT('Ctrl Pts',(-1.04747189214599,-2.2892376209481,112.294378998187));
#37124=CARTESIAN_POINT('Ctrl Pts',(-1.12457420295903,-2.25395840717967,
112.289017656568));
#37125=CARTESIAN_POINT('Ctrl Pts',(-1.19980612546018,-2.21481909560088,
112.283656314949));
#37126=CARTESIAN_POINT('Ctrl Pts',(-1.27277206411672,-2.17206296474206,
112.278294973331));
#37127=CARTESIAN_POINT('Ctrl Pts',(-1.34573800277327,-2.12930683388324,
112.272933631712));
#37128=CARTESIAN_POINT('Ctrl Pts',(-1.41643756936656,-2.0829342182641,112.267572290094));
#37129=CARTESIAN_POINT('Ctrl Pts',(-1.48451012278353,-2.03323288025578,
112.262210948475));
#37130=CARTESIAN_POINT('Ctrl Pts',(-1.55068772048485,-1.98491509302979,
112.256998852102));
#37131=CARTESIAN_POINT('Ctrl Pts',(-1.61463601602439,-1.93326638368646,
112.251786755729));
#37132=CARTESIAN_POINT('Ctrl Pts',(-1.67599642208737,-1.87852129164147,
112.246574659355));
#37133=CARTESIAN_POINT('Ctrl Pts',(-1.73726957135127,-1.82385404917089,
112.241369974779));
#37134=CARTESIAN_POINT('Ctrl Pts',(-1.79596179018046,-1.76609947623745,
112.236165290202));
#37135=CARTESIAN_POINT('Ctrl Pts',(-1.85174473417749,-1.70553442927604,
112.230960605626));
#37136=CARTESIAN_POINT('Ctrl Pts',(-1.90746426549754,-1.64503823116848,
112.225761837606));
#37137=CARTESIAN_POINT('Ctrl Pts',(-1.9602807762888,-1.58173825061738,112.220563069587));
#37138=CARTESIAN_POINT('Ctrl Pts',(-2.00990135412894,-1.51594947035535,
112.215364301568));
#37139=CARTESIAN_POINT('Ctrl Pts',(-2.05949157030876,-1.45020094469505,
112.210168714552));
#37140=CARTESIAN_POINT('Ctrl Pts',(-2.10588945199941,-1.38196701550506,
112.204973127536));
#37141=CARTESIAN_POINT('Ctrl Pts',(-2.14884192972162,-1.31159620732536,
112.19977754052));
#37142=CARTESIAN_POINT('Ctrl Pts',(-2.19178162429527,-1.24124634230291,
112.19458349977));
#37143=CARTESIAN_POINT('Ctrl Pts',(-2.23127770634118,-1.16876126189922,
112.18938945902));
#37144=CARTESIAN_POINT('Ctrl Pts',(-2.26712091182993,-1.09451771166274,
112.18419541827));
#37145=CARTESIAN_POINT('Ctrl Pts',(-2.30296471405867,-1.02027292537342,
112.179001291047));
#37146=CARTESIAN_POINT('Ctrl Pts',(-2.33515531662749,-0.944270035186615,
112.173807163823));
#37147=CARTESIAN_POINT('Ctrl Pts',(-2.3635304945719,-0.866908213843155,
112.1686130366));
#37148=CARTESIAN_POINT('Ctrl Pts',(-2.39193263046187,-0.789472894607527,
112.163413974676));
#37149=CARTESIAN_POINT('Ctrl Pts',(-2.41651194329919,-0.710676508807594,
112.158214912753));
#37150=CARTESIAN_POINT('Ctrl Pts',(-2.43715550178047,-0.630935266205005,
112.153015850829));
#37151=CARTESIAN_POINT('Ctrl Pts',(-2.45780970186655,-0.551152917569743,
112.147814108826));
#37152=CARTESIAN_POINT('Ctrl Pts',(-2.47452401436576,-0.470425202882062,
112.142612366824));
#37153=CARTESIAN_POINT('Ctrl Pts',(-2.48723676413951,-0.389178017252802,
112.137410624821));
#37154=CARTESIAN_POINT('Ctrl Pts',(-2.49997002052968,-0.307799773835037,
112.13220049202));
#37155=CARTESIAN_POINT('Ctrl Pts',(-2.50868877897406,-0.225900853751341,
112.126990359219));
#37156=CARTESIAN_POINT('Ctrl Pts',(-2.51338333819124,-0.143911241057328,
112.121780226417));
#37157=CARTESIAN_POINT('Ctrl Pts',(-2.51614561607506,-0.0956685662137815,
112.11871458512));
#37158=CARTESIAN_POINT('Ctrl Pts',(-2.51751564850944,-0.0473944948304982,
112.115648943822));
#37159=CARTESIAN_POINT('Ctrl Pts',(-2.51749986513132,0.000824053271280102,
112.112583302525));
#37160=CARTESIAN_POINT('Ctrl Pts',(-2.51749986513115,0.000824053789601987,
112.112583302492));
#37161=CARTESIAN_POINT('Ctrl Pts',(-2.51748486373191,0.0466536113198584,
112.109669548558));
#37162=CARTESIAN_POINT('Ctrl Pts',(-2.51621849457345,0.0924610145605964,
112.106755794625));
#37163=CARTESIAN_POINT('Ctrl Pts',(-2.51370388884508,0.138199164994239,
112.103842040691));
#37164=CARTESIAN_POINT('Ctrl Pts',(-2.50916909978691,0.220682419441518,
112.098587435841));
#37165=CARTESIAN_POINT('Ctrl Pts',(-2.50056179900052,0.303094538210816,
112.093332830991));
#37166=CARTESIAN_POINT('Ctrl Pts',(-2.48788671813419,0.385001204844178,
112.088078226141));
#37167=CARTESIAN_POINT('Ctrl Pts',(-2.47505746494527,0.467904136603143,
112.082759707329));
#37168=CARTESIAN_POINT('Ctrl Pts',(-2.45806075103824,0.550288760222616,
112.077441188517));
#37169=CARTESIAN_POINT('Ctrl Pts',(-2.43695593026938,0.631705662413221,
112.072122669705));
#37170=CARTESIAN_POINT('Ctrl Pts',(-2.41585110950051,0.713122564603827,
112.066804150893));
#37171=CARTESIAN_POINT('Ctrl Pts',(-2.39063823988411,0.79357125371448,112.061485632081));
#37172=CARTESIAN_POINT('Ctrl Pts',(-2.36143112101026,0.872610629504506,
112.056167113269));
#37173=CARTESIAN_POINT('',(-2.51749910744234,-0.00211991202945377,112.387416697508));
#37174=CARTESIAN_POINT('Ctrl Pts',(-2.36143112095427,0.872610629656001,
112.333400434891));
#37175=CARTESIAN_POINT('Ctrl Pts',(-2.3650344949,0.862859293737455,112.334066402852));
#37176=CARTESIAN_POINT('Ctrl Pts',(-2.36857751691473,0.853085505298505,
112.334730382634));
#37177=CARTESIAN_POINT('Ctrl Pts',(-2.37687869028287,0.829735429620577,
112.336308382216));
#37178=CARTESIAN_POINT('Ctrl Pts',(-2.38158121680321,0.816139763304604,
112.337220539836));
#37179=CARTESIAN_POINT('Ctrl Pts',(-2.38986696712902,0.791502905673892,
112.338861746031));
#37180=CARTESIAN_POINT('Ctrl Pts',(-2.39349082628695,0.780475907393607,
112.339592108014));
#37181=CARTESIAN_POINT('Ctrl Pts',(-2.4011034084151,0.756759920999845,112.341154070631));
#37182=CARTESIAN_POINT('Ctrl Pts',(-2.40506810801852,0.744063547359317,
112.341984870282));
#37183=CARTESIAN_POINT('Ctrl Pts',(-2.4156536523985,0.709196055633934,112.344252095484));
#37184=CARTESIAN_POINT('Ctrl Pts',(-2.42206985904975,0.686963802837211,
112.345681889193));
#37185=CARTESIAN_POINT('Ctrl Pts',(-2.44042072433761,0.619921791530085,
112.3499487849));
#37186=CARTESIAN_POINT('Ctrl Pts',(-2.45142517742808,0.574866362517649,
112.352756647249));
#37187=CARTESIAN_POINT('Ctrl Pts',(-2.49877388886716,0.354796558801355,
112.366229596784));
#37188=CARTESIAN_POINT('Ctrl Pts',(-2.51765262075168,0.176565366880527,
112.376362442797));
#37189=CARTESIAN_POINT('Ctrl Pts',(-2.51749907092304,-0.00216284572706931,
112.386672407636));
#37190=CARTESIAN_POINT('Ctrl Pts',(-2.51749910744234,-0.00211991202945377,
112.387416697508));
#37191=CARTESIAN_POINT('Ctrl Pts',(-2.517394492057,-0.126355793312804,112.395287272283));
#37192=CARTESIAN_POINT('Ctrl Pts',(-2.50809026557141,-0.250215159424013,
112.403157847058));
#37193=CARTESIAN_POINT('Ctrl Pts',(-2.48977141696794,-0.372618492897856,
112.411028421832));
#37194=CARTESIAN_POINT('Ctrl Pts',(-2.48567305793243,-0.400003009172713,
112.412789255275));
#37195=CARTESIAN_POINT('Ctrl Pts',(-2.48112366278329,-0.427314773939724,
112.414550088717));
#37196=CARTESIAN_POINT('Ctrl Pts',(-2.47612558836571,-0.454541879963322,
112.416310922159));
#37197=CARTESIAN_POINT('Ctrl Pts',(-2.46120841196053,-0.535803483857776,
112.421566278699));
#37198=CARTESIAN_POINT('Ctrl Pts',(-2.44225918248003,-0.616480029859821,
112.426821635238));
#37199=CARTESIAN_POINT('Ctrl Pts',(-2.41933747375667,-0.696141105004374,
112.432076991778));
#37200=CARTESIAN_POINT('Ctrl Pts',(-2.39644826496086,-0.775689231363018,
112.437324896923));
#37201=CARTESIAN_POINT('Ctrl Pts',(-2.36959789113806,-0.854224307023324,
112.442572802068));
#37202=CARTESIAN_POINT('Ctrl Pts',(-2.33889710448583,-0.931325176631549,
112.447820707212));
#37203=CARTESIAN_POINT('Ctrl Pts',(-2.30797464785383,-1.00898274038578,
112.453106503993));
#37204=CARTESIAN_POINT('Ctrl Pts',(-2.27314602759454,-1.0851848340452,112.458392300773));
#37205=CARTESIAN_POINT('Ctrl Pts',(-2.23457591223811,-1.15951573617836,
112.463678097553));
#37206=CARTESIAN_POINT('Ctrl Pts',(-2.19635069926193,-1.23318195517964,
112.468916627587));
#37207=CARTESIAN_POINT('Ctrl Pts',(-2.15445085484626,-1.30500989711631,
112.47415515762));
#37208=CARTESIAN_POINT('Ctrl Pts',(-2.10908460417848,-1.37461572172637,
112.479393687653));
#37209=CARTESIAN_POINT('Ctrl Pts',(-2.06373328289616,-1.44419864005322,
112.484630493761));
#37210=CARTESIAN_POINT('Ctrl Pts',(-2.01491807268369,-1.51156050714949,
112.489867299869));
#37211=CARTESIAN_POINT('Ctrl Pts',(-1.96289159043833,-1.57634477643264,
112.495104105976));
#37212=CARTESIAN_POINT('Ctrl Pts',(-1.91086653752487,-1.64112726588717,
112.500340768213));
#37213=CARTESIAN_POINT('Ctrl Pts',(-1.85563067770148,-1.70333193921773,
112.505577430449));
#37214=CARTESIAN_POINT('Ctrl Pts',(-1.79747727089641,-1.76263487728196,
112.510814092685));
#37215=CARTESIAN_POINT('Ctrl Pts',(-1.73837457608633,-1.82290586813724,
112.516136237456));
#37216=CARTESIAN_POINT('Ctrl Pts',(-1.67625856063912,-1.88017917589626,
112.521458382228));
#37217=CARTESIAN_POINT('Ctrl Pts',(-1.61147511894358,-1.93415464506481,
112.526780526999));
#37218=CARTESIAN_POINT('Ctrl Pts',(-1.54764071556149,-1.98733940619305,
112.532024705562));
#37219=CARTESIAN_POINT('Ctrl Pts',(-1.48121693190589,-2.03732207957786,
112.537268884126));
#37220=CARTESIAN_POINT('Ctrl Pts',(-1.41256561689279,-2.08385811128596,
112.542513062689));
#37221=CARTESIAN_POINT('Ctrl Pts',(-1.34238332348644,-2.13143193315203,
112.547874190564));
#37222=CARTESIAN_POINT('Ctrl Pts',(-1.26987338934837,-2.17540327228873,
112.55323531844));
#37223=CARTESIAN_POINT('Ctrl Pts',(-1.19544907037609,-2.21556037384156,
112.558596446315));
#37224=CARTESIAN_POINT('Ctrl Pts',(-1.12102475140381,-2.25571747539439,
112.563957574191));
#37225=CARTESIAN_POINT('Ctrl Pts',(-1.04468653489811,-2.29206018128933,
112.569318702066));
#37226=CARTESIAN_POINT('Ctrl Pts',(-0.96686754316836,-2.32442969434818,
112.574679829942));
#37227=CARTESIAN_POINT('Ctrl Pts',(-0.89058272767988,-2.35616105293121,
112.579935264916));
#37228=CARTESIAN_POINT('Ctrl Pts',(-0.812593390130238,-2.38419164189191,
112.58519069989));
#37229=CARTESIAN_POINT('Ctrl Pts',(-0.733293014203989,-2.4083371037543,
112.590446134864));
#37230=CARTESIAN_POINT('Ctrl Pts',(-0.654105036246838,-2.43244834256484,
112.595694120943));
#37231=CARTESIAN_POINT('Ctrl Pts',(-0.573610148598829,-2.45268525887052,
112.600942107022));
#37232=CARTESIAN_POINT('Ctrl Pts',(-0.492221931378017,-2.46891146464803,
112.6061900931));
#37233=CARTESIAN_POINT('Ctrl Pts',(-0.4102476370936,-2.48525451543531,112.61147586996));
#37234=CARTESIAN_POINT('Ctrl Pts',(-0.327367531017245,-2.49752866920101,
112.616761646819));
#37235=CARTESIAN_POINT('Ctrl Pts',(-0.244019962235263,-2.50564572676001,
112.622047423679));
#37236=CARTESIAN_POINT('Ctrl Pts',(-0.161416032483974,-2.51369036276067,
112.627286040075));
#37237=CARTESIAN_POINT('Ctrl Pts',(-0.0783534159409274,-2.51765174180607,
112.632524656471));
#37238=CARTESIAN_POINT('Ctrl Pts',(0.00473254203868963,-2.51749555174301,
112.637763272866));
#37239=CARTESIAN_POINT('Ctrl Pts',(0.0877911870741211,-2.5173394130245,
112.643000167166));
#37240=CARTESIAN_POINT('Ctrl Pts',(0.170872697288985,-2.51306839434201,
112.648237061465));
#37241=CARTESIAN_POINT('Ctrl Pts',(0.253540453805012,-2.50470027913209,
112.653473955765));
#37242=CARTESIAN_POINT('Ctrl Pts',(0.336205966006391,-2.49633239110485,
112.65871070789));
#37243=CARTESIAN_POINT('Ctrl Pts',(0.418457287910135,-2.48386767519843,
112.663947460015));
#37244=CARTESIAN_POINT('Ctrl Pts',(0.49986304174694,-2.46737576982013,112.66918421214));
#37245=CARTESIAN_POINT('Ctrl Pts',(0.582594661855428,-2.4506152585993,112.674506255939));
#37246=CARTESIAN_POINT('Ctrl Pts',(0.664452438431347,-2.42969528180324,
112.679828299738));
#37247=CARTESIAN_POINT('Ctrl Pts',(0.744996318223181,-2.40474255084279,
112.685150343537));
#37248=CARTESIAN_POINT('Ctrl Pts',(0.824363193475616,-2.38015445935199,
112.690394615198));
#37249=CARTESIAN_POINT('Ctrl Pts',(0.902453900400525,-2.35165091673453,
112.695638886859));
#37250=CARTESIAN_POINT('Ctrl Pts',(0.978866290327585,-2.3194023013829,112.70088315852));
#37251=CARTESIAN_POINT('Ctrl Pts',(1.05697846488503,-2.28643631937415,112.706244088388));
#37252=CARTESIAN_POINT('Ctrl Pts',(1.13333629730785,-2.24955686941383,112.711605018256));
#37253=CARTESIAN_POINT('Ctrl Pts',(1.2075372273684,-2.20899526810707,112.716965948124));
#37254=CARTESIAN_POINT('Ctrl Pts',(1.28173815742895,-2.16843366680032,112.722326877992));
#37255=CARTESIAN_POINT('Ctrl Pts',(1.35378178735331,-2.12419023673152,112.72768780786));
#37256=CARTESIAN_POINT('Ctrl Pts',(1.42329915397842,-2.076541781011,112.733048737727));
#37257=CARTESIAN_POINT('Ctrl Pts',(1.49143551226082,-2.02983989329299,112.738303169187));
#37258=CARTESIAN_POINT('Ctrl Pts',(1.55739689094368,-1.97969447023556,112.743557600647));
#37259=CARTESIAN_POINT('Ctrl Pts',(1.6208144873514,-1.92633502994464,112.748812032107));
#37260=CARTESIAN_POINT('Ctrl Pts',(1.68414214036774,-1.87305126784548,112.754059011354));
#37261=CARTESIAN_POINT('Ctrl Pts',(1.74493282690168,-1.81656283733393,112.759305990602));
#37262=CARTESIAN_POINT('Ctrl Pts',(1.80284702815229,-1.75714223757853,112.76455296985));
#37263=CARTESIAN_POINT('Ctrl Pts',(1.86119223666162,-1.69727941969252,112.769838998002));
#37264=CARTESIAN_POINT('Ctrl Pts',(1.91661756868385,-1.63444086821441,112.775125026155));
#37265=CARTESIAN_POINT('Ctrl Pts',(1.96881021294934,-1.5689463328573,112.780411054307));
#37266=CARTESIAN_POINT('Ctrl Pts',(2.02052477966809,-1.50405171856625,112.785648663159));
#37267=CARTESIAN_POINT('Ctrl Pts',(2.06906534526677,-1.43654994610255,112.79088627201));
#37268=CARTESIAN_POINT('Ctrl Pts',(2.11416615756703,-1.36678736758804,112.796123880861));
#37269=CARTESIAN_POINT('Ctrl Pts',(2.15925215781729,-1.29704770056335,112.801359769572));
#37270=CARTESIAN_POINT('Ctrl Pts',(2.2009003979641,-1.22504908943391,112.806595658283));
#37271=CARTESIAN_POINT('Ctrl Pts',(2.23888812772545,-1.151167321257,112.811831546994));
#37272=CARTESIAN_POINT('Ctrl Pts',(2.27687484992131,-1.07728751267919,112.817067296831));
#37273=CARTESIAN_POINT('Ctrl Pts',(2.31120104462378,-1.00152505733288,112.822303046668));
#37274=CARTESIAN_POINT('Ctrl Pts',(2.3416903101504,-0.924279579644446,112.827538796505));
#37275=CARTESIAN_POINT('Ctrl Pts',(2.37268904082374,-0.845743356575832,
112.832862033922));
#37276=CARTESIAN_POINT('Ctrl Pts',(2.39972124217637,-0.765674547015846,
112.838185271339));
#37277=CARTESIAN_POINT('Ctrl Pts',(2.4226535098227,-0.684511666331364,112.843508508756));
#37278=CARTESIAN_POINT('Ctrl Pts',(2.44524135761816,-0.60456777138757,112.848751796442));
#37279=CARTESIAN_POINT('Ctrl Pts',(2.4638515439096,-0.523562915881689,112.853995084128));
#37280=CARTESIAN_POINT('Ctrl Pts',(2.4784081037197,-0.441927054406641,112.859238371814));
#37281=CARTESIAN_POINT('Ctrl Pts',(2.49329760150187,-0.35842401562299,112.864601584097));
#37282=CARTESIAN_POINT('Ctrl Pts',(2.50394569344754,-0.274261259748748,
112.869964796379));
#37283=CARTESIAN_POINT('Ctrl Pts',(2.51032728221455,-0.189903096787059,
112.875328008662));
#37284=CARTESIAN_POINT('Ctrl Pts',(2.51670887098156,-0.10554493382537,112.880691220945));
#37285=CARTESIAN_POINT('Ctrl Pts',(2.51882401098646,-0.0209918748079631,
112.886054433228));
#37286=CARTESIAN_POINT('Ctrl Pts',(2.51670418718245,0.0632952148137509,
112.891417645511));
#37287=CARTESIAN_POINT('Ctrl Pts',(2.51462662621131,0.145901876479592,112.896673931669));
#37288=CARTESIAN_POINT('Ctrl Pts',(2.50847378596393,0.228558455639894,112.901930217827));
#37289=CARTESIAN_POINT('Ctrl Pts',(2.49823752228716,0.310830391429945,112.907186503985));
#37290=CARTESIAN_POINT('Ctrl Pts',(2.48801577640484,0.392985643331266,112.912435335306));
#37291=CARTESIAN_POINT('Ctrl Pts',(2.47372216709517,0.474756881565425,112.917684166627));
#37292=CARTESIAN_POINT('Ctrl Pts',(2.45540054576482,0.555710724980039,112.922932997947));
#37293=CARTESIAN_POINT('Ctrl Pts',(2.4369507021753,0.637231116764084,112.928218562754));
#37294=CARTESIAN_POINT('Ctrl Pts',(2.41441624917947,0.717922152827627,112.93350412756));
#37295=CARTESIAN_POINT('Ctrl Pts',(2.38789507312428,0.797347709439735,112.938789692366));
#37296=CARTESIAN_POINT('Ctrl Pts',(2.36160532964296,0.87608017231575,112.944029133581));
#37297=CARTESIAN_POINT('Ctrl Pts',(2.33139831929238,0.953568710295907,112.949268574797));
#37298=CARTESIAN_POINT('Ctrl Pts',(2.29741997646057,1.0294016231578,112.954508016012));
#37299=CARTESIAN_POINT('Ctrl Pts',(2.26345286275538,1.10520947483927,112.959745725703));
#37300=CARTESIAN_POINT('Ctrl Pts',(2.22571708035768,1.17936236751307,112.964983435394));
#37301=CARTESIAN_POINT('Ctrl Pts',(2.1844066653329,1.25146864541194,112.970221145084));
#37302=CARTESIAN_POINT('Ctrl Pts',(2.14309745424578,1.32357282186827,112.975458702129));
#37303=CARTESIAN_POINT('Ctrl Pts',(2.09821404782988,1.39363010244888,112.980696259173));
#37304=CARTESIAN_POINT('Ctrl Pts',(2.04999571311091,1.46127472647237,112.985933816217));
#37305=CARTESIAN_POINT('Ctrl Pts',(2.00100861500654,1.52999783465486,112.99125487764));
#37306=CARTESIAN_POINT('Ctrl Pts',(1.9485795864765,1.5962302700184,112.996575939064));
#37307=CARTESIAN_POINT('Ctrl Pts',(1.89300325696989,1.65962192052931,113.001897000487));
#37308=CARTESIAN_POINT('Ctrl Pts',(1.83822091095501,1.72210793505335,113.007142043307));
#37309=CARTESIAN_POINT('Ctrl Pts',(1.78038098060945,1.78183351701213,113.012387086127));
#37310=CARTESIAN_POINT('Ctrl Pts',(1.71980284219268,1.83850059395856,113.017632128947));
#37311=CARTESIAN_POINT('Ctrl Pts',(1.65790772726718,1.89639962043509,113.022991199672));
#37312=CARTESIAN_POINT('Ctrl Pts',(1.593154337339,1.95110526570919,113.028350270397));
#37313=CARTESIAN_POINT('Ctrl Pts',(1.52591732836573,2.00234426535329,113.033709341121));
#37314=CARTESIAN_POINT('Ctrl Pts',(1.45868031939246,2.05358326499738,113.039068411846));
#37315=CARTESIAN_POINT('Ctrl Pts',(1.38896014656823,2.10135538743775,113.04442748257));
#37316=CARTESIAN_POINT('Ctrl Pts',(1.31715929980568,2.14543646583519,113.049786553295));
#37317=CARTESIAN_POINT('Ctrl Pts',(1.24673647755657,2.1886715262628,113.055042771043));
#37318=CARTESIAN_POINT('Ctrl Pts',(1.17405308457764,2.22851507030959,113.060298988791));
#37319=CARTESIAN_POINT('Ctrl Pts',(1.0994692615796,2.26472373433088,113.065555206539));
#37320=CARTESIAN_POINT('Ctrl Pts',(1.02499095534393,2.30088117248518,113.070803988102));
#37321=CARTESIAN_POINT('Ctrl Pts',(0.948617970996891,2.33341374532276,113.076052769665));
#37322=CARTESIAN_POINT('Ctrl Pts',(0.870737757582827,2.36212235236019,113.081301551228));
#37323=CARTESIAN_POINT('Ctrl Pts',(0.792311543702488,2.39103222891322,113.086587130805));
#37324=CARTESIAN_POINT('Ctrl Pts',(0.71235728434331,2.41606405520106,113.091872710382));
#37325=CARTESIAN_POINT('Ctrl Pts',(0.631294148703212,2.43706256542853,113.097158289959));
#37326=CARTESIAN_POINT('Ctrl Pts',(0.550938690802791,2.45787775955137,113.102397726651));
#37327=CARTESIAN_POINT('Ctrl Pts',(0.469494096436055,2.47472966663647,113.107637163342));
#37328=CARTESIAN_POINT('Ctrl Pts',(0.387385185996597,2.48751662661185,113.112876600033));
#37329=CARTESIAN_POINT('Ctrl Pts',(0.305303146901558,2.50029940186715,113.118114322042));
#37330=CARTESIAN_POINT('Ctrl Pts',(0.222557678887009,2.50901980121052,113.123352044051));
#37331=CARTESIAN_POINT('Ctrl Pts',(0.139582965417676,2.51362742779538,113.12858976606));
#37332=CARTESIAN_POINT('Ctrl Pts',(0.0566104053883257,2.51823493479865,
113.133827352135));
#37333=CARTESIAN_POINT('Ctrl Pts',(-0.0265909277041498,2.51872985673671,
113.139064938209));
#37334=CARTESIAN_POINT('Ctrl Pts',(-0.109583957800032,2.51511383563307,
113.144302524284));
#37335=CARTESIAN_POINT('Ctrl Pts',(-0.193899973960553,2.51144017179094,
113.14962360235));
#37336=CARTESIAN_POINT('Ctrl Pts',(-0.278000496800515,2.50352335519607,
113.154944680416));
#37337=CARTESIAN_POINT('Ctrl Pts',(-0.361431454613059,2.49141998740001,
113.160265758482));
#37338=CARTESIAN_POINT('Ctrl Pts',(-0.443671318679541,2.47948941212686,
113.165510870709));
#37339=CARTESIAN_POINT('Ctrl Pts',(-0.525260165375897,2.4634912036727,113.170755982935));
#37340=CARTESIAN_POINT('Ctrl Pts',(-0.605774102804838,2.44353104878391,
113.176001095161));
#37341=CARTESIAN_POINT('Ctrl Pts',(-0.68803718552538,2.42313726448811,113.181360156147));
#37342=CARTESIAN_POINT('Ctrl Pts',(-0.769177618051617,2.39860751598606,
113.186719217133));
#37343=CARTESIAN_POINT('Ctrl Pts',(-0.848762257034507,2.37010735643635,
113.19207827812));
#37344=CARTESIAN_POINT('Ctrl Pts',(-0.928346896017398,2.34160719688663,
113.197437339106));
#37345=CARTESIAN_POINT('Ctrl Pts',(-1.00637529954214,2.30913688217573,113.202796400093));
#37346=CARTESIAN_POINT('Ctrl Pts',(-1.08244036615458,2.27291203167196,113.208155461079));
#37347=CARTESIAN_POINT('Ctrl Pts',(-1.15692394512336,2.23744034100905,113.213403100501));
#37348=CARTESIAN_POINT('Ctrl Pts',(-1.22980151935485,2.1982370958742,113.218650739923));
#37349=CARTESIAN_POINT('Ctrl Pts',(-1.30067385925454,2.15547065900974,113.223898379344));
#37350=CARTESIAN_POINT('Ctrl Pts',(-1.37145410650413,2.11275979353621,113.2291391999));
#37351=CARTESIAN_POINT('Ctrl Pts',(-1.44023389914469,2.06649516329565,113.234380020455));
#37352=CARTESIAN_POINT('Ctrl Pts',(-1.50663601379298,2.01689220632685,113.23962084101));
#37353=CARTESIAN_POINT('Ctrl Pts',(-1.57297200614256,1.96733864329009,113.24485644283));
#37354=CARTESIAN_POINT('Ctrl Pts',(-1.63693465311243,1.91445362927206,113.250092044649));
#37355=CARTESIAN_POINT('Ctrl Pts',(-1.69817449725118,1.85849660394786,113.255327646469));
#37356=CARTESIAN_POINT('Ctrl Pts',(-1.75937195072917,1.80257831247921,113.260559624167));
#37357=CARTESIAN_POINT('Ctrl Pts',(-1.81785000481565,1.74359254496606,113.265791601865));
#37358=CARTESIAN_POINT('Ctrl Pts',(-1.87329228644203,1.68183895173016,113.271023579563));
#37359=CARTESIAN_POINT('Ctrl Pts',(-1.92872820551493,1.62009244533354,113.27625495684));
#37360=CARTESIAN_POINT('Ctrl Pts',(-1.98112872478702,1.55557907868882,113.281486334116));
#37361=CARTESIAN_POINT('Ctrl Pts',(-2.03021511929681,1.48863454863127,113.286717711393));
#37362=CARTESIAN_POINT('Ctrl Pts',(-2.07929599431949,1.42169754610706,113.291948500431));
#37363=CARTESIAN_POINT('Ctrl Pts',(-2.12506321658873,1.35233030042306,113.297179289469));
#37364=CARTESIAN_POINT('Ctrl Pts',(-2.16728017390901,1.28089925356405,113.302410078507));
#37365=CARTESIAN_POINT('Ctrl Pts',(-2.20952850283878,1.20941512597516,113.307644754567));
#37366=CARTESIAN_POINT('Ctrl Pts',(-2.24822106488964,1.13586453494511,113.312879430628));
#37367=CARTESIAN_POINT('Ctrl Pts',(-2.2831665462605,1.06063979372684,113.318114106689));
#37368=CARTESIAN_POINT('Ctrl Pts',(-2.31179587196648,0.999011407652224,
113.322402651016));
#37369=CARTESIAN_POINT('Ctrl Pts',(-2.33791103692983,0.936259932685513,
113.326691195344));
#37370=CARTESIAN_POINT('Ctrl Pts',(-2.36143112101026,0.872610629504504,
113.330979739671));
#37371=CARTESIAN_POINT('Origin',(0.,0.,116.208423447177));
#37372=CARTESIAN_POINT('',(-3.07507881988988,-0.00258943352280184,112.708423447177));
#37373=CARTESIAN_POINT('Ctrl Pts',(1.8746157427793,2.44019679077305,113.354075550313));
#37374=CARTESIAN_POINT('Ctrl Pts',(2.59111649989829,1.8811118882516,113.306858498602));
#37375=CARTESIAN_POINT('Ctrl Pts',(3.57307016162635,-0.0172528294224368,
113.206851810963));
#37376=CARTESIAN_POINT('Ctrl Pts',(2.0520963509033,-2.99395850450348,113.054055487396));
#37377=CARTESIAN_POINT('Ctrl Pts',(-1.39401273850626,-3.35130756079173,
112.895686579612));
#37378=CARTESIAN_POINT('Ctrl Pts',(-2.97703420005838,-1.39005018037111,
112.780475899539));
#37379=CARTESIAN_POINT('Ctrl Pts',(-3.07674611060127,-0.188293282082768,
112.718054855394));
#37380=CARTESIAN_POINT('Ctrl Pts',(-3.07507881988988,-0.00258943352280184,
112.708423447177));
#37381=CARTESIAN_POINT('Ctrl Pts',(-3.07507881988988,-0.00258943352280184,
112.708423447177));
#37382=CARTESIAN_POINT('Ctrl Pts',(-3.06760770968837,0.829547342602012,
112.665265219466));
#37383=CARTESIAN_POINT('Ctrl Pts',(-2.28977932831436,2.69183713313171,112.569317355827));
#37384=CARTESIAN_POINT('Ctrl Pts',(0.207333768054169,3.35545528762516,112.451210495639));
#37385=CARTESIAN_POINT('Ctrl Pts',(1.53027089159208,2.69684180982145,112.376261863162));
#37386=CARTESIAN_POINT('Ctrl Pts',(1.8696729405724,2.43383856956497,112.354102866614));
#37387=CARTESIAN_POINT('',(-3.07349937844406,0.00195466210857263,112.791576552787));
#37388=CARTESIAN_POINT('Ctrl Pts',(-3.07349937844406,0.00195466210857065,
112.791576552787));
#37389=CARTESIAN_POINT('Ctrl Pts',(-3.07343002419229,0.11100688591123,112.78595145356));
#37390=CARTESIAN_POINT('Ctrl Pts',(-3.06755261508276,0.219839360792043,
112.780326354332));
#37391=CARTESIAN_POINT('Ctrl Pts',(-3.05596138339884,0.327875392756234,
112.774701255105));
#37392=CARTESIAN_POINT('Ctrl Pts',(-3.04431879347594,0.436390108996588,
112.76905123228));
#37393=CARTESIAN_POINT('Ctrl Pts',(-3.02691175843935,0.544101106734187,
112.763401209456));
#37394=CARTESIAN_POINT('Ctrl Pts',(-3.00388543327814,0.650441814261192,
112.757751186631));
#37395=CARTESIAN_POINT('Ctrl Pts',(-2.9807318632009,0.757370167202966,112.752069941426));
#37396=CARTESIAN_POINT('Ctrl Pts',(-2.95189683807177,0.862912846042479,
112.746388696222));
#37397=CARTESIAN_POINT('Ctrl Pts',(-2.91757627648976,0.966514832200808,
112.740707451017));
#37398=CARTESIAN_POINT('Ctrl Pts',(-2.90215410924504,1.01306905753307,112.738154546587));
#37399=CARTESIAN_POINT('Ctrl Pts',(-2.88562493226943,1.05923171481558,112.735601642157));
#37400=CARTESIAN_POINT('Ctrl Pts',(-2.86800958296797,1.10495397279882,112.733048737727));
#37401=CARTESIAN_POINT('Ctrl Pts',(-2.83351112480162,1.19449789141844,112.728049048809));
#37402=CARTESIAN_POINT('Ctrl Pts',(-2.79475452621709,1.28258180731632,112.723049359891));
#37403=CARTESIAN_POINT('Ctrl Pts',(-2.75188381854915,1.36877233286159,112.718049670973));
#37404=CARTESIAN_POINT('Ctrl Pts',(-2.70907125272974,1.4548459656203,112.713056762703));
#37405=CARTESIAN_POINT('Ctrl Pts',(-2.66215586076226,1.53903092181659,112.708063854433));
#37406=CARTESIAN_POINT('Ctrl Pts',(-2.61133036493258,1.62091208126199,112.703070946162));
#37407=CARTESIAN_POINT('Ctrl Pts',(-2.56055847765614,1.70270687597206,112.698083304198));
#37408=CARTESIAN_POINT('Ctrl Pts',(-2.50588491546618,1.78220233358484,112.693095662233));
#37409=CARTESIAN_POINT('Ctrl Pts',(-2.44754862974388,1.85900724986183,112.688108020268));
#37410=CARTESIAN_POINT('Ctrl Pts',(-2.38925407682615,1.93575722118439,112.683123946379));
#37411=CARTESIAN_POINT('Ctrl Pts',(-2.32730227404646,2.00982012899545,112.67813987249));
#37412=CARTESIAN_POINT('Ctrl Pts',(-2.26197530990461,2.08083395478398,112.673155798601));
#37413=CARTESIAN_POINT('Ctrl Pts',(-2.19667213165785,2.15182192406086,112.66817353944));
#37414=CARTESIAN_POINT('Ctrl Pts',(-2.12799653063372,2.21976269443926,112.663191280279));
#37415=CARTESIAN_POINT('Ctrl Pts',(-2.0562700499957,2.28432828890479,112.658209021118));
#37416=CARTESIAN_POINT('Ctrl Pts',(-1.98455010812994,2.34888799740304,112.653227216152));
#37417=CARTESIAN_POINT('Ctrl Pts',(-1.90978016596492,2.41007284821533,112.648245411187));
#37418=CARTESIAN_POINT('Ctrl Pts',(-1.83231690711452,2.46759336234767,112.643263606221));
#37419=CARTESIAN_POINT('Ctrl Pts',(-1.75483956727324,2.52512433235092,112.638280895681));
#37420=CARTESIAN_POINT('Ctrl Pts',(-1.67466829084932,2.57898938117476,112.633298185141));
#37421=CARTESIAN_POINT('Ctrl Pts',(-1.59219007572955,2.62894142436615,112.628315474601));
#37422=CARTESIAN_POINT('Ctrl Pts',(-1.50962298743371,2.67894729264,112.623327395015));
#37423=CARTESIAN_POINT('Ctrl Pts',(-1.42474437381568,2.72503150986534,112.61833931543));
#37424=CARTESIAN_POINT('Ctrl Pts',(-1.33796705881446,2.76699230203616,112.613351235844));
#37425=CARTESIAN_POINT('Ctrl Pts',(-1.2511384940778,2.80897787579302,112.608360210353));
#37426=CARTESIAN_POINT('Ctrl Pts',(-1.16240939868322,2.84683500333169,112.603369184862));
#37427=CARTESIAN_POINT('Ctrl Pts',(-1.07221188821519,2.88041037297987,112.598378159371));
#37428=CARTESIAN_POINT('Ctrl Pts',(-0.981868668646718,2.91403998178479,
112.593379071153));
#37429=CARTESIAN_POINT('Ctrl Pts',(-0.890052715180372,2.94337388759342,
112.588379982936));
#37430=CARTESIAN_POINT('Ctrl Pts',(-0.797210516660054,2.96830888590231,
112.583380894719));
#37431=CARTESIAN_POINT('Ctrl Pts',(-0.743345628491891,2.9827755930332,112.580480539793));
#37432=CARTESIAN_POINT('Ctrl Pts',(-0.689135496025451,2.99576256182403,
112.577580184868));
#37433=CARTESIAN_POINT('Ctrl Pts',(-0.634668327413694,3.00725761519992,
112.574679829942));
#37434=CARTESIAN_POINT('Ctrl Pts',(-0.54076977135301,3.0270744872964,112.569679769419));
#37435=CARTESIAN_POINT('Ctrl Pts',(-0.445777316233022,3.04252410781941,
112.564679708896));
#37436=CARTESIAN_POINT('Ctrl Pts',(-0.350133011604329,3.05349130082024,
112.559679648374));
#37437=CARTESIAN_POINT('Ctrl Pts',(-0.252675795866729,3.06466637390449,
112.554584813099));
#37438=CARTESIAN_POINT('Ctrl Pts',(-0.15454219264561,3.07118717701671,112.549489977824));
#37439=CARTESIAN_POINT('Ctrl Pts',(-0.0562137622642027,3.07298588720028,
112.544395142549));
#37440=CARTESIAN_POINT('Ctrl Pts',(0.040033845638921,3.07474653314783,112.539408123983));
#37441=CARTESIAN_POINT('Ctrl Pts',(0.136467652143309,3.07198294492465,112.534421105417));
#37442=CARTESIAN_POINT('Ctrl Pts',(0.232629515719199,3.06468363104844,112.529434086851));
#37443=CARTESIAN_POINT('Ctrl Pts',(0.328727479536893,3.05738916758147,112.524450382169));
#37444=CARTESIAN_POINT('Ctrl Pts',(0.424553423212515,3.04556500077522,112.519466677487));
#37445=CARTESIAN_POINT('Ctrl Pts',(0.519650264770887,3.02925169841061,112.514482972805));
#37446=CARTESIAN_POINT('Ctrl Pts',(0.614709873716475,3.01294478308115,112.509501219359));
#37447=CARTESIAN_POINT('Ctrl Pts',(0.709040516019149,2.99215230062805,112.504519465913));
#37448=CARTESIAN_POINT('Ctrl Pts',(0.802192351484012,2.96696641053123,112.499537712467));
#37449=CARTESIAN_POINT('Ctrl Pts',(0.899010779616596,2.94078916691465,112.494359869909));
#37450=CARTESIAN_POINT('Ctrl Pts',(0.994555193225898,2.90986560914487,112.489182027351));
#37451=CARTESIAN_POINT('Ctrl Pts',(1.08833567477371,2.87435692095029,112.484004184794));
#37452=CARTESIAN_POINT('Ctrl Pts',(1.17860282536295,2.84017850715262,112.479020321561));
#37453=CARTESIAN_POINT('Ctrl Pts',(1.26723543317313,2.80175257466065,112.474036458329));
#37454=CARTESIAN_POINT('Ctrl Pts',(1.35381659437577,2.75927216468271,112.469052595097));
#37455=CARTESIAN_POINT('Ctrl Pts',(1.44042783864438,2.71677699466969,112.464067000196));
#37456=CARTESIAN_POINT('Ctrl Pts',(1.52498583030879,2.67022474944789,112.459081405295));
#37457=CARTESIAN_POINT('Ctrl Pts',(1.60709882997935,2.61985411820563,112.454095810394));
#37458=CARTESIAN_POINT('Ctrl Pts',(1.68929350361451,2.5694333856497,112.449105256555));
#37459=CARTESIAN_POINT('Ctrl Pts',(1.76903796889166,2.51518693317379,112.444114702716));
#37460=CARTESIAN_POINT('Ctrl Pts',(1.84597045576914,2.45739604590458,112.439124148876));
#37461=CARTESIAN_POINT('Ctrl Pts',(1.85481155648619,2.4507547026228,112.438550633176));
#37462=CARTESIAN_POINT('Ctrl Pts',(1.86361555744202,2.44406659195225,112.437977117475));
#37463=CARTESIAN_POINT('Ctrl Pts',(1.87238193903529,2.43733217358128,112.437403601774));
#37464=CARTESIAN_POINT('Ctrl Pts',(1.8723819390353,2.43733217358127,113.437353936953));
#37465=CARTESIAN_POINT('Ctrl Pts',(1.94902778074786,2.37845210328134,113.432362769506));
#37466=CARTESIAN_POINT('Ctrl Pts',(2.0228783853614,2.31596491432207,113.427371602059));
#37467=CARTESIAN_POINT('Ctrl Pts',(2.09358857238406,2.25017535751836,113.422380434612));
#37468=CARTESIAN_POINT('Ctrl Pts',(2.16437424616697,2.18431556698014,113.417383938837));
#37469=CARTESIAN_POINT('Ctrl Pts',(2.23201248708662,2.11514666725556,113.412387443062));
#37470=CARTESIAN_POINT('Ctrl Pts',(2.29619450083181,2.0430107841981,113.407390947287));
#37471=CARTESIAN_POINT('Ctrl Pts',(2.3604125894477,1.97083435562795,113.402391643125));
#37472=CARTESIAN_POINT('Ctrl Pts',(2.42117030685143,1.89568796237903,113.397392338963));
#37473=CARTESIAN_POINT('Ctrl Pts',(2.47820008932934,1.81794569975235,113.392393034801));
#37474=CARTESIAN_POINT('Ctrl Pts',(2.53532458293881,1.74007432813483,113.387385428139));
#37475=CARTESIAN_POINT('Ctrl Pts',(2.58870853348055,1.6595988406701,113.382377821478));
#37476=CARTESIAN_POINT('Ctrl Pts',(2.63812849265039,1.57692114776427,113.377370214816));
#37477=CARTESIAN_POINT('Ctrl Pts',(2.6738076304336,1.51723132109631,113.373754932832));
#37478=CARTESIAN_POINT('Ctrl Pts',(2.70742158929765,1.45639421551074,113.370139650847));
#37479=CARTESIAN_POINT('Ctrl Pts',(2.73890182080391,1.39456769860665,113.366524368863));
#37480=CARTESIAN_POINT('Ctrl Pts',(2.78238710748423,1.3091635041843,113.361530391183));
#37481=CARTESIAN_POINT('Ctrl Pts',(2.82195198542918,1.22157018123046,113.356536413502));
#37482=CARTESIAN_POINT('Ctrl Pts',(2.85737001572186,1.13218321982516,113.351542435822));
#37483=CARTESIAN_POINT('Ctrl Pts',(2.89273942558394,1.04291896520276,113.346555313671));
#37484=CARTESIAN_POINT('Ctrl Pts',(2.92397314004963,0.951866370848382,113.34156819152));
#37485=CARTESIAN_POINT('Ctrl Pts',(2.95089079206454,0.85944504379785,113.336581069369));
#37486=CARTESIAN_POINT('Ctrl Pts',(2.97777966031034,0.76712254535755,113.331599280081));
#37487=CARTESIAN_POINT('Ctrl Pts',(3.00036151800224,0.673434643831087,113.326617490794));
#37488=CARTESIAN_POINT('Ctrl Pts',(3.01850464563966,0.578819448750456,113.321635701507));
#37489=CARTESIAN_POINT('Ctrl Pts',(3.03663450464151,0.484273448715349,113.316657555558));
#37490=CARTESIAN_POINT('Ctrl Pts',(3.0503320039826,0.388801934157765,113.311679409608));
#37491=CARTESIAN_POINT('Ctrl Pts',(3.05951594227669,0.292855679396463,113.306701263659));
#37492=CARTESIAN_POINT('Ctrl Pts',(3.06869645062395,0.196945257906474,113.30172497691));
#37493=CARTESIAN_POINT('Ctrl Pts',(3.07336670507928,0.100560886087044,113.29674869016));
#37494=CARTESIAN_POINT('Ctrl Pts',(3.07349718469151,0.00416001121787148,
113.291772403411));
#37495=CARTESIAN_POINT('Ctrl Pts',(3.07362765141657,-0.0922313423484138,
113.286796608158));
#37496=CARTESIAN_POINT('Ctrl Pts',(3.06921923426622,-0.188638755635504,
113.281820812906));
#37497=CARTESIAN_POINT('Ctrl Pts',(3.06029453420285,-0.284604311155291,
113.276845017653));
#37498=CARTESIAN_POINT('Ctrl Pts',(3.05136826397639,-0.380586750331861,
113.271868346986));
#37499=CARTESIAN_POINT('Ctrl Pts',(3.03792417377253,-0.476126739170055,
113.266891676319));
#37500=CARTESIAN_POINT('Ctrl Pts',(3.0200366652607,-0.570772100300162,113.261915005653));
#37501=CARTESIAN_POINT('Ctrl Pts',(3.00212989325235,-0.665519387340322,
113.256932975487));
#37502=CARTESIAN_POINT('Ctrl Pts',(2.97977023157995,-0.759369690085068,
113.251950945322));
#37503=CARTESIAN_POINT('Ctrl Pts',(2.95308305439377,-0.851881872005937,
113.246968915156));
#37504=CARTESIAN_POINT('Ctrl Pts',(2.92638017443914,-0.944448488210441,
113.241983953558));
#37505=CARTESIAN_POINT('Ctrl Pts',(2.89534485085943,-1.03567499950709,113.236998991959));
#37506=CARTESIAN_POINT('Ctrl Pts',(2.86015140590259,-1.12513829608338,113.232014030361));
#37507=CARTESIAN_POINT('Ctrl Pts',(2.82490077734008,-1.21474695591924,113.227020969014));
#37508=CARTESIAN_POINT('Ctrl Pts',(2.78547871686333,-1.30258627922447,113.222027907666));
#37509=CARTESIAN_POINT('Ctrl Pts',(2.74210643107271,-1.38825594566337,113.217034846319));
#37510=CARTESIAN_POINT('Ctrl Pts',(2.71639613649571,-1.43903935078733,113.214075051239));
#37511=CARTESIAN_POINT('Ctrl Pts',(2.68929863301414,-1.489060862037,113.211115256159));
#37512=CARTESIAN_POINT('Ctrl Pts',(2.66086710191638,-1.53824202124994,113.208155461079));
#37513=CARTESIAN_POINT('Ctrl Pts',(2.61283286910437,-1.62133213846793,113.203154974631));
#37514=CARTESIAN_POINT('Ctrl Pts',(2.56081879647391,-1.70231576269226,113.198154488184));
#37515=CARTESIAN_POINT('Ctrl Pts',(2.50503479940379,-1.78078715847123,113.193154001736));
#37516=CARTESIAN_POINT('Ctrl Pts',(2.44932643402042,-1.85915216309257,113.188160294925));
#37517=CARTESIAN_POINT('Ctrl Pts',(2.38985855462289,-1.9350113541123,113.183166588113));
#37518=CARTESIAN_POINT('Ctrl Pts',(2.32688632254462,-2.0079846343921,113.178172881302));
#37519=CARTESIAN_POINT('Ctrl Pts',(2.26398050177324,-2.08088095613397,113.173184440917));
#37520=CARTESIAN_POINT('Ctrl Pts',(2.19757796042873,-2.15089708710934,113.168196000532));
#37521=CARTESIAN_POINT('Ctrl Pts',(2.12797579427881,-2.21768376216345,113.163207560147));
#37522=CARTESIAN_POINT('Ctrl Pts',(2.05842346278849,-2.28442261842972,113.158222691449));
#37523=CARTESIAN_POINT('Ctrl Pts',(1.98567637646282,-2.34793631260673,113.153237822752));
#37524=CARTESIAN_POINT('Ctrl Pts',(1.91006969057551,-2.40791113356469,113.148252954055));
#37525=CARTESIAN_POINT('Ctrl Pts',(1.83449056775726,-2.46786409018469,113.143269902635));
#37526=CARTESIAN_POINT('Ctrl Pts',(1.75605426011781,-2.5242804645642,113.138286851214));
#37527=CARTESIAN_POINT('Ctrl Pts',(1.6751295900509,-2.57688632006457,113.133303799794));
#37528=CARTESIAN_POINT('Ctrl Pts',(1.5942123538351,-2.62948734311894,113.128321206124));
#37529=CARTESIAN_POINT('Ctrl Pts',(1.51080757763404,-2.67827830426429,113.123338612453));
#37530=CARTESIAN_POINT('Ctrl Pts',(1.42531279674618,-2.72302876985014,113.118356018783));
#37531=CARTESIAN_POINT('Ctrl Pts',(1.33980255567569,-2.76778732774717,113.113372524101));
#37532=CARTESIAN_POINT('Ctrl Pts',(1.25220194807059,-2.80850373556424,113.108389029419));
#37533=CARTESIAN_POINT('Ctrl Pts',(1.16293184976043,-2.84499415866057,113.103405534736));
#37534=CARTESIAN_POINT('Ctrl Pts',(1.07356578717905,-2.88152380851845,113.098416682858));
#37535=CARTESIAN_POINT('Ctrl Pts',(0.982527057780247,-2.9138182378906,113.09342783098));
#37536=CARTESIAN_POINT('Ctrl Pts',(0.890254990788898,-2.94174239208253,
113.088438979101));
#37537=CARTESIAN_POINT('Ctrl Pts',(0.797928540084588,-2.96968300433415,
113.083447186871));
#37538=CARTESIAN_POINT('Ctrl Pts',(0.704367729648516,-2.99324810541254,
113.078455394642));
#37539=CARTESIAN_POINT('Ctrl Pts',(0.610023400508049,-3.01235351524893,
113.073463602412));
#37540=CARTESIAN_POINT('Ctrl Pts',(0.515526997266067,-3.03148972119211,
113.068463763887));
#37541=CARTESIAN_POINT('Ctrl Pts',(0.420244986836002,-3.04615181509973,
113.063463925362));
#37542=CARTESIAN_POINT('Ctrl Pts',(0.32463460720452,-3.05630735067748,113.058464086837));
#37543=CARTESIAN_POINT('Ctrl Pts',(0.269322002464767,-3.0621825404581,113.055571575657));
#37544=CARTESIAN_POINT('Ctrl Pts',(0.213899540344203,-3.0665504184687,113.052679064476));
#37545=CARTESIAN_POINT('Ctrl Pts',(0.158455515214029,-3.0694126636375,113.049786553295));
#37546=CARTESIAN_POINT('Ctrl Pts',(0.0626073974904463,-3.07436073173408,
113.044786163234));
#37547=CARTESIAN_POINT('Ctrl Pts',(-0.0336403558292232,-3.07482359911457,
113.039785773174));
#37548=CARTESIAN_POINT('Ctrl Pts',(-0.129833121082185,-3.07075652090329,
113.034785383113));
#37549=CARTESIAN_POINT('Ctrl Pts',(-0.225895770170549,-3.0666949440685,
113.029791756883));
#37550=CARTESIAN_POINT('Ctrl Pts',(-0.321903144356099,-3.05811561812003,
113.024798130653));
#37551=CARTESIAN_POINT('Ctrl Pts',(-0.417397502528618,-3.04502571005285,
113.019804504424));
#37552=CARTESIAN_POINT('Ctrl Pts',(-0.51279145266298,-3.0319495654374,113.014816128768));
#37553=CARTESIAN_POINT('Ctrl Pts',(-0.607673026698114,-3.01437232623717,
113.009827753112));
#37554=CARTESIAN_POINT('Ctrl Pts',(-0.701587525637013,-2.99235311984908,
113.004839377457));
#37555=CARTESIAN_POINT('Ctrl Pts',(-0.795435235314147,-2.97034957288053,
112.999854549389));
#37556=CARTESIAN_POINT('Ctrl Pts',(-0.888316811141023,-2.94391043854237,
112.994869721321));
#37557=CARTESIAN_POINT('Ctrl Pts',(-0.979786664578253,-2.91314612436703,
112.989884893253));
#37558=CARTESIAN_POINT('Ctrl Pts',(-1.07122344596474,-2.88239293340792,
112.984901867511));
#37559=CARTESIAN_POINT('Ctrl Pts',(-1.16124910366457,-2.84731780952579,
112.979918841769));
#37560=CARTESIAN_POINT('Ctrl Pts',(-1.24943309351804,-2.80808105203926,
112.974935816027));
#37561=CARTESIAN_POINT('Ctrl Pts',(-1.33760924880958,-2.76884778047809,
112.969953232994));
#37562=CARTESIAN_POINT('Ctrl Pts',(-1.42394366075278,-2.72545378896544,
112.96497064996));
#37563=CARTESIAN_POINT('Ctrl Pts',(-1.50802665397815,-2.67810714141378,
112.959988066927));
#37564=CARTESIAN_POINT('Ctrl Pts',(-1.59212510768468,-2.63075178815452,
112.955004567738));
#37565=CARTESIAN_POINT('Ctrl Pts',(-1.67397093819443,-2.57944255075047,
112.950021068549));
#37566=CARTESIAN_POINT('Ctrl Pts',(-1.7531808602772,-2.52443243545112,112.94503756936));
#37567=CARTESIAN_POINT('Ctrl Pts',(-1.8324763021253,-2.469362927944,112.940048689687));
#37568=CARTESIAN_POINT('Ctrl Pts',(-1.90912979301477,-2.41058481622441,
112.935059810014));
#37569=CARTESIAN_POINT('Ctrl Pts',(-1.98278892570486,-2.34839313704119,
112.930070930341));
#37570=CARTESIAN_POINT('Ctrl Pts',(-2.05649166654478,-2.28616463874315,
112.92507909712));
#37571=CARTESIAN_POINT('Ctrl Pts',(-2.12719619794431,-2.22051884737279,
112.920087263899));
#37572=CARTESIAN_POINT('Ctrl Pts',(-2.1945865282105,-2.15178814482211,112.915095430678));
#37573=CARTESIAN_POINT('Ctrl Pts',(-2.26208576240159,-2.08294637228203,
112.910095530569));
#37574=CARTESIAN_POINT('Ctrl Pts',(-2.32625980919352,-2.01101006127668,
112.905095630461));
#37575=CARTESIAN_POINT('Ctrl Pts',(-2.38683259562793,-1.93634511656575,
112.900095730352));
#37576=CARTESIAN_POINT('Ctrl Pts',(-2.42187701440332,-1.89314767189933,
112.897203035405));
#37577=CARTESIAN_POINT('Ctrl Pts',(-2.45571680882079,-1.84903746242192,
112.894310340458));
#37578=CARTESIAN_POINT('Ctrl Pts',(-2.48830532630393,-1.8040894803439,112.891417645511));
#37579=CARTESIAN_POINT('Ctrl Pts',(-2.54500547120761,-1.72588533686696,
112.88638470031));
#37580=CARTESIAN_POINT('Ctrl Pts',(-2.59811448861188,-1.64486892120071,
112.881351755109));
#37581=CARTESIAN_POINT('Ctrl Pts',(-2.64734378267396,-1.561401020346,112.876318809909));
#37582=CARTESIAN_POINT('Ctrl Pts',(-2.69650461378654,-1.47804919791147,
112.871292864002));
#37583=CARTESIAN_POINT('Ctrl Pts',(-2.7417962276114,-1.39225303355378,112.866266918094));
#37584=CARTESIAN_POINT('Ctrl Pts',(-2.7829717140169,-1.30440434259544,112.861240972187));
#37585=CARTESIAN_POINT('Ctrl Pts',(-2.8241006655227,-1.21665493473923,112.856220706405));
#37586=CARTESIAN_POINT('Ctrl Pts',(-2.86112255541327,-1.12685799962256,
112.851200440622));
#37587=CARTESIAN_POINT('Ctrl Pts',(-2.89383555741939,-1.0354313191203,112.846180174839));
#37588=CARTESIAN_POINT('Ctrl Pts',(-2.92651788308417,-0.944090373215514,
112.841164616768));
#37589=CARTESIAN_POINT('Ctrl Pts',(-2.95489921487249,-0.851123126818456,
112.836149058698));
#37590=CARTESIAN_POINT('Ctrl Pts',(-2.97882560649874,-0.756967803851286,
112.831133500627));
#37591=CARTESIAN_POINT('Ctrl Pts',(-3.00273870135661,-0.662864806430717,
112.826120729884));
#37592=CARTESIAN_POINT('Ctrl Pts',(-3.02220167352493,-0.56757546246408,
112.821107959142));
#37593=CARTESIAN_POINT('Ctrl Pts',(-3.03711049196263,-0.471552870429743,
112.8160951884));
#37594=CARTESIAN_POINT('Ctrl Pts',(-3.05201703766413,-0.375544916310658,
112.811083181816));
#37595=CARTESIAN_POINT('Ctrl Pts',(-3.0623707379808,-0.278804361265467,
112.806071175233));
#37596=CARTESIAN_POINT('Ctrl Pts',(-3.06811886878855,-0.181793445931633,
112.80105916865));
#37597=CARTESIAN_POINT('Ctrl Pts',(-3.071743984815,-0.120612544577855,112.797898296707));
#37598=CARTESIAN_POINT('Ctrl Pts',(-3.07353835017132,-0.0593242779513427,
112.794737424765));
#37599=CARTESIAN_POINT('Ctrl Pts',(-3.07349937844451,0.00195466141179594,
112.791576552823));
#37600=CARTESIAN_POINT('Origin',(0.,0.,10.));
#37601=CARTESIAN_POINT('',(2.51749986510683,0.000824128084735556,1.88741669747532));
#37602=CARTESIAN_POINT('Ctrl Pts',(2.36142200728636,0.872635292378022,0.943739684385605));
#37603=CARTESIAN_POINT('Ctrl Pts',(2.35741605103208,0.88347573550666,0.944474627125061));
#37604=CARTESIAN_POINT('Ctrl Pts',(2.3533359497583,0.894287232847126,0.945209569864519));
#37605=CARTESIAN_POINT('Ctrl Pts',(2.34918212370971,0.905068836963642,0.945944512603976));
#37606=CARTESIAN_POINT('Ctrl Pts',(2.31947828172392,0.982167651715261,0.951200058393829));
#37607=CARTESIAN_POINT('Ctrl Pts',(2.28592010378836,1.05794487781423,0.95645560418368));
#37608=CARTESIAN_POINT('Ctrl Pts',(2.24864585244449,1.13198855130438,0.961711149973533));
#37609=CARTESIAN_POINT('Ctrl Pts',(2.21142442782955,1.2059272868031,0.96695924736985));
#37610=CARTESIAN_POINT('Ctrl Pts',(2.17049759653951,1.27813694111076,0.972207344766169));
#37611=CARTESIAN_POINT('Ctrl Pts',(2.12605219964104,1.34822412617543,0.977455442162485));
#37612=CARTESIAN_POINT('Ctrl Pts',(2.08128793583427,1.41881414135464,0.982741191255221));
#37613=CARTESIAN_POINT('Ctrl Pts',(2.03295457895778,1.48725066327916,0.988026940347957));
#37614=CARTESIAN_POINT('Ctrl Pts',(1.98129091356592,1.5531556798406,0.993312689440693));
#37615=CARTESIAN_POINT('Ctrl Pts',(1.93008683787469,1.61847441847148,0.998551417559892));
#37616=CARTESIAN_POINT('Ctrl Pts',(1.8756117595696,1.68130614258371,1.00379014567909));
#37617=CARTESIAN_POINT('Ctrl Pts',(1.81814139472729,1.74131218303298,1.00902887379829));
#37618=CARTESIAN_POINT('Ctrl Pts',(1.76068992282892,1.80129849695431,1.01426587972559));
#37619=CARTESIAN_POINT('Ctrl Pts',(1.70024543888877,1.85846063917763,1.0195028856529));
#37620=CARTESIAN_POINT('Ctrl Pts',(1.63712222913025,1.91249498218625,1.0247398915802));
#37621=CARTESIAN_POINT('Ctrl Pts',(1.57400073599957,1.96652785573764,1.02997675508778));
#37622=CARTESIAN_POINT('Ctrl Pts',(1.50820101304804,2.01743279995885,1.03521361859535));
#37623=CARTESIAN_POINT('Ctrl Pts',(1.44007124555414,2.0649457759777,1.04045048210293));
#37624=CARTESIAN_POINT('Ctrl Pts',(1.37083503303633,2.11323037500102,1.0457723936267));
#37625=CARTESIAN_POINT('Ctrl Pts',(1.29919281266649,2.15801155432841,1.05109430515047));
#37626=CARTESIAN_POINT('Ctrl Pts',(1.22553999658496,2.19905842732078,1.05641621667424));
#37627=CARTESIAN_POINT('Ctrl Pts',(1.15296016317774,2.23950732475839,1.06166059798038));
#37628=CARTESIAN_POINT('Ctrl Pts',(1.07842837649574,2.27632985131858,1.06690497928653));
#37629=CARTESIAN_POINT('Ctrl Pts',(1.00234552948139,2.30935265594683,1.07214936059267));
#37630=CARTESIAN_POINT('Ctrl Pts',(0.92457552834666,2.34310774864106,1.07751003722525));
#37631=CARTESIAN_POINT('Ctrl Pts',(0.845185332141628,2.37289240318282,1.08287071385783));
#37632=CARTESIAN_POINT('Ctrl Pts',(0.764620117506867,2.39857506155296,1.08823139049041));
#37633=CARTESIAN_POINT('Ctrl Pts',(0.684054902872107,2.4242577199231,1.09359206712299));
#37634=CARTESIAN_POINT('Ctrl Pts',(0.602315177591028,2.44583831702018,1.09895274375557));
#37635=CARTESIAN_POINT('Ctrl Pts',(0.519855834697462,2.46324098722212,1.10431342038815));
#37636=CARTESIAN_POINT('Ctrl Pts',(0.439016490774304,2.48030176399125,1.10956878099078));
#37637=CARTESIAN_POINT('Ctrl Pts',(0.357187192540811,2.4934103011927,1.11482414159342));
#37638=CARTESIAN_POINT('Ctrl Pts',(0.274788740783649,2.50245827096848,1.12007950219605));
#37639=CARTESIAN_POINT('Ctrl Pts',(0.192507064452293,2.51149341792416,1.12532741487995));
#37640=CARTESIAN_POINT('Ctrl Pts',(0.109658291574247,2.51647937795004,1.13057532756386));
#37641=CARTESIAN_POINT('Ctrl Pts',(0.0266740919933808,2.51735868378273,
1.13582324024776));
#37642=CARTESIAN_POINT('Ctrl Pts',(-0.0569091383392196,2.51824433698319,
1.14110903557795));
#37643=CARTESIAN_POINT('Ctrl Pts',(-0.14062929514562,2.51496370024881,1.14639483090814));
#37644=CARTESIAN_POINT('Ctrl Pts',(-0.224039265615039,2.50751124772406,
1.15168062623833));
#37645=CARTESIAN_POINT('Ctrl Pts',(-0.306703640454684,2.50012541212775,
1.15691917223039));
#37646=CARTESIAN_POINT('Ctrl Pts',(-0.389062884281737,2.48864208789595,
1.16215771822245));
#37647=CARTESIAN_POINT('Ctrl Pts',(-0.470682834843838,2.47310814947171,
1.16739626421452));
#37648=CARTESIAN_POINT('Ctrl Pts',(-0.552275974182039,2.45757931376927,
1.1726330894039));
#37649=CARTESIAN_POINT('Ctrl Pts',(-0.633129849663377,2.43800259268168,
1.17786991459328));
#37650=CARTESIAN_POINT('Ctrl Pts',(-0.712818692105644,2.41447629149362,
1.18310673978267));
#37651=CARTESIAN_POINT('Ctrl Pts',(-0.792505392365057,2.39095062273587,
1.18834342419654));
#37652=CARTESIAN_POINT('Ctrl Pts',(-0.87102667963085,2.36347571660908,1.19358010861042));
#37653=CARTESIAN_POINT('Ctrl Pts',(-0.94797153545844,2.33219986664106,1.1988167930243));
#37654=CARTESIAN_POINT('Ctrl Pts',(-1.02617184959384,2.3004137093204,1.2041389209533));
#37655=CARTESIAN_POINT('Ctrl Pts',(-1.10274336598909,2.2647016303736,1.2094610488823));
#37656=CARTESIAN_POINT('Ctrl Pts',(-1.17727707310553,2.22526963380622,1.2147831768113));
#37657=CARTESIAN_POINT('Ctrl Pts',(-1.25071955316008,2.18641495002018,1.22002738496082));
#37658=CARTESIAN_POINT('Ctrl Pts',(-1.32218312830499,2.1439488445509,1.22527159311034));
#37659=CARTESIAN_POINT('Ctrl Pts',(-1.39130415572782,2.09811319910402,1.23051580125985));
#37660=CARTESIAN_POINT('Ctrl Pts',(-1.46196570987878,2.05125599712731,1.2358768890786));
#37661=CARTESIAN_POINT('Ctrl Pts',(-1.53017863021198,2.00087755633266,1.24123797689734));
#37662=CARTESIAN_POINT('Ctrl Pts',(-1.59559010990904,1.94727975677879,1.24659906471609));
#37663=CARTESIAN_POINT('Ctrl Pts',(-1.66100158960609,1.89368195722492,1.25196015253483));
#37664=CARTESIAN_POINT('Ctrl Pts',(-1.72361129743041,1.8368651896704,1.25732124035358));
#37665=CARTESIAN_POINT('Ctrl Pts',(-1.78310787212359,1.77716981922688,1.26268232817233));
#37666=CARTESIAN_POINT('Ctrl Pts',(-1.84142826271774,1.71865456286325,1.26793743297813));
#37667=CARTESIAN_POINT('Ctrl Pts',(-1.89697297047442,1.65715734036253,1.27319253778393));
#37668=CARTESIAN_POINT('Ctrl Pts',(-1.94942202226096,1.59297207418209,1.27844764258973));
#37669=CARTESIAN_POINT('Ctrl Pts',(-2.00179668862533,1.52887783821019,1.28369529438778));
#37670=CARTESIAN_POINT('Ctrl Pts',(-2.05108413004565,1.46210348521478,1.28894294618583));
#37671=CARTESIAN_POINT('Ctrl Pts',(-2.09700111239218,1.39297975025697,1.29419059798388));
#37672=CARTESIAN_POINT('Ctrl Pts',(-2.1432524159786,1.32335272584946,1.29947645789941));
#37673=CARTESIAN_POINT('Ctrl Pts',(-2.18608363723758,1.25134229844012,1.30476231781493));
#37674=CARTESIAN_POINT('Ctrl Pts',(-2.2252466527171,1.17732051055408,1.31004817773046));
#37675=CARTESIAN_POINT('Ctrl Pts',(-2.26405710768549,1.10396509524056,1.31528645230428));
#37676=CARTESIAN_POINT('Ctrl Pts',(-2.29926491670469,1.0286348033467,1.32052472687811));
#37677=CARTESIAN_POINT('Ctrl Pts',(-2.33067300630846,0.951719279864126,
1.32576300145193));
#37678=CARTESIAN_POINT('Ctrl Pts',(-2.36207075803671,0.874829072888122,
1.33099955186389));
#37679=CARTESIAN_POINT('Ctrl Pts',(-2.3896710999261,0.796355097461274,1.33623610227585));
#37680=CARTESIAN_POINT('Ctrl Pts',(-2.41332466618592,0.716707963942493,
1.3414726526878));
#37681=CARTESIAN_POINT('Ctrl Pts',(-2.43697758302428,0.637063017178899,
1.34670905932743));
#37682=CARTESIAN_POINT('Ctrl Pts',(-2.4566838092984,0.556245419012755,1.35194546596706));
#37683=CARTESIAN_POINT('Ctrl Pts',(-2.47234393902441,0.474680626494553,
1.35718187260669));
#37684=CARTESIAN_POINT('Ctrl Pts',(-2.48826138305951,0.391775628716241,
1.36250431955251));
#37685=CARTESIAN_POINT('Ctrl Pts',(-2.49999845664743,0.308099140257614,
1.36782676649832));
#37686=CARTESIAN_POINT('Ctrl Pts',(-2.50750523858282,0.224106511462149,
1.37314921344414));
#37687=CARTESIAN_POINT('Ctrl Pts',(-2.51490127421607,0.14135301191348,1.37839313921769));
#37688=CARTESIAN_POINT('Ctrl Pts',(-2.51819104635629,0.0582931078956557,
1.38363706499124));
#37689=CARTESIAN_POINT('Ctrl Pts',(-2.51737944929493,-0.0246365230413177,
1.38888099076478));
#37690=CARTESIAN_POINT('Ctrl Pts',(-2.51654962327054,-0.109428803866461,
1.39424269829674));
#37691=CARTESIAN_POINT('Ctrl Pts',(-2.51143198821274,-0.194084377305427,
1.39960440582869));
#37692=CARTESIAN_POINT('Ctrl Pts',(-2.50208769964345,-0.278142757038487,
1.40496611336064));
#37693=CARTESIAN_POINT('Ctrl Pts',(-2.49274341107416,-0.362201136771545,
1.41032782089259));
#37694=CARTESIAN_POINT('Ctrl Pts',(-2.47917261656255,-0.445661831741165,
1.41568952842455));
#37695=CARTESIAN_POINT('Ctrl Pts',(-2.46149135464734,-0.528078176974207,
1.4210512359565));
#37696=CARTESIAN_POINT('Ctrl Pts',(-2.44416098751678,-0.608858922562213,
1.42630653732701));
#37697=CARTESIAN_POINT('Ctrl Pts',(-2.42281783783166,-0.688934803476395,
1.43156183869753));
#37698=CARTESIAN_POINT('Ctrl Pts',(-2.39753427145321,-0.767877377715569,
1.43681714006804));
#37699=CARTESIAN_POINT('Ctrl Pts',(-2.37228654861054,-0.846708038115462,
1.44206499120073));
#37700=CARTESIAN_POINT('Ctrl Pts',(-2.34310964442233,-0.924408147350833,
1.44731284233341));
#37701=CARTESIAN_POINT('Ctrl Pts',(-2.31012680467993,-1.0005600413265,1.4525606934661));
#37702=CARTESIAN_POINT('Ctrl Pts',(-2.27690539007593,-1.07726276499748,
1.45784650389421));
#37703=CARTESIAN_POINT('Ctrl Pts',(-2.23982284843275,-1.15239431832373,
1.46313231432231));
#37704=CARTESIAN_POINT('Ctrl Pts',(-2.19905616306047,-1.22554405947145,
1.46841812475042));
#37705=CARTESIAN_POINT('Ctrl Pts',(-2.15865451862396,-1.29803878906462,
1.47365660395286));
#37706=CARTESIAN_POINT('Ctrl Pts',(-2.11463467386477,-1.36858664591832,
1.47889508315531));
#37707=CARTESIAN_POINT('Ctrl Pts',(-2.06721619339767,-1.43681016830841,
1.48413356235775));
#37708=CARTESIAN_POINT('Ctrl Pts',(-2.01981330608276,-1.5050112559904,1.48937031893217));
#37709=CARTESIAN_POINT('Ctrl Pts',(-1.96901426583195,-1.57088914864235,
1.49460707550659));
#37710=CARTESIAN_POINT('Ctrl Pts',(-1.91508219607761,-1.63409498875266,
1.499843832081));
#37711=CARTESIAN_POINT('Ctrl Pts',(-1.86115159404794,-1.69729910875893,
1.50508044614064));
#37712=CARTESIAN_POINT('Ctrl Pts',(-1.80408843232335,-1.757830970477,1.51031706020028));
#37713=CARTESIAN_POINT('Ctrl Pts',(-1.74419548713124,-1.81537554039681,
1.51555367425992));
#37714=CARTESIAN_POINT('Ctrl Pts',(-1.68332360005784,-1.87386066832983,
1.52087588004998));
#37715=CARTESIAN_POINT('Ctrl Pts',(-1.61952893661369,-1.92925962070465,
1.52619808584005));
#37716=CARTESIAN_POINT('Ctrl Pts',(-1.55316619771348,-1.98128266844493,
1.53152029163011));
#37717=CARTESIAN_POINT('Ctrl Pts',(-1.48777693586776,-2.03254258850062,
1.53676442582003));
#37718=CARTESIAN_POINT('Ctrl Pts',(-1.41989485917923,-2.080524769985,1.54200856000995));
#37719=CARTESIAN_POINT('Ctrl Pts',(-1.34988893798851,-2.12499555413565,
1.54725269419986));
#37720=CARTESIAN_POINT('Ctrl Pts',(-1.27831970603312,-2.17045942079122,
1.55261393579));
#37721=CARTESIAN_POINT('Ctrl Pts',(-1.20453107637456,-2.21225292119087,
1.55797517738014));
#37722=CARTESIAN_POINT('Ctrl Pts',(-1.12894246264074,-2.25017669662777,
1.56333641897027));
#37723=CARTESIAN_POINT('Ctrl Pts',(-1.05335384890691,-2.28810047206467,
1.56869766056041));
#37724=CARTESIAN_POINT('Ctrl Pts',(-0.975965742979037,-2.32215437904821,
1.57405890215054));
#37725=CARTESIAN_POINT('Ctrl Pts',(-0.897215838955941,-2.35219259167411,
1.57942014374068));
#37726=CARTESIAN_POINT('Ctrl Pts',(-0.820022679874984,-2.38163700248964,
1.58467540316064));
#37727=CARTESIAN_POINT('Ctrl Pts',(-0.741235998405527,-2.40733182677623,
1.58993066258061));
#37728=CARTESIAN_POINT('Ctrl Pts',(-0.661254560651124,-2.42910449672674,
1.59518592200058));
#37729=CARTESIAN_POINT('Ctrl Pts',(-0.581386513209035,-2.45084629939211,
1.600433730998));
#37730=CARTESIAN_POINT('Ctrl Pts',(-0.500327515397368,-2.46867687225071,
1.60568153999542));
#37731=CARTESIAN_POINT('Ctrl Pts',(-0.418494995123038,-2.4824721930078,
1.61092934899284));
#37732=CARTESIAN_POINT('Ctrl Pts',(-0.336069729768283,-2.49636743869064,
1.61621516993167));
#37733=CARTESIAN_POINT('Ctrl Pts',(-0.252860131598111,-2.50616855897815,
1.62150099087051));
#37734=CARTESIAN_POINT('Ctrl Pts',(-0.169307009444033,-2.51180042729376,
1.62678681180934));
#37735=CARTESIAN_POINT('Ctrl Pts',(-0.0865028875865664,-2.51738180951226,
1.63202524874446));
#37736=CARTESIAN_POINT('Ctrl Pts',(-0.00336184488425226,-2.5188683582142,
1.63726368567957));
#37737=CARTESIAN_POINT('Ctrl Pts',(0.0796799703382311,-2.51623873118727,
1.64250212261468));
#37738=CARTESIAN_POINT('Ctrl Pts',(0.162694478496319,-2.51360996887402,
1.64773883696781));
#37739=CARTESIAN_POINT('Ctrl Pts',(0.245609363154774,-2.50686773363573,
1.65297555132094));
#37740=CARTESIAN_POINT('Ctrl Pts',(0.327988753101664,-2.49604279367138,
1.65821226567407));
#37741=CARTESIAN_POINT('Ctrl Pts',(0.410365902771813,-2.48521814808722,
1.66344883761671));
#37742=CARTESIAN_POINT('Ctrl Pts',(0.492207129333078,-2.47031107966633,
1.66868540955935));
#37743=CARTESIAN_POINT('Ctrl Pts',(0.573083343760946,-2.45140403261147,
1.67392198150199));
#37744=CARTESIAN_POINT('Ctrl Pts',(0.65528290272542,-2.43218761725098,1.67924423733723));
#37745=CARTESIAN_POINT('Ctrl Pts',(0.736485102719983,-2.40883924168981,
1.68456649317246));
#37746=CARTESIAN_POINT('Ctrl Pts',(0.816253787080165,-2.38149868886743,
1.6898887490077));
#37747=CARTESIAN_POINT('Ctrl Pts',(0.894850982246054,-2.35455966156167,
1.69513284177368));
#37748=CARTESIAN_POINT('Ctrl Pts',(0.972056075902965,-2.32374516825423,
1.70037693453966));
#37749=CARTESIAN_POINT('Ctrl Pts',(1.04747219653616,-2.2892374816702,1.70562102730564));
#37750=CARTESIAN_POINT('Ctrl Pts',(1.12457443020833,-2.25395829080027,1.71098236467551));
#37751=CARTESIAN_POINT('Ctrl Pts',(1.19980627785168,-2.21481900996775,1.71634370204538));
#37752=CARTESIAN_POINT('Ctrl Pts',(1.27277214531568,-2.17206291716159,1.72170503941524));
#37753=CARTESIAN_POINT('Ctrl Pts',(1.34573801277968,-2.12930682435543,1.72706637678511));
#37754=CARTESIAN_POINT('Ctrl Pts',(1.4164375118487,-2.08293425409358,1.73242771415498));
#37755=CARTESIAN_POINT('Ctrl Pts',(1.48451000265987,-2.03323296796083,1.73778905152485));
#37756=CARTESIAN_POINT('Ctrl Pts',(1.55068750294995,-1.98491525785101,1.74300114088902));
#37757=CARTESIAN_POINT('Ctrl Pts',(1.61463571171944,-1.93326663287857,1.74821323025319));
#37758=CARTESIAN_POINT('Ctrl Pts',(1.67599604186995,-1.87852163086728,1.75342531961736));
#37759=CARTESIAN_POINT('Ctrl Pts',(1.73726911392309,-1.82385447955698,1.7586299970755));
#37760=CARTESIAN_POINT('Ctrl Pts',(1.79596126648459,-1.76610000357143,1.76383467453364));
#37761=CARTESIAN_POINT('Ctrl Pts',(1.8517441552362,-1.705535057848,1.76903935199177));
#37762=CARTESIAN_POINT('Ctrl Pts',(1.90746362981707,-1.64503896255333,1.77423811275552));
#37763=CARTESIAN_POINT('Ctrl Pts',(1.96028009502652,-1.58173908925178,1.77943687351927));
#37764=CARTESIAN_POINT('Ctrl Pts',(2.00990063841765,-1.51595041927113,1.78463563428302));
#37765=CARTESIAN_POINT('Ctrl Pts',(2.05949081933144,-1.45020200493593,1.78983121395996));
#37766=CARTESIAN_POINT('Ctrl Pts',(2.10588867698112,-1.3819681901832,1.79502679363691));
#37767=CARTESIAN_POINT('Ctrl Pts',(2.14884114177652,-1.3115974982473,1.80022237331385));
#37768=CARTESIAN_POINT('Ctrl Pts',(2.19178082278171,-1.2412477504916,1.80541640664878));
#37769=CARTESIAN_POINT('Ctrl Pts',(2.2312769024684,-1.16876278922474,1.81061043998372));
#37770=CARTESIAN_POINT('Ctrl Pts',(2.26712011663423,-1.09451935878376,1.81580447331866));
#37771=CARTESIAN_POINT('Ctrl Pts',(2.30296392706817,-1.02027469326965,1.82099859305869));
#37772=CARTESIAN_POINT('Ctrl Pts',(2.3351545489735,-0.944271924563801,1.82619271279873));
#37773=CARTESIAN_POINT('Ctrl Pts',(2.36352975717215,-0.866910224280322,
1.83138683253876));
#37774=CARTESIAN_POINT('Ctrl Pts',(2.3919319230396,-0.789475027052617,1.83658588691606));
#37775=CARTESIAN_POINT('Ctrl Pts',(2.41651127687384,-0.710678762869131,
1.84178494129336));
#37776=CARTESIAN_POINT('Ctrl Pts',(2.43715488713422,-0.630937640435078,
1.84698399567066));
#37777=CARTESIAN_POINT('Ctrl Pts',(2.45780913885177,-0.551155412703653,
1.85218573007891));
#37778=CARTESIAN_POINT('Ctrl Pts',(2.47452351384133,-0.470427817487587,
1.85738746448715));
#37779=CARTESIAN_POINT('Ctrl Pts',(2.48723633671725,-0.389180748898689,
1.8625891988954));
#37780=CARTESIAN_POINT('Ctrl Pts',(2.49996966634842,-0.307802622576515,
1.86779932409894));
#37781=CARTESIAN_POINT('Ctrl Pts',(2.50868850866609,-0.225903817148933,
1.87300944930248));
#37782=CARTESIAN_POINT('Ctrl Pts',(2.51338316214037,-0.143914315720466,
1.87821957450602));
#37783=CARTESIAN_POINT('Ctrl Pts',(2.51614555930706,-0.0956705917298165,
1.88128528216246));
#37784=CARTESIAN_POINT('Ctrl Pts',(2.51751565026114,-0.0473954685790145,
1.88435098981889));
#37785=CARTESIAN_POINT('Ctrl Pts',(2.51749986510683,0.000824128084736925,
1.88741669747533));
#37786=CARTESIAN_POINT('Ctrl Pts',(2.51749986510666,0.000824128598839498,
1.88741669750801));
#37787=CARTESIAN_POINT('Ctrl Pts',(2.51748486234407,0.0466536907109408,
1.89033045144168));
#37788=CARTESIAN_POINT('Ctrl Pts',(2.5162184915714,0.092461097738171,1.89324420537535));
#37789=CARTESIAN_POINT('Ctrl Pts',(2.51370388411283,0.13819925106905,1.89615795930902));
#37790=CARTESIAN_POINT('Ctrl Pts',(2.50916908870937,0.220682569402365,1.90141256789624));
#37791=CARTESIAN_POINT('Ctrl Pts',(2.50056177537896,0.303094749686193,1.90666717648346));
#37792=CARTESIAN_POINT('Ctrl Pts',(2.4878866763403,0.385001474917191,1.91192178507068));
#37793=CARTESIAN_POINT('Ctrl Pts',(2.47505675342768,0.467908674895217,1.91724057768164));
#37794=CARTESIAN_POINT('Ctrl Pts',(2.45805894040082,0.550297511071083,1.92255937029261));
#37795=CARTESIAN_POINT('Ctrl Pts',(2.43695260213126,0.631718501364096,1.92787816290357));
#37796=CARTESIAN_POINT('Ctrl Pts',(2.41584626386169,0.713139491657106,1.93319695551454));
#37797=CARTESIAN_POINT('Ctrl Pts',(2.39063145838279,0.793592144292747,1.93851574812551));
#37798=CARTESIAN_POINT('Ctrl Pts',(2.36142200728636,0.872635292378021,1.94383454073647));
#37799=CARTESIAN_POINT('Ctrl Pts',(2.36142200724207,0.872635292497862,1.66658329180866));
#37800=CARTESIAN_POINT('Ctrl Pts',(2.36656543969622,0.858716746348728,1.66563271745266));
#37801=CARTESIAN_POINT('Ctrl Pts',(2.37158585374055,0.844752622564022,1.66468620664304));
#37802=CARTESIAN_POINT('Ctrl Pts',(2.38080595803352,0.818376983810189,1.66291166730899));
#37803=CARTESIAN_POINT('Ctrl Pts',(2.38503272622791,0.805975683755325,1.6620827793949));
#37804=CARTESIAN_POINT('Ctrl Pts',(2.39282966260543,0.782500991670894,1.66052385439014));
#37805=CARTESIAN_POINT('Ctrl Pts',(2.39642023989896,0.771434791357363,1.65979316648514));
#37806=CARTESIAN_POINT('Ctrl Pts',(2.40436963235919,0.746343492191642,1.6581457159186));
#37807=CARTESIAN_POINT('Ctrl Pts',(2.4086827141935,0.732304263350909,1.65723046023622));
#37808=CARTESIAN_POINT('Ctrl Pts',(2.42139113165543,0.689610577587668,1.65446630588026));
#37809=CARTESIAN_POINT('Ctrl Pts',(2.42939997034476,0.660843143891866,1.65262986890035));
#37810=CARTESIAN_POINT('Ctrl Pts',(2.49059591268727,0.424858194389506,1.63776019526306));
#37811=CARTESIAN_POINT('Ctrl Pts',(2.51768324236378,0.211782042153157,1.62565128598905));
#37812=CARTESIAN_POINT('Ctrl Pts',(2.51739093025033,-0.127785717720968,
1.60606337558893));
#37813=CARTESIAN_POINT('Ctrl Pts',(2.50788069886021,-0.253203986703153,
1.59873916266813));
#37814=CARTESIAN_POINT('Ctrl Pts',(2.48700526467906,-0.3908940581761,1.59010798259596));
#37815=CARTESIAN_POINT('Ctrl Pts',(2.48484474075353,-0.404400725109235,
1.58925487696615));
#37816=CARTESIAN_POINT('Ctrl Pts',(2.48118054135853,-0.426168831867675,
1.58786859686673));
#37817=CARTESIAN_POINT('Ctrl Pts',(2.47974537598193,-0.434441730935338,
1.58733908762811));
#37818=CARTESIAN_POINT('Ctrl Pts',(2.47712211251085,-0.449126725621398,
1.58639419630881));
#37819=CARTESIAN_POINT('Ctrl Pts',(2.4759504515319,-0.45554158541987,1.58597973779078));
#37820=CARTESIAN_POINT('Ctrl Pts',(2.47334715535131,-0.46948787875069,1.58507491750255));
#37821=CARTESIAN_POINT('Ctrl Pts',(2.47190606094343,-0.477017233788878,
1.58458405255122));
#37822=CARTESIAN_POINT('Ctrl Pts',(2.46771816485463,-0.498369261827021,
1.58318553733568));
#37823=CARTESIAN_POINT('Ctrl Pts',(2.46488970136792,-0.512175361361853,
1.58227351696751));
#37824=CARTESIAN_POINT('Ctrl Pts',(2.44477084175596,-0.60634955073007,1.57600275167017));
#37825=CARTESIAN_POINT('Ctrl Pts',(2.4236703567482,-0.685845053535465,1.57046285555256));
#37826=CARTESIAN_POINT('Ctrl Pts',(2.3483866980391,-0.922163718528844,1.5535083985936));
#37827=CARTESIAN_POINT('Ctrl Pts',(2.28255663280725,-1.07482428696749,1.5419208038596));
#37828=CARTESIAN_POINT('Ctrl Pts',(2.15183824649078,-1.31079994526167,1.5236467305738));
#37829=CARTESIAN_POINT('Ctrl Pts',(2.09590038454559,-1.39850304947431,1.51675438044685));
#37830=CARTESIAN_POINT('Ctrl Pts',(2.02104047874389,-1.50124587682293,1.50856553305453));
#37831=CARTESIAN_POINT('Ctrl Pts',(2.00712864537521,-1.51979553198557,1.50708190695098));
#37832=CARTESIAN_POINT('Ctrl Pts',(1.98474553343597,-1.54879704001827,1.50475341472479));
#37833=CARTESIAN_POINT('Ctrl Pts',(1.97644361486455,-1.55937736046654,1.50390201356791));
#37834=CARTESIAN_POINT('Ctrl Pts',(1.96082482738877,-1.57895749080838,1.50232258882636));
#37835=CARTESIAN_POINT('Ctrl Pts',(1.95352981079476,-1.58797419596896,1.50159372919805));
#37836=CARTESIAN_POINT('Ctrl Pts',(1.93716559474296,-1.60791707663917,1.49997805037261));
#37837=CARTESIAN_POINT('Ctrl Pts',(1.92806569741186,-1.61881763838051,1.49909249317092));
#37838=CARTESIAN_POINT('Ctrl Pts',(1.90113476112544,-1.65052835088087,1.49650859240089));
#37839=CARTESIAN_POINT('Ctrl Pts',(1.88305523784894,-1.67112545256159,1.49482038667756));
#37840=CARTESIAN_POINT('Ctrl Pts',(1.76354870964592,-1.80287063360472,1.48394694410274));
#37841=CARTESIAN_POINT('Ctrl Pts',(1.65266250970589,-1.90503574388943,1.47518536761765));
#37842=CARTESIAN_POINT('Ctrl Pts',(1.40600277148995,-2.09445070982781,1.45727959958589));
#37843=CARTESIAN_POINT('Ctrl Pts',(1.26965976969582,-2.179798451262,1.44818533483113));
#37844=CARTESIAN_POINT('Ctrl Pts',(1.09175449762358,-2.26877861709355,1.43618752125606));
#37845=CARTESIAN_POINT('Ctrl Pts',(1.05698270855391,-2.28518521912782,1.43383570487106));
#37846=CARTESIAN_POINT('Ctrl Pts',(1.01111560348713,-2.30555621739638,1.43070726752831));
#37847=CARTESIAN_POINT('Ctrl Pts',(1.00034708024753,-2.31024889171167,1.42997092878311));
#37848=CARTESIAN_POINT('Ctrl Pts',(0.982967518019296,-2.31767821291206,
1.42877894484695));
#37849=CARTESIAN_POINT('Ctrl Pts',(0.976376817056206,-2.32046239964535,
1.42832609374267));
#37850=CARTESIAN_POINT('Ctrl Pts',(0.963628097224575,-2.32578406140048,
1.42744836388935));
#37851=CARTESIAN_POINT('Ctrl Pts',(0.95747176652422,-2.32832523979474,1.42702370890395));
#37852=CARTESIAN_POINT('Ctrl Pts',(0.942613873060686,-2.33438931317987,
1.42599701260429));
#37853=CARTESIAN_POINT('Ctrl Pts',(0.93390259285422,-2.33788800406963,1.42539356082793));
#37854=CARTESIAN_POINT('Ctrl Pts',(0.903454709871901,-2.34991938714786,
1.42327967486417));
#37855=CARTESIAN_POINT('Ctrl Pts',(0.881619858616303,-2.35819801369008,
1.4217554696473));
#37856=CARTESIAN_POINT('Ctrl Pts',(0.827386175562193,-2.37790211697935,
1.41795467061492));
#37857=CARTESIAN_POINT('Ctrl Pts',(0.794863207675124,-2.38897019878293,
1.41566238926392));
#37858=CARTESIAN_POINT('Ctrl Pts',(0.65531274963024,-2.43329643217257,1.40579971212265));
#37859=CARTESIAN_POINT('Ctrl Pts',(0.546358666576271,-2.46005207385707,
1.39803880137519));
#37860=CARTESIAN_POINT('Ctrl Pts',(0.262868816349941,-2.50990121328572,
1.37816170852405));
#37861=CARTESIAN_POINT('Ctrl Pts',(0.0870067161732809,-2.52213284563033,
1.36616427820632));
#37862=CARTESIAN_POINT('Ctrl Pts',(-0.121636934455914,-2.5147754627749,
1.35259908983483));
#37863=CARTESIAN_POINT('Ctrl Pts',(-0.15452987533737,-2.51296873385376,
1.35047852459925));
#37864=CARTESIAN_POINT('Ctrl Pts',(-0.202446906603256,-2.50939231696444,
1.34741431040695));
#37865=CARTESIAN_POINT('Ctrl Pts',(-0.217504439501805,-2.50813205103853,
1.34645499664912));
#37866=CARTESIAN_POINT('Ctrl Pts',(-0.24422201692004,-2.5056534607268,1.3447589458145));
#37867=CARTESIAN_POINT('Ctrl Pts',(-0.2558864989076,-2.50448912275189,1.34402055233592));
#37868=CARTESIAN_POINT('Ctrl Pts',(-0.280220601410862,-2.50188833337961,
1.34248430342288));
#37869=CARTESIAN_POINT('Ctrl Pts',(-0.292888322795294,-2.50043701341345,
1.34168693361905));
#37870=CARTESIAN_POINT('Ctrl Pts',(-0.325975323416193,-2.49639139380267,
1.3396101343631));
#37871=CARTESIAN_POINT('Ctrl Pts',(-0.34637503332979,-2.49364277267559,
1.33833554342853));
#37872=CARTESIAN_POINT('Ctrl Pts',(-0.440190940368616,-2.47982868701533,
1.33249805008895));
#37873=CARTESIAN_POINT('Ctrl Pts',(-0.513132614592708,-2.46576861029378,
1.32802935804034));
#37874=CARTESIAN_POINT('Ctrl Pts',(-0.727243864530593,-2.414582092351,1.31499916526967));
#37875=CARTESIAN_POINT('Ctrl Pts',(-0.865919528759469,-2.36839103674545,
1.30668866142716));
#37876=CARTESIAN_POINT('Ctrl Pts',(-1.04957041471071,-2.28891828583806,
1.29516554157286));
#37877=CARTESIAN_POINT('Ctrl Pts',(-1.09861214049467,-2.26578816326281,
1.29203207360484));
#37878=CARTESIAN_POINT('Ctrl Pts',(-1.17895241075164,-2.22467447114124,
1.28674773770486));
#37879=CARTESIAN_POINT('Ctrl Pts',(-1.21067995163597,-2.20756860751117,
1.28462002908492));
#37880=CARTESIAN_POINT('Ctrl Pts',(-1.28484763643677,-2.16550136465571,
1.27952356771145));
#37881=CARTESIAN_POINT('Ctrl Pts',(-1.32694241878387,-2.13996558501632,
1.27653312981781));
#37882=CARTESIAN_POINT('Ctrl Pts',(-1.37898932053784,-2.10626639598085,
1.27267529347276));
#37883=CARTESIAN_POINT('Ctrl Pts',(-1.38966687462304,-2.09923691815071,
1.27187509398411));
#37884=CARTESIAN_POINT('Ctrl Pts',(-1.406426091292,-2.08801973545374,1.27060446596708));
#37885=CARTESIAN_POINT('Ctrl Pts',(-1.41254382697707,-2.08388596124216,
1.27013752462182));
#37886=CARTESIAN_POINT('Ctrl Pts',(-1.42406967394163,-2.07602383463924,
1.26925172190527));
#37887=CARTESIAN_POINT('Ctrl Pts',(-1.42948146327859,-2.07230117032128,
1.26883323387935));
#37888=CARTESIAN_POINT('Ctrl Pts',(-1.44215159956868,-2.06351238505439,
1.26784747427176));
#37889=CARTESIAN_POINT('Ctrl Pts',(-1.4493978514199,-2.05842912486194,1.26727906805272));
#37890=CARTESIAN_POINT('Ctrl Pts',(-1.47309527551402,-2.04161816728942,
1.26540534249235));
#37891=CARTESIAN_POINT('Ctrl Pts',(-1.48943161417041,-2.02973097663667,
1.26408996742194));
#37892=CARTESIAN_POINT('Ctrl Pts',(-1.57971103058448,-1.96236211027759,
1.25669561353447));
#37893=CARTESIAN_POINT('Ctrl Pts',(-1.65069118883201,-1.90304157608034,
1.25040991818945));
#37894=CARTESIAN_POINT('Ctrl Pts',(-1.76600654219503,-1.79535462737379,
1.23956359173785));
#37895=CARTESIAN_POINT('Ctrl Pts',(-1.81201595312015,-1.74890691488186,
1.23504028551456));
#37896=CARTESIAN_POINT('Ctrl Pts',(-1.97026482301445,-1.57619433766027,
1.21886823707869));
#37897=CARTESIAN_POINT('Ctrl Pts',(-2.0715606228624,-1.44048142063773,1.20736201829065));
#37898=CARTESIAN_POINT('Ctrl Pts',(-2.1755690361032,-1.26720336113626,1.19422814539507));
#37899=CARTESIAN_POINT('Ctrl Pts',(-2.19206581820173,-1.23844766104923,
1.19209385732476));
#37900=CARTESIAN_POINT('Ctrl Pts',(-2.21526099540895,-1.1960995056953,1.18901456229561));
#37901=CARTESIAN_POINT('Ctrl Pts',(-2.22241172162173,-1.18276010298937,
1.18805362881769));
#37902=CARTESIAN_POINT('Ctrl Pts',(-2.23488197523751,-1.15898489114969,
1.18635660193945));
#37903=CARTESIAN_POINT('Ctrl Pts',(-2.24024972895498,-1.14857502174127,
1.18561883144596));
#37904=CARTESIAN_POINT('Ctrl Pts',(-2.25129047338053,-1.12679145533303,
1.18408575018006));
#37905=CARTESIAN_POINT('Ctrl Pts',(-2.25695038380481,-1.11541147288014,
1.18329091072057));
#37906=CARTESIAN_POINT('Ctrl Pts',(-2.27149189740842,-1.08560997626709,
1.18122484708161));
#37907=CARTESIAN_POINT('Ctrl Pts',(-2.28023575827393,-1.06712201058154,
1.17995838622634));
#37908=CARTESIAN_POINT('Ctrl Pts',(-2.31914163026448,-0.982197374822059,
1.17420746917555));
#37909=CARTESIAN_POINT('Ctrl Pts',(-2.34663354137771,-0.914572072470814,
1.16981388960174));
#37910=CARTESIAN_POINT('Ctrl Pts',(-2.41863151487462,-0.712740190435884,
1.15712255284373));
#37911=CARTESIAN_POINT('Ctrl Pts',(-2.45482131764587,-0.575874891250182,
1.14905874520011));
#37912=CARTESIAN_POINT('Ctrl Pts',(-2.50210461114167,-0.307421040012571,
1.13337671137171));
#37913=CARTESIAN_POINT('Ctrl Pts',(-2.51472556831109,-0.176584357740824,
1.12578562450538));
#37914=CARTESIAN_POINT('Ctrl Pts',(-2.51747699164142,-0.0239675245480319,
1.11641198267612));
#37915=CARTESIAN_POINT('Ctrl Pts',(-2.51758977161679,-0.00255291875063406,
1.11508469686271));
#37916=CARTESIAN_POINT('Ctrl Pts',(-2.51736627858063,0.0272793813710361,
1.11321572584653));
#37917=CARTESIAN_POINT('Ctrl Pts',(-2.51726096245127,0.0356985622833955,
1.11268605584854));
#37918=CARTESIAN_POINT('Ctrl Pts',(-2.51700638023353,0.0502238825068801,
1.11176817023207));
#37919=CARTESIAN_POINT('Ctrl Pts',(-2.5168771215311,0.0563303622931436,
1.11138104914158));
#37920=CARTESIAN_POINT('Ctrl Pts',(-2.51655739789115,0.0692180181425276,
1.11056130419081));
#37921=CARTESIAN_POINT('Ctrl Pts',(-2.51636174345143,0.0759989717104931,
1.11012838721149));
#37922=CARTESIAN_POINT('Ctrl Pts',(-2.51580817111654,0.0928252914642239,
1.10905030570795));
#37923=CARTESIAN_POINT('Ctrl Pts',(-2.51541749435442,0.102869381056326,
1.10840337456075));
#37924=CARTESIAN_POINT('Ctrl Pts',(-2.51371669962756,0.140752802940339,
1.10595120031646));
#37925=CARTESIAN_POINT('Ctrl Pts',(-2.51200451551857,0.16857093217028,1.10412582232164));
#37926=CARTESIAN_POINT('Ctrl Pts',(-2.50642071789218,0.239944187505855,
1.09938838297947));
#37927=CARTESIAN_POINT('Ctrl Pts',(-2.50187559255897,0.283436266433752,
1.09644979197519));
#37928=CARTESIAN_POINT('Ctrl Pts',(-2.48000642087177,0.450487332390012,
1.08501403096829));
#37929=CARTESIAN_POINT('Ctrl Pts',(-2.45463985197404,0.572811289169149,
1.07633449028049));
#37930=CARTESIAN_POINT('Ctrl Pts',(-2.37586517245021,0.848032835916339,
1.05662272753545));
#37931=CARTESIAN_POINT('Ctrl Pts',(-2.31657169888543,0.998702906564747,
1.04571316478046));
#37932=CARTESIAN_POINT('Ctrl Pts',(-2.23313614944323,1.16249913871672,1.03385680195097));
#37933=CARTESIAN_POINT('Ctrl Pts',(-2.22277443712753,1.18219083188889,1.03243078460233));
#37934=CARTESIAN_POINT('Ctrl Pts',(-2.2052806196052,1.21439321907345,1.03009714934354));
#37935=CARTESIAN_POINT('Ctrl Pts',(-2.19829999591787,1.22698436978636,1.02918427653099));
#37936=CARTESIAN_POINT('Ctrl Pts',(-2.18549288326325,1.24962474966612,1.02754182461858));
#37937=CARTESIAN_POINT('Ctrl Pts',(-2.17970416578576,1.25969477045726,1.02681093050002));
#37938=CARTESIAN_POINT('Ctrl Pts',(-2.16713323835683,1.28121696579934,1.02524786792946));
#37939=CARTESIAN_POINT('Ctrl Pts',(-2.16032946261532,1.29265618398572,1.02441650086985));
#37940=CARTESIAN_POINT('Ctrl Pts',(-2.14144275436363,1.32384485015468,1.02214779819336));
#37941=CARTESIAN_POINT('Ctrl Pts',(-2.12917741681121,1.34348272789404,1.02071709777966));
#37942=CARTESIAN_POINT('Ctrl Pts',(-2.05517542143316,1.45840688211109,1.01232588492245));
#37943=CARTESIAN_POINT('Ctrl Pts',(-1.98731729199051,1.5496035716431,1.00559927193119));
#37944=CARTESIAN_POINT('Ctrl Pts',(-1.84647924280528,1.71434140723486,0.992990036373422));
#37945=CARTESIAN_POINT('Ctrl Pts',(-1.77467308201424,1.78857147535461,0.987096789431059));
#37946=CARTESIAN_POINT('Ctrl Pts',(-1.65419597377087,1.89869618159393,0.977693553605859));
#37947=CARTESIAN_POINT('Ctrl Pts',(-1.60844356219811,1.93760685230893,0.974219198148781));
#37948=CARTESIAN_POINT('Ctrl Pts',(-1.50268902896809,2.02121824115617,0.966295336365825));
#37949=CARTESIAN_POINT('Ctrl Pts',(-1.44200096120561,2.06495242296029,0.961819855323459));
#37950=CARTESIAN_POINT('Ctrl Pts',(-1.36857846245463,2.11304722288093,0.956373645305415));
#37951=CARTESIAN_POINT('Ctrl Pts',(-1.35763854417802,2.12009271986527,0.955561358746048));
#37952=CARTESIAN_POINT('Ctrl Pts',(-1.33971318339815,2.1314413295364,0.954228254723307));
#37953=CARTESIAN_POINT('Ctrl Pts',(-1.33276030356428,2.13579575891417,0.953710649395945));
#37954=CARTESIAN_POINT('Ctrl Pts',(-1.32023670507718,2.14355403738605,0.952777165954427));
#37955=CARTESIAN_POINT('Ctrl Pts',(-1.31467388413465,2.14697029434183,0.952362100371873));
#37956=CARTESIAN_POINT('Ctrl Pts',(-1.30237757332989,2.15445603456975,0.951443662991297));
#37957=CARTESIAN_POINT('Ctrl Pts',(-1.29563833649191,2.15851556525145,0.950939687533825));
#37958=CARTESIAN_POINT('Ctrl Pts',(-1.27604270308395,2.17019460299725,0.949472774181139));
#37959=CARTESIAN_POINT('Ctrl Pts',(-1.26313760098367,2.17773115202909,0.948504838792789));
#37960=CARTESIAN_POINT('Ctrl Pts',(-1.15265456121644,2.24094057200843,0.940207266830241));
#37961=CARTESIAN_POINT('Ctrl Pts',(-1.05152801730223,2.290133260865,0.932545733957284));
#37962=CARTESIAN_POINT('Ctrl Pts',(-0.780969670107453,2.40003935503442,
0.912437887868524));
#37963=CARTESIAN_POINT('Ctrl Pts',(-0.607682965337253,2.4496611024057,0.899971032799213));
#37964=CARTESIAN_POINT('Ctrl Pts',(-0.368361763167782,2.4912051683072,0.883847074843666));
#37965=CARTESIAN_POINT('Ctrl Pts',(-0.305758577773296,2.49966126030663,
0.879721041319345));
#37966=CARTESIAN_POINT('Ctrl Pts',(-0.222793506888974,2.5077035962604,0.874370822732703));
#37967=CARTESIAN_POINT('Ctrl Pts',(-0.202664970584672,2.50941053274065,
0.873081794874619));
#37968=CARTESIAN_POINT('Ctrl Pts',(-0.169865486393625,2.51179475432956,
0.870995499692251));
#37969=CARTESIAN_POINT('Ctrl Pts',(-0.157206437510141,2.5126188164712,0.870193717441192));
#37970=CARTESIAN_POINT('Ctrl Pts',(-0.132780564651753,2.51402353787054,
0.868653089468399));
#37971=CARTESIAN_POINT('Ctrl Pts',(-0.121014859847978,2.51461735430326,
0.867913855711089));
#37972=CARTESIAN_POINT('Ctrl Pts',(-0.0936402624622615,2.51580637700057,
0.866200390827621));
#37973=CARTESIAN_POINT('Ctrl Pts',(-0.078029028714933,2.51633895038967,
0.865228121713024));
#37974=CARTESIAN_POINT('Ctrl Pts',(-0.0276854629661903,2.51758744598396,
0.862107690332712));
#37975=CARTESIAN_POINT('Ctrl Pts',(0.00705795139312717,2.51772981026285,
0.859977222248272));
#37976=CARTESIAN_POINT('Ctrl Pts',(0.0891350918806768,2.5163670107066,0.854990676225652));
#37977=CARTESIAN_POINT('Ctrl Pts',(0.136445916993481,2.51424559199206,0.852152956507963));
#37978=CARTESIAN_POINT('Ctrl Pts',(0.415894458664718,2.49380320122993,0.835541552342684));
#37979=CARTESIAN_POINT('Ctrl Pts',(0.644609876897895,2.44468485578048,0.822674399909907));
#37980=CARTESIAN_POINT('Ctrl Pts',(0.915564057244588,2.34577152690151,0.805516637889768));
#37981=CARTESIAN_POINT('Ctrl Pts',(0.967175439674964,2.3249671528889,0.802150154356566));
#37982=CARTESIAN_POINT('Ctrl Pts',(1.03007820508638,2.29715434293162,0.797874728427992));
#37983=CARTESIAN_POINT('Ctrl Pts',(1.04206326138337,2.29174242133527,0.797052206144096));
#37984=CARTESIAN_POINT('Ctrl Pts',(1.06085439440756,2.28307929958075,0.795749254049853));
#37985=CARTESIAN_POINT('Ctrl Pts',(1.06768939223993,2.2798908948638,0.795272526338978));
#37986=CARTESIAN_POINT('Ctrl Pts',(1.0803382042062,2.27392109603348,0.794384909369086));
#37987=CARTESIAN_POINT('Ctrl Pts',(1.0861557561688,2.27114804826618,0.793974528119976));
#37988=CARTESIAN_POINT('Ctrl Pts',(1.09944351722231,2.26475145105282,0.793032277277408));
#37989=CARTESIAN_POINT('Ctrl Pts',(1.10690642264452,2.26111329866756,0.792499529111765));
#37990=CARTESIAN_POINT('Ctrl Pts',(1.1301119031017,2.24965825636622,0.790832221380776));
#37991=CARTESIAN_POINT('Ctrl Pts',(1.14579031064432,2.2417135648613,0.789690227407963));
#37992=CARTESIAN_POINT('Ctrl Pts',(1.18262143696868,2.22256288323565,0.786972932151512));
#37993=CARTESIAN_POINT('Ctrl Pts',(1.20369977129088,2.21121821730328,0.785390543523805));
#37994=CARTESIAN_POINT('Ctrl Pts',(1.27895341386057,2.16932079241609,0.779650522444104));
#37995=CARTESIAN_POINT('Ctrl Pts',(1.33215134737835,2.13706488542584,0.775421939469041));
#37996=CARTESIAN_POINT('Ctrl Pts',(1.54739685076904,1.99539187579499,0.757741237801217));
#37997=CARTESIAN_POINT('Ctrl Pts',(1.69764724291739,1.86923442008128,0.744071612891362));
#37998=CARTESIAN_POINT('Ctrl Pts',(1.88022188371325,1.67557675566218,0.726320675551551));
#37999=CARTESIAN_POINT('Ctrl Pts',(1.92647841543517,1.62218196228031,0.721692405615313));
#38000=CARTESIAN_POINT('Ctrl Pts',(1.98344694453827,1.55054238344843,0.715812239542089));
#38001=CARTESIAN_POINT('Ctrl Pts',(1.99625717361339,1.5340146038628,0.71447706447666));
#38002=CARTESIAN_POINT('Ctrl Pts',(2.01654999056128,1.50714802297689,0.712340315980959));
#38003=CARTESIAN_POINT('Ctrl Pts',(2.02416226702043,1.49690886635203,0.711533676958355));
#38004=CARTESIAN_POINT('Ctrl Pts',(2.03854723543726,1.47724947481052,0.709999345304622));
#38005=CARTESIAN_POINT('Ctrl Pts',(2.04533326912431,1.46783945560564,0.709271147858374));
#38006=CARTESIAN_POINT('Ctrl Pts',(2.06075770921005,1.44613610924909,0.707605620887821));
#38007=CARTESIAN_POINT('Ctrl Pts',(2.06935165275714,1.43381161080969,0.706670008377926));
#38008=CARTESIAN_POINT('Ctrl Pts',(2.09588090904142,1.39503083157344,0.703756918313447));
#38009=CARTESIAN_POINT('Ctrl Pts',(2.1134234986342,1.36830883320872,0.701794195195356));
#38010=CARTESIAN_POINT('Ctrl Pts',(2.19955504256816,1.2314976679287,0.691954816867849));
#38011=CARTESIAN_POINT('Ctrl Pts',(2.26007538360321,1.11655441533893,0.684374831861546));
#38012=CARTESIAN_POINT('Ctrl Pts',(2.32923370738789,0.956287682709663,0.674308477894333));
#38013=CARTESIAN_POINT('Ctrl Pts',(2.34588901247795,0.914668837099738,0.671735936903445));
#38014=CARTESIAN_POINT('Ctrl Pts',(2.36142199806814,0.872635317323264,0.66916271832655));
#38015=CARTESIAN_POINT('Origin',(0.,0.,-2.20842344717744));
#38016=CARTESIAN_POINT('',(3.07504124793238,-0.00259082838863623,1.29157655282254));
#38017=CARTESIAN_POINT('Ctrl Pts',(-1.87460960294492,2.44013607231272,0.645925936011554));
#38018=CARTESIAN_POINT('Ctrl Pts',(-2.59108721142439,1.88105535536774,0.693142492280968));
#38019=CARTESIAN_POINT('Ctrl Pts',(-3.57302986143905,-0.0172401031001995,
0.793148684478441));
#38020=CARTESIAN_POINT('Ctrl Pts',(-2.05206621173493,-2.99393512365163,
0.945944512603972));
#38021=CARTESIAN_POINT('Ctrl Pts',(1.39399303947859,-3.35125838105565,1.10431342038815));
#38022=CARTESIAN_POINT('Ctrl Pts',(2.97699768626307,-1.39003409856734,1.219524100461));
#38023=CARTESIAN_POINT('Ctrl Pts',(3.076708517471,-0.188292403425034,1.2819451446058));
#38024=CARTESIAN_POINT('Ctrl Pts',(3.07504124793238,-0.00259082838863623,
1.29157655282254));
#38025=CARTESIAN_POINT('Ctrl Pts',(3.07504124793238,-0.00259082838863623,
1.29157655282254));
#38026=CARTESIAN_POINT('Ctrl Pts',(3.06757023260577,0.829535760103501,1.33473478053386));
#38027=CARTESIAN_POINT('Ctrl Pts',(2.28975044149764,2.69180612852788,1.43068264417324));
#38028=CARTESIAN_POINT('Ctrl Pts',(-0.207342744971815,3.35541631029136,
1.54879005713849));
#38029=CARTESIAN_POINT('Ctrl Pts',(-1.53027139183725,2.69679833931267,1.62373924239242));
#38030=CARTESIAN_POINT('Ctrl Pts',(-1.86967516139566,2.43378849843609,1.64589879171829));
#38031=CARTESIAN_POINT('',(3.07349937966369,0.00195274342530456,1.20842344721377));
#38032=CARTESIAN_POINT('Ctrl Pts',(3.07349937966369,0.00195274342531009,
1.20842344721377));
#38033=CARTESIAN_POINT('Ctrl Pts',(3.07343009793609,0.110997968751781,1.21404815002136));
#38034=CARTESIAN_POINT('Ctrl Pts',(3.06755350611745,0.219823458127608,1.21967285282894));
#38035=CARTESIAN_POINT('Ctrl Pts',(3.05596382899217,0.327852597811126,1.22529755563653));
#38036=CARTESIAN_POINT('Ctrl Pts',(3.0443228227567,0.436360183922003,1.230947169491));
#38037=CARTESIAN_POINT('Ctrl Pts',(3.02691813728145,0.544064148491547,1.23659678334547));
#38038=CARTESIAN_POINT('Ctrl Pts',(3.0038949192498,0.650398004382886,1.24224639719993));
#38039=CARTESIAN_POINT('Ctrl Pts',(2.98074448250616,0.757319426103119,1.24792722895786));
#38040=CARTESIAN_POINT('Ctrl Pts',(2.95191336117846,0.862855358188295,1.25360806071578));
#38041=CARTESIAN_POINT('Ctrl Pts',(2.91759746433215,0.96645087103411,1.2592888924737));
#38042=CARTESIAN_POINT('Ctrl Pts',(2.90216890839473,1.01302780218549,1.26184301574027));
#38043=CARTESIAN_POINT('Ctrl Pts',(2.88563227776604,1.05921278948065,1.26439713900684));
#38044=CARTESIAN_POINT('Ctrl Pts',(2.86800844378224,1.10495692965552,1.2669512622734));
#38045=CARTESIAN_POINT('Ctrl Pts',(2.83350913215343,1.19450278832257,1.27195105372586));
#38046=CARTESIAN_POINT('Ctrl Pts',(2.79475151626034,1.28258851739022,1.27695084517831));
#38047=CARTESIAN_POINT('Ctrl Pts',(2.75187964773997,1.36878071814098,1.28195063663076));
#38048=CARTESIAN_POINT('Ctrl Pts',(2.70906591298316,1.45485604325297,1.28694364842317));
#38049=CARTESIAN_POINT('Ctrl Pts',(2.66214920708533,1.53904255338566,1.29193666021558));
#38050=CARTESIAN_POINT('Ctrl Pts',(2.61132227195232,1.62092511918526,1.29692967200798));
#38051=CARTESIAN_POINT('Ctrl Pts',(2.56054893723817,1.70272133431641,1.30191741833391));
#38052=CARTESIAN_POINT('Ctrl Pts',(2.50587380102546,1.78221806423109,1.30690516465983));
#38053=CARTESIAN_POINT('Ctrl Pts',(2.44753583352583,1.8590240971023,1.31189291098575));
#38054=CARTESIAN_POINT('Ctrl Pts',(2.38923958960003,1.93577519795718,1.31687709005332));
#38055=CARTESIAN_POINT('Ctrl Pts',(2.32728598690376,2.009839078879,1.32186126912088));
#38056=CARTESIAN_POINT('Ctrl Pts',(2.26195713196696,2.08085371497946,1.32684544818845));
#38057=CARTESIAN_POINT('Ctrl Pts',(2.1966520569979,2.15184250146479,1.33182781299465));
#38058=CARTESIAN_POINT('Ctrl Pts',(2.12797446775194,2.21978392577767,1.33681017780085));
#38059=CARTESIAN_POINT('Ctrl Pts',(2.05624592462546,2.28435000546352,1.34179254260705));
#38060=CARTESIAN_POINT('Ctrl Pts',(1.98452391546502,2.34891020363341,1.34677445355484));
#38061=CARTESIAN_POINT('Ctrl Pts',(1.90975183131845,2.41009537498492,1.35175636450264));
#38062=CARTESIAN_POINT('Ctrl Pts',(1.83228637233234,2.4676160357246,1.35673827545043));
#38063=CARTESIAN_POINT('Ctrl Pts',(1.75480682901544,2.52514715454488,1.36172109218104));
#38064=CARTESIAN_POINT('Ctrl Pts',(1.67463329072286,2.57901217792974,1.36670390891165));
#38065=CARTESIAN_POINT('Ctrl Pts',(1.59215277132944,2.62896401701278,1.37168672564226));
#38066=CARTESIAN_POINT('Ctrl Pts',(1.50958338360504,2.67896967652034,1.37667491109036));
#38067=CARTESIAN_POINT('Ctrl Pts',(1.42470242845596,2.72505350663459,1.38166309653845));
#38068=CARTESIAN_POINT('Ctrl Pts',(1.33792274537938,2.76701372916661,1.38665128198655));
#38069=CARTESIAN_POINT('Ctrl Pts',(1.25109181275541,2.80899873218107,1.39164241331134));
#38070=CARTESIAN_POINT('Ctrl Pts',(1.16236032294793,2.84685510639286,1.39663354463613));
#38071=CARTESIAN_POINT('Ctrl Pts',(1.07216040699722,2.88042953596639,1.40162467596093));
#38072=CARTESIAN_POINT('Ctrl Pts',(0.981814800859125,2.91405819469174,1.40662386892137));
#38073=CARTESIAN_POINT('Ctrl Pts',(0.889996450440418,2.94339096524173,1.41162306188182));
#38074=CARTESIAN_POINT('Ctrl Pts',(0.797151859972865,2.96832463894059,1.41662225484226));
#38075=CARTESIAN_POINT('Ctrl Pts',(0.743306210453191,2.98278503828606,1.41952155991403));
#38076=CARTESIAN_POINT('Ctrl Pts',(0.689115582699021,2.99576676899764,1.42242086498581));
#38077=CARTESIAN_POINT('Ctrl Pts',(0.634668086571051,3.00725766602868,1.42532017005758));
#38078=CARTESIAN_POINT('Ctrl Pts',(0.54076914544621,3.02707461153619,1.43032024711525));
#38079=CARTESIAN_POINT('Ctrl Pts',(0.445776314329343,3.04252426601338,1.43532032417293));
#38080=CARTESIAN_POINT('Ctrl Pts',(0.350131646875332,3.05349145730856,1.44032040123061));
#38081=CARTESIAN_POINT('Ctrl Pts',(0.252673050139253,3.06466664461609,1.44541530622202));
#38082=CARTESIAN_POINT('Ctrl Pts',(0.154538065542236,3.07118742824564,1.45051021121343));
#38083=CARTESIAN_POINT('Ctrl Pts',(0.0562082719914919,3.07298598762828,
1.45560511620484));
#38084=CARTESIAN_POINT('Ctrl Pts',(-0.0400396967687125,3.0747464681604,
1.46059215257238));
#38085=CARTESIAN_POINT('Ctrl Pts',(-0.136473842897125,3.07198268032219,
1.46557918893991));
#38086=CARTESIAN_POINT('Ctrl Pts',(-0.232636021868556,3.06468313718224,
1.47056622530744));
#38087=CARTESIAN_POINT('Ctrl Pts',(-0.328734310230141,3.05738844389353,
1.47554994826425));
#38088=CARTESIAN_POINT('Ctrl Pts',(-0.42456055420376,3.04556401678089,1.48053367122106));
#38089=CARTESIAN_POINT('Ctrl Pts',(-0.519657669423997,3.02925042817672,
1.48551739417788));
#38090=CARTESIAN_POINT('Ctrl Pts',(-0.614717560680323,3.0129432252177,1.49049916635076));
#38091=CARTESIAN_POINT('Ctrl Pts',(-0.709048458548368,2.99215042840172,
1.49548093852365));
#38092=CARTESIAN_POINT('Ctrl Pts',(-0.802200520997021,2.96696420169036,
1.50046271069654));
#38093=CARTESIAN_POINT('Ctrl Pts',(-0.899020846212493,2.94078615906797,
1.5056406615572));
#38094=CARTESIAN_POINT('Ctrl Pts',(-0.994567082253931,2.9098616152258,1.51081861241787));
#38095=CARTESIAN_POINT('Ctrl Pts',(-1.08834928517019,2.87435176752421,1.51599656327853));
#38096=CARTESIAN_POINT('Ctrl Pts',(-1.17861656379949,2.84017281654109,1.52098044634519));
#38097=CARTESIAN_POINT('Ctrl Pts',(-1.26724926143468,2.80174633023389,1.52596432941184));
#38098=CARTESIAN_POINT('Ctrl Pts',(-1.35383047369533,2.75926535485333,1.5309482124785));
#38099=CARTESIAN_POINT('Ctrl Pts',(-1.44044177501539,2.71676961630928,1.53593382756473));
#38100=CARTESIAN_POINT('Ctrl Pts',(-1.52499978465994,2.67021679040478,1.54091944265095));
#38101=CARTESIAN_POINT('Ctrl Pts',(-1.60711276316665,2.61984557111042,1.54590505773717));
#38102=CARTESIAN_POINT('Ctrl Pts',(-1.68930742471596,2.56942424433577,1.55089563233427));
#38103=CARTESIAN_POINT('Ctrl Pts',(-1.76905183814869,2.5151771894122,1.55588620693136));
#38104=CARTESIAN_POINT('Ctrl Pts',(-1.84598423370511,2.45738569600137,1.56087678152846));
#38105=CARTESIAN_POINT('Ctrl Pts',(-1.85482935887853,2.45074125201285,1.56145056136047));
#38106=CARTESIAN_POINT('Ctrl Pts',(-1.86363734989752,2.44404999788814,1.56202434119248));
#38107=CARTESIAN_POINT('Ctrl Pts',(-1.87240768645123,2.4373123939533,1.56259812102449));
#38108=CARTESIAN_POINT('Ctrl Pts',(-1.87240768645124,2.43731239395329,0.562647869306095));
#38109=CARTESIAN_POINT('Ctrl Pts',(-1.94905896554419,2.37842685900668,0.567639530215172));
#38110=CARTESIAN_POINT('Ctrl Pts',(-2.02291441462503,2.31593375215335,0.57263119112425));
#38111=CARTESIAN_POINT('Ctrl Pts',(-2.09362883246835,2.25013789840917,0.577622852033327));
#38112=CARTESIAN_POINT('Ctrl Pts',(-2.16441886594012,2.18427168850591,0.582619850574929));
#38113=CARTESIAN_POINT('Ctrl Pts',(-2.23206084063887,2.11509597791773,0.587616849116532));
#38114=CARTESIAN_POINT('Ctrl Pts',(-2.29624594476156,2.04295296352268,0.592613847658134));
#38115=CARTESIAN_POINT('Ctrl Pts',(-2.36046719375466,1.97076932288044,0.597613660183871));
#38116=CARTESIAN_POINT('Ctrl Pts',(-2.42122742015232,1.89561539037743,0.602613472709608));
#38117=CARTESIAN_POINT('Ctrl Pts',(-2.47825904536878,1.81786532890855,0.607613285235344));
#38118=CARTESIAN_POINT('Ctrl Pts',(-2.5353854370201,1.73998607427524,0.612621405685083));
#38119=CARTESIAN_POINT('Ctrl Pts',(-2.58877061037479,1.6595024385294,0.617629526134822));
#38120=CARTESIAN_POINT('Ctrl Pts',(-2.63819110377384,1.57681639703821,0.622637646584561));
#38121=CARTESIAN_POINT('Ctrl Pts',(-2.67384110789506,1.51716993223815,0.626250308101941));
#38122=CARTESIAN_POINT('Ctrl Pts',(-2.70742899249457,1.45637798245718,0.629862969619322));
#38123=CARTESIAN_POINT('Ctrl Pts',(-2.73888636901132,1.39459804518865,0.633475631136703));
#38124=CARTESIAN_POINT('Ctrl Pts',(-2.78236147074177,1.30921619345601,0.638468445044824));
#38125=CARTESIAN_POINT('Ctrl Pts',(-2.82191856036241,1.22164556821355,0.643461258952946));
#38126=CARTESIAN_POINT('Ctrl Pts',(-2.85733111600709,1.13228138883303,0.648454072861068));
#38127=CARTESIAN_POINT('Ctrl Pts',(-2.89269493641044,1.04304019365317,0.653440015590695));
#38128=CARTESIAN_POINT('Ctrl Pts',(-2.92392539698329,0.952010755250424,
0.658425958320322));
#38129=CARTESIAN_POINT('Ctrl Pts',(-2.95084203474825,0.859612433578535,
0.66341190104995));
#38130=CARTESIAN_POINT('Ctrl Pts',(-2.97772980731311,0.767313199172595,
0.668392496892055));
#38131=CARTESIAN_POINT('Ctrl Pts',(-3.00031283028168,0.673648419926478,
0.673373092734159));
#38132=CARTESIAN_POINT('Ctrl Pts',(-3.018459279418,0.579055980450372,0.678353688576264));
#38133=CARTESIAN_POINT('Ctrl Pts',(-3.03659239523886,0.484533043874101,
0.683330624867396));
#38134=CARTESIAN_POINT('Ctrl Pts',(-3.0502953346203,0.389084233159763,0.688307561158528));
#38135=CARTESIAN_POINT('Ctrl Pts',(-3.05948678636867,0.29316011672043,0.693284497449659));
#38136=CARTESIAN_POINT('Ctrl Pts',(-3.0686747867071,0.197272019993435,0.698259564890494));
#38137=CARTESIAN_POINT('Ctrl Pts',(-3.07335462310795,0.100909409968239,
0.703234632331328));
#38138=CARTESIAN_POINT('Ctrl Pts',(-3.07349666230747,0.00452954576419626,
0.708209699772163));
#38139=CARTESIAN_POINT('Ctrl Pts',(-3.07363868723893,-0.0918406369259107,
0.71318426745939));
#38140=CARTESIAN_POINT('Ctrl Pts',(-3.06924382066654,-0.188227630029704,
0.718158835146618));
#38141=CARTESIAN_POINT('Ctrl Pts',(-3.06033455102816,-0.2841736894634,0.723133402833845));
#38142=CARTESIAN_POINT('Ctrl Pts',(-3.05142372585751,-0.380136500796889,
0.72810883906596));
#38143=CARTESIAN_POINT('Ctrl Pts',(-3.03799697319906,-0.475657787148692,
0.733084275298076));
#38144=CARTESIAN_POINT('Ctrl Pts',(-3.02012858349012,-0.570285533032338,
0.738059711530191));
#38145=CARTESIAN_POINT('Ctrl Pts',(-3.00224095756202,-0.665015150438181,
0.743040504069357));
#38146=CARTESIAN_POINT('Ctrl Pts',(-2.97990223035542,-0.758848873551352,
0.748021296608524));
#38147=CARTESIAN_POINT('Ctrl Pts',(-2.9532376668212,-0.851345719005196,
0.753002089147691));
#38148=CARTESIAN_POINT('Ctrl Pts',(-2.92655742970267,-0.943896934638524,
0.757985809425452));
#38149=CARTESIAN_POINT('Ctrl Pts',(-2.89554643530498,-1.03510929134487,
0.762969529703214));
#38150=CARTESIAN_POINT('Ctrl Pts',(-2.86037889876275,-1.12455982744931,
0.767953249980975));
#38151=CARTESIAN_POINT('Ctrl Pts',(-2.82515416180484,-1.21415585591263,
0.772945076338932));
#38152=CARTESIAN_POINT('Ctrl Pts',(-2.78575956342682,-1.30198394035763,
0.777936902696889));
#38153=CARTESIAN_POINT('Ctrl Pts',(-2.74241620542279,-1.38764390469402,
0.782928729054846));
#38154=CARTESIAN_POINT('Ctrl Pts',(-2.71661127878151,-1.43864247050864,
0.785900665676857));
#38155=CARTESIAN_POINT('Ctrl Pts',(-2.68940756252767,-1.48887304044717,
0.788872602298868));
#38156=CARTESIAN_POINT('Ctrl Pts',(-2.66085892417018,-1.53825616711389,
0.791844538920878));
#38157=CARTESIAN_POINT('Ctrl Pts',(-2.61281902951214,-1.62135505867035,
0.79684553127869));
#38158=CARTESIAN_POINT('Ctrl Pts',(-2.56079859453099,-1.70234671456233,
0.8018465236365));
#38159=CARTESIAN_POINT('Ctrl Pts',(-2.50500764161483,-1.78082536073903,
0.806847515994311));
#38160=CARTESIAN_POINT('Ctrl Pts',(-2.44929226877616,-1.85919769179027,
0.81184173350118));
#38161=CARTESIAN_POINT('Ctrl Pts',(-2.38981678184086,-1.93506342472989,
0.81683595100805));
#38162=CARTESIAN_POINT('Ctrl Pts',(-2.32683644438054,-2.00804243259511,
0.821830168514919));
#38163=CARTESIAN_POINT('Ctrl Pts',(-2.26392246891729,-2.08094454292532,
0.826819123645293));
#38164=CARTESIAN_POINT('Ctrl Pts',(-2.19751126966771,-2.15096564470491,
0.831808078775667));
#38165=CARTESIAN_POINT('Ctrl Pts',(-2.12790003961761,-2.21775644997267,
0.836797033906041));
#38166=CARTESIAN_POINT('Ctrl Pts',(-2.05833859131106,-2.28449949049418,
0.841782421237301));
#38167=CARTESIAN_POINT('Ctrl Pts',(-1.9855819772832,-2.34801652415295,0.84676780856856));
#38168=CARTESIAN_POINT('Ctrl Pts',(-1.9099654452319,-2.40799382225539,0.851753195899819));
#38169=CARTESIAN_POINT('Ctrl Pts',(-1.83437644348645,-2.46794928395095,
0.856736768161883));
#38170=CARTESIAN_POINT('Ctrl Pts',(-1.75592993590305,-2.52436729840681,
0.861720340423947));
#38171=CARTESIAN_POINT('Ctrl Pts',(-1.6749948327486,-2.57697391532501,0.866703912686011));
#38172=CARTESIAN_POINT('Ctrl Pts',(-1.59406713818946,-2.6295757167661,0.871687028764434));
#38173=CARTESIAN_POINT('Ctrl Pts',(-1.51065166887184,-2.67836657542674,
0.876670144842856));
#38174=CARTESIAN_POINT('Ctrl Pts',(-1.42514604412366,-2.72311604653909,
0.881653260921278));
#38175=CARTESIAN_POINT('Ctrl Pts',(-1.33962494296209,-2.76787361725092,
0.886637278937609));
#38176=CARTESIAN_POINT('Ctrl Pts',(-1.25201332369129,-2.80858814429552,
0.891621296953941));
#38177=CARTESIAN_POINT('Ctrl Pts',(-1.16273214328596,-2.84507578334385,
0.896605314970273));
#38178=CARTESIAN_POINT('Ctrl Pts',(-1.07335502862711,-2.88160262902452,
0.901594688404685));
#38179=CARTESIAN_POINT('Ctrl Pts',(-0.982305178048635,-2.91389335302891,
0.906584061839098));
#38180=CARTESIAN_POINT('Ctrl Pts',(-0.890021999705784,-2.94181289174545,
0.911573435273511));
#38181=CARTESIAN_POINT('Ctrl Pts',(-0.797684441172705,-2.96974888275431,
0.916565748822053));
#38182=CARTESIAN_POINT('Ctrl Pts',(-0.704112532915942,-2.99330845238699,
0.921558062370594));
#38183=CARTESIAN_POINT('Ctrl Pts',(-0.609757194458012,-3.01240741165711,
0.926550375919135));
#38184=CARTESIAN_POINT('Ctrl Pts',(-0.515249884375504,-3.03153713230137,
0.931550730242187));
#38185=CARTESIAN_POINT('Ctrl Pts',(-0.419957057788829,-3.04619183021403,
0.936551084565239));
#38186=CARTESIAN_POINT('Ctrl Pts',(-0.324336030925877,-3.05633905007989,
0.94155143888829));
#38187=CARTESIAN_POINT('Ctrl Pts',(-0.269121938175487,-3.06219832138468,
0.94443877482721));
#38188=CARTESIAN_POINT('Ctrl Pts',(-0.213798459573521,-3.0665556748148,
0.94732611076613));
#38189=CARTESIAN_POINT('Ctrl Pts',(-0.158453405166694,-3.06941277256596,
0.950213446705049));
#38190=CARTESIAN_POINT('Ctrl Pts',(-0.0626027152455783,-3.07436090738228,
0.955213950268477));
#38191=CARTESIAN_POINT('Ctrl Pts',(0.0336475200514081,-3.07482359536837,
0.960214453831906));
#38192=CARTESIAN_POINT('Ctrl Pts',(0.129842654367104,-3.07075611781641,
0.965214957395334));
#38193=CARTESIAN_POINT('Ctrl Pts',(0.225907730009681,-3.06669413961468,
0.970208700129714));
#38194=CARTESIAN_POINT('Ctrl Pts',(0.321917418088531,-3.05811418728265,
0.975202442864094));
#38195=CARTESIAN_POINT('Ctrl Pts',(0.417413958539367,-3.04502345429662,
0.980196185598474));
#38196=CARTESIAN_POINT('Ctrl Pts',(0.512810145125333,-3.03194647788902,
0.985184680588997));
#38197=CARTESIAN_POINT('Ctrl Pts',(0.607693823691037,-3.01436820348801,
0.990173175579519));
#38198=CARTESIAN_POINT('Ctrl Pts',(0.701610279724667,-2.99234778483128,
0.995161670570041));
#38199=CARTESIAN_POINT('Ctrl Pts',(0.795460017432848,-2.97034300949758,
1.00014662172973));
#38200=CARTESIAN_POINT('Ctrl Pts',(0.888343472603172,-2.94390246317094,
1.00513157288943));
#38201=CARTESIAN_POINT('Ctrl Pts',(0.979815043976995,-2.91313657928981,
1.01011652404912));
#38202=CARTESIAN_POINT('Ctrl Pts',(1.07125358537939,-2.88238180483045,1.01509967516546));
#38203=CARTESIAN_POINT('Ctrl Pts',(1.16128084051803,-2.8473049358334,1.02008282628179));
#38204=CARTESIAN_POINT('Ctrl Pts',(1.24946625528609,-2.80806629674254,1.02506597739813));
#38205=CARTESIAN_POINT('Ctrl Pts',(1.33764387342051,-2.76883112681145,1.03004868794497));
#38206=CARTESIAN_POINT('Ctrl Pts',(1.42397957415623,-2.72543509689045,1.03503139849181));
#38207=CARTESIAN_POINT('Ctrl Pts',(1.50806367453896,-2.67808629501293,1.04001410903866));
#38208=CARTESIAN_POINT('Ctrl Pts',(1.59216326892317,-2.63072876827062,1.04499773773916));
#38209=CARTESIAN_POINT('Ctrl Pts',(1.67401005665726,-2.57941723830154,1.04998136643966));
#38210=CARTESIAN_POINT('Ctrl Pts',(1.75322074687176,-2.52440473433609,1.05496499514017));
#38211=CARTESIAN_POINT('Ctrl Pts',(1.83251699190992,-2.46933281181154,1.05995400661758));
#38212=CARTESIAN_POINT('Ctrl Pts',(1.90917109423952,-2.41055218556782,1.064943018095));
#38213=CARTESIAN_POINT('Ctrl Pts',(1.98283064243665,-2.34835791424865,1.06993202957242));
#38214=CARTESIAN_POINT('Ctrl Pts',(2.0565338198878,-2.28612680466847,1.074923996089));
#38215=CARTESIAN_POINT('Ctrl Pts',(2.12723859006732,-2.22047832237597,1.07991596260557));
#38216=CARTESIAN_POINT('Ctrl Pts',(2.19462895830496,-2.15174486995305,1.08490792912214));
#38217=CARTESIAN_POINT('Ctrl Pts',(2.26212824199178,-2.08290033140552,1.089907963591));
#38218=CARTESIAN_POINT('Ctrl Pts',(2.32630213572037,-2.01096119419358,1.09490799805986));
#38219=CARTESIAN_POINT('Ctrl Pts',(2.38687456445779,-1.93629338261133,1.09990803252872));
#38220=CARTESIAN_POINT('Ctrl Pts',(2.42190263956881,-1.89311417109553,1.10279947318222));
#38221=CARTESIAN_POINT('Ctrl Pts',(2.45572713142748,-1.84902302175565,1.10569091383573));
#38222=CARTESIAN_POINT('Ctrl Pts',(2.48830145039687,-1.80409482620865,1.10858235448924));
#38223=CARTESIAN_POINT('Ctrl Pts',(2.54499894872664,-1.72589468657169,1.11361507525852));
#38224=CARTESIAN_POINT('Ctrl Pts',(2.59810577807862,-1.64488241326908,1.11864779602781));
#38225=CARTESIAN_POINT('Ctrl Pts',(2.6473333336295,-1.56141873648747,1.1236805167971));
#38226=CARTESIAN_POINT('Ctrl Pts',(2.69649239275006,-1.47807119311645,1.12870623491506));
#38227=CARTESIAN_POINT('Ctrl Pts',(2.74178268845003,-1.39227939287324,1.13373195303301));
#38228=CARTESIAN_POINT('Ctrl Pts',(2.78295729814532,-1.30443509869204,1.13875767115097));
#38229=CARTESIAN_POINT('Ctrl Pts',(2.82408534728155,-1.21669013950095,1.14377770614899));
#38230=CARTESIAN_POINT('Ctrl Pts',(2.8611067804729,-1.12689768830382,1.14879774114701));
#38231=CARTESIAN_POINT('Ctrl Pts',(2.89381975642089,-1.03547547887341,1.15381777614503));
#38232=CARTESIAN_POINT('Ctrl Pts',(2.92650203182348,-0.944139067558604,
1.15883309992959));
#38233=CARTESIAN_POINT('Ctrl Pts',(2.95488374949979,-0.851176345363529,
1.16384842371416));
#38234=CARTESIAN_POINT('Ctrl Pts',(2.97881094644113,-0.757025491884187,
1.16886374749872));
#38235=CARTESIAN_POINT('Ctrl Pts',(3.00272483622375,-0.662927000591433,
1.17387628200088));
#38236=CARTESIAN_POINT('Ctrl Pts',(3.02218902592584,-0.567642109118777,
1.17888881650303));
#38237=CARTESIAN_POINT('Ctrl Pts',(3.03709946663982,-0.471623875282121,
1.18390135100518));
#38238=CARTESIAN_POINT('Ctrl Pts',(3.05200762896964,-0.375620313474767,
1.18891311956892));
#38239=CARTESIAN_POINT('Ctrl Pts',(3.06236335379107,-0.278884057045305,
1.19392488813267));
#38240=CARTESIAN_POINT('Ctrl Pts',(3.06811389854472,-0.181877309075922,
1.19893665669641));
#38241=CARTESIAN_POINT('Ctrl Pts',(3.0717423058648,-0.120669195843547,1.20209892019009));
#38242=CARTESIAN_POINT('Ctrl Pts',(3.0735383305219,-0.0593535603866601,
1.20526118368377));
#38243=CARTESIAN_POINT('Ctrl Pts',(3.07349937966414,0.00195274272110892,
1.20842344717745));
#38244=CARTESIAN_POINT('Origin',(3.42660592399111E-16,1.36827403442078E-16,
19.));
#38245=CARTESIAN_POINT('Ctrl Pts',(1.91346599666504,1.63598720337497,19.));
#38246=CARTESIAN_POINT('Ctrl Pts',(1.97549316674761,1.57769689441576,19.));
#38247=CARTESIAN_POINT('Ctrl Pts',(2.0341596855751,1.51616828548999,19.));
#38248=CARTESIAN_POINT('Ctrl Pts',(2.08945330857753,1.45177509691646,19.));
#38249=CARTESIAN_POINT('Ctrl Pts',(2.14629304460953,1.38558135445508,19.));
#38250=CARTESIAN_POINT('Ctrl Pts',(2.19956910898861,1.31636012908618,19.));
#38251=CARTESIAN_POINT('Ctrl Pts',(2.24923921204997,1.24447092433007,19.));
#38252=CARTESIAN_POINT('Ctrl Pts',(2.26226627213726,1.22561642368954,19.));
#38253=CARTESIAN_POINT('Ctrl Pts',(2.27504511769678,1.20657818234704,19.));
#38254=CARTESIAN_POINT('Ctrl Pts',(2.28757460208665,1.18736224336636,19.));
#38255=CARTESIAN_POINT('Ctrl Pts',(2.29767202536097,1.17187625340348,19.));
#38256=CARTESIAN_POINT('Ctrl Pts',(2.30760787575165,1.15627404914224,19.));
#38257=CARTESIAN_POINT('Ctrl Pts',(2.3173728786525,1.14057310445739,19.));
#38258=CARTESIAN_POINT('Ctrl Pts',(2.36626838236995,1.06195504289599,19.));
#38259=CARTESIAN_POINT('Ctrl Pts',(2.41093732554403,0.980784092604621,19.));
#38260=CARTESIAN_POINT('Ctrl Pts',(2.45134078885768,0.897488002841355,19.));
#38261=CARTESIAN_POINT('Ctrl Pts',(2.49174425217133,0.814191913078089,19.));
#38262=CARTESIAN_POINT('Ctrl Pts',(2.52788268151298,0.728769767807054,19.));
#38263=CARTESIAN_POINT('Ctrl Pts',(2.55967588129444,0.641608270327732,19.));
#38264=CARTESIAN_POINT('Ctrl Pts',(2.56709861757521,0.621258736022559,19.));
#38265=CARTESIAN_POINT('Ctrl Pts',(2.57428579191308,0.600809491436937,19.));
#38266=CARTESIAN_POINT('Ctrl Pts',(2.58122657684236,0.580294271376261,19.));
#38267=CARTESIAN_POINT('Ctrl Pts',(2.61095617640783,0.492421028851814,19.));
#38268=CARTESIAN_POINT('Ctrl Pts',(2.63620257234987,0.403252571641342,19.));
#38269=CARTESIAN_POINT('Ctrl Pts',(2.65693219715155,0.313192377058794,19.));
#38270=CARTESIAN_POINT('Ctrl Pts',(2.67785890801516,0.222275938851151,19.));
#38271=CARTESIAN_POINT('Ctrl Pts',(2.69418301617952,0.130449883986704,19.));
#38272=CARTESIAN_POINT('Ctrl Pts',(2.70582812757014,0.0380961537513598,
19.));
#38273=CARTESIAN_POINT('Ctrl Pts',(2.7173871594921,-0.053574907185146,19.));
#38274=CARTESIAN_POINT('Ctrl Pts',(2.72433645988727,-0.145766797275223,
19.));
#38275=CARTESIAN_POINT('Ctrl Pts',(2.72655438838951,-0.238125122553047,
19.));
#38276=CARTESIAN_POINT('Ctrl Pts',(2.72766307746563,-0.284292826435247,
19.));
#38277=CARTESIAN_POINT('Ctrl Pts',(2.72758874267574,-0.330502332613507,
19.));
#38278=CARTESIAN_POINT('Ctrl Pts',(2.7263113205947,-0.376710079492555,19.));
#38279=CARTESIAN_POINT('Ctrl Pts',(2.72590026760623,-0.391578956997802,
19.));
#38280=CARTESIAN_POINT('Ctrl Pts',(2.72536453099617,-0.406449511013278,
19.));
#38281=CARTESIAN_POINT('Ctrl Pts',(2.72470363155247,-0.421314426811493,
19.));
#38282=CARTESIAN_POINT('Ctrl Pts',(2.72044884926157,-0.517012768060392,
19.));
#38283=CARTESIAN_POINT('Ctrl Pts',(2.71102631571702,-0.612146448503198,
19.));
#38284=CARTESIAN_POINT('Ctrl Pts',(2.69637150956148,-0.706317860645507,
19.));
#38285=CARTESIAN_POINT('Ctrl Pts',(2.69188202618866,-0.735167166772145,
19.));
#38286=CARTESIAN_POINT('Ctrl Pts',(2.68690115838408,-0.763926315013593,
19.));
#38287=CARTESIAN_POINT('Ctrl Pts',(2.68142612955932,-0.792584206033749,
19.));
#38288=CARTESIAN_POINT('Ctrl Pts',(2.66426531149033,-0.882408911944773,
19.));
#38289=CARTESIAN_POINT('Ctrl Pts',(2.64225376298974,-0.971238746161415,
19.));
#38290=CARTESIAN_POINT('Ctrl Pts',(2.6156937144733,-1.05884271791686,19.));
#38291=CARTESIAN_POINT('Ctrl Pts',(2.58843258219245,-1.1487590996914,19.));
#38292=CARTESIAN_POINT('Ctrl Pts',(2.55637947329957,-1.23738475688051,19.));
#38293=CARTESIAN_POINT('Ctrl Pts',(2.51980654956128,-1.32446593606375,19.));
#38294=CARTESIAN_POINT('Ctrl Pts',(2.50496207587815,-1.35981105317639,19.0000000000001));
#38295=CARTESIAN_POINT('Ctrl Pts',(2.48937238980909,-1.39490162057123,19.));
#38296=CARTESIAN_POINT('Ctrl Pts',(2.47305333806873,-1.42972006310193,19.));
#38297=CARTESIAN_POINT('Ctrl Pts',(2.46410614090769,-1.4488098653232,19.));
#38298=CARTESIAN_POINT('Ctrl Pts',(2.45493674697894,-1.4678235108951,19.));
#38299=CARTESIAN_POINT('Ctrl Pts',(2.4455633016621,-1.48672715429945,19.));
#38300=CARTESIAN_POINT('Ctrl Pts',(2.40280960551886,-1.57294951958685,19.));
#38301=CARTESIAN_POINT('Ctrl Pts',(2.35577316937404,-1.65697997837645,19.0000000000001));
#38302=CARTESIAN_POINT('Ctrl Pts',(2.30479723925007,-1.73857029447992,19.0000000000001));
#38303=CARTESIAN_POINT('Ctrl Pts',(2.25290166294845,-1.82163256454589,19.0000000000001));
#38304=CARTESIAN_POINT('Ctrl Pts',(2.19692283851795,-1.90216661241328,19.));
#38305=CARTESIAN_POINT('Ctrl Pts',(2.13716847969409,-1.97990352796869,19.));
#38306=CARTESIAN_POINT('Ctrl Pts',(2.0767383010823,-2.05851964542366,19.));
#38307=CARTESIAN_POINT('Ctrl Pts',(2.0124462676305,-2.13427584401283,19.));
#38308=CARTESIAN_POINT('Ctrl Pts',(1.94456136809724,-2.20687471793412,19.));
#38309=CARTESIAN_POINT('Ctrl Pts',(1.90683095180258,-2.24722516043911,19.));
#38310=CARTESIAN_POINT('Ctrl Pts',(1.86798981428088,-2.28659984954058,19.));
#38311=CARTESIAN_POINT('Ctrl Pts',(1.82807845289491,-2.32494369604583,19.));
#38312=CARTESIAN_POINT('Ctrl Pts',(1.81563649922765,-2.33689699317917,19.));
#38313=CARTESIAN_POINT('Ctrl Pts',(1.8030905122664,-2.3487500864603,19.));
#38314=CARTESIAN_POINT('Ctrl Pts',(1.79044164710463,-2.36050123580217,19.));
#38315=CARTESIAN_POINT('Ctrl Pts',(1.77881491495006,-2.37130279500602,19.));
#38316=CARTESIAN_POINT('Ctrl Pts',(1.76710642618068,-2.38201336392629,19.));
#38317=CARTESIAN_POINT('Ctrl Pts',(1.75532326360259,-2.3926265773167,19.));
#38318=CARTESIAN_POINT('Ctrl Pts',(1.67947459249907,-2.46094424046239,19.));
#38319=CARTESIAN_POINT('Ctrl Pts',(1.60046191187938,-2.52529830027693,19.));
#38320=CARTESIAN_POINT('Ctrl Pts',(1.51861373809775,-2.58540650642712,19.));
#38321=CARTESIAN_POINT('Ctrl Pts',(1.43669065585186,-2.64556972435346,19.));
#38322=CARTESIAN_POINT('Ctrl Pts',(1.3519263069689,-2.70148015019673,19.));
#38323=CARTESIAN_POINT('Ctrl Pts',(1.26460510700938,-2.75282858062769,19.));
#38324=CARTESIAN_POINT('Ctrl Pts',(1.17908172869413,-2.80311981853642,19.));
#38325=CARTESIAN_POINT('Ctrl Pts',(1.09110502956105,-2.84903564783563,19.));
#38326=CARTESIAN_POINT('Ctrl Pts',(1.00090853688297,-2.89024952005485,19.));
#38327=CARTESIAN_POINT('Ctrl Pts',(0.958564568973025,-2.90959793184868,
19.));
#38328=CARTESIAN_POINT('Ctrl Pts',(0.915730940586028,-2.92790946721792,
19.));
#38329=CARTESIAN_POINT('Ctrl Pts',(0.872429800746574,-2.9451468693802,19.));
#38330=CARTESIAN_POINT('Ctrl Pts',(0.847090664778629,-2.95523392202463,
19.));
#38331=CARTESIAN_POINT('Ctrl Pts',(0.821591411205071,-2.96495310066958,
19.));
#38332=CARTESIAN_POINT('Ctrl Pts',(0.795939046661962,-2.9743059911117,19.));
#38333=CARTESIAN_POINT('Ctrl Pts',(-0.793799282532847,-2.9692229537457,
19.));
#38334=CARTESIAN_POINT('Ctrl Pts',(-0.888615130963527,-2.93453889285012,
19.));
#38335=CARTESIAN_POINT('Ctrl Pts',(-0.981388558303585,-2.89487155596002,
19.));
#38336=CARTESIAN_POINT('Ctrl Pts',(-1.07187896565258,-2.85054012617705,
19.));
#38337=CARTESIAN_POINT('Ctrl Pts',(-1.15599932688489,-2.80932939460297,
19.));
#38338=CARTESIAN_POINT('Ctrl Pts',(-1.23814690070078,-2.76408714469173,
19.));
#38339=CARTESIAN_POINT('Ctrl Pts',(-1.31810348196186,-2.71503958519401,
19.));
#38340=CARTESIAN_POINT('Ctrl Pts',(-1.35017372493085,-2.69536681873353,
19.));
#38341=CARTESIAN_POINT('Ctrl Pts',(-1.38189112492164,-2.67508161858673,
19.));
#38342=CARTESIAN_POINT('Ctrl Pts',(-1.41324046584797,-2.65419744845672,
19.));
#38343=CARTESIAN_POINT('Ctrl Pts',(-1.43613725714475,-2.63894416176093,
19.));
#38344=CARTESIAN_POINT('Ctrl Pts',(-1.45883823398285,-2.62337064619425,
19.));
#38345=CARTESIAN_POINT('Ctrl Pts',(-1.48131237055426,-2.60750044237383,
19.));
#38346=CARTESIAN_POINT('Ctrl Pts',(-1.56372381597803,-2.54930526180017,
19.));
#38347=CARTESIAN_POINT('Ctrl Pts',(-1.64317247712071,-2.48706837685107,
19.));
#38348=CARTESIAN_POINT('Ctrl Pts',(-1.71939078398944,-2.42108429282079,
19.));
#38349=CARTESIAN_POINT('Ctrl Pts',(-1.79517577692462,-2.35547533944059,
19.));
#38350=CARTESIAN_POINT('Ctrl Pts',(-1.86776755723005,-2.28616087364922,
19.));
#38351=CARTESIAN_POINT('Ctrl Pts',(-1.93685978978932,-2.21340329421133,
19.));
#38352=CARTESIAN_POINT('Ctrl Pts',(-1.94744191636753,-2.20225978521449,
19.));
#38353=CARTESIAN_POINT('Ctrl Pts',(-1.957941859472,-2.19103546959794,19.));
#38354=CARTESIAN_POINT('Ctrl Pts',(-1.96835841626289,-2.17973125176718,
19.));
#38355=CARTESIAN_POINT('Ctrl Pts',(-1.97910256215294,-2.16807152888707,
19.));
#38356=CARTESIAN_POINT('Ctrl Pts',(-1.98975557035597,-2.15632935540799,
19.));
#38357=CARTESIAN_POINT('Ctrl Pts',(-2.00030982273794,-2.14451320385199,
19.));
#38358=CARTESIAN_POINT('Ctrl Pts',(-2.06583921208678,-2.07114891731656,
19.));
#38359=CARTESIAN_POINT('Ctrl Pts',(-2.12764079549692,-1.99485340794642,
19.));
#38360=CARTESIAN_POINT('Ctrl Pts',(-2.18547080821429,-1.91590255754304,
19.));
#38361=CARTESIAN_POINT('Ctrl Pts',(-2.2427282128697,-1.83773344470661,19.));
#38362=CARTESIAN_POINT('Ctrl Pts',(-2.29609272962286,-1.75696053678876,
19.));
#38363=CARTESIAN_POINT('Ctrl Pts',(-2.34528221055344,-1.67382965172358,
19.));
#38364=CARTESIAN_POINT('Ctrl Pts',(-2.39315017704695,-1.59293214385006,
19.));
#38365=CARTESIAN_POINT('Ctrl Pts',(-2.43706464605655,-1.50980096441262,
19.));
#38366=CARTESIAN_POINT('Ctrl Pts',(-2.47671778170977,-1.42465253741248,
19.));
#38367=CARTESIAN_POINT('Ctrl Pts',(-2.4975495968377,-1.37991972472364,19.));
#38368=CARTESIAN_POINT('Ctrl Pts',(-2.51720448567013,-1.33463005646684,
19.));
#38369=CARTESIAN_POINT('Ctrl Pts',(-2.53563199193951,-1.28881469101987,
19.));
#38370=CARTESIAN_POINT('Ctrl Pts',(-2.54352364960637,-1.26919406657378,
19.));
#38371=CARTESIAN_POINT('Ctrl Pts',(-2.55119015084139,-1.24947702985283,
19.));
#38372=CARTESIAN_POINT('Ctrl Pts',(-2.558627292172,-1.22966604205277,19.));
#38373=CARTESIAN_POINT('Ctrl Pts',(-2.56380159783432,-1.21588277482774,
19.));
#38374=CARTESIAN_POINT('Ctrl Pts',(-2.56886136486992,-1.2020633573541,19.));
#38375=CARTESIAN_POINT('Ctrl Pts',(-2.57380496377742,-1.1882106589647,19.));
#38376=CARTESIAN_POINT('Ctrl Pts',(-2.60500114582706,-1.10079432343262,
19.));
#38377=CARTESIAN_POINT('Ctrl Pts',(-2.63158503259151,-1.01202802807364,
19.));
#38378=CARTESIAN_POINT('Ctrl Pts',(-2.65330350896804,-0.922133451262639,
19.));
#38379=CARTESIAN_POINT('Ctrl Pts',(-2.657652648649,-0.904132001053431,19.));
#38380=CARTESIAN_POINT('Ctrl Pts',(-2.66180651953586,-0.886085276269219,
19.));
#38381=CARTESIAN_POINT('Ctrl Pts',(-2.66576283715123,-0.867995020296969,
19.));
#38382=CARTESIAN_POINT('Ctrl Pts',(-2.68634765000717,-0.773870996417419,
19.));
#38383=CARTESIAN_POINT('Ctrl Pts',(-2.70158902014984,-0.678568135390762,
19.));
#38384=CARTESIAN_POINT('Ctrl Pts',(-2.71160493858769,-0.582507485590656,
19.));
#38385=CARTESIAN_POINT('Ctrl Pts',(-2.72162085702555,-0.486446835790551,
19.));
#38386=CARTESIAN_POINT('Ctrl Pts',(-2.72641091914393,-0.389627299878367,
19.));
#38387=CARTESIAN_POINT('Ctrl Pts',(-2.72603908754498,-0.292484286395949,
19.));
#38388=CARTESIAN_POINT('Ctrl Pts',(-2.72590978680933,-0.258703770857363,
19.));
#38389=CARTESIAN_POINT('Ctrl Pts',(-2.72515584320796,-0.224884343071014,
19.));
#38390=CARTESIAN_POINT('Ctrl Pts',(-2.72377855213201,-0.191045091866269,
19.));
#38391=CARTESIAN_POINT('Ctrl Pts',(-2.7231767189462,-0.176258395928407,
19.));
#38392=CARTESIAN_POINT('Ctrl Pts',(-2.72245573154192,-0.161467085930695,
19.));
#38393=CARTESIAN_POINT('Ctrl Pts',(-2.72161681874514,-0.146689284135826,
19.));
#38394=CARTESIAN_POINT('Ctrl Pts',(-2.71634351414503,-0.0537978054471125,
19.));
#38395=CARTESIAN_POINT('Ctrl Pts',(-2.70640974169451,0.0387150029297866,
19.));
#38396=CARTESIAN_POINT('Ctrl Pts',(-2.69194108921809,0.13047643871239,19.));
#38397=CARTESIAN_POINT('Ctrl Pts',(-2.67748555890325,0.222154652620047,
19.));
#38398=CARTESIAN_POINT('Ctrl Pts',(-2.65850296606126,0.313083812823312,
19.));
#38399=CARTESIAN_POINT('Ctrl Pts',(-2.63506963364658,0.402875196637659,
19.));
#38400=CARTESIAN_POINT('Ctrl Pts',(-2.61213985997088,0.490737053946578,
19.));
#38401=CARTESIAN_POINT('Ctrl Pts',(-2.58494807707803,0.577510266859945,
19.));
#38402=CARTESIAN_POINT('Ctrl Pts',(-2.55352582338791,0.662801815998425,
19.));
#38403=CARTESIAN_POINT('Ctrl Pts',(-2.53742957959053,0.706492939567349,
19.));
#38404=CARTESIAN_POINT('Ctrl Pts',(-2.52022262780236,0.749794726035084,
19.));
#38405=CARTESIAN_POINT('Ctrl Pts',(-2.50190563126205,0.792650359973834,
19.));
#38406=CARTESIAN_POINT('Ctrl Pts',(-2.49657257443339,0.80512792586302,19.));
#38407=CARTESIAN_POINT('Ctrl Pts',(-2.49114540403142,0.81756765143535,19.));
#38408=CARTESIAN_POINT('Ctrl Pts',(-2.48562410083644,0.829968083953126,
19.));
#38409=CARTESIAN_POINT('Ctrl Pts',(-2.47996475337123,0.84267855353951,19.));
#38410=CARTESIAN_POINT('Ctrl Pts',(-2.47421005306852,0.855339737996612,
19.));
#38411=CARTESIAN_POINT('Ctrl Pts',(-2.46836165037947,0.867947484860423,
19.));
#38412=CARTESIAN_POINT('Ctrl Pts',(-2.43086233923552,0.948786963194456,
19.));
#38413=CARTESIAN_POINT('Ctrl Pts',(-2.38949695437655,1.02747039787255,19.));
#38414=CARTESIAN_POINT('Ctrl Pts',(-2.34433717506969,1.10364922240285,18.9999999999999));
#38415=CARTESIAN_POINT('Ctrl Pts',(-2.29994053932711,1.17854072045439,19.));
#38416=CARTESIAN_POINT('Ctrl Pts',(-2.25187620865753,1.25101221296806,19.));
#38417=CARTESIAN_POINT('Ctrl Pts',(-2.20017617040085,1.32069832886965,19.));
#38418=CARTESIAN_POINT('Ctrl Pts',(-2.15008171884632,1.3882202858114,19.));
#38419=CARTESIAN_POINT('Ctrl Pts',(-2.09657342616567,1.45312762148621,18.9999999999999));
#38420=CARTESIAN_POINT('Ctrl Pts',(-2.03965286195605,1.51504773829594,19.));
#38421=CARTESIAN_POINT('Ctrl Pts',(-2.01565725834268,1.54115096828483,19.));
#38422=CARTESIAN_POINT('Ctrl Pts',(-1.99105493705542,1.5667227863261,19.));
#38423=CARTESIAN_POINT('Ctrl Pts',(-1.96584476256622,1.59173275781375,19.));
#38424=CARTESIAN_POINT('Ctrl Pts',(-1.94982433031677,1.60762596608768,19.));
#38425=CARTESIAN_POINT('Ctrl Pts',(-1.93355840885751,1.62329224800863,19.));
#38426=CARTESIAN_POINT('Ctrl Pts',(-1.91705291980301,1.6387286579029,19.));
#38427=CARTESIAN_POINT('Ctrl Pts',(-1.90925347387187,1.63408080983891,0.00248200680218311));
#38428=CARTESIAN_POINT('Ctrl Pts',(-2.45156644640155,1.00049596865414,0.0552988434666635));
#38429=CARTESIAN_POINT('Ctrl Pts',(-2.84651267184705,-0.837496618391379,
0.160905316059202));
#38430=CARTESIAN_POINT('Ctrl Pts',(-0.842979713689217,-2.8475711288532,
0.3193014245798));
#38431=CARTESIAN_POINT('Ctrl Pts',(1.92769349397626,-2.25538582349437,0.477670332363976));
#38432=CARTESIAN_POINT('Ctrl Pts',(2.94229596891705,0.387912730907106,0.636039240148151));
#38433=CARTESIAN_POINT('Ctrl Pts',(1.2760586532515,2.67973607720936,0.794408147932327));
#38434=CARTESIAN_POINT('Ctrl Pts',(-1.55272782208431,2.52904086654082,0.952777055716503));
#38435=CARTESIAN_POINT('Ctrl Pts',(-2.96686221862994,0.0746779472267705,
1.11114596350068));
#38436=CARTESIAN_POINT('Ctrl Pts',(-1.67788023304716,-2.44800315617183,
1.26951487128486));
#38437=CARTESIAN_POINT('Ctrl Pts',(1.13980404363706,-2.74016996198817,1.42788377906903));
#38438=CARTESIAN_POINT('Ctrl Pts',(2.91902120615094,-0.535853057404118,
1.5862526868532));
#38439=CARTESIAN_POINT('Ctrl Pts',(2.03872475226955,2.15671799727073,1.74462159463738));
#38440=CARTESIAN_POINT('Ctrl Pts',(-0.699046144647114,2.88428901959944,
1.90299050242156));
#38441=CARTESIAN_POINT('Ctrl Pts',(-2.79991896953276,0.984004316378271,
2.06135941020573));
#38442=CARTESIAN_POINT('Ctrl Pts',(-2.34979400265249,-1.81280940468846,
2.21972831798991));
#38443=CARTESIAN_POINT('Ctrl Pts',(0.241220755203426,-2.95797512221762,
2.37809722577408));
#38444=CARTESIAN_POINT('Ctrl Pts',(2.61246013485936,-1.40814051945854,2.53646613355826));
#38445=CARTESIAN_POINT('Ctrl Pts',(2.60349519023718,1.42464734080985,2.69483504134244));
#38446=CARTESIAN_POINT('Ctrl Pts',(0.222493933180336,2.95944302392479,2.85320394912661));
#38447=CARTESIAN_POINT('Ctrl Pts',(-2.36122086593176,1.79789963417574,3.01157285691079));
#38448=CARTESIAN_POINT('Ctrl Pts',(-2.79363469858403,-1.00170461775365,
3.16994176469496));
#38449=CARTESIAN_POINT('Ctrl Pts',(-0.680776683187599,-2.88865885771179,
3.32831067247914));
#38450=CARTESIAN_POINT('Ctrl Pts',(2.05233484485897,-2.14376506356077,3.48667958026332));
#38451=CARTESIAN_POINT('Ctrl Pts',(2.91557050223709,0.554306404036049,3.64504848804749));
#38452=CARTESIAN_POINT('Ctrl Pts',(1.12243897822204,2.74735102858266,3.80341739583167));
#38453=CARTESIAN_POINT('Ctrl Pts',(-1.6933431948019,2.4372927131013,3.96178630361584));
#38454=CARTESIAN_POINT('Ctrl Pts',(-2.96632566963744,-0.0933753863158161,
4.12015521140002));
#38455=CARTESIAN_POINT('Ctrl Pts',(-1.53669808804495,-2.5389694615051,4.27852411918419));
#38456=CARTESIAN_POINT('Ctrl Pts',(1.29301032391677,-2.67131638784702,4.43689302696837));
#38457=CARTESIAN_POINT('Ctrl Pts',(2.94466106661435,-0.369835292927075,
4.59526193475254));
#38458=CARTESIAN_POINT('Ctrl Pts',(1.91344030499105,2.26860158254042,4.75363084253672));
#38459=CARTESIAN_POINT('Ctrl Pts',(-0.861109944606757,2.84012263900151,
4.91199975032089));
#38460=CARTESIAN_POINT('Ctrl Pts',(-2.85110561212216,0.824016826100779,
5.07036865810507));
#38461=CARTESIAN_POINT('Ctrl Pts',(-2.24346785780728,-1.9428481443896,5.22873756588924));
#38462=CARTESIAN_POINT('Ctrl Pts',(0.408186457476231,-2.93959023626285,
5.38710647367343));
#38463=CARTESIAN_POINT('Ctrl Pts',(2.68794336574243,-1.2580808414982,5.54547538145759));
#38464=CARTESIAN_POINT('Ctrl Pts',(2.51872346544836,1.56966208012581,5.70384428924178));
#38465=CARTESIAN_POINT('Ctrl Pts',(0.054702479433918,2.9672907811558,5.86221319702594));
#38466=CARTESIAN_POINT('Ctrl Pts',(-2.45915776480731,1.66143011558536,6.02058210481013));
#38467=CARTESIAN_POINT('Ctrl Pts',(-2.73248704721367,-1.15815434118082,
6.1789510125943));
#38468=CARTESIAN_POINT('Ctrl Pts',(-0.516255911939875,-2.92254799354502,
6.33731992037847));
#38469=CARTESIAN_POINT('Ctrl Pts',(2.17033437291138,-2.02421729341143,6.49568882816265));
#38470=CARTESIAN_POINT('Ctrl Pts',(2.87953978655513,0.718371462986052,6.65405773594683));
#38471=CARTESIAN_POINT('Ctrl Pts',(0.965205490814753,2.80645422226833,6.812426643731));
#38472=CARTESIAN_POINT('Ctrl Pts',(-1.82852451416062,2.3375853016094,6.97079555151518));
#38473=CARTESIAN_POINT('Ctrl Pts',(-2.95629154307943,-0.261050289223455,
7.12916445929935));
#38474=CARTESIAN_POINT('Ctrl Pts',(-1.39059057686979,-2.62184377656405,
7.28753336708353));
#38475=CARTESIAN_POINT('Ctrl Pts',(1.44207312239444,-2.5938835846765,7.4459022748677));
#38476=CARTESIAN_POINT('Ctrl Pts',(2.96086850210907,-0.202644157095674,
7.60427118265188));
#38477=CARTESIAN_POINT('Ctrl Pts',(1.78202583361296,2.37322372934426,7.76264009043606));
#38478=CARTESIAN_POINT('Ctrl Pts',(-1.02041500826522,2.78685488536697,7.92100899822022));
#38479=CARTESIAN_POINT('Ctrl Pts',(-2.89315892192767,0.661391256108661,
8.07937790600442));
#38480=CARTESIAN_POINT('Ctrl Pts',(-2.12995477448807,-2.06666388167551,
8.23774681378858));
#38481=CARTESIAN_POINT('Ctrl Pts',(0.573844518103784,-2.91178800914985,
8.39611572157276));
#38482=CARTESIAN_POINT('Ctrl Pts',(2.75481586183833,-1.1039911723155,8.55448462935694));
#38483=CARTESIAN_POINT('Ctrl Pts',(2.42588307460051,1.70964857486957,8.7128535371411));
#38484=CARTESIAN_POINT('Ctrl Pts',(-0.113264208110999,2.96563284314625,
8.8712224449253));
#38485=CARTESIAN_POINT('Ctrl Pts',(-2.54921682443218,1.51963828696783,9.02959135270946));
#38486=CARTESIAN_POINT('Ctrl Pts',(-2.66258595086561,-1.3108939680385,9.18796026049363));
#38487=CARTESIAN_POINT('Ctrl Pts',(-0.350081330264974,-2.94707482147749,
9.34632916827782));
#38488=CARTESIAN_POINT('Ctrl Pts',(2.28138129735905,-1.89818500606422,9.50469807606198));
#38489=CARTESIAN_POINT('Ctrl Pts',(2.83428454760838,0.880135242093526,9.66306698384617));
#38490=CARTESIAN_POINT('Ctrl Pts',(0.804879995387632,2.85656701903027,9.82143589163034));
#38491=CARTESIAN_POINT('Ctrl Pts',(-1.95784820773308,2.23038950335204,9.97980479941452));
#38492=CARTESIAN_POINT('Ctrl Pts',(-2.93678702134196,-0.427888925381411,
10.1381737071986));
#38493=CARTESIAN_POINT('Ctrl Pts',(-1.24002834868274,-2.69631909010226,
10.2965426149829));
#38494=CARTESIAN_POINT('Ctrl Pts',(1.58651628099675,-2.50814134994797,10.4549115227671));
#38495=CARTESIAN_POINT('Ctrl Pts',(2.96759088028684,-0.0348038564676998,
10.6132804305513));
#38496=CARTESIAN_POINT('Ctrl Pts',(1.6449026935962,2.47024332197998,10.7716493383355));
#38497=CARTESIAN_POINT('Ctrl Pts',(-1.17645120171631,2.72465952206268,10.9300182461196));
#38498=CARTESIAN_POINT('Ctrl Pts',(-2.92594408011687,0.496646938192196,
11.0883871539037));
#38499=CARTESIAN_POINT('Ctrl Pts',(-2.00961844214704,-2.18385912049501,
11.2467560616879));
#38500=CARTESIAN_POINT('Ctrl Pts',(0.73766428427855,-2.87465795267654,11.4051249694722));
#38501=CARTESIAN_POINT('Ctrl Pts',(2.81286338434295,-0.946364899079276,
11.5634938772563));
#38502=CARTESIAN_POINT('Ctrl Pts',(2.32527143690989,1.84415825944458,11.7218627850405));
#38503=CARTESIAN_POINT('Ctrl Pts',(-0.280868057014231,2.95447458539345,
11.8802316928247));
#38504=CARTESIAN_POINT('Ctrl Pts',(-2.6311095410845,1.37297834068884,12.0386006006089));
#38505=CARTESIAN_POINT('Ctrl Pts',(-2.5841553368005,-1.4594341836726,12.196969508393));
#38506=CARTESIAN_POINT('Ctrl Pts',(-0.182785273090703,-2.96216077975654,
12.3553384161772));
#38507=CARTESIAN_POINT('Ctrl Pts',(2.38511988226226,-1.7660719374997,12.5137073239614));
#38508=CARTESIAN_POINT('Ctrl Pts',(2.7799497594151,1.03907953319971,12.6720762317456));
#38509=CARTESIAN_POINT('Ctrl Pts',(0.641976089983368,2.89752888528765,12.8304451395297));
#38510=CARTESIAN_POINT('Ctrl Pts',(-2.08089999073317,2.11604871629969,12.9888140473139));
#38511=CARTESIAN_POINT('Ctrl Pts',(-2.9078745866236,-0.593356831641015,
13.1471829550981));
#38512=CARTESIAN_POINT('Ctrl Pts',(-1.08549372525115,-2.76215682277935,
13.3055518628823));
#38513=CARTESIAN_POINT('Ctrl Pts',(1.72587708020246,-2.41436435635144,13.4639207706664));
#38514=CARTESIAN_POINT('Ctrl Pts',(2.96480666620496,0.133147937316626,13.6222896784505));
#38515=CARTESIAN_POINT('Ctrl Pts',(1.50251015498524,2.55934956099197,13.7806585862348));
#38516=CARTESIAN_POINT('Ctrl Pts',(-1.32871866749039,2.6537357901384,13.939027494019));
#38517=CARTESIAN_POINT('Ctrl Pts',(-2.94935606037441,0.330311626052199,
14.0973964018031));
#38518=CARTESIAN_POINT('Ctrl Pts',(-1.88284435477652,-2.29405842925977,
14.2557653095873));
#38519=CARTESIAN_POINT('Ctrl Pts',(0.899120964085925,-2.828319011924,14.4141342173715));
#38520=CARTESIAN_POINT('Ctrl Pts',(2.86189997966902,-0.785706973011972,
14.5725031251557));
#38521=CARTESIAN_POINT('Ctrl Pts',(2.21721085889867,1.97276023589046,14.7308720329398));
#38522=CARTESIAN_POINT('Ctrl Pts',(-0.447572153204858,2.93385175314142,
14.889240940724));
#38523=CARTESIAN_POINT('Ctrl Pts',(-2.70457357369761,1.22192009751584,15.0476098485082));
#38524=CARTESIAN_POINT('Ctrl Pts',(-2.49744645542791,-1.60329914345083,
15.2059787562924));
#38525=CARTESIAN_POINT('Ctrl Pts',(-0.0149036681797597,-2.96775754154435,
15.3643476640765));
#38526=CARTESIAN_POINT('Ctrl Pts',(2.48121780335728,-1.6283013070035,15.5227165718607));
#38527=CARTESIAN_POINT('Ctrl Pts',(2.71670948321466,1.19469516065056,15.6810854796449));
#38528=CARTESIAN_POINT('Ctrl Pts',(0.47701563009963,2.92920860503424,15.8394543874291));
#38529=CARTESIAN_POINT('Ctrl Pts',(-2.19728566554779,1.99492921994414,15.9978232952133));
#38530=CARTESIAN_POINT('Ctrl Pts',(-2.86964686816259,-0.756923921148106,
16.1561922029974));
#38531=CARTESIAN_POINT('Ctrl Pts',(-0.927481736461798,-2.81914609426518,
16.3145611107816));
#38532=CARTESIAN_POINT('Ctrl Pts',(1.85970904856091,-2.31285296049272,16.4729300185658));
#38533=CARTESIAN_POINT('Ctrl Pts',(2.95252484228036,0.300673089886709,16.6312989263498));
#38534=CARTESIAN_POINT('Ctrl Pts',(1.35530424736705,2.64025719880453,16.7896678341341));
#38535=CARTESIAN_POINT('Ctrl Pts',(-1.47672939037767,2.57431050652288,16.9480367419183));
#38536=CARTESIAN_POINT('Ctrl Pts',(-2.9633203037766,0.162918905759724,17.1064056497025));
#38537=CARTESIAN_POINT('Ctrl Pts',(-1.75003778792055,-2.39691019261269,
17.2647745574867));
#38538=CARTESIAN_POINT('Ctrl Pts',(1.05769572839716,-2.77291694918154,17.4231434652708));
#38539=CARTESIAN_POINT('Ctrl Pts',(2.90177163005296,-0.622537181450101,
17.581512373055));
#38540=CARTESIAN_POINT('Ctrl Pts',(2.10204164733985,2.09505231770878,17.7398812808392));
#38541=CARTESIAN_POINT('Ctrl Pts',(-0.612831269401328,2.90381172146501,
17.8982501886234));
#38542=CARTESIAN_POINT('Ctrl Pts',(-2.7693949632942,1.06698316123474,18.0566190964075));
#38543=CARTESIAN_POINT('Ctrl Pts',(-2.40269624306919,-1.74209614650769,
18.2149880041917));
#38544=CARTESIAN_POINT('Ctrl Pts',(0.152947696564397,-2.96371698990033,
18.3733569119759));
#38545=CARTESIAN_POINT('Ctrl Pts',(2.56951616178647,-1.48556313374885,18.53172581976));
#38546=CARTESIAN_POINT('Ctrl Pts',(2.64448170946715,1.34695892431768,18.6900947275442));
#38547=CARTESIAN_POINT('Ctrl Pts',(0.311071818696124,2.95059345609503,18.8484636353284));
#38548=CARTESIAN_POINT('Ctrl Pts',(-2.30768370382183,1.86919021361793,19.0068325431126));
#38549=CARTESIAN_POINT('Ctrl Pts',(-2.8201996789474,-0.922146939298692,
19.1652256218881));
#38550=CARTESIAN_POINT('Ctrl Pts',(-1.45369664976329,-2.21310559305866,
19.2708290647355));
#38551=CARTESIAN_POINT('Ctrl Pts',(-0.647946980571831,-2.42809259672558,
19.3236428716548));
#38552=CARTESIAN_POINT('Ctrl Pts',(-2.05218096726007,1.75640876541957,-0.106134133512484));
#38553=CARTESIAN_POINT('Ctrl Pts',(-2.63509170999486,1.07539350473389,-0.0533172968480037));
#38554=CARTESIAN_POINT('Ctrl Pts',(-3.0596037708826,-0.900191956661482,
0.0522891757445352));
#38555=CARTESIAN_POINT('Ctrl Pts',(-0.906085518708576,-3.06074146441173,
0.210685284265133));
#38556=CARTESIAN_POINT('Ctrl Pts',(2.0720014147868,-2.42422492568104,0.369054192049308));
#38557=CARTESIAN_POINT('Ctrl Pts',(3.1625574446187,0.416952036080915,0.527423099833484));
#38558=CARTESIAN_POINT('Ctrl Pts',(1.37158492423724,2.88034221238152,0.685792007617659));
#38559=CARTESIAN_POINT('Ctrl Pts',(-1.66896565983697,2.7183658968093,0.844160915401836));
#38560=CARTESIAN_POINT('Ctrl Pts',(-3.18896273379987,0.0802683687996882,
1.00252982318601));
#38561=CARTESIAN_POINT('Ctrl Pts',(-1.80348703130465,-2.63126167040592,
1.16089873097018));
#38562=CARTESIAN_POINT('Ctrl Pts',(1.22513023900094,-2.94530020241159,1.31926763875436));
#38563=CARTESIAN_POINT('Ctrl Pts',(3.13754032362361,-0.575967235729459,
1.47763654653853));
#38564=CARTESIAN_POINT('Ctrl Pts',(2.19134451833939,2.31817078576297,1.63600545432271));
#38565=CARTESIAN_POINT('Ctrl Pts',(-0.75137702401143,3.1002080714278,1.79437436210689));
#38566=CARTESIAN_POINT('Ctrl Pts',(-3.0095220450185,1.05766728064561,1.95274326989106));
#38567=CARTESIAN_POINT('Ctrl Pts',(-2.52570053961777,-1.94851705574079,
2.11111217767524));
#38568=CARTESIAN_POINT('Ctrl Pts',(0.259278639275,-3.17941034572717,2.26948108545941));
#38569=CARTESIAN_POINT('Ctrl Pts',(2.80802996556119,-1.51355449279358,2.42784999324359));
#38570=CARTESIAN_POINT('Ctrl Pts',(2.79839390152992,1.53129702152048,2.58621890102776));
#38571=CARTESIAN_POINT('Ctrl Pts',(0.239149919721012,3.18098813515455,2.74458780881194));
#38572=CARTESIAN_POINT('Ctrl Pts',(-2.53798282254046,1.93249113372931,2.90295671659612));
#38573=CARTESIAN_POINT('Ctrl Pts',(-3.00276733098466,-1.07669263379773,
3.06132562438029));
#38574=CARTESIAN_POINT('Ctrl Pts',(-0.731739903219251,-3.10490503740267,
3.21969453216447));
#38575=CARTESIAN_POINT('Ctrl Pts',(2.20597346800839,-2.30424819015504,3.37806343994865));
#38576=CARTESIAN_POINT('Ctrl Pts',(3.13383129860806,0.595802007413021,3.53643234773282));
#38577=CARTESIAN_POINT('Ctrl Pts',(1.20646521770984,2.95301884657881,3.694801255517));
#38578=CARTESIAN_POINT('Ctrl Pts',(-1.82010755668003,2.61974943920086,3.85317016330117));
#38579=CARTESIAN_POINT('Ctrl Pts',(-3.18838601853105,-0.100365505801211,
4.01153907108535));
#38580=CARTESIAN_POINT('Ctrl Pts',(-1.65173593337267,-2.72903775044013,
4.16990797886952));
#38581=CARTESIAN_POINT('Ctrl Pts',(1.38980560387911,-2.8712922216411,4.3282768866537));
#38582=CARTESIAN_POINT('Ctrl Pts',(3.16509959449378,-0.39752131372418,4.48664579443787));
#38583=CARTESIAN_POINT('Ctrl Pts',(2.05668122626364,2.43843002183688,4.64501470222205));
#38584=CARTESIAN_POINT('Ctrl Pts',(-0.925572986103647,3.05273537757325,
4.80338361000622));
#38585=CARTESIAN_POINT('Ctrl Pts',(-3.06454054053909,0.885703061624783,
4.9617525177904));
#38586=CARTESIAN_POINT('Ctrl Pts',(-2.41141477622409,-2.0882905485081,5.12012142557457));
#38587=CARTESIAN_POINT('Ctrl Pts',(0.438743462085874,-3.15964915971496,
5.27849033335875));
#38588=CARTESIAN_POINT('Ctrl Pts',(2.88916390187998,-1.35226128616718,5.43685924114294));
#38589=CARTESIAN_POINT('Ctrl Pts',(2.70727613086501,1.68716762333896,5.5952281489271));
#38590=CARTESIAN_POINT('Ctrl Pts',(0.0587975293445813,3.18942337869112,
5.75359705671128));
#38591=CARTESIAN_POINT('Ctrl Pts',(-2.64325131759118,1.78580545134354,5.91196596449545));
#38592=CARTESIAN_POINT('Ctrl Pts',(-2.93704214150503,-1.24485424729959,
6.07033487227964));
#38593=CARTESIAN_POINT('Ctrl Pts',(-0.554903039966712,-3.14133112775976,
6.22870378006381));
#38594=CARTESIAN_POINT('Ctrl Pts',(2.33280648883499,-2.17575102519698,6.38707268784798));
#38595=CARTESIAN_POINT('Ctrl Pts',(3.0951033088617,0.77214904355946,6.54544159563215));
#38596=CARTESIAN_POINT('Ctrl Pts',(1.0374611673368,3.01654652943803,6.70381050341633));
#38597=CARTESIAN_POINT('Ctrl Pts',(-1.96540860471453,2.51257789023753,6.86217941120051));
#38598=CARTESIAN_POINT('Ctrl Pts',(-3.17760073316836,-0.280592620295555,
7.02054831898468));
#38599=CARTESIAN_POINT('Ctrl Pts',(-1.49469075434814,-2.81811607050928,
7.17891722676886));
#38600=CARTESIAN_POINT('Ctrl Pts',(1.55002730421837,-2.78806276725866,7.33728613455304));
#38601=CARTESIAN_POINT('Ctrl Pts',(3.18252032521683,-0.217814181306611,
7.49565504233721));
#38602=CARTESIAN_POINT('Ctrl Pts',(1.91542901398523,2.55088422520114,7.65402395012139));
#38603=CARTESIAN_POINT('Ctrl Pts',(-1.09680369177055,2.99547997818629,7.81239285790555));
#38604=CARTESIAN_POINT('Ctrl Pts',(-3.10974197826028,0.710903275166445,
7.97076176568975));
#38605=CARTESIAN_POINT('Ctrl Pts',(-2.2894040572124,-2.22137518236246,8.1291306734739));
#38606=CARTESIAN_POINT('Ctrl Pts',(0.616802752664856,-3.12976564654632,
8.28749958125809));
#38607=CARTESIAN_POINT('Ctrl Pts',(2.96104250029515,-1.18663640153263,8.44586848904227));
#38608=CARTESIAN_POINT('Ctrl Pts',(2.60748567051059,1.83763356414668,8.60423739682644));
#38609=CARTESIAN_POINT('Ctrl Pts',(-0.121743212903944,3.18764132676628,
8.76260630461062));
#38610=CARTESIAN_POINT('Ctrl Pts',(-2.74005223513341,1.63339902863226,8.9209752123948));
#38611=CARTESIAN_POINT('Ctrl Pts',(-2.86190822058818,-1.40902802489031,
9.07934412017897));
#38612=CARTESIAN_POINT('Ctrl Pts',(-0.376288561364208,-3.16769404402997,
9.23771302796314));
#38613=CARTESIAN_POINT('Ctrl Pts',(2.45216643131664,-2.04028390944011,9.39608193574732));
#38614=CARTESIAN_POINT('Ctrl Pts',(3.04646024427847,0.946022525116211,9.55445084353148));
#38615=CARTESIAN_POINT('Ctrl Pts',(0.865133639963048,3.07041079059476,9.71281975131568));
#38616=CARTESIAN_POINT('Ctrl Pts',(-2.10441352270846,2.39735737082276,9.87118865909984));
#38617=CARTESIAN_POINT('Ctrl Pts',(-3.15663609498233,-0.459920864770426,
10.029557566884));
#38618=CARTESIAN_POINT('Ctrl Pts',(-1.3328573763802,-2.89816663637986,10.1879264746682));
#38619=CARTESIAN_POINT('Ctrl Pts',(1.70528353655795,-2.69590183388433,10.3462953824524));
#38620=CARTESIAN_POINT('Ctrl Pts',(3.18974594336544,-0.0374092873511558,
10.5046642902366));
#38621=CARTESIAN_POINT('Ctrl Pts',(1.76804077980663,2.65516674409297,10.6630331980207));
#38622=CARTESIAN_POINT('Ctrl Pts',(-1.26452081827374,2.92862864463024,10.8214021058049));
#38623=CARTESIAN_POINT('Ctrl Pts',(-3.14498144675684,0.533826130450403,
10.9797710135891));
#38624=CARTESIAN_POINT('Ctrl Pts',(-2.1600592979755,-2.34734370453628,11.1381399213733));
#38625=CARTESIAN_POINT('Ctrl Pts',(0.792886133318907,-3.08985601890883,
11.2965088291574));
#38626=CARTESIAN_POINT('Ctrl Pts',(3.02343548399835,-1.01721016122337,11.4548777369416));
#38627=CARTESIAN_POINT('Ctrl Pts',(2.4993422046067,1.98221269854377,11.6132466447258));
#38628=CARTESIAN_POINT('Ctrl Pts',(-0.301893954262147,3.17564775728929,
11.77161555251));
#38629=CARTESIAN_POINT('Ctrl Pts',(-2.82807547393906,1.47576005898683,11.9299844602941));
#38630=CARTESIAN_POINT('Ctrl Pts',(-2.77760625878081,-1.56868802162129,
12.0883533680783));
#38631=CARTESIAN_POINT('Ctrl Pts',(-0.196468653149268,-3.18390934329579,
12.2467222758625));
#38632=CARTESIAN_POINT('Ctrl Pts',(2.56367092897621,-1.89828080270509,12.4050911836467));
#38633=CARTESIAN_POINT('Ctrl Pts',(2.9880579316907,1.11686545065049,12.5634600914308));
#38634=CARTESIAN_POINT('Ctrl Pts',(0.690034681790139,3.11443907885885,12.721828999215));
#38635=CARTESIAN_POINT('Ctrl Pts',(-2.23667701234773,2.27445698583902,12.8801979069992));
#38636=CARTESIAN_POINT('Ctrl Pts',(-3.12555926361439,-0.637775765947956,
13.0385668147834));
#38637=CARTESIAN_POINT('Ctrl Pts',(-1.1667542280403,-2.96893300856485,13.1969357225676));
#38638=CARTESIAN_POINT('Ctrl Pts',(1.85507694200457,-2.59510465631764,13.3553046303517));
#38639=CARTESIAN_POINT('Ctrl Pts',(3.18675330188238,0.143115446183788,13.5136735381359));
#38640=CARTESIAN_POINT('Ctrl Pts',(1.61498867770692,2.75094351248282,13.6720424459201));
#38641=CARTESIAN_POINT('Ctrl Pts',(-1.42818708860966,2.85239553322103,13.8304113537043));
#38642=CARTESIAN_POINT('Ctrl Pts',(-3.17014605740068,0.355038889034663,
13.9887802614884));
#38643=CARTESIAN_POINT('Ctrl Pts',(-2.02379485074318,-2.46579257847948,
14.1471491692726));
#38644=CARTESIAN_POINT('Ctrl Pts',(0.96642952599676,-3.04004812616082,14.3055180770568));
#38645=CARTESIAN_POINT('Ctrl Pts',(3.07614297884099,-0.844525317316191,
14.463886984841));
#38646=CARTESIAN_POINT('Ctrl Pts',(2.38319216767315,2.12044187137279,14.6222558926251));
#38647=CARTESIAN_POINT('Ctrl Pts',(-0.481077587052887,3.15348109140769,
14.7806248004093));
#38648=CARTESIAN_POINT('Ctrl Pts',(-2.90703905398222,1.31339353414885,14.9389937081935));
#38649=CARTESIAN_POINT('Ctrl Pts',(-2.68440631520056,-1.72332277093709,
15.0973626159776));
#38650=CARTESIAN_POINT('Ctrl Pts',(-0.0160193628553846,-3.18992508095263,
15.2557315237618));
#38651=CARTESIAN_POINT('Ctrl Pts',(2.66696277962007,-1.7501966066458,15.414100431546));
#38652=CARTESIAN_POINT('Ctrl Pts',(2.9200834626331,1.28413052741122,15.5724693393302));
#38653=CARTESIAN_POINT('Ctrl Pts',(0.512725214631047,3.14849035534036,15.7308382471144));
#38654=CARTESIAN_POINT('Ctrl Pts',(-2.36177536622523,2.14427043461023,15.8892071548985));
#38655=CARTESIAN_POINT('Ctrl Pts',(-3.08446980256532,-0.81358755445598,
16.0475760626827));
#38656=CARTESIAN_POINT('Ctrl Pts',(-0.99691339735436,-3.03018852014659,
16.2059449704669));
#38657=CARTESIAN_POINT('Ctrl Pts',(1.99892762607284,-2.48599407598237,16.364313878251));
#38658=CARTESIAN_POINT('Ctrl Pts',(3.17355205561192,0.323181599969261,16.5226827860353));
#38659=CARTESIAN_POINT('Ctrl Pts',(1.45676287583387,2.83790792904517,16.6810516938194));
#38660=CARTESIAN_POINT('Ctrl Pts',(-1.58727795455092,2.76702444049522,16.8394206016036));
#38661=CARTESIAN_POINT('Ctrl Pts',(-3.18515566975668,0.175115081461092,
16.9977895093878));
#38662=CARTESIAN_POINT('Ctrl Pts',(-1.88104633015191,-2.57634386676597,
17.1561584171719));
#38663=CARTESIAN_POINT('Ctrl Pts',(1.13687526180957,-2.98049864241602,17.3145273249561));
#38664=CARTESIAN_POINT('Ctrl Pts',(3.11899943722691,-0.669140568639529,
17.4728962327403));
#38665=CARTESIAN_POINT('Ctrl Pts',(2.25940134198667,2.25188878829013,17.6312651405244));
#38666=CARTESIAN_POINT('Ctrl Pts',(-0.658708068058032,3.12119225071374,
17.7896340483087));
#38667=CARTESIAN_POINT('Ctrl Pts',(-2.97671299922937,1.14685795565552,17.9480029560928));
#38668=CARTESIAN_POINT('Ctrl Pts',(-2.58256306331841,-1.87251017422536,
18.106371863877));
#38669=CARTESIAN_POINT('Ctrl Pts',(0.164397423480497,-3.18558205196536,
18.2647407716612));
#38670=CARTESIAN_POINT('Ctrl Pts',(2.76187118915734,-1.59677299555207,18.4231096794454));
#38671=CARTESIAN_POINT('Ctrl Pts',(2.84244868829818,1.44779281849893,18.5814785872295));
#38672=CARTESIAN_POINT('Ctrl Pts',(0.334358781856534,3.1714760850694,18.7398474950137));
#38673=CARTESIAN_POINT('Ctrl Pts',(-2.48043784664977,2.00911855501116,18.8982164027979));
#38674=CARTESIAN_POINT('Ctrl Pts',(-3.03132097660764,-0.991179235100812,
19.0566094815733));
#38675=CARTESIAN_POINT('Ctrl Pts',(-1.56252097358454,-2.37877957995877,
19.1622129244208));
#38676=CARTESIAN_POINT('Ctrl Pts',(-0.696452555682176,-2.60986059836271,
19.2150267313402));
#38677=CARTESIAN_POINT('Ctrl Pts',(-2.19510846064826,1.87873672100023,-0.214750273827152));
#38678=CARTESIAN_POINT('Ctrl Pts',(-2.81861697358817,1.15029104081366,-0.161933437162671));
#38679=CARTESIAN_POINT('Ctrl Pts',(-3.27269486991817,-0.962887294931585,
-0.0563269645701317));
#38680=CARTESIAN_POINT('Ctrl Pts',(-0.969191323727936,-3.27391179997027,
0.102069143950466));
#38681=CARTESIAN_POINT('Ctrl Pts',(2.21630933559734,-2.59306402786772,0.260438051734641));
#38682=CARTESIAN_POINT('Ctrl Pts',(3.38281892032033,0.445991341254727,0.418806959518817));
#38683=CARTESIAN_POINT('Ctrl Pts',(1.46711119522298,3.08094834755367,0.577175867302993));
#38684=CARTESIAN_POINT('Ctrl Pts',(-1.78520349758962,2.90769092707777,0.735544775087169));
#38685=CARTESIAN_POINT('Ctrl Pts',(-3.41106324896979,0.0858587903725989,
0.893913682871344));
#38686=CARTESIAN_POINT('Ctrl Pts',(-1.92909382956213,-2.81452018464,1.05228259065552));
#38687=CARTESIAN_POINT('Ctrl Pts',(1.31045643436484,-3.15043044283502,1.2106514984397));
#38688=CARTESIAN_POINT('Ctrl Pts',(3.35605944109629,-0.616081414054793,
1.36902040622387));
#38689=CARTESIAN_POINT('Ctrl Pts',(2.34396428440923,2.4796235742552,1.52738931400805));
#38690=CARTESIAN_POINT('Ctrl Pts',(-0.803707903375748,3.31612712325617,
1.68575822179222));
#38691=CARTESIAN_POINT('Ctrl Pts',(-3.21912512050423,1.13133024491295,1.8441271295764));
#38692=CARTESIAN_POINT('Ctrl Pts',(-2.70160707658305,-2.08422470679312,
2.00249603736058));
#38693=CARTESIAN_POINT('Ctrl Pts',(0.277336523346577,-3.40084556923671,
2.16086494514475));
#38694=CARTESIAN_POINT('Ctrl Pts',(3.00359979626304,-1.61896846612861,2.31923385292893));
#38695=CARTESIAN_POINT('Ctrl Pts',(2.99329261282266,1.63794670223112,2.4776027607131));
#38696=CARTESIAN_POINT('Ctrl Pts',(0.255805906261685,3.4025332463843,2.63597166849728));
#38697=CARTESIAN_POINT('Ctrl Pts',(-2.71474477914914,2.06708263328288,2.79434057628146));
#38698=CARTESIAN_POINT('Ctrl Pts',(-3.2118999633853,-1.1516806498418,2.95270948406563));
#38699=CARTESIAN_POINT('Ctrl Pts',(-0.782703123250905,-3.32115121709356,
3.11107839184981));
#38700=CARTESIAN_POINT('Ctrl Pts',(2.35961209115783,-2.46473131674929,3.26944729963398));
#38701=CARTESIAN_POINT('Ctrl Pts',(3.352092094979,0.637297610789994,3.42781620741816));
#38702=CARTESIAN_POINT('Ctrl Pts',(1.29049145719765,3.15868666457495,3.58618511520233));
#38703=CARTESIAN_POINT('Ctrl Pts',(-1.94687191855818,2.80220616530042,3.74455402298651));
#38704=CARTESIAN_POINT('Ctrl Pts',(-3.41044636742465,-0.107355625286608,
3.90292293077069));
#38705=CARTESIAN_POINT('Ctrl Pts',(-1.76677377870039,-2.91910603937516,
4.06129183855486));
#38706=CARTESIAN_POINT('Ctrl Pts',(1.48660088384143,-3.07126805543518,4.21966074633904));
#38707=CARTESIAN_POINT('Ctrl Pts',(3.3855381223732,-0.425207334521279,4.3780296541232));
#38708=CARTESIAN_POINT('Ctrl Pts',(2.19992214753625,2.60825846113332,4.5363985619074));
#38709=CARTESIAN_POINT('Ctrl Pts',(-0.99003602760054,3.26534811614501,4.69476746969156));
#38710=CARTESIAN_POINT('Ctrl Pts',(-3.27797546895602,0.947389297148782,
4.85313637747574));
#38711=CARTESIAN_POINT('Ctrl Pts',(-2.5793616946409,-2.23373295262659,5.01150528525992));
#38712=CARTESIAN_POINT('Ctrl Pts',(0.46930046669552,-3.37970808316707,5.16987419304408));
#38713=CARTESIAN_POINT('Ctrl Pts',(3.09038443801754,-1.44644173083616,5.32824310082827));
#38714=CARTESIAN_POINT('Ctrl Pts',(2.89582879628167,1.80467316655209,5.48661200861244));
#38715=CARTESIAN_POINT('Ctrl Pts',(0.0628925792552412,3.41155597622644,
5.64498091639662));
#38716=CARTESIAN_POINT('Ctrl Pts',(-2.82734487037505,1.91018078710171,5.8033498241808));
#38717=CARTESIAN_POINT('Ctrl Pts',(-3.14159723579638,-1.33155415341836,
5.96171873196497));
#38718=CARTESIAN_POINT('Ctrl Pts',(-0.593550167993543,-3.36011426197451,
6.12008763974915));
#38719=CARTESIAN_POINT('Ctrl Pts',(2.4952786047586,-2.32728475698253,6.27845654753331));
#38720=CARTESIAN_POINT('Ctrl Pts',(3.31066683116828,0.825926624132867,6.43682545531751));
#38721=CARTESIAN_POINT('Ctrl Pts',(1.10971684385883,3.22663883660774,6.59519436310167));
#38722=CARTESIAN_POINT('Ctrl Pts',(-2.10229269526844,2.68757047886569,6.75356327088585));
#38723=CARTESIAN_POINT('Ctrl Pts',(-3.39890992325729,-0.300134951367665,
6.91193217867001));
#38724=CARTESIAN_POINT('Ctrl Pts',(-1.59879093182649,-3.0143883644545,7.07030108645421));
#38725=CARTESIAN_POINT('Ctrl Pts',(1.65798148604228,-2.98224194984082,7.22866999423837));
#38726=CARTESIAN_POINT('Ctrl Pts',(3.40417214832457,-0.232984205517543,
7.38703890202256));
#38727=CARTESIAN_POINT('Ctrl Pts',(2.04883219435749,2.72854472105802,7.54540780980672));
#38728=CARTESIAN_POINT('Ctrl Pts',(-1.17319237527587,3.20410507100562,7.7037767175909));
#38729=CARTESIAN_POINT('Ctrl Pts',(-3.32632503459287,0.760415294224224,
7.86214562537508));
#38730=CARTESIAN_POINT('Ctrl Pts',(-2.44885333993672,-2.3760864830494,8.02051453315925));
#38731=CARTESIAN_POINT('Ctrl Pts',(0.659760987225929,-3.34774328394278,
8.17888344094343));
#38732=CARTESIAN_POINT('Ctrl Pts',(3.16726913875196,-1.26928163074977,8.3372523487276));
#38733=CARTESIAN_POINT('Ctrl Pts',(2.78908826642068,1.9656185534238,8.49562125651178));
#38734=CARTESIAN_POINT('Ctrl Pts',(-0.130222217696887,3.40964981038632,
8.65399016429595));
#38735=CARTESIAN_POINT('Ctrl Pts',(-2.93088764583465,1.74715977029668,8.81235907208013));
#38736=CARTESIAN_POINT('Ctrl Pts',(-3.06123049031075,-1.50716208174212,
8.97072797986429));
#38737=CARTESIAN_POINT('Ctrl Pts',(-0.402495792463442,-3.38831326658245,
9.12909688764848));
#38738=CARTESIAN_POINT('Ctrl Pts',(2.62295156527424,-2.182382812816,9.28746579543266));
#38739=CARTESIAN_POINT('Ctrl Pts',(3.25863594094856,1.0119098081389,9.44583470321683));
#38740=CARTESIAN_POINT('Ctrl Pts',(0.925387284538464,3.28425456215925,9.604203611001));
#38741=CARTESIAN_POINT('Ctrl Pts',(-2.25097883768382,2.56432523829347,9.76257251878518));
#38742=CARTESIAN_POINT('Ctrl Pts',(-3.37648516862269,-0.49195280415944,
9.92094142656936));
#38743=CARTESIAN_POINT('Ctrl Pts',(-1.42568640407767,-3.10001418265748,
10.0793103343535));
#38744=CARTESIAN_POINT('Ctrl Pts',(1.82405079211913,-2.88366231782067,10.2376792421377));
#38745=CARTESIAN_POINT('Ctrl Pts',(3.41190100644405,-0.0400147182346128,
10.3960481499219));
#38746=CARTESIAN_POINT('Ctrl Pts',(1.89117886601706,2.84009016620598,10.554417057706));
#38747=CARTESIAN_POINT('Ctrl Pts',(-1.35259043483117,3.13259776719778,10.7127859654902));
#38748=CARTESIAN_POINT('Ctrl Pts',(-3.36401881339682,0.571005322708608,
10.8711548732744));
#38749=CARTESIAN_POINT('Ctrl Pts',(-2.31050015380398,-2.51082828857755,
11.0295237810586));
#38750=CARTESIAN_POINT('Ctrl Pts',(0.848107982359261,-3.30505408514111,
11.1878926888427));
#38751=CARTESIAN_POINT('Ctrl Pts',(3.23400758365375,-1.08805542336746,11.3462615966269));
#38752=CARTESIAN_POINT('Ctrl Pts',(2.67341297230351,2.12026713764294,11.5046305044111));
#38753=CARTESIAN_POINT('Ctrl Pts',(-0.32291985151006,3.39682092918513,11.6629994121952));
#38754=CARTESIAN_POINT('Ctrl Pts',(-3.02504140679361,1.5785417772848,11.8213683199794));
#38755=CARTESIAN_POINT('Ctrl Pts',(-2.97105718076111,-1.67794185956998,
11.9797372277636));
#38756=CARTESIAN_POINT('Ctrl Pts',(-0.210152033207837,-3.40565790683504,
12.1381061355478));
#38757=CARTESIAN_POINT('Ctrl Pts',(2.74222197569018,-2.03048966791049,12.296475043332));
#38758=CARTESIAN_POINT('Ctrl Pts',(3.19616610396629,1.19465136810128,12.4548439511161));
#38759=CARTESIAN_POINT('Ctrl Pts',(0.738093273596913,3.33134927243006,12.6132128589003));
#38760=CARTESIAN_POINT('Ctrl Pts',(-2.39245403396228,2.43286525537836,12.7715817666845));
#38761=CARTESIAN_POINT('Ctrl Pts',(-3.34324394060518,-0.682194700254892,
12.9299506744687));
#38762=CARTESIAN_POINT('Ctrl Pts',(-1.24801473082944,-3.17570919435036,
13.0883195822528));
#38763=CARTESIAN_POINT('Ctrl Pts',(1.9842768038067,-2.77584495628384,13.246688490037));
#38764=CARTESIAN_POINT('Ctrl Pts',(3.40869993755978,0.153082955050945,13.4050573978212));
#38765=CARTESIAN_POINT('Ctrl Pts',(1.7274672004286,2.94253746397368,13.5634263056053));
#38766=CARTESIAN_POINT('Ctrl Pts',(-1.52765550972892,3.05105527630366,13.7217952133896));
#38767=CARTESIAN_POINT('Ctrl Pts',(-3.39093605442697,0.379766152017132,
13.8801641211737));
#38768=CARTESIAN_POINT('Ctrl Pts',(-2.16474534670984,-2.63752672769918,
14.0385330289579));
#38769=CARTESIAN_POINT('Ctrl Pts',(1.03373808790759,-3.25177724039764,14.1969019367421));
#38770=CARTESIAN_POINT('Ctrl Pts',(3.29038597801295,-0.903343661620412,
14.3552708445262));
#38771=CARTESIAN_POINT('Ctrl Pts',(2.54917347644763,2.26812350685512,14.5136397523104));
#38772=CARTESIAN_POINT('Ctrl Pts',(-0.514583020900911,3.37311042967397,
14.6720086600946));
#38773=CARTESIAN_POINT('Ctrl Pts',(-3.10950453426685,1.40486697078187,14.8303775678788));
#38774=CARTESIAN_POINT('Ctrl Pts',(-2.87136617497321,-1.84334639842336,
14.9887464756629));
#38775=CARTESIAN_POINT('Ctrl Pts',(-0.0171350575310117,-3.41209262036092,
15.1471153834471));
#38776=CARTESIAN_POINT('Ctrl Pts',(2.85270775588288,-1.8720919062881,15.3054842912313));
#38777=CARTESIAN_POINT('Ctrl Pts',(3.12345744205154,1.37356589417187,15.4638531990155));
#38778=CARTESIAN_POINT('Ctrl Pts',(0.548434799162462,3.36777210564648,15.6222221067996));
#38779=CARTESIAN_POINT('Ctrl Pts',(-2.52626506690267,2.29361164927632,15.7805910145838));
#38780=CARTESIAN_POINT('Ctrl Pts',(-3.29929273696804,-0.870251187763856,
15.938959922368));
#38781=CARTESIAN_POINT('Ctrl Pts',(-1.06634505824692,-3.24123094602799,
16.0973288301521));
#38782=CARTESIAN_POINT('Ctrl Pts',(2.13814620358477,-2.65913519147203,16.2556977379364));
#38783=CARTESIAN_POINT('Ctrl Pts',(3.39457926894347,0.345690110051812,16.4140666457205));
#38784=CARTESIAN_POINT('Ctrl Pts',(1.55822150430069,3.03555865928581,16.5724355535047));
#38785=CARTESIAN_POINT('Ctrl Pts',(-1.69782651872419,2.95973837446756,16.7308044612889));
#38786=CARTESIAN_POINT('Ctrl Pts',(-3.40699103573678,0.187311257162456,
16.8891733690731));
#38787=CARTESIAN_POINT('Ctrl Pts',(-2.01205487238326,-2.75577754091925,
17.0475422768572));
#38788=CARTESIAN_POINT('Ctrl Pts',(1.21605479522199,-3.18808033565051,17.2059111846414));
#38789=CARTESIAN_POINT('Ctrl Pts',(3.33622724440086,-0.715743955828957,
17.3642800924256));
#38790=CARTESIAN_POINT('Ctrl Pts',(2.4167610366335,2.40872525887147,17.5226490002097));
#38791=CARTESIAN_POINT('Ctrl Pts',(-0.704584866714741,3.33857277996247,
17.6810179079939));
#38792=CARTESIAN_POINT('Ctrl Pts',(-3.18403103516454,1.22673275007632,17.8393868157781));
#38793=CARTESIAN_POINT('Ctrl Pts',(-2.76242988356763,-2.00292420194302,
17.9977557235623));
#38794=CARTESIAN_POINT('Ctrl Pts',(0.175847150396599,-3.40744711403038,
18.1561246313465));
#38795=CARTESIAN_POINT('Ctrl Pts',(2.95422621652823,-1.70798285735531,18.3144935391306));
#38796=CARTESIAN_POINT('Ctrl Pts',(3.04041566712921,1.54862671268017,18.4728624469148));
#38797=CARTESIAN_POINT('Ctrl Pts',(0.357645745016943,3.39235871404377,18.631231354699));
#38798=CARTESIAN_POINT('Ctrl Pts',(-2.65319198947773,2.14904689640439,18.7896002624832));
#38799=CARTESIAN_POINT('Ctrl Pts',(-3.24244227426787,-1.06021153090294,
18.9479933412587));
#38800=CARTESIAN_POINT('Ctrl Pts',(-1.67134529740578,-2.5444535668589,19.0535967841062));
#38801=CARTESIAN_POINT('Ctrl Pts',(-0.74495813079252,-2.79162859999982,
19.1064105910255));
#38802=CARTESIAN_POINT('Ctrl Pts',(-2.33803595403645,2.00106467658089,-0.323366414141818));
#38803=CARTESIAN_POINT('Ctrl Pts',(-3.00214223718147,1.22518857689341,-0.270549577477338));
#38804=CARTESIAN_POINT('Ctrl Pts',(-3.48578596895374,-1.02558263320169,
-0.164943104884798));
#38805=CARTESIAN_POINT('Ctrl Pts',(-1.0322971287473,-3.48708213552881,-0.00654699636420169));
#38806=CARTESIAN_POINT('Ctrl Pts',(2.36061725640788,-2.76190313005438,0.151821911419974));
#38807=CARTESIAN_POINT('Ctrl Pts',(3.60308039602196,0.475030646428534,0.31019081920415));
#38808=CARTESIAN_POINT('Ctrl Pts',(1.56263746620872,3.28155448272582,0.468559726988325));
#38809=CARTESIAN_POINT('Ctrl Pts',(-1.90144133534228,3.09701595734625,0.626928634772501));
#38810=CARTESIAN_POINT('Ctrl Pts',(-3.63316376413971,0.0914492119455178,
0.785297542556676));
#38811=CARTESIAN_POINT('Ctrl Pts',(-2.05470062781962,-2.99777869887408,
0.943666450340852));
#38812=CARTESIAN_POINT('Ctrl Pts',(1.39578262972872,-3.35556068325843,1.10203535812503));
#38813=CARTESIAN_POINT('Ctrl Pts',(3.57457855856896,-0.656195592380133,
1.2604042659092));
#38814=CARTESIAN_POINT('Ctrl Pts',(2.49658405047906,2.64107636274744,1.41877317369338));
#38815=CARTESIAN_POINT('Ctrl Pts',(-0.856038782740064,3.53204617508454,
1.57714208147756));
#38816=CARTESIAN_POINT('Ctrl Pts',(-3.42872819598997,1.20499320918028,1.73551098926173));
#38817=CARTESIAN_POINT('Ctrl Pts',(-2.87751361354832,-2.21993235784546,
1.89387989704591));
#38818=CARTESIAN_POINT('Ctrl Pts',(0.29539440741815,-3.62228079274625,2.05224880483008));
#38819=CARTESIAN_POINT('Ctrl Pts',(3.19916962696489,-1.72438243946365,2.21061771261426));
#38820=CARTESIAN_POINT('Ctrl Pts',(3.18819132411539,1.74459638294176,2.36898662039843));
#38821=CARTESIAN_POINT('Ctrl Pts',(0.272461892802362,3.62407835761407,2.52735552818261));
#38822=CARTESIAN_POINT('Ctrl Pts',(-2.89150673575782,2.20167413283645,2.68572443596679));
#38823=CARTESIAN_POINT('Ctrl Pts',(-3.42103259578594,-1.22666866588587,
2.84409334375096));
#38824=CARTESIAN_POINT('Ctrl Pts',(-0.833666343282555,-3.53739739678445,
3.00246225153514));
#38825=CARTESIAN_POINT('Ctrl Pts',(2.51325071430724,-2.62521444334356,3.16083115931931));
#38826=CARTESIAN_POINT('Ctrl Pts',(3.57035289134998,0.678793214166964,3.31920006710349));
#38827=CARTESIAN_POINT('Ctrl Pts',(1.37451769668545,3.3643544825711,3.47756897488767));
#38828=CARTESIAN_POINT('Ctrl Pts',(-2.07363628043631,2.98466289139998,3.63593788267183));
#38829=CARTESIAN_POINT('Ctrl Pts',(-3.63250671631828,-0.114345744772007,
3.79430679045602));
#38830=CARTESIAN_POINT('Ctrl Pts',(-1.88181162402811,-3.10917432831019,
3.95267569824018));
#38831=CARTESIAN_POINT('Ctrl Pts',(1.58339616380376,-3.27124388922926,4.11104460602437));
#38832=CARTESIAN_POINT('Ctrl Pts',(3.60597665025262,-0.452893355318378,
4.26941351380853));
#38833=CARTESIAN_POINT('Ctrl Pts',(2.34316306880883,2.77808690042977,4.42778242159272));
#38834=CARTESIAN_POINT('Ctrl Pts',(-1.05449906909743,3.47796085471677,4.58615132937689));
#38835=CARTESIAN_POINT('Ctrl Pts',(-3.49141039737296,1.00907553267278,4.74452023716107));
#38836=CARTESIAN_POINT('Ctrl Pts',(-2.7473086130577,-2.37917535674507,4.90288914494524));
#38837=CARTESIAN_POINT('Ctrl Pts',(0.499857471305165,-3.59976700661918,
5.06125805272942));
#38838=CARTESIAN_POINT('Ctrl Pts',(3.2916049741551,-1.54062217550514,5.2196269605136));
#38839=CARTESIAN_POINT('Ctrl Pts',(3.08438146169832,1.92217870976522,5.37799586829777));
#38840=CARTESIAN_POINT('Ctrl Pts',(0.0669876291659018,3.63368857376175,
5.53636477608195));
#38841=CARTESIAN_POINT('Ctrl Pts',(-3.01143842315892,2.03455612285989,5.69473368386612));
#38842=CARTESIAN_POINT('Ctrl Pts',(-3.34615233008773,-1.41825405953713,
5.85310259165031));
#38843=CARTESIAN_POINT('Ctrl Pts',(-0.632197296020375,-3.57889739618926,
6.01147149943446));
#38844=CARTESIAN_POINT('Ctrl Pts',(2.6577507206822,-2.47881848876807,6.16984040721865));
#38845=CARTESIAN_POINT('Ctrl Pts',(3.52623035347487,0.879704204706274,6.32820931500282));
#38846=CARTESIAN_POINT('Ctrl Pts',(1.18197252038088,3.43673114377745,6.48657822278701));
#38847=CARTESIAN_POINT('Ctrl Pts',(-2.23917678582234,2.86256306749383,6.64494713057117));
#38848=CARTESIAN_POINT('Ctrl Pts',(-3.62021911334622,-0.319677282439768,
6.80331603835535));
#38849=CARTESIAN_POINT('Ctrl Pts',(-1.70289110930486,-3.21066065839974,
6.96168494613953));
#38850=CARTESIAN_POINT('Ctrl Pts',(1.76593566786621,-3.17642113242298,7.12005385392371));
#38851=CARTESIAN_POINT('Ctrl Pts',(3.62582397143231,-0.248154229728482,
7.27842276170788));
#38852=CARTESIAN_POINT('Ctrl Pts',(2.18223537472976,2.90620521691491,7.43679166949206));
#38853=CARTESIAN_POINT('Ctrl Pts',(-1.2495810587812,3.41273016382494,7.59516057727622));
#38854=CARTESIAN_POINT('Ctrl Pts',(-3.54290809092547,0.809927313282007,
7.75352948506041));
#38855=CARTESIAN_POINT('Ctrl Pts',(-2.60830262266105,-2.53079778373636,
7.91189839284458));
#38856=CARTESIAN_POINT('Ctrl Pts',(0.702719221787002,-3.56572092133924,
8.07026730062876));
#38857=CARTESIAN_POINT('Ctrl Pts',(3.37349577720877,-1.35192685996691,8.22863620841293));
#38858=CARTESIAN_POINT('Ctrl Pts',(2.97069086233078,2.09360354270093,8.38700511619711));
#38859=CARTESIAN_POINT('Ctrl Pts',(-0.138701222489833,3.63165829400636,
8.54537402398129));
#38860=CARTESIAN_POINT('Ctrl Pts',(-3.12172305653588,1.86092051196111,8.70374293176545));
#38861=CARTESIAN_POINT('Ctrl Pts',(-3.26055276003331,-1.60529613859391,
8.86211183954965));
#38862=CARTESIAN_POINT('Ctrl Pts',(-0.428703023562676,-3.60893248913491,
9.0204807473338));
#38863=CARTESIAN_POINT('Ctrl Pts',(2.79373669923185,-2.3244817161919,9.178849655118));
#38864=CARTESIAN_POINT('Ctrl Pts',(3.47081163761864,1.07779709116158,9.33721856290215));
#38865=CARTESIAN_POINT('Ctrl Pts',(0.985640929113881,3.49809833372375,9.49558747068635));
#38866=CARTESIAN_POINT('Ctrl Pts',(-2.3975441526592,2.73129310576418,9.6539563784705));
#38867=CARTESIAN_POINT('Ctrl Pts',(-3.59633424226306,-0.523984743548459,
9.8123252862547));
#38868=CARTESIAN_POINT('Ctrl Pts',(-1.51851543177513,-3.30186172893509,
9.97069419403885));
#38869=CARTESIAN_POINT('Ctrl Pts',(1.94281804768031,-3.07142280175702,10.1290631018231));
#38870=CARTESIAN_POINT('Ctrl Pts',(3.63405606952266,-0.0426201491180682,
10.2874320096072));
#38871=CARTESIAN_POINT('Ctrl Pts',(2.01431695222748,3.02501358831897,10.4458009173914));
#38872=CARTESIAN_POINT('Ctrl Pts',(-1.4406600513886,3.33656688976533,10.6041698251756));
#38873=CARTESIAN_POINT('Ctrl Pts',(-3.5830561800368,0.608184514966817,10.7625387329598));
#38874=CARTESIAN_POINT('Ctrl Pts',(-2.46094100963244,-2.67431287261882,
10.9209076407439));
#38875=CARTESIAN_POINT('Ctrl Pts',(0.903329831399618,-3.52025215137339,
11.0792765485281));
#38876=CARTESIAN_POINT('Ctrl Pts',(3.44457968330915,-1.15890068551155,11.2376454563123));
#38877=CARTESIAN_POINT('Ctrl Pts',(2.84748374000033,2.25832157674212,11.3960143640965));
#38878=CARTESIAN_POINT('Ctrl Pts',(-0.343945748757976,3.61799410108097,
11.5543832718806));
#38879=CARTESIAN_POINT('Ctrl Pts',(-3.22200733964816,1.68132349558278,11.7127521796648));
#38880=CARTESIAN_POINT('Ctrl Pts',(-3.16450810274141,-1.78719569751867,
11.871121087449));
#38881=CARTESIAN_POINT('Ctrl Pts',(-0.223835413266404,-3.62740647037429,
12.0294899952332));
#38882=CARTESIAN_POINT('Ctrl Pts',(2.92077302240413,-2.16269853311588,12.1878589030173));
#38883=CARTESIAN_POINT('Ctrl Pts',(3.40427427624188,1.27243728555206,12.3462278108015));
#38884=CARTESIAN_POINT('Ctrl Pts',(0.786151865403689,3.54825946600126,12.5045967185857));
#38885=CARTESIAN_POINT('Ctrl Pts',(-2.54823105557683,2.59127352491771,12.6629656263699));
#38886=CARTESIAN_POINT('Ctrl Pts',(-3.56092861759596,-0.726613634561833,
12.8213345341541));
#38887=CARTESIAN_POINT('Ctrl Pts',(-1.32927523361859,-3.38248538013586,
12.9797034419382));
#38888=CARTESIAN_POINT('Ctrl Pts',(2.11347666560882,-2.95658525625003,13.1380723497224));
#38889=CARTESIAN_POINT('Ctrl Pts',(3.6306465732372,0.163050463918102,13.2964412575066));
#38890=CARTESIAN_POINT('Ctrl Pts',(1.83994572315028,3.13413141546453,13.4548101652907));
#38891=CARTESIAN_POINT('Ctrl Pts',(-1.62712393084818,3.24971501938629,13.6131790730749));
#38892=CARTESIAN_POINT('Ctrl Pts',(-3.61172605145325,0.4044934149996,13.7715479808591));
#38893=CARTESIAN_POINT('Ctrl Pts',(-2.30569584267649,-2.80926087691889,
13.9299168886433));
#38894=CARTESIAN_POINT('Ctrl Pts',(1.10104664981842,-3.46350635463446,14.0882857964275));
#38895=CARTESIAN_POINT('Ctrl Pts',(3.50462897718492,-0.962162005924634,
14.2466547042116));
#38896=CARTESIAN_POINT('Ctrl Pts',(2.7151547852221,2.41580514233745,14.4050236119958));
#38897=CARTESIAN_POINT('Ctrl Pts',(-0.548088454748935,3.59273976794022,
14.56339251978));
#38898=CARTESIAN_POINT('Ctrl Pts',(-3.31197001455146,1.4963404074149,14.7217614275642));
#38899=CARTESIAN_POINT('Ctrl Pts',(-3.05832603474587,-1.96337002590963,
14.8801303353483));
#38900=CARTESIAN_POINT('Ctrl Pts',(-0.0182507522066404,-3.6342601597692,
15.0384992431325));
#38901=CARTESIAN_POINT('Ctrl Pts',(3.03845273214569,-1.99398720593042,15.1968681509167));
#38902=CARTESIAN_POINT('Ctrl Pts',(3.32683142146999,1.46300126093254,15.3552370587008));
#38903=CARTESIAN_POINT('Ctrl Pts',(0.584144383693881,3.5870538559526,15.513605966485));
#38904=CARTESIAN_POINT('Ctrl Pts',(-2.69075476758011,2.44295286394241,15.6719748742692));
#38905=CARTESIAN_POINT('Ctrl Pts',(-3.51411567137077,-0.926914821071728,
15.8303437820534));
#38906=CARTESIAN_POINT('Ctrl Pts',(-1.13577671913948,-3.45227337190941,
15.9887126898375));
#38907=CARTESIAN_POINT('Ctrl Pts',(2.2773647810967,-2.83227630696169,16.1470815976217));
#38908=CARTESIAN_POINT('Ctrl Pts',(3.61560648227504,0.36819862013436,16.3054505054059));
#38909=CARTESIAN_POINT('Ctrl Pts',(1.6596801327675,3.23320938952646,16.4638194131901));
#38910=CARTESIAN_POINT('Ctrl Pts',(-1.80837508289745,3.1524523084399,16.6221883209743));
#38911=CARTESIAN_POINT('Ctrl Pts',(-3.62882640171686,0.199507432863826,
16.7805572287584));
#38912=CARTESIAN_POINT('Ctrl Pts',(-2.14306341461461,-2.93521121507253,
16.9389261365426));
#38913=CARTESIAN_POINT('Ctrl Pts',(1.2952343286344,-3.39566202888499,17.0972950443268));
#38914=CARTESIAN_POINT('Ctrl Pts',(3.55345505157481,-0.762347343018389,
17.255663952111));
#38915=CARTESIAN_POINT('Ctrl Pts',(2.57412073128032,2.56556172945283,17.4140328598952));
#38916=CARTESIAN_POINT('Ctrl Pts',(-0.750461665371445,3.55595330921119,
17.5724017676793));
#38917=CARTESIAN_POINT('Ctrl Pts',(-3.39134907109971,1.3066075444971,17.7307706754635));
#38918=CARTESIAN_POINT('Ctrl Pts',(-2.94229670381685,-2.13333822966068,
17.8891395832477));
#38919=CARTESIAN_POINT('Ctrl Pts',(0.187296877312696,-3.62931217609541,
18.0475084910319));
#38920=CARTESIAN_POINT('Ctrl Pts',(3.14658124389912,-1.81919271915853,18.205877398816));
#38921=CARTESIAN_POINT('Ctrl Pts',(3.23838264596023,1.64946060686142,18.3642463066002));
#38922=CARTESIAN_POINT('Ctrl Pts',(0.38093270817736,3.61324134301813,18.5226152143844));
#38923=CARTESIAN_POINT('Ctrl Pts',(-2.82594613230569,2.28897523779762,18.6809841221686));
#38924=CARTESIAN_POINT('Ctrl Pts',(-3.45356357192809,-1.12924382670507,
18.839377200944));
#38925=CARTESIAN_POINT('Ctrl Pts',(-1.78016962122703,-2.71012755375903,
18.9449806437914));
#38926=CARTESIAN_POINT('Ctrl Pts',(-0.793463705902866,-2.97339660163694,
18.9977944507108));
#38927=CARTESIAN_POINT('Ctrl Pts',(-1.91346599666507,1.63598720337494,-1.49186218934005E-15));
#38928=CARTESIAN_POINT('Ctrl Pts',(-1.97562728140449,1.57757085957046,-2.50614906192051E-15));
#38929=CARTESIAN_POINT('Ctrl Pts',(-2.03436145510481,1.51595110656798,-4.44124286950301E-15));
#38930=CARTESIAN_POINT('Ctrl Pts',(-2.08967050234655,1.45152218121991,-3.68455266297474E-15));
#38931=CARTESIAN_POINT('Ctrl Pts',(-2.14612535197374,1.38575852276691,-2.91218658627838E-15));
#38932=CARTESIAN_POINT('Ctrl Pts',(-2.1990121164881,1.31706760569438,-1.5430458858727E-15));
#38933=CARTESIAN_POINT('Ctrl Pts',(-2.24830698708946,1.24581947769238,-1.76247905159244E-15));
#38934=CARTESIAN_POINT('Ctrl Pts',(-2.29883933734524,1.1727827638245,-1.98742078391902E-15));
#38935=CARTESIAN_POINT('Ctrl Pts',(-2.34559771595042,1.09705825975981,-6.50009313603642E-16));
#38936=CARTESIAN_POINT('Ctrl Pts',(-2.38852219321958,1.0190015549115,1.2490009027033E-16));
#38937=CARTESIAN_POINT('Ctrl Pts',(-2.41751206249941,0.966284461683361,
6.48250023716466E-16));
#38938=CARTESIAN_POINT('Ctrl Pts',(-2.44475247983232,0.912502700494791,
2.25064873853325E-15));
#38939=CARTESIAN_POINT('Ctrl Pts',(-2.47021462141466,0.857757311203253,
1.31838984174237E-15));
#38940=CARTESIAN_POINT('Ctrl Pts',(-2.47883400081736,0.83922504127118,1.06850379779826E-15));
#38941=CARTESIAN_POINT('Ctrl Pts',(-2.48725198934881,0.820576366164846,
-8.41426332219623E-16));
#38942=CARTESIAN_POINT('Ctrl Pts',(-2.49545335573811,0.801847661549147,
-6.52256026967279E-16));
#38943=CARTESIAN_POINT('Ctrl Pts',(-2.53213167303446,0.718088768477345,
-9.03468916911122E-16));
#38944=CARTESIAN_POINT('Ctrl Pts',(-2.56452720083354,0.632638163527894,
-2.74682372953375E-16));
#38945=CARTESIAN_POINT('Ctrl Pts',(-2.59261423848372,0.545897077960933,
1.01307850997046E-15));
#38946=CARTESIAN_POINT('Ctrl Pts',(-2.62108392241438,0.457974267422819,
2.31838331896207E-15));
#38947=CARTESIAN_POINT('Ctrl Pts',(-2.64512739967565,0.368724800334353,
-2.85563347547353E-15));
#38948=CARTESIAN_POINT('Ctrl Pts',(-2.66467879117549,0.278529425245449,
-1.1518563880486E-15));
#38949=CARTESIAN_POINT('Ctrl Pts',(-2.68425447613445,0.188221978457852,
5.5403771693064E-16));
#38950=CARTESIAN_POINT('Ctrl Pts',(-2.69932732669291,0.0969653795285389,
-3.58400398648576E-16));
#38951=CARTESIAN_POINT('Ctrl Pts',(-2.70978561266556,0.00511753876573948,
1.80411241501588E-16));
#38952=CARTESIAN_POINT('Ctrl Pts',(-2.71365156263523,-0.0288344069106642,
3.79585260011577E-16));
#38953=CARTESIAN_POINT('Ctrl Pts',(-2.71688647879056,-0.0628673128703889,
-1.31650542657094E-15));
#38954=CARTESIAN_POINT('Ctrl Pts',(-2.71948296230813,-0.0969635581463529,
-1.37390099297363E-15));
#38955=CARTESIAN_POINT('Ctrl Pts',(-2.72117333325281,-0.119161004017789,
-1.37858239915481E-15));
#38956=CARTESIAN_POINT('Ctrl Pts',(-2.72259309670265,-0.141385298884962,
1.35912043257924E-15));
#38957=CARTESIAN_POINT('Ctrl Pts',(-2.72373998089586,-0.163631606082652,
4.02455846426619E-16));
#38958=CARTESIAN_POINT('Ctrl Pts',(-2.72438165410587,-0.17607825015966,
-5.8898284204301E-16));
#38959=CARTESIAN_POINT('Ctrl Pts',(-2.72493780860265,-0.18853085131645,
1.50166758541897E-16));
#38960=CARTESIAN_POINT('Ctrl Pts',(-2.72540781340729,-0.200978281065814,
-1.38777878078145E-16));
#38961=CARTESIAN_POINT('Ctrl Pts',(-2.72916559147235,-0.300497856221906,
-8.51642209848428E-16));
#38962=CARTESIAN_POINT('Ctrl Pts',(-2.72743044903818,-0.399859077131394,
-9.16883136981344E-17));
#38963=CARTESIAN_POINT('Ctrl Pts',(-2.72013295703714,-0.498607340903291,
-1.80411241501588E-15));
#38964=CARTESIAN_POINT('Ctrl Pts',(-2.71283546503611,-0.597355604675174,
-4.27462052636193E-15));
#38965=CARTESIAN_POINT('Ctrl Pts',(-2.69997611686452,-0.695492103877208,
-1.71117497003209E-15));
#38966=CARTESIAN_POINT('Ctrl Pts',(-2.68142706905932,-0.792583196929577,
-2.19269047363468E-15));
#38967=CARTESIAN_POINT('Ctrl Pts',(-2.664117508035,-0.88318645687896,-2.61840637124098E-15));
#38968=CARTESIAN_POINT('Ctrl Pts',(-2.64185312691352,-0.972880370486868,
-5.09040680058174E-15));
#38969=CARTESIAN_POINT('Ctrl Pts',(-2.61490988468309,-1.06142534465363,
-4.91273688396632E-15));
#38970=CARTESIAN_POINT('Ctrl Pts',(-2.60515225760836,-1.09349234052115,
-4.84839285387875E-15));
#38971=CARTESIAN_POINT('Ctrl Pts',(-2.59478046819329,-1.12540860314951,
-4.2189522678695E-15));
#38972=CARTESIAN_POINT('Ctrl Pts',(-2.58380597441444,-1.15716250955434,
-3.83026943495679E-15));
#38973=CARTESIAN_POINT('Ctrl Pts',(-2.57707836097892,-1.17662837391802,
-3.42200387609689E-15));
#38974=CARTESIAN_POINT('Ctrl Pts',(-2.57012423657022,-1.19603322188682,
-6.35130850184293E-15));
#38975=CARTESIAN_POINT('Ctrl Pts',(-2.56294608765656,-1.21537433488221,
-5.82867087928207E-15));
#38976=CARTESIAN_POINT('Ctrl Pts',(-2.55803440850288,-1.22860857432904,
-5.55861431346926E-15));
#38977=CARTESIAN_POINT('Ctrl Pts',(-2.55301817112519,-1.24181188707138,
-4.25409719012689E-15));
#38978=CARTESIAN_POINT('Ctrl Pts',(-2.54790299736969,-1.25497158263782,
-4.30211422042248E-15));
#38979=CARTESIAN_POINT('Ctrl Pts',(-2.51363258640273,-1.3431383188659,-3.82292319133049E-15));
#38980=CARTESIAN_POINT('Ctrl Pts',(-2.47487338179404,-1.42948978193878,
-3.5983761671373E-15));
#38981=CARTESIAN_POINT('Ctrl Pts',(-2.43197011073125,-1.5137843727111,-4.69069227904129E-15));
#38982=CARTESIAN_POINT('Ctrl Pts',(-2.38822425227513,-1.59973444470317,
-5.80446064301425E-15));
#38983=CARTESIAN_POINT('Ctrl Pts',(-2.34016967457277,-1.68354677501953,
-4.78147958264788E-15));
#38984=CARTESIAN_POINT('Ctrl Pts',(-2.2881164923778,-1.76496219714289,-5.80091530366644E-15));
#38985=CARTESIAN_POINT('Ctrl Pts',(-2.23518331119972,-1.84775400944371,
-6.8375853677168E-15));
#38986=CARTESIAN_POINT('Ctrl Pts',(-2.17811482141291,-1.92806801277158,
-4.24679705205495E-15));
#38987=CARTESIAN_POINT('Ctrl Pts',(-2.11718543714367,-2.00561675751096,
-6.30051566474776E-15));
#38988=CARTESIAN_POINT('Ctrl Pts',(-2.07494196997557,-2.05938273416762,
-7.72439670061111E-15));
#38989=CARTESIAN_POINT('Ctrl Pts',(-2.03084151659921,-2.11181917678613,
-7.36061663108968E-15));
#38990=CARTESIAN_POINT('Ctrl Pts',(-1.98496281732071,-2.16282291589316,
-6.93889390390723E-15));
#38991=CARTESIAN_POINT('Ctrl Pts',(-1.97399768439553,-2.1750129471666,-6.87133739263459E-15));
#38992=CARTESIAN_POINT('Ctrl Pts',(-1.96293062927649,-2.18712132010553,
-7.50498138722435E-15));
#38993=CARTESIAN_POINT('Ctrl Pts',(-1.95177323750925,-2.19913549001593,
-7.18869408444789E-15));
#38994=CARTESIAN_POINT('Ctrl Pts',(-1.88308475485779,-2.27309857374356,
-6.58819740314064E-15));
#38995=CARTESIAN_POINT('Ctrl Pts',(-1.81088310049948,-2.34359790276572,
-8.33506234338686E-15));
#38996=CARTESIAN_POINT('Ctrl Pts',(-1.73548098567592,-2.41034417373154,
-7.27196081129478E-15));
#38997=CARTESIAN_POINT('Ctrl Pts',(-1.67159483308639,-2.4668964662194,-6.3827680954257E-15));
#38998=CARTESIAN_POINT('Ctrl Pts',(-1.60541009649036,-2.52075457683924,
-8.56307881259928E-15));
#38999=CARTESIAN_POINT('Ctrl Pts',(-1.53709204750604,-2.57172803359375,
-7.04991620636974E-15));
#39000=CARTESIAN_POINT('Ctrl Pts',(-1.51139262450419,-2.59090288484428,
-5.70535958527313E-15));
#39001=CARTESIAN_POINT('Ctrl Pts',(-1.48539160198016,-2.60966903460802,
-8.28152629487784E-15));
#39002=CARTESIAN_POINT('Ctrl Pts',(-1.45909549992335,-2.62801676553979,
-8.38218383591993E-15));
#39003=CARTESIAN_POINT('Ctrl Pts',(-1.43771162959308,-2.64293705670128,
-8.46403808948036E-15));
#39004=CARTESIAN_POINT('Ctrl Pts',(-1.41613408952649,-2.65757933351224,
-8.74660806298987E-15));
#39005=CARTESIAN_POINT('Ctrl Pts',(-1.39438874927187,-2.67192417048441,
-8.32667268468867E-15));
#39006=CARTESIAN_POINT('Ctrl Pts',(-1.30923746902616,-2.72809626155285,
-6.6822727965235E-15));
#39007=CARTESIAN_POINT('Ctrl Pts',(-1.22144049509827,-2.77976395162219,
-5.87210663195867E-15));
#39008=CARTESIAN_POINT('Ctrl Pts',(-1.13128845941444,-2.8266186852154,-4.77395900588817E-15));
#39009=CARTESIAN_POINT('Ctrl Pts',(-1.04699210296153,-2.87043004559701,
-3.74713977742599E-15));
#39010=CARTESIAN_POINT('Ctrl Pts',(-0.960635894698547,-2.91003369441993,
-3.99091700432708E-15));
#39011=CARTESIAN_POINT('Ctrl Pts',(-0.872429377952129,-2.94514712713841,
-4.77395900588817E-15));
#39012=CARTESIAN_POINT('Ctrl Pts',(-0.847142239363335,-2.95521348359633,
-4.82011908673854E-15));
#39013=CARTESIAN_POINT('Ctrl Pts',(-0.821702883756235,-2.96491059049498,
-4.33795729134559E-15));
#39014=CARTESIAN_POINT('Ctrl Pts',(-0.796118629904262,-2.97424061993174,
1.66533453693773E-16));
#39015=CARTESIAN_POINT('Ctrl Pts',(0.794818364480303,-2.97303485125766,
0.00227809062281707));
#39016=CARTESIAN_POINT('Ctrl Pts',(1.78093556794474,-2.7094038808666,0.0550677265508756));
#39017=CARTESIAN_POINT('Ctrl Pts',(3.4534673386373,-1.12871913187498,0.160646998406993));
#39018=CARTESIAN_POINT('Ctrl Pts',(2.82594663323224,2.28897348571344,0.319015906191168));
#39019=CARTESIAN_POINT('Ctrl Pts',(-0.380932805352938,3.61324274555714,
0.477384813975344));
#39020=CARTESIAN_POINT('Ctrl Pts',(-3.23838288724328,1.6494600182536,0.635753721759519));
#39021=CARTESIAN_POINT('Ctrl Pts',(-3.14658141599552,-1.81919242326023,
0.794122629543696));
#39022=CARTESIAN_POINT('Ctrl Pts',(-0.187296929226849,-3.62931267164117,
0.952491537327871));
#39023=CARTESIAN_POINT('Ctrl Pts',(2.94229693385074,-2.13333823050325,1.11086044511205));
#39024=CARTESIAN_POINT('Ctrl Pts',(3.3913492823706,1.30660755011612,1.26922935289622));
#39025=CARTESIAN_POINT('Ctrl Pts',(0.750461729472986,3.55595359950969,1.4275982606804));
#39026=CARTESIAN_POINT('Ctrl Pts',(-2.57412091487803,2.56556187728594,1.58596716846457));
#39027=CARTESIAN_POINT('Ctrl Pts',(-3.5534552890492,-0.762347379687072,
1.74433607624876));
#39028=CARTESIAN_POINT('Ctrl Pts',(-1.29523441987398,-3.39566226908073,
1.90270498403292));
#39029=CARTESIAN_POINT('Ctrl Pts',(2.14306356247744,-2.93521141044675,2.06107389181711));
#39030=CARTESIAN_POINT('Ctrl Pts',(3.62882664822082,0.1995074437915,2.21944279960128));
#39031=CARTESIAN_POINT('Ctrl Pts',(1.80837520679842,3.15245252492811,2.37781170738546));
#39032=CARTESIAN_POINT('Ctrl Pts',(-1.65968024628328,3.23320960921406,2.53618061516963));
#39033=CARTESIAN_POINT('Ctrl Pts',(-3.61560672868174,0.368198645699416,
2.69454952295381));
#39034=CARTESIAN_POINT('Ctrl Pts',(-2.27736493651933,-2.83227650037644,
2.85291843073798));
#39035=CARTESIAN_POINT('Ctrl Pts',(1.13577679665878,-3.45227360722268,3.01128733852215));
#39036=CARTESIAN_POINT('Ctrl Pts',(3.51411591100643,-0.926914884363649,
3.16965624630634));
#39037=CARTESIAN_POINT('Ctrl Pts',(2.69075495111143,2.44295303059633,3.32802515409051));
#39038=CARTESIAN_POINT('Ctrl Pts',(-0.584144423543271,3.58705410057259,
3.48639406187469));
#39039=CARTESIAN_POINT('Ctrl Pts',(-3.3268316483593,1.46300136072356,3.64476296965886));
#39040=CARTESIAN_POINT('Ctrl Pts',(-3.03845293937564,-1.99398734192987,
3.80313187744304));
#39041=CARTESIAN_POINT('Ctrl Pts',(0.0182507534530098,-3.63426040762749,
3.96150078522721));
#39042=CARTESIAN_POINT('Ctrl Pts',(3.05832624332729,-1.9633701598163,4.11986969301138));
#39043=CARTESIAN_POINT('Ctrl Pts',(3.31197024043316,1.49634050946856,4.27823860079557));
#39044=CARTESIAN_POINT('Ctrl Pts',(0.548088492129132,3.59274001296977,4.43660750857973));
#39045=CARTESIAN_POINT('Ctrl Pts',(-2.71515497039948,2.41580530709925,4.59497641636392));
#39046=CARTESIAN_POINT('Ctrl Pts',(-3.50462921620585,-0.962162071545632,
4.75334532414809));
#39047=CARTESIAN_POINT('Ctrl Pts',(-1.1010467249114,-3.46350659085057,4.91171423193227));
#39048=CARTESIAN_POINT('Ctrl Pts',(2.3056959999283,-2.80926106851468,5.07008313971643));
#39049=CARTESIAN_POINT('Ctrl Pts',(3.61172629777829,0.404493442586659,5.22845204750063));
#39050=CARTESIAN_POINT('Ctrl Pts',(1.62712404182042,3.2497152410216,5.38682095528478));
#39051=CARTESIAN_POINT('Ctrl Pts',(-1.83994584863726,3.13413162921692,5.54518986306898));
#39052=CARTESIAN_POINT('Ctrl Pts',(-3.63064682085263,0.163050475038392,
5.70355877085314));
#39053=CARTESIAN_POINT('Ctrl Pts',(-2.11347680975103,-2.95658545789347,
5.86192767863733));
#39054=CARTESIAN_POINT('Ctrl Pts',(1.32927532427707,-3.38248561082633,6.02029658642149));
#39055=CARTESIAN_POINT('Ctrl Pts',(3.56092886045652,-0.726613684117993,
6.17866549420568));
#39056=CARTESIAN_POINT('Ctrl Pts',(2.54823122936997,2.59127370164634,6.33703440198984));
#39057=CARTESIAN_POINT('Ctrl Pts',(-0.786151919020366,3.54825970799776,
6.49540330977403));
#39058=CARTESIAN_POINT('Ctrl Pts',(-3.40427450841839,1.27243737233417,6.6537722175582));
#39059=CARTESIAN_POINT('Ctrl Pts',(-2.92077322160515,-2.16269868061508,
6.81214112534238));
#39060=CARTESIAN_POINT('Ctrl Pts',(0.223835428532286,-3.62740671776872,
6.97051003312655));
#39061=CARTESIAN_POINT('Ctrl Pts',(3.1645083185655,-1.78719581940807,7.12887894091072));
#39062=CARTESIAN_POINT('Ctrl Pts',(3.2220075593938,1.6813236102515,7.28724784869491));
#39063=CARTESIAN_POINT('Ctrl Pts',(0.343945772215585,3.61799434783347,7.44561675647908));
#39064=CARTESIAN_POINT('Ctrl Pts',(-2.8474839342029,2.25832173076298,7.60398566426325));
#39065=CARTESIAN_POINT('Ctrl Pts',(-3.44457991823455,-1.15890076455028,
7.76235457204742));
#39066=CARTESIAN_POINT('Ctrl Pts',(-0.903329893008045,-3.52025239145974,
7.9207234798316));
#39067=CARTESIAN_POINT('Ctrl Pts',(2.46094117747219,-2.6743130550109,8.07909238761578));
#39068=CARTESIAN_POINT('Ctrl Pts',(3.5830564244065,0.608184556445852,8.23746129539996));
#39069=CARTESIAN_POINT('Ctrl Pts',(1.44066014964377,3.33656711732408,8.39583020318411));
#39070=CARTESIAN_POINT('Ctrl Pts',(-2.01431708960681,3.02501379462936,8.5541991109683));
#39071=CARTESIAN_POINT('Ctrl Pts',(-3.63405631737063,-0.0426201520247982,
8.71256801875249));
#39072=CARTESIAN_POINT('Ctrl Pts',(-1.94281818018336,-3.07142301123257,
8.87093692653665));
#39073=CARTESIAN_POINT('Ctrl Pts',(1.5185155353401,-3.3018619541269,9.02930583432084));
#39074=CARTESIAN_POINT('Ctrl Pts',(3.59633448753833,-0.523984779285016,
9.18767474210499));
#39075=CARTESIAN_POINT('Ctrl Pts',(2.39754431617524,2.73129329204238,9.34604364988919));
#39076=CARTESIAN_POINT('Ctrl Pts',(-0.985640996336014,3.49809857229919,
9.50441255767334));
#39077=CARTESIAN_POINT('Ctrl Pts',(-3.47081187433309,1.07779716466894,9.66278146545754));
#39078=CARTESIAN_POINT('Ctrl Pts',(-2.79373688976881,-2.32448187472495,
9.82115037324171));
#39079=CARTESIAN_POINT('Ctrl Pts',(0.42870305280083,-3.60893273526941,9.97951928102589));
#39080=CARTESIAN_POINT('Ctrl Pts',(3.26055298240778,-1.60529624807749,10.13788818881));
#39081=CARTESIAN_POINT('Ctrl Pts',(3.121723269442,1.86092063887863,10.2962570965942));
#39082=CARTESIAN_POINT('Ctrl Pts',(0.138701231949454,3.63165854169077,10.4546260043784));
#39083=CARTESIAN_POINT('Ctrl Pts',(-2.97069106493622,2.09360368548778,10.6129949121626));
#39084=CARTESIAN_POINT('Ctrl Pts',(-3.37349600728616,-1.35192695217027,
10.7713638199467));
#39085=CARTESIAN_POINT('Ctrl Pts',(-0.702719269713518,-3.56572116452664,
10.9297327277309));
#39086=CARTESIAN_POINT('Ctrl Pts',(2.60830280055109,-2.5307979563405,11.0881016355151));
#39087=CARTESIAN_POINT('Ctrl Pts',(3.54290833255702,0.809927368520206,11.2464705432993));
#39088=CARTESIAN_POINT('Ctrl Pts',(1.24958114400447,3.41273039657815,11.4048394510835));
#39089=CARTESIAN_POINT('Ctrl Pts',(-2.1822355235614,2.90620541512237,11.5632083588676));
#39090=CARTESIAN_POINT('Ctrl Pts',(-3.62582421871883,-0.248154246652957,
11.7215772666518));
#39091=CARTESIAN_POINT('Ctrl Pts',(-1.76593578830562,-3.17642134905957,
11.879946174436));
#39092=CARTESIAN_POINT('Ctrl Pts',(1.70289122544452,-3.21066087737151,12.0383150822201));
#39093=CARTESIAN_POINT('Ctrl Pts',(3.62021936025047,-0.319677304242251,
12.1966839900043));
#39094=CARTESIAN_POINT('Ctrl Pts',(2.23917693853751,2.86256326272481,12.3550528977885));
#39095=CARTESIAN_POINT('Ctrl Pts',(-1.18197260099312,3.43673137816756,12.5134218055727));
#39096=CARTESIAN_POINT('Ctrl Pts',(-3.52623059396893,0.879704264703417,
12.6717907133568));
#39097=CARTESIAN_POINT('Ctrl Pts',(-2.65775090194473,-2.47881865782711,
12.8301596211411));
#39098=CARTESIAN_POINT('Ctrl Pts',(0.632197339137122,-3.57889764027531,
12.9885285289252));
#39099=CARTESIAN_POINT('Ctrl Pts',(3.34615255830021,-1.41825415626418,13.1468974367094));
#39100=CARTESIAN_POINT('Ctrl Pts',(3.01143862854347,2.03455626161957,13.3052663444935));
#39101=CARTESIAN_POINT('Ctrl Pts',(-0.0669876337345568,3.63368882158465,
13.4636352522777));
#39102=CARTESIAN_POINT('Ctrl Pts',(-3.08438167205765,1.92217884086064,13.6220041600619));
#39103=CARTESIAN_POINT('Ctrl Pts',(-3.29160519864739,-1.54062228057782,
13.7803730678461));
#39104=CARTESIAN_POINT('Ctrl Pts',(-0.499857505396188,-3.59976725212857,
13.9387419756303));
#39105=CARTESIAN_POINT('Ctrl Pts',(2.74730880042816,-2.37917551900835,14.0971108834144));
#39106=CARTESIAN_POINT('Ctrl Pts',(3.49141063549228,1.00907560149324,14.2554797911986));
#39107=CARTESIAN_POINT('Ctrl Pts',(1.05449914101583,3.47796109191871,14.4138486989828));
#39108=CARTESIAN_POINT('Ctrl Pts',(-2.34316322861594,2.77808708989957,14.572217606767));
#39109=CARTESIAN_POINT('Ctrl Pts',(-3.60597689618556,-0.452893386206675,
14.7305865145511));
#39110=CARTESIAN_POINT('Ctrl Pts',(-1.58339627179364,-3.27124411233226,
14.8889554223353));
#39111=CARTESIAN_POINT('Ctrl Pts',(1.88181175237025,-3.10917454036161,15.0473243301195));
#39112=CARTESIAN_POINT('Ctrl Pts',(3.63250696406091,-0.114345752568428,
15.2056932379037));
#39113=CARTESIAN_POINT('Ctrl Pts',(2.07363642186069,2.98466309495445,15.3640621456878));
#39114=CARTESIAN_POINT('Ctrl Pts',(-1.3745177904283,3.36435471203218,15.522431053472));
#39115=CARTESIAN_POINT('Ctrl Pts',(-3.57035313485565,0.678793260448534,
15.6807999612562));
#39116=CARTESIAN_POINT('Ctrl Pts',(-2.51325088571015,-2.62521462236299,
15.8391688690404));
#39117=CARTESIAN_POINT('Ctrl Pts',(0.833666400131346,-3.53739763808404,
15.9975377768245));
#39118=CARTESIAN_POINT('Ctrl Pts',(3.42103282912131,-1.22666874946649,16.1559066846087));
#39119=CARTESIAN_POINT('Ctrl Pts',(2.89150693293287,2.20167428284837,16.3142755923929));
#39120=CARTESIAN_POINT('Ctrl Pts',(-0.272461911328257,3.62407860504538,
16.4726445001771));
#39121=CARTESIAN_POINT('Ctrl Pts',(-3.18819154166072,1.74459650144857,16.6310134079612));
#39122=CARTESIAN_POINT('Ctrl Pts',(-3.19916984495366,-1.72438255620852,
16.7893823157454));
#39123=CARTESIAN_POINT('Ctrl Pts',(-0.29539442793911,-3.62228104133726,
16.9477512235296));
#39124=CARTESIAN_POINT('Ctrl Pts',(2.87751381050283,-2.21993250648107,17.1061201313138));
#39125=CARTESIAN_POINT('Ctrl Pts',(3.42872842851207,1.20499328643291,17.2644890390979));
#39126=CARTESIAN_POINT('Ctrl Pts',(0.856038843606223,3.53204642471219,17.4228579468821));
#39127=CARTESIAN_POINT('Ctrl Pts',(-2.49658422541149,2.64107652748156,17.5812268546663));
#39128=CARTESIAN_POINT('Ctrl Pts',(-3.57457879361101,-0.656195610212313,
17.7395957624505));
#39129=CARTESIAN_POINT('Ctrl Pts',(-1.39578274133968,-3.35556095880372,
17.8979646702347));
#39130=CARTESIAN_POINT('Ctrl Pts',(2.05470079874548,-2.99777882317738,18.0563335780188));
#39131=CARTESIAN_POINT('Ctrl Pts',(3.63316395418835,0.0914490823390936,
18.214702485803));
#39132=CARTESIAN_POINT('Ctrl Pts',(1.90144157325746,3.09701639513276,18.3730713935872));
#39133=CARTESIAN_POINT('Ctrl Pts',(-1.56263777564272,3.28155433635805,18.5314403013714));
#39134=CARTESIAN_POINT('Ctrl Pts',(-3.60308026145187,0.47503126817419,18.6898092091555));
#39135=CARTESIAN_POINT('Ctrl Pts',(-2.36061813094683,-2.76190423084517,
18.8481781169397));
#39136=CARTESIAN_POINT('Ctrl Pts',(1.03229853401496,-3.48708097537846,19.0065470247239));
#39137=CARTESIAN_POINT('Ctrl Pts',(3.48536252450907,-1.02600760740019,19.164915932508));
#39138=CARTESIAN_POINT('Ctrl Pts',(3.00239128577455,1.22402918834916,19.2704952043642));
#39139=CARTESIAN_POINT('Ctrl Pts',(2.33906170208295,1.99986569877995,19.3232848402922));
#39140=CARTESIAN_POINT('Ctrl Pts',(0.746306651681278,-2.79157576665282,
-0.106166650550309));
#39141=CARTESIAN_POINT('Ctrl Pts',(1.67223622398558,-2.54403550389017,-0.0533770146222503));
#39142=CARTESIAN_POINT('Ctrl Pts',(3.24268507292766,-1.05982779669291,0.0522022572338669));
#39143=CARTESIAN_POINT('Ctrl Pts',(2.6534650731888,2.14926606411138,0.210571165018042));
#39144=CARTESIAN_POINT('Ctrl Pts',(-0.357682584076165,3.39270859312819,
0.368940072802219));
#39145=CARTESIAN_POINT('Ctrl Pts',(-3.04072829396782,1.54878528015627,0.527308980586394));
#39146=CARTESIAN_POINT('Ctrl Pts',(-2.95452992250576,-1.70815807339205,
0.68567788837057));
#39147=CARTESIAN_POINT('Ctrl Pts',(-0.175865267296476,-3.40779769180092,
0.844046796154745));
#39148=CARTESIAN_POINT('Ctrl Pts',(2.76271393702636,-2.00313000159674,1.00241570393892));
#39149=CARTESIAN_POINT('Ctrl Pts',(3.18435839018718,1.22685880116299,1.16078461172309));
#39150=CARTESIAN_POINT('Ctrl Pts',(0.704657322436346,3.33891608823015,1.31915351950727));
#39151=CARTESIAN_POINT('Ctrl Pts',(-2.41700952929224,2.40897289227878,1.47752242729144));
#39152=CARTESIAN_POINT('Ctrl Pts',(-3.33657026206665,-0.715817532379567,
1.63589133507562));
#39153=CARTESIAN_POINT('Ctrl Pts',(-1.21617982955205,-3.18840813389497,
1.7942602428598));
#39154=CARTESIAN_POINT('Ctrl Pts',(2.01226174825295,-2.75606087831087,1.95262915064397));
#39155=CARTESIAN_POINT('Ctrl Pts',(3.40734133280407,0.187330513505284,2.11099805842815));
#39156=CARTESIAN_POINT('Ctrl Pts',(1.69800108538207,2.96004268849728,2.26936696621232));
#39157=CARTESIAN_POINT('Ctrl Pts',(-1.55838171690348,3.03587076679338,2.4277358739965));
#39158=CARTESIAN_POINT('Ctrl Pts',(-3.39492829062034,0.345725653439304,
2.58610478178067));
#39159=CARTESIAN_POINT('Ctrl Pts',(-2.13836604233647,-2.65940859709953,
2.74447368956486));
#39160=CARTESIAN_POINT('Ctrl Pts',(1.06645469713818,-3.24156420087077,2.90284259734902));
#39161=CARTESIAN_POINT('Ctrl Pts',(3.29963196167206,-0.87034066480747,3.0612115051332));
#39162=CARTESIAN_POINT('Ctrl Pts',(2.52652481095076,2.29384747252421,3.21958041291738));
#39163=CARTESIAN_POINT('Ctrl Pts',(-0.548491187817377,3.36811837123105,
3.37794932070155));
#39164=CARTESIAN_POINT('Ctrl Pts',(-3.12377858785101,1.37370712067109,3.53631822848573));
#39165=CARTESIAN_POINT('Ctrl Pts',(-2.8530010639088,-1.87228438993549,3.6946871362699));
#39166=CARTESIAN_POINT('Ctrl Pts',(0.0171368193147903,-3.41244344288364,
3.85305604405408));
#39167=CARTESIAN_POINT('Ctrl Pts',(2.8716614014058,-1.84353592652772,4.01142495183826));
#39168=CARTESIAN_POINT('Ctrl Pts',(3.10982424547006,1.40501141556627,4.16979385962243));
#39169=CARTESIAN_POINT('Ctrl Pts',(0.514635928994152,3.37345724415162,4.32816276740661));
#39170=CARTESIAN_POINT('Ctrl Pts',(-2.5494355758621,2.26835670944009,4.48653167519078));
#39171=CARTESIAN_POINT('Ctrl Pts',(-3.29072428697737,-0.903436541076219,
4.64490058297496));
#39172=CARTESIAN_POINT('Ctrl Pts',(-1.03384437418045,-3.25211157971146,
4.80326949075913));
#39173=CARTESIAN_POINT('Ctrl Pts',(2.16496792021978,-2.63779791136634,4.96163839854332));
#39174=CARTESIAN_POINT('Ctrl Pts',(3.39128470168976,0.379805198589325,5.12000730632749));
#39175=CARTESIAN_POINT('Ctrl Pts',(1.52781257931188,3.05136897790507,5.27837621411166));
#39176=CARTESIAN_POINT('Ctrl Pts',(-1.72764481413208,2.94284000805473,5.43674512189584));
#39177=CARTESIAN_POINT('Ctrl Pts',(-3.40905041125902,0.153098694643912,
5.59511402968001));
#39178=CARTESIAN_POINT('Ctrl Pts',(-1.98448082200849,-2.77613036147294,
5.75348293746419));
#39179=CARTESIAN_POINT('Ctrl Pts',(1.24814304847173,-3.17603571254481,5.91185184524837));
#39180=CARTESIAN_POINT('Ctrl Pts',(3.34358768428832,-0.682264841747166,
6.07022075303254));
#39181=CARTESIAN_POINT('Ctrl Pts',(2.39270001988976,2.43311539628292,6.22858966081672));
#39182=CARTESIAN_POINT('Ctrl Pts',(-0.738169162435656,3.33169179313424,
6.38695856860088));
#39183=CARTESIAN_POINT('Ctrl Pts',(-3.1964947254872,1.19477419906089,6.54532747638508));
#39184=CARTESIAN_POINT('Ctrl Pts',(-2.74250392385152,-2.03069843759927,
6.70369638416923));
#39185=CARTESIAN_POINT('Ctrl Pts',(0.210173640495589,-3.40600806776054,
6.86206529195343));
#39186=CARTESIAN_POINT('Ctrl Pts',(2.97136265716555,-1.67811438120623,7.02043419973758));
#39187=CARTESIAN_POINT('Ctrl Pts',(3.02535243371638,1.578704078862,7.17880310752178));
#39188=CARTESIAN_POINT('Ctrl Pts',(0.322953053292851,3.39717018151548,7.33717201530594));
#39189=CARTESIAN_POINT('Ctrl Pts',(-2.67368784570132,2.12048513801866,7.49554092309013));
#39190=CARTESIAN_POINT('Ctrl Pts',(-3.23434009593761,-1.08816729440808,
7.65390983087429));
#39191=CARTESIAN_POINT('Ctrl Pts',(-0.848195182625461,-3.30539390224222,
7.81227873865848));
#39192=CARTESIAN_POINT('Ctrl Pts',(2.31073771344569,-2.51108644543929,7.97064764644264));
#39193=CARTESIAN_POINT('Ctrl Pts',(3.3643646930986,0.571064031996978,8.12901655422683));
#39194=CARTESIAN_POINT('Ctrl Pts',(1.35272950467657,3.13291985278694,8.287385462011));
#39195=CARTESIAN_POINT('Ctrl Pts',(-1.89137331212997,2.8403821769212,8.44575436979517));
#39196=CARTESIAN_POINT('Ctrl Pts',(-3.41225180926891,-0.0400188324442784,
8.60412327757936));
#39197=CARTESIAN_POINT('Ctrl Pts',(-1.82423833629739,-2.88395880851166,
8.76249218536352));
#39198=CARTESIAN_POINT('Ctrl Pts',(1.42583298946127,-3.10033291808686,8.9208610931477));
#39199=CARTESIAN_POINT('Ctrl Pts',(3.37683233008282,-0.492003385472662,
9.07923000093188));
#39200=CARTESIAN_POINT('Ctrl Pts',(2.25121027749802,2.564588895573,9.23759890871605));
#39201=CARTESIAN_POINT('Ctrl Pts',(-0.925482430462337,3.2845922407073,9.39596781650024));
#39202=CARTESIAN_POINT('Ctrl Pts',(-3.25897098545631,1.0120138500846,9.55433672428439));
#39203=CARTESIAN_POINT('Ctrl Pts',(-2.6232212503609,-2.18260719976455,9.71270563206859));
#39204=CARTESIAN_POINT('Ctrl Pts',(0.402537176038361,-3.38866164417696,
9.87107453985274));
#39205=CARTESIAN_POINT('Ctrl Pts',(3.06154523810132,-1.50731704424391,10.0294434476369));
#39206=CARTESIAN_POINT('Ctrl Pts',(2.93118899211157,1.74733940873922,10.1878123554211));
#39207=CARTESIAN_POINT('Ctrl Pts',(0.130235606808038,3.410000381749,10.3461812632053));
#39208=CARTESIAN_POINT('Ctrl Pts',(-2.78937503325262,1.96582065323264,10.5045501709895));
#39209=CARTESIAN_POINT('Ctrl Pts',(-3.16759478916177,-1.26941213499964,
10.6629190787736));
#39210=CARTESIAN_POINT('Ctrl Pts',(-0.659828822141922,-3.34808749023676,
10.8212879865578));
#39211=CARTESIAN_POINT('Ctrl Pts',(2.44910512469472,-2.37633078610767,10.979656894342));
#39212=CARTESIAN_POINT('Ctrl Pts',(3.32666703871794,0.760493478155309,11.1380258021261));
#39213=CARTESIAN_POINT('Ctrl Pts',(1.1733129998774,3.20443450879057,11.2963947099104));
#39214=CARTESIAN_POINT('Ctrl Pts',(-2.04904284997734,2.72882526295945,11.4547636176945));
#39215=CARTESIAN_POINT('Ctrl Pts',(-3.40452215648823,-0.233008160350131,
11.6131325254787));
#39216=CARTESIAN_POINT('Ctrl Pts',(-1.6581519554046,-2.98254857623426,11.7715014332628));
#39217=CARTESIAN_POINT('Ctrl Pts',(1.59895531536931,-3.01469829605903,11.9298703410471));
#39218=CARTESIAN_POINT('Ctrl Pts',(3.3992593903726,-0.300165810466054,12.0882392488312));
#39219=CARTESIAN_POINT('Ctrl Pts',(2.10250884755856,2.68784680790165,12.2466081566154));
#39220=CARTESIAN_POINT('Ctrl Pts',(-1.10983094207061,3.2269705912561,12.4049770643995));
#39221=CARTESIAN_POINT('Ctrl Pts',(-3.3110072253574,0.826011543769279,12.5633459721838));
#39222=CARTESIAN_POINT('Ctrl Pts',(-2.49553516284214,-2.32752404237368,
12.7217148799679));
#39223=CARTESIAN_POINT('Ctrl Pts',(0.593611195284521,-3.36045974022041,
12.8800837877521));
#39224=CARTESIAN_POINT('Ctrl Pts',(3.14192024668758,-1.3316910603678,13.0384526955363));
#39225=CARTESIAN_POINT('Ctrl Pts',(2.82763557065198,1.91037718694295,13.1968216033204));
#39226=CARTESIAN_POINT('Ctrl Pts',(-0.0628990457073522,3.41190674357617,
13.3551905111046));
#39227=CARTESIAN_POINT('Ctrl Pts',(-2.89612653789845,1.80485871837307,13.5135594188888));
#39228=CARTESIAN_POINT('Ctrl Pts',(-3.09070218334153,-1.44659045022871,
13.671928326673));
#39229=CARTESIAN_POINT('Ctrl Pts',(-0.469348718954053,-3.38005557599891,
13.8302972344571));
#39230=CARTESIAN_POINT('Ctrl Pts',(2.57962689792991,-2.23396261926356,13.9886661422413));
#39231=CARTESIAN_POINT('Ctrl Pts',(3.27831250190397,0.947486705262652,14.1470350500255));
#39232=CARTESIAN_POINT('Ctrl Pts',(0.990137820540776,3.26568385078115,14.3054039578097));
#39233=CARTESIAN_POINT('Ctrl Pts',(-2.20014833783372,2.60852663551323,14.4637728655938));
#39234=CARTESIAN_POINT('Ctrl Pts',(-3.38588621463462,-0.425251053238435,
14.6221417733781));
#39235=CARTESIAN_POINT('Ctrl Pts',(-1.48675373229403,-3.07158383526162,
14.7805106811622));
#39236=CARTESIAN_POINT('Ctrl Pts',(1.7669554338043,-2.91940617429889,14.9388795889464));
#39237=CARTESIAN_POINT('Ctrl Pts',(3.41079702068761,-0.107366663311963,
15.0972484967305));
#39238=CARTESIAN_POINT('Ctrl Pts',(1.94707209088592,2.8024942808771,15.2556174045147));
#39239=CARTESIAN_POINT('Ctrl Pts',(-1.29062414218578,3.15901143256371,15.4139863122989));
#39240=CARTESIAN_POINT('Ctrl Pts',(-3.35243674840872,0.637363136067446,
15.5723552200831));
#39241=CARTESIAN_POINT('Ctrl Pts',(-2.35985470035756,-2.46498473401718,
15.7307241278673));
#39242=CARTESIAN_POINT('Ctrl Pts',(0.782783598750917,-3.32149268930132,
15.8890930356514));
#39243=CARTESIAN_POINT('Ctrl Pts',(3.21223020263583,-1.15179906258833,16.0474619434356));
#39244=CARTESIAN_POINT('Ctrl Pts',(2.71502390214816,2.06729516522899,16.2058308512198));
#39245=CARTESIAN_POINT('Ctrl Pts',(-0.255832207509483,3.40288308628807,
16.364199759004));
#39246=CARTESIAN_POINT('Ctrl Pts',(-2.99360037551616,1.63811511122076,16.5225686667881));
#39247=CARTESIAN_POINT('Ctrl Pts',(-3.0039086184278,-1.61913492346524,16.6809375745723));
#39248=CARTESIAN_POINT('Ctrl Pts',(-0.277365038721381,-3.40119523682191,
16.8393064823565));
#39249=CARTESIAN_POINT('Ctrl Pts',(2.70188484948655,-2.0844389987813,16.9976753901407));
#39250=CARTESIAN_POINT('Ctrl Pts',(3.21945610137027,1.13144656072985,17.1560442979248));
#39251=CARTESIAN_POINT('Ctrl Pts',(0.803790540872318,3.31646808706206,17.314413205709));
#39252=CARTESIAN_POINT('Ctrl Pts',(-2.34420528912341,2.47987850827725,17.4727821134932));
#39253=CARTESIAN_POINT('Ctrl Pts',(-3.35640449422057,-0.616144732671989,
17.6311510212774));
#39254=CARTESIAN_POINT('Ctrl Pts',(-1.31059118751595,-3.15075440577503,
17.7895199290615));
#39255=CARTESIAN_POINT('Ctrl Pts',(1.92929220290631,-2.81480949105824,17.9478888368457));
#39256=CARTESIAN_POINT('Ctrl Pts',(3.41141391144418,0.0858674905988609,
18.1062577446299));
#39257=CARTESIAN_POINT('Ctrl Pts',(1.78538714921769,2.90799010106519,18.264626652414));
#39258=CARTESIAN_POINT('Ctrl Pts',(-1.46726223027463,3.08126477510226,18.4229955601983));
#39259=CARTESIAN_POINT('Ctrl Pts',(-3.38316637590686,0.44603775030638,18.5813644679824));
#39260=CARTESIAN_POINT('Ctrl Pts',(-2.21653788077352,-2.59333149673027,
18.7397333757666));
#39261=CARTESIAN_POINT('Ctrl Pts',(0.969292226859822,-3.27424710245315,
18.8981022835507));
#39262=CARTESIAN_POINT('Ctrl Pts',(3.27263353717619,-0.963385266744592,
19.056471191335));
#39263=CARTESIAN_POINT('Ctrl Pts',(2.81914043215213,1.14932060699719,19.1620504631911));
#39264=CARTESIAN_POINT('Ctrl Pts',(2.19629714783811,1.87780396146808,19.2148400991191));
#39265=CARTESIAN_POINT('Ctrl Pts',(0.697794938882252,-2.61011668204799,
-0.214611391723435));
#39266=CARTESIAN_POINT('Ctrl Pts',(1.56353688002641,-2.37866712691375,-0.161821755795376));
#39267=CARTESIAN_POINT('Ctrl Pts',(3.03190280721802,-0.990936461510826,
-0.056242483939259));
#39268=CARTESIAN_POINT('Ctrl Pts',(2.48098351314537,2.00955864250931,0.102126423844917));
#39269=CARTESIAN_POINT('Ctrl Pts',(-0.334432362799391,3.17217444069923,
0.260495331629093));
#39270=CARTESIAN_POINT('Ctrl Pts',(-2.84307370069235,1.44811054205896,0.418864239413268));
#39271=CARTESIAN_POINT('Ctrl Pts',(-2.76247842901601,-1.59712372352387,
0.577233147197444));
#39272=CARTESIAN_POINT('Ctrl Pts',(-0.164433605366102,-3.18628271196066,
0.73560205498162));
#39273=CARTESIAN_POINT('Ctrl Pts',(2.58313094020199,-1.87292177269022,0.893970962765795));
#39274=CARTESIAN_POINT('Ctrl Pts',(2.97736749800375,1.14711005220988,1.05233987054997));
#39275=CARTESIAN_POINT('Ctrl Pts',(0.658852915399703,3.12187857695061,1.21070877833415));
#39276=CARTESIAN_POINT('Ctrl Pts',(-2.25989814370645,2.25238390727161,1.36907768611832));
#39277=CARTESIAN_POINT('Ctrl Pts',(-3.1196852350841,-0.66928768507206,1.5274465939025));
#39278=CARTESIAN_POINT('Ctrl Pts',(-1.13712523923012,-2.98115399870921,
1.68581550168667));
#39279=CARTESIAN_POINT('Ctrl Pts',(1.88145993402846,-2.576910346175,1.84418440947086));
#39280=CARTESIAN_POINT('Ctrl Pts',(3.18585601738733,0.175153583219069,2.00255331725503));
#39281=CARTESIAN_POINT('Ctrl Pts',(1.58762696396573,2.76763285206644,2.16092222503921));
#39282=CARTESIAN_POINT('Ctrl Pts',(-1.45708318752367,2.8385319243727,2.31929113282338));
#39283=CARTESIAN_POINT('Ctrl Pts',(-3.17424985255893,0.323252661179191,
2.47766004060756));
#39284=CARTESIAN_POINT('Ctrl Pts',(-1.99936714815359,-2.48654069382262,
2.63602894839173));
#39285=CARTESIAN_POINT('Ctrl Pts',(0.997132597617568,-3.03085479451885,
2.7943978561759));
#39286=CARTESIAN_POINT('Ctrl Pts',(3.08514801233767,-0.813766445251292,
2.95276676396009));
#39287=CARTESIAN_POINT('Ctrl Pts',(2.36229467079009,2.14474191445211,3.11113567174426));
#39288=CARTESIAN_POINT('Ctrl Pts',(-0.512837952091488,3.14918264188951,
3.26950457952844));
#39289=CARTESIAN_POINT('Ctrl Pts',(-2.92072552734273,1.28441288061864,3.4278734873126));
#39290=CARTESIAN_POINT('Ctrl Pts',(-2.66754918844198,-1.75058143794112,
3.58624239509679));
#39291=CARTESIAN_POINT('Ctrl Pts',(0.0160228851765723,-3.19062647813978,
3.74461130288096));
#39292=CARTESIAN_POINT('Ctrl Pts',(2.6849965594843,-1.72370169323913,3.90298021066514));
#39293=CARTESIAN_POINT('Ctrl Pts',(2.90767825050696,1.31368232166397,4.06134911844931));
#39294=CARTESIAN_POINT('Ctrl Pts',(0.48118336585917,3.15417447533345,4.21971802623349));
#39295=CARTESIAN_POINT('Ctrl Pts',(-2.38371618132472,2.12090811178094,4.37808693401766));
#39296=CARTESIAN_POINT('Ctrl Pts',(-3.0768193577489,-0.844711010606807,
4.53645584180184));
#39297=CARTESIAN_POINT('Ctrl Pts',(-0.966642023449493,-3.04071656857237,
4.69482474958602));
#39298=CARTESIAN_POINT('Ctrl Pts',(2.02423984051125,-2.46633475421801,4.85319365737019));
#39299=CARTESIAN_POINT('Ctrl Pts',(3.17084310560123,0.355116954591987,5.01156256515437));
#39300=CARTESIAN_POINT('Ctrl Pts',(1.42850111680335,2.85302271478855,5.16993147293854));
#39301=CARTESIAN_POINT('Ctrl Pts',(-1.61534377962691,2.75154838689254,5.32830038072272));
#39302=CARTESIAN_POINT('Ctrl Pts',(-3.18745400166542,0.143146914249436,
5.48666928850689));
#39303=CARTESIAN_POINT('Ctrl Pts',(-1.85548483426596,-2.59567526505241,
5.64503819629107));
#39304=CARTESIAN_POINT('Ctrl Pts',(1.1670107726664,-2.96958581426328,5.80340710407524));
#39305=CARTESIAN_POINT('Ctrl Pts',(3.12624650812014,-0.637915999376343,
5.96177601185942));
#39306=CARTESIAN_POINT('Ctrl Pts',(2.23716881040954,2.27495709091949,6.1201449196436));
#39307=CARTESIAN_POINT('Ctrl Pts',(-0.690186405850939,3.1151238782707,6.27851382742777));
#39308=CARTESIAN_POINT('Ctrl Pts',(-2.98871494255602,1.1171110257876,6.43688273521195));
#39309=CARTESIAN_POINT('Ctrl Pts',(-2.56423462609788,-1.89869819458346,
6.59525164299611));
#39310=CARTESIAN_POINT('Ctrl Pts',(0.19651185245889,-3.18460941775236,6.75362055078031));
#39311=CARTESIAN_POINT('Ctrl Pts',(2.77821699576559,-1.56903294300439,6.91198945856447));
#39312=CARTESIAN_POINT('Ctrl Pts',(2.82869730803894,1.47608454747249,7.07035836634865));
#39313=CARTESIAN_POINT('Ctrl Pts',(0.30196033437012,3.17634601519748,7.22872727413282));
#39314=CARTESIAN_POINT('Ctrl Pts',(-2.49989175719976,1.98264854527436,7.387096181917));
#39315=CARTESIAN_POINT('Ctrl Pts',(-3.02410027364065,-1.01743382426589,
7.54546508970118));
#39316=CARTESIAN_POINT('Ctrl Pts',(-0.793060472242878,-3.09053541302469,
7.70383399748535));
#39317=CARTESIAN_POINT('Ctrl Pts',(2.16053424941917,-2.34785983586768,7.86220290526953));
#39318=CARTESIAN_POINT('Ctrl Pts',(3.1456729617907,0.533943507548107,8.0205718130537));
#39319=CARTESIAN_POINT('Ctrl Pts',(1.26479885970938,2.92927258824979,8.17894072083787));
#39320=CARTESIAN_POINT('Ctrl Pts',(-1.76842953465313,2.65575055921304,8.33730962862206));
#39321=CARTESIAN_POINT('Ctrl Pts',(-3.19044730116719,-0.0374175128637604,
8.49567853640622));
#39322=CARTESIAN_POINT('Ctrl Pts',(-1.70565849241141,-2.69649460579077,
8.65404744419042));
#39323=CARTESIAN_POINT('Ctrl Pts',(1.33315044358244,-2.89880388204682,8.81241635197457));
#39324=CARTESIAN_POINT('Ctrl Pts',(3.1573301726273,-0.460021991660309,8.97078525975877));
#39325=CARTESIAN_POINT('Ctrl Pts',(2.10487623882079,2.39788449910363,9.12915416754292));
#39326=CARTESIAN_POINT('Ctrl Pts',(-0.865323864588658,3.07108590911539,
9.28752307532712));
#39327=CARTESIAN_POINT('Ctrl Pts',(-3.04713009657952,0.946230535500251,
9.44589198311128));
#39328=CARTESIAN_POINT('Ctrl Pts',(-2.45270561095299,-2.04073252480415,
9.60426089089545));
#39329=CARTESIAN_POINT('Ctrl Pts',(0.37637129927589,-3.16839055308451,9.76262979867964));
#39330=CARTESIAN_POINT('Ctrl Pts',(2.86253749379487,-1.40933784041033,9.9209987064638));
#39331=CARTESIAN_POINT('Ctrl Pts',(2.74065471478115,1.63375817859982,10.079367614248));
#39332=CARTESIAN_POINT('Ctrl Pts',(0.121769981666623,3.18834222180723,10.2377365220322));
#39333=CARTESIAN_POINT('Ctrl Pts',(-2.60805900156902,1.8380376209775,10.3961054298164));
#39334=CARTESIAN_POINT('Ctrl Pts',(-2.96169357103739,-1.18689731782901,
10.5544743376005));
#39335=CARTESIAN_POINT('Ctrl Pts',(-0.616938374570327,-3.13045381594687,
10.7128432453847));
#39336=CARTESIAN_POINT('Ctrl Pts',(2.28990744883834,-2.22186361587486,10.8712121531689));
#39337=CARTESIAN_POINT('Ctrl Pts',(3.11042574487886,0.711059587790419,11.029581060953));
#39338=CARTESIAN_POINT('Ctrl Pts',(1.09704485575034,2.99613862100298,11.1879499687372));
#39339=CARTESIAN_POINT('Ctrl Pts',(-1.91585017639328,2.55144511079655,11.3463188765214));
#39340=CARTESIAN_POINT('Ctrl Pts',(-3.18322009425763,-0.217862074047309,
11.5046877843056));
#39341=CARTESIAN_POINT('Ctrl Pts',(-1.55036812250359,-2.78867580340896,
11.6630566920897));
#39342=CARTESIAN_POINT('Ctrl Pts',(1.49501940529411,-2.81873571474656,11.821425599874));
#39343=CARTESIAN_POINT('Ctrl Pts',(3.17829942049473,-0.280654316689852,
11.9797945076581));
#39344=CARTESIAN_POINT('Ctrl Pts',(1.96584075657961,2.51313035307848,12.1381634154423));
#39345=CARTESIAN_POINT('Ctrl Pts',(-1.03768928314808,3.01720980434465,12.2965323232264));
#39346=CARTESIAN_POINT('Ctrl Pts',(-3.09578385674587,0.772318822835137,
12.4549012310106));
#39347=CARTESIAN_POINT('Ctrl Pts',(-2.33331942373952,-2.17622942692025,
12.6132701387948));
#39348=CARTESIAN_POINT('Ctrl Pts',(0.555025051431915,-3.14202184016551,
12.771639046579));
#39349=CARTESIAN_POINT('Ctrl Pts',(2.93768793507494,-1.24512796447142,12.9300079543632));
#39350=CARTESIAN_POINT('Ctrl Pts',(2.64383251276049,1.78619811226633,13.0883768621473));
#39351=CARTESIAN_POINT('Ctrl Pts',(-0.0588104576801453,3.19012466556769,
13.2467457699315));
#39352=CARTESIAN_POINT('Ctrl Pts',(-2.70787140373924,1.6875385958855,13.4051146777157));
#39353=CARTESIAN_POINT('Ctrl Pts',(-2.88979916803567,-1.35255861987959,
13.5634835854999));
#39354=CARTESIAN_POINT('Ctrl Pts',(-0.438839932511918,-3.16034389986926,
13.721852493284));
#39355=CARTESIAN_POINT('Ctrl Pts',(2.41194499543166,-2.08874971951875,13.8802214010682));
#39356=CARTESIAN_POINT('Ctrl Pts',(3.06521436831565,0.885897809032061,14.0385903088524));
#39357=CARTESIAN_POINT('Ctrl Pts',(0.925776500065717,3.05340660964359,14.1969592166366));
#39358=CARTESIAN_POINT('Ctrl Pts',(-2.0571334470515,2.43896618112689,14.3553281244207));
#39359=CARTESIAN_POINT('Ctrl Pts',(-3.16579553308368,-0.397608720270194,
14.5136970322049));
#39360=CARTESIAN_POINT('Ctrl Pts',(-1.39011119279443,-2.871923558191,14.6720659399891));
#39361=CARTESIAN_POINT('Ctrl Pts',(1.65209911523836,-2.72963780823618,14.8304348477733));
#39362=CARTESIAN_POINT('Ctrl Pts',(3.18908707731431,-0.100387574055494,
14.9888037555574));
#39363=CARTESIAN_POINT('Ctrl Pts',(1.82050775991116,2.62032546679975,15.1471726633416));
#39364=CARTESIAN_POINT('Ctrl Pts',(-1.20673049394325,2.95366815309523,15.3055415711258));
#39365=CARTESIAN_POINT('Ctrl Pts',(-3.13452036196177,0.595933011686356,
15.46391047891));
#39366=CARTESIAN_POINT('Ctrl Pts',(-2.20645851500496,-2.30475484567138,
15.6222793866941));
#39367=CARTESIAN_POINT('Ctrl Pts',(0.731900797370488,-3.1055877405186,15.7806482944783));
#39368=CARTESIAN_POINT('Ctrl Pts',(3.00342757615037,-1.07692937571016,15.9390172022625));
#39369=CARTESIAN_POINT('Ctrl Pts',(2.53854087136345,1.93291604760962,16.0973861100467));
#39370=CARTESIAN_POINT('Ctrl Pts',(-0.239202503690712,3.18168756753077,
16.2557550178309));
#39371=CARTESIAN_POINT('Ctrl Pts',(-2.79900920937161,1.53163372099295,16.414123925615));
#39372=CARTESIAN_POINT('Ctrl Pts',(-2.80864739190195,-1.51388729072196,
16.5724928333992));
#39373=CARTESIAN_POINT('Ctrl Pts',(-0.259335649503649,-3.18010943230655,
16.7308617411834));
#39374=CARTESIAN_POINT('Ctrl Pts',(2.52625588847025,-1.94894549108153,16.8892306489676));
#39375=CARTESIAN_POINT('Ctrl Pts',(3.01018377422847,1.05789983502679,17.0475995567517));
#39376=CARTESIAN_POINT('Ctrl Pts',(0.751542238138412,3.10088974941192,17.2059684645359));
#39377=CARTESIAN_POINT('Ctrl Pts',(-2.19182635283533,2.31868048907294,17.3643373723201));
#39378=CARTESIAN_POINT('Ctrl Pts',(-3.13823019483013,-0.576093855131663,
17.5227062801042));
#39379=CARTESIAN_POINT('Ctrl Pts',(-1.22539963369223,-2.94594785274635,
17.6810751878884));
#39380=CARTESIAN_POINT('Ctrl Pts',(1.80388360706713,-2.63184015893912,17.8394440956726));
#39381=CARTESIAN_POINT('Ctrl Pts',(3.18966386870002,0.0802858988586278,
17.9978130034568));
#39382=CARTESIAN_POINT('Ctrl Pts',(1.66933272517792,2.71896380699763,18.1561819112409));
#39383=CARTESIAN_POINT('Ctrl Pts',(-1.37188668490652,2.88097521384648,18.3145508190252));
#39384=CARTESIAN_POINT('Ctrl Pts',(-3.16325249036186,0.417044232438571,
18.4729197268093));
#39385=CARTESIAN_POINT('Ctrl Pts',(-2.0724576306002,-2.42475876261538,18.6312886345935));
#39386=CARTESIAN_POINT('Ctrl Pts',(0.906285919704686,-3.06141322952783,
18.7896575423776));
#39387=CARTESIAN_POINT('Ctrl Pts',(3.05990454984331,-0.900762926088991,
18.9480264501619));
#39388=CARTESIAN_POINT('Ctrl Pts',(2.63588957852971,1.07461202564522,19.053605722018));
#39389=CARTESIAN_POINT('Ctrl Pts',(2.05353259359326,1.75574222415622,19.106395357946));
#39390=CARTESIAN_POINT('Ctrl Pts',(0.649283226083226,-2.42865759744316,
-0.323056132896561));
#39391=CARTESIAN_POINT('Ctrl Pts',(1.45483753606724,-2.21329874993732,-0.270266496968503));
#39392=CARTESIAN_POINT('Ctrl Pts',(2.82112054150838,-0.922045126328744,
-0.164687225112385));
#39393=CARTESIAN_POINT('Ctrl Pts',(2.30850195310193,1.86985122090724,-0.00631831732820976));
#39394=CARTESIAN_POINT('Ctrl Pts',(-0.311182141522623,2.95164028827028,
0.152050590455966));
#39395=CARTESIAN_POINT('Ctrl Pts',(-2.64541910741689,1.34743580396164,0.310419498240141));
#39396=CARTESIAN_POINT('Ctrl Pts',(-2.57042693552626,-1.48608937365568,
0.468788406024318));
#39397=CARTESIAN_POINT('Ctrl Pts',(-0.153001943435726,-2.96476773212039,
0.627157313808493));
#39398=CARTESIAN_POINT('Ctrl Pts',(2.40354794337761,-1.7427135437837,0.785526221592669));
#39399=CARTESIAN_POINT('Ctrl Pts',(2.77037660582034,1.06736130325675,0.943895129376844));
#39400=CARTESIAN_POINT('Ctrl Pts',(0.613048508363059,2.90484106567108,1.10226403716102));
#39401=CARTESIAN_POINT('Ctrl Pts',(-2.10278675812066,2.09579492226445,1.2606329449452));
#39402=CARTESIAN_POINT('Ctrl Pts',(-2.90280020810156,-0.622757837764556,
1.41900185272937));
#39403=CARTESIAN_POINT('Ctrl Pts',(-1.05807064890818,-2.77389986352343,
1.57737076051355));
#39404=CARTESIAN_POINT('Ctrl Pts',(1.75065811980397,-2.39775981403912,1.73573966829772));
#39405=CARTESIAN_POINT('Ctrl Pts',(2.9643707019706,0.162976652932851,1.8941085760819));
#39406=CARTESIAN_POINT('Ctrl Pts',(1.4772528425494,2.57522301563561,2.05247748386607));
#39407=CARTESIAN_POINT('Ctrl Pts',(-1.35578465814388,2.64119308195202,2.21084639165025));
#39408=CARTESIAN_POINT('Ctrl Pts',(-2.95357141449753,0.30077966891908,2.36921529943442));
#39409=CARTESIAN_POINT('Ctrl Pts',(-1.86036825397072,-2.3136727905457,2.5275842072186));
#39410=CARTESIAN_POINT('Ctrl Pts',(0.927810498096964,-2.82014538816694,
2.68595311500277));
#39411=CARTESIAN_POINT('Ctrl Pts',(2.87066406300329,-0.757192225695111,
2.84432202278695));
#39412=CARTESIAN_POINT('Ctrl Pts',(2.19806453062942,1.99563635637999,3.00269093057112));
#39413=CARTESIAN_POINT('Ctrl Pts',(-0.477184716365594,2.93024691254798,
3.16105983835531));
#39414=CARTESIAN_POINT('Ctrl Pts',(-2.71767246683444,1.19511864056618,3.31942874613947));
#39415=CARTESIAN_POINT('Ctrl Pts',(-2.48209731297516,-1.62887848594674,
3.47779765392366));
#39416=CARTESIAN_POINT('Ctrl Pts',(0.0149089510383518,-2.96880951339593,
3.63616656170783));
#39417=CARTESIAN_POINT('Ctrl Pts',(2.49833171756281,-1.60386745995054,3.79453546949201));
#39418=CARTESIAN_POINT('Ctrl Pts',(2.70553225554386,1.22235322776168,3.95290437727618));
#39419=CARTESIAN_POINT('Ctrl Pts',(0.447730802724189,2.93489170651531,4.11127328506035));
#39420=CARTESIAN_POINT('Ctrl Pts',(-2.21799678678734,1.97345951412179,4.26964219284454));
#39421=CARTESIAN_POINT('Ctrl Pts',(-2.86291442852043,-0.785985480137393,
4.42801110062871));
#39422=CARTESIAN_POINT('Ctrl Pts',(-0.899439672718537,-2.82932155743327,
4.58638000841288));
#39423=CARTESIAN_POINT('Ctrl Pts',(1.88351176080272,-2.29487159706967,4.74474891619707));
#39424=CARTESIAN_POINT('Ctrl Pts',(2.95040150951271,0.330428710594652,4.90311782398123));
#39425=CARTESIAN_POINT('Ctrl Pts',(1.32918965429481,2.65467645167202,5.06148673176541));
#39426=CARTESIAN_POINT('Ctrl Pts',(-1.50304274512173,2.56025676573035,5.21985563954959));
#39427=CARTESIAN_POINT('Ctrl Pts',(-2.96585759207181,0.133195133854954,
5.37822454733376));
#39428=CARTESIAN_POINT('Ctrl Pts',(-1.72648884652342,-2.41522016863187,
5.53659345511794));
#39429=CARTESIAN_POINT('Ctrl Pts',(1.08587849686107,-2.76313591598177,5.69496236290211));
#39430=CARTESIAN_POINT('Ctrl Pts',(2.90890533195194,-0.593567157005514,
5.85333127068629));
#39431=CARTESIAN_POINT('Ctrl Pts',(2.08163760092934,2.11679878555605,6.01170017847047));
#39432=CARTESIAN_POINT('Ctrl Pts',(-0.642203649266225,2.89855596340717,
6.17006908625463));
#39433=CARTESIAN_POINT('Ctrl Pts',(-2.78093515962483,1.03944785251432,6.32843799403883));
#39434=CARTESIAN_POINT('Ctrl Pts',(-2.38596532834426,-1.76669795156764,
6.48680690182298));
#39435=CARTESIAN_POINT('Ctrl Pts',(0.182850064422192,-2.96321076774417,
6.64517580960718));
#39436=CARTESIAN_POINT('Ctrl Pts',(2.58507133436564,-1.45995150480255,6.80354471739134));
#39437=CARTESIAN_POINT('Ctrl Pts',(2.63204218236152,1.37346501608299,6.96191362517552));
#39438=CARTESIAN_POINT('Ctrl Pts',(0.280967615447384,2.95552184887948,7.12028253295969));
#39439=CARTESIAN_POINT('Ctrl Pts',(-2.32609566869819,1.84481195253004,7.27865144074388));
#39440=CARTESIAN_POINT('Ctrl Pts',(-2.81386045134371,-0.946700354123697,
7.43702034852803));
#39441=CARTESIAN_POINT('Ctrl Pts',(-0.737925761860293,-2.87567692380717,
7.59538925631224));
#39442=CARTESIAN_POINT('Ctrl Pts',(2.01033078539266,-2.18463322629606,7.75375816409638));
#39443=CARTESIAN_POINT('Ctrl Pts',(2.9269812304828,0.496822983099234,7.91212707188058));
#39444=CARTESIAN_POINT('Ctrl Pts',(1.17686821474219,2.72562532371265,8.07049597966474));
#39445=CARTESIAN_POINT('Ctrl Pts',(-1.64548575717628,2.47111894150488,8.22886488744892));
#39446=CARTESIAN_POINT('Ctrl Pts',(-2.96864279306547,-0.0348161932832441,
8.3872337952331));
#39447=CARTESIAN_POINT('Ctrl Pts',(-1.58707864852543,-2.50903040306986,
8.54560270301728));
#39448=CARTESIAN_POINT('Ctrl Pts',(1.24046789770362,-2.69727484600679,8.70397161080145));
#39449=CARTESIAN_POINT('Ctrl Pts',(2.93782801517178,-0.428040597847953,
8.86234051858563));
#39450=CARTESIAN_POINT('Ctrl Pts',(1.95854220014356,2.23118010263425,9.02070942636979));
#39451=CARTESIAN_POINT('Ctrl Pts',(-0.805165298714976,2.8575795775235,9.17907833415399));
#39452=CARTESIAN_POINT('Ctrl Pts',(-2.83528920770275,0.880447220915903,
9.33744724193814));
#39453=CARTESIAN_POINT('Ctrl Pts',(-2.28218997154508,-1.89885784984376,
9.49581614972234));
#39454=CARTESIAN_POINT('Ctrl Pts',(0.35020542251342,-2.94811946199206,9.6541850575065));
#39455=CARTESIAN_POINT('Ctrl Pts',(2.66352974948841,-1.31135863657675,9.81255396529068));
#39456=CARTESIAN_POINT('Ctrl Pts',(2.55012043745071,1.52017694846043,9.97092287307486));
#39457=CARTESIAN_POINT('Ctrl Pts',(0.11330435652521,2.96668406186547,10.1292917808591));
#39458=CARTESIAN_POINT('Ctrl Pts',(-2.42674296988542,1.71025458872235,10.2876606886432));
#39459=CARTESIAN_POINT('Ctrl Pts',(-2.755792352913,-1.10438250065839,10.4460295964274));
#39460=CARTESIAN_POINT('Ctrl Pts',(-0.574047926998734,-2.91282014165699,
10.6043985042116));
#39461=CARTESIAN_POINT('Ctrl Pts',(2.13070977298197,-2.06739644564203,10.7627674119958));
#39462=CARTESIAN_POINT('Ctrl Pts',(2.89418445103978,0.661625697425526,10.9211363197799));
#39463=CARTESIAN_POINT('Ctrl Pts',(1.02077671162327,2.78784273321539,11.0795052275641));
#39464=CARTESIAN_POINT('Ctrl Pts',(-1.78265750280922,2.37406495863365,11.2378741353483));
#39465=CARTESIAN_POINT('Ctrl Pts',(-2.96191803202705,-0.202715987744488,
11.3962430431325));
#39466=CARTESIAN_POINT('Ctrl Pts',(-1.44258428960257,-2.59480303058365,
11.5546119509167));
#39467=CARTESIAN_POINT('Ctrl Pts',(1.39108349521891,-2.6227731334341,11.7129808587008));
#39468=CARTESIAN_POINT('Ctrl Pts',(2.95733945061687,-0.261142822913652,
11.871349766485));
#39469=CARTESIAN_POINT('Ctrl Pts',(1.82917266560066,2.33841389825531,12.0297186742692));
#39470=CARTESIAN_POINT('Ctrl Pts',(-0.965547624225554,2.80744901743319,
12.1880875820533));
#39471=CARTESIAN_POINT('Ctrl Pts',(-2.88056048813434,0.718626101900998,
12.3464564898375));
#39472=CARTESIAN_POINT('Ctrl Pts',(-2.17110368463692,-2.02493481146681,
12.5048253976217));
#39473=CARTESIAN_POINT('Ctrl Pts',(0.51643890757931,-2.92358394011061,12.6631943054059));
#39474=CARTESIAN_POINT('Ctrl Pts',(2.73345562346231,-1.15856486857504,12.8215632131901));
#39475=CARTESIAN_POINT('Ctrl Pts',(2.460029454869,1.66201903758971,12.9799321209742));
#39476=CARTESIAN_POINT('Ctrl Pts',(-0.0547218696529407,2.96834258755921,
13.1383010287584));
#39477=CARTESIAN_POINT('Ctrl Pts',(-2.51961626958004,1.57021847339793,13.2966699365426));
#39478=CARTESIAN_POINT('Ctrl Pts',(-2.68889615272982,-1.25852678953048,
13.4550388443267));
#39479=CARTESIAN_POINT('Ctrl Pts',(-0.408331146069782,-2.94063222373961,
13.6134077521109));
#39480=CARTESIAN_POINT('Ctrl Pts',(2.24426309293342,-1.94353681977395,13.7717766598951));
#39481=CARTESIAN_POINT('Ctrl Pts',(2.85211623472735,0.824308912801474,13.9301455676793));
#39482=CARTESIAN_POINT('Ctrl Pts',(0.861415179590656,2.84112936850602,14.0885144754634));
#39483=CARTESIAN_POINT('Ctrl Pts',(-1.91411855626928,2.26940572674055,14.2468833832476));
#39484=CARTESIAN_POINT('Ctrl Pts',(-2.94570485153274,-0.369966387301956,
14.4052522910318));
#39485=CARTESIAN_POINT('Ctrl Pts',(-1.29346865329481,-2.67226328112036,
14.563621198816));
#39486=CARTESIAN_POINT('Ctrl Pts',(1.53724279667241,-2.53986944217347,14.7219901066002));
#39487=CARTESIAN_POINT('Ctrl Pts',(2.96737713394102,-0.0934084847990243,
14.8803590143843));
#39488=CARTESIAN_POINT('Ctrl Pts',(1.69394342893639,2.43815665272238,15.0387279221685));
#39489=CARTESIAN_POINT('Ctrl Pts',(-1.12283684570072,2.74832487362677,15.1970968299527));
#39490=CARTESIAN_POINT('Ctrl Pts',(-2.91660397551482,0.554502887305266,
15.3554657377369));
#39491=CARTESIAN_POINT('Ctrl Pts',(-2.05306232965237,-2.14452495732557,
15.513834645521));
#39492=CARTESIAN_POINT('Ctrl Pts',(0.681017995990055,-2.88968279173588,
15.6722035533052));
#39493=CARTESIAN_POINT('Ctrl Pts',(2.7946249496649,-1.00205968883199,15.8305724610894));
#39494=CARTESIAN_POINT('Ctrl Pts',(2.36205784057873,1.79853692999024,15.9889413688736));
#39495=CARTESIAN_POINT('Ctrl Pts',(-0.222572799871934,2.96049204877346,
16.1473102766577));
#39496=CARTESIAN_POINT('Ctrl Pts',(-2.60441804322706,1.42515233076513,16.3056791844419));
#39497=CARTESIAN_POINT('Ctrl Pts',(-2.6133861653761,-1.40863965797868,16.4640480922261));
#39498=CARTESIAN_POINT('Ctrl Pts',(-0.241306260285921,-2.95902362779119,
16.6224170000102));
#39499=CARTESIAN_POINT('Ctrl Pts',(2.35062692745395,-1.81345198338176,16.7807859077945));
#39500=CARTESIAN_POINT('Ctrl Pts',(2.80091144708667,0.984353109323726,16.9391548155786));
#39501=CARTESIAN_POINT('Ctrl Pts',(0.699293935404505,2.88531141176178,17.0975237233628));
#39502=CARTESIAN_POINT('Ctrl Pts',(-2.03944741654725,2.15748246986864,17.255892631147));
#39503=CARTESIAN_POINT('Ctrl Pts',(-2.92005589543968,-0.536042977591341,
17.4142615389312));
#39504=CARTESIAN_POINT('Ctrl Pts',(-1.14020807986851,-2.74114129971766,
17.5726304467153));
#39505=CARTESIAN_POINT('Ctrl Pts',(1.67847501122794,-2.44887082681998,17.7309993544995));
#39506=CARTESIAN_POINT('Ctrl Pts',(2.96791382595584,0.0747043071183943,
17.8893682622837));
#39507=CARTESIAN_POINT('Ctrl Pts',(1.55327830113815,2.52993751293006,18.0477371700679));
#39508=CARTESIAN_POINT('Ctrl Pts',(-1.27651113953843,2.68068565259069,18.206106077852));
#39509=CARTESIAN_POINT('Ctrl Pts',(-2.94333860481685,0.388050714570759,
18.3644749856362));
#39510=CARTESIAN_POINT('Ctrl Pts',(-1.92837738042689,-2.25618602850048,
18.5228438934204));
#39511=CARTESIAN_POINT('Ctrl Pts',(0.843279612549552,-2.84857935660253,
18.6812128012046));
#39512=CARTESIAN_POINT('Ctrl Pts',(2.84717556251043,-0.838140585433388,
18.8395817089887));
#39513=CARTESIAN_POINT('Ctrl Pts',(2.45263872490728,0.999903444293248,18.9451609808448));
#39514=CARTESIAN_POINT('Ctrl Pts',(1.91076803934841,1.63368048684437,18.9979506167729));
#39515=CARTESIAN_POINT('Ctrl Pts',(0.793799282532864,-2.9692229537457,-2.78423117894278E-16));
#39516=CARTESIAN_POINT('Ctrl Pts',(0.887766721915256,-2.9348492446698,-2.60122598584039E-15));
#39517=CARTESIAN_POINT('Ctrl Pts',(0.979628067005363,-2.89561800221144,
-3.49555003596041E-15));
#39518=CARTESIAN_POINT('Ctrl Pts',(1.06916866443155,-2.85186613382074,-3.23005511226881E-15));
#39519=CARTESIAN_POINT('Ctrl Pts',(1.16002904452701,-2.80746938523814,-2.96064692901515E-15));
#39520=CARTESIAN_POINT('Ctrl Pts',(1.24850040694621,-2.75841707910134,-1.70928927322073E-15));
#39521=CARTESIAN_POINT('Ctrl Pts',(1.33432908742408,-2.70501521020721,-1.35308431126191E-15));
#39522=CARTESIAN_POINT('Ctrl Pts',(1.42022858512866,-2.65156927944197,-9.96585444661768E-16));
#39523=CARTESIAN_POINT('Ctrl Pts',(1.50348162410068,-2.59376582386862,-1.74304591459404E-15));
#39524=CARTESIAN_POINT('Ctrl Pts',(1.58379549048954,-2.53187705873125,-9.22872889219661E-16));
#39525=CARTESIAN_POINT('Ctrl Pts',(1.64739785919492,-2.48286594476085,-2.73359305730904E-16));
#39526=CARTESIAN_POINT('Ctrl Pts',(1.70915630400023,-2.43129195631135,-1.21478549956335E-15));
#39527=CARTESIAN_POINT('Ctrl Pts',(1.76890471985533,-2.37727978170559,-1.85268467234323E-15));
#39528=CARTESIAN_POINT('Ctrl Pts',(1.78260832618103,-2.36489181179879,-1.69449446100029E-15));
#39529=CARTESIAN_POINT('Ctrl Pts',(1.79620839750475,-2.3523732880026,-1.18822258932526E-16));
#39530=CARTESIAN_POINT('Ctrl Pts',(1.80968464748918,-2.33974304084967,-5.13478148889135E-16));
#39531=CARTESIAN_POINT('Ctrl Pts',(1.88211680870653,-2.27185797645468,-2.7899651133437E-15));
#39532=CARTESIAN_POINT('Ctrl Pts',(1.95108361340707,-2.20065250268282,-1.95723578809634E-15));
#39533=CARTESIAN_POINT('Ctrl Pts',(2.01634525032625,-2.12641641087435,-2.42861286636753E-15));
#39534=CARTESIAN_POINT('Ctrl Pts',(2.08117756282225,-2.05266868204296,-2.89688898515044E-15));
#39535=CARTESIAN_POINT('Ctrl Pts',(2.14235377267705,-1.97592928079205,8.44765968358672E-17));
#39536=CARTESIAN_POINT('Ctrl Pts',(2.19959532795681,-1.8964556490341,-9.71445146547012E-17));
#39537=CARTESIAN_POINT('Ctrl Pts',(2.25534354159704,-1.81905535862701,-2.74027418612624E-16));
#39538=CARTESIAN_POINT('Ctrl Pts',(2.30735997993029,-1.73906090637942,-2.45691015070983E-16));
#39539=CARTESIAN_POINT('Ctrl Pts',(2.35534084620635,-1.6566960329301,-3.33066907387547E-16));
#39540=CARTESIAN_POINT('Ctrl Pts',(2.39218550638746,-1.59344778402104,-4.00163133660391E-16));
#39541=CARTESIAN_POINT('Ctrl Pts',(2.4266496194399,-1.52880139924722,-3.4098607149105E-15));
#39542=CARTESIAN_POINT('Ctrl Pts',(2.45857474179235,-1.46285623457986,-1.30451205393456E-15));
#39543=CARTESIAN_POINT('Ctrl Pts',(2.46497201772008,-1.4496418947938,-7.93110398226214E-16));
#39544=CARTESIAN_POINT('Ctrl Pts',(2.47126331594316,-1.43638355863672,-2.07413338548309E-15));
#39545=CARTESIAN_POINT('Ctrl Pts',(2.47744641392549,-1.42308498824342,-1.88737914186277E-15));
#39546=CARTESIAN_POINT('Ctrl Pts',(2.51763430459499,-1.3366491118342,-8.64305086289203E-16));
#39547=CARTESIAN_POINT('Ctrl Pts',(2.55327433966832,-1.24847578889075,-1.3994068644472E-15));
#39548=CARTESIAN_POINT('Ctrl Pts',(2.58410580530037,-1.15880673981673,-1.33226762955019E-15));
#39549=CARTESIAN_POINT('Ctrl Pts',(2.61493727093243,-1.0691376907427,-1.26512839465317E-15));
#39550=CARTESIAN_POINT('Ctrl Pts',(2.64096062227041,-0.977972194521965,
-2.18326778438127E-15));
#39551=CARTESIAN_POINT('Ctrl Pts',(2.66185969210236,-0.885542657827795,
-4.16333634234434E-16));
#39552=CARTESIAN_POINT('Ctrl Pts',(2.66318121106867,-0.879698025182872,
-4.41723660151723E-16));
#39553=CARTESIAN_POINT('Ctrl Pts',(2.66448222104045,-0.873848337361808,
-3.11073001984487E-15));
#39554=CARTESIAN_POINT('Ctrl Pts',(2.66576263396923,-0.867993652908594,
-3.05311331771918E-15));
#39555=CARTESIAN_POINT('Ctrl Pts',(2.68612379311485,-0.774892310974501,
-2.15199967091541E-15));
#39556=CARTESIAN_POINT('Ctrl Pts',(2.70128071441176,-0.680526434244495,
-1.93615779328757E-15));
#39557=CARTESIAN_POINT('Ctrl Pts',(2.71131135145323,-0.585305736937107,
4.9960036108132E-16));
#39558=CARTESIAN_POINT('Ctrl Pts',(2.71436145645041,-0.556351132808682,
1.24026300173247E-15));
#39559=CARTESIAN_POINT('Ctrl Pts',(2.71693721397202,-0.527317589420452,
1.97945944668223E-16));
#39560=CARTESIAN_POINT('Ctrl Pts',(2.71903992025458,-0.498216958905591,
-8.60422844084496E-16));
#39561=CARTESIAN_POINT('Ctrl Pts',(2.72066941215208,-0.475665429940494,
-1.37880795766708E-15));
#39562=CARTESIAN_POINT('Ctrl Pts',(2.72201480614158,-0.453073615260271,
8.79161143954925E-16));
#39563=CARTESIAN_POINT('Ctrl Pts',(2.72307654238584,-0.430447121184021,
-8.32667268468867E-16));
#39564=CARTESIAN_POINT('Ctrl Pts',(2.72389118828461,-0.413086330589785,
-1.4285468048314E-15));
#39565=CARTESIAN_POINT('Ctrl Pts',(2.72453854393588,-0.395709062278408,
-1.32916983722708E-15));
#39566=CARTESIAN_POINT('Ctrl Pts',(2.72501883608608,-0.378334978099651,
-1.4432899320127E-15));
#39567=CARTESIAN_POINT('Ctrl Pts',(2.72759253700532,-0.285233942817064,
-2.05481563096606E-15));
#39568=CARTESIAN_POINT('Ctrl Pts',(2.72538042696458,-0.192083586758562,
-2.13427839413234E-15));
#39569=CARTESIAN_POINT('Ctrl Pts',(2.71851698412385,-0.0992587649797202,
-9.71445146547012E-16));
#39570=CARTESIAN_POINT('Ctrl Pts',(2.71162359278202,-0.00602890387282495,
1.96462101593499E-16));
#39571=CARTESIAN_POINT('Ctrl Pts',(2.70003782829147,0.0868735649517466,
3.96254244904816E-17));
#39572=CARTESIAN_POINT('Ctrl Pts',(2.68384500310791,0.179056180964395,0.));
#39573=CARTESIAN_POINT('Ctrl Pts',(2.66789631164747,0.269848990998196,-3.90280054297808E-17));
#39574=CARTESIAN_POINT('Ctrl Pts',(2.64747795906825,0.359944334746189,-1.65158417179709E-16));
#39575=CARTESIAN_POINT('Ctrl Pts',(2.62262856771139,0.448941443309629,-9.15933995315754E-16));
#39576=CARTESIAN_POINT('Ctrl Pts',(2.61402331282022,0.479760822052851,-1.17592487892117E-15));
#39577=CARTESIAN_POINT('Ctrl Pts',(2.60488633276693,0.510448211838593,-1.13142427929418E-15));
#39578=CARTESIAN_POINT('Ctrl Pts',(2.59521816034902,0.540985954218381,-1.11022302462516E-16));
#39579=CARTESIAN_POINT('Ctrl Pts',(2.58935888158599,0.55949298301996,5.41220718109879E-16));
#39580=CARTESIAN_POINT('Ctrl Pts',(2.58330449519924,0.577945037913408,-2.99423739596185E-16));
#39581=CARTESIAN_POINT('Ctrl Pts',(2.57705502797514,0.596338078066865,-5.82867087928207E-16));
#39582=CARTESIAN_POINT('Ctrl Pts',(2.57172583534412,0.612022623730196,-7.85788564701402E-16));
#39583=CARTESIAN_POINT('Ctrl Pts',(2.56625440043226,0.62766507688344,1.26864793468056E-15));
#39584=CARTESIAN_POINT('Ctrl Pts',(2.56064652768341,0.643247423606782,6.38378239159465E-16));
#39585=CARTESIAN_POINT('Ctrl Pts',(2.53007794912311,0.728186974002932,-1.52047584428395E-15));
#39586=CARTESIAN_POINT('Ctrl Pts',(2.49542222163634,0.81145269313479,-1.76096677592892E-15));
#39587=CARTESIAN_POINT('Ctrl Pts',(2.45674013243295,0.892671608124275,-2.27595720048157E-15));
#39588=CARTESIAN_POINT('Ctrl Pts',(2.42447605561005,0.960414932403238,-2.70550200953925E-15));
#39589=CARTESIAN_POINT('Ctrl Pts',(2.38941000579241,1.02673410646938,3.17065263267535E-16));
#39590=CARTESIAN_POINT('Ctrl Pts',(2.35155730975954,1.0913933075816,-2.16493489801906E-15));
#39591=CARTESIAN_POINT('Ctrl Pts',(2.33605432532997,1.11787518848119,-3.35396722920609E-15));
#39592=CARTESIAN_POINT('Ctrl Pts',(2.320083711266,1.1440783883098,2.22663090102326E-15));
#39593=CARTESIAN_POINT('Ctrl Pts',(2.30364573463797,1.16998563950688,1.0547118733939E-15));
#39594=CARTESIAN_POINT('Ctrl Pts',(2.28749640854811,1.19543795989525,-9.12481855642604E-17));
#39595=CARTESIAN_POINT('Ctrl Pts',(2.270909458915,1.22058319968122,-2.3008581611839E-16));
#39596=CARTESIAN_POINT('Ctrl Pts',(2.25389204750165,1.24539904737372,-1.66533453693773E-16));
#39597=CARTESIAN_POINT('Ctrl Pts',(2.20547130452195,1.31600918623414,1.42961996517205E-17));
#39598=CARTESIAN_POINT('Ctrl Pts',(2.1535546231662,1.38397612037656,2.23917548796031E-15));
#39599=CARTESIAN_POINT('Ctrl Pts',(2.09817041824585,1.44894279750897,9.99200722162641E-16));
#39600=CARTESIAN_POINT('Ctrl Pts',(2.05606612958433,1.49833189195019,5.65446788514969E-17));
#39601=CARTESIAN_POINT('Ctrl Pts',(2.01195712795118,1.54598639386782,-9.49244954967883E-16));
#39602=CARTESIAN_POINT('Ctrl Pts',(1.96584492925679,1.59173238567462,-1.0547118733939E-15));
#39603=CARTESIAN_POINT('Ctrl Pts',(1.94982090639806,1.60762915137139,-9.57905766773421E-16));
#39604=CARTESIAN_POINT('Ctrl Pts',(1.93355490152675,1.62329530307694,-1.35256693880661E-15));
#39605=CARTESIAN_POINT('Ctrl Pts',(1.91705309021378,1.63872826997869,-1.11022302462516E-16));
#39606=CARTESIAN_POINT('Origin',(0.,0.,20.));
#39607=CARTESIAN_POINT('Origin',(-3.42660592399111E-16,1.36827403442078E-16,
95.));
#39608=CARTESIAN_POINT('Ctrl Pts',(-1.91346599666497,1.63598720337506,95.));
#39609=CARTESIAN_POINT('Ctrl Pts',(-1.97637476724345,1.57686840642878,95.));
#39610=CARTESIAN_POINT('Ctrl Pts',(-2.03582478755404,1.5144166806707,95.));
#39611=CARTESIAN_POINT('Ctrl Pts',(-2.09180351026492,1.44902198639524,95.));
#39612=CARTESIAN_POINT('Ctrl Pts',(-2.1477822329758,1.38362729211977,95.));
#39613=CARTESIAN_POINT('Ctrl Pts',(-2.20029000314911,1.31528896999456,95.));
#39614=CARTESIAN_POINT('Ctrl Pts',(-2.24928637120995,1.24435238874975,95.));
#39615=CARTESIAN_POINT('Ctrl Pts',(-2.26224868442742,1.22558564702861,95.));
#39616=CARTESIAN_POINT('Ctrl Pts',(-2.27496506671204,1.20663684103107,95.));
#39617=CARTESIAN_POINT('Ctrl Pts',(-2.28743439477761,1.18751193473744,95.));
#39618=CARTESIAN_POINT('Ctrl Pts',(-2.29756668986916,1.17197146670692,95.));
#39619=CARTESIAN_POINT('Ctrl Pts',(-2.30753626837218,1.15631386661634,95.));
#39620=CARTESIAN_POINT('Ctrl Pts',(-2.317333768862,1.14055678391561,95.));
#39621=CARTESIAN_POINT('Ctrl Pts',(-2.36475924951746,1.06428353222387,95.));
#39622=CARTESIAN_POINT('Ctrl Pts',(-2.40820610202563,0.985606532640625,
95.));
#39623=CARTESIAN_POINT('Ctrl Pts',(-2.44763974844671,0.904917347557528,
95.));
#39624=CARTESIAN_POINT('Ctrl Pts',(-2.47963771154829,0.83944306857721,95.));
#39625=CARTESIAN_POINT('Ctrl Pts',(-2.50899276273707,0.772642817262913,
95.));
#39626=CARTESIAN_POINT('Ctrl Pts',(-2.53566897579507,0.70470769674724,95.));
#39627=CARTESIAN_POINT('Ctrl Pts',(-2.5438361703979,0.683908666974472,95.));
#39628=CARTESIAN_POINT('Ctrl Pts',(-2.55175214712428,0.663003164647788,
95.));
#39629=CARTESIAN_POINT('Ctrl Pts',(-2.55941554913515,0.641996437555638,
95.));
#39630=CARTESIAN_POINT('Ctrl Pts',(-2.56690183605693,0.621475213942943,
95.));
#39631=CARTESIAN_POINT('Ctrl Pts',(-2.5741486191131,0.600852476167031,95.));
#39632=CARTESIAN_POINT('Ctrl Pts',(-2.5811448836277,0.580162579357833,95.));
#39633=CARTESIAN_POINT('Ctrl Pts',(-2.61086044692886,0.492285407612116,
95.));
#39634=CARTESIAN_POINT('Ctrl Pts',(-2.63609351198065,0.403113198746262,
95.));
#39635=CARTESIAN_POINT('Ctrl Pts',(-2.65681095036009,0.313049768475568,
95.));
#39636=CARTESIAN_POINT('Ctrl Pts',(-2.67772663470034,0.222124517793465,
95.));
#39637=CARTESIAN_POINT('Ctrl Pts',(-2.69404032074682,0.130290065147494,
95.));
#39638=CARTESIAN_POINT('Ctrl Pts',(-2.70567605344102,0.0379287688478774,
95.));
#39639=CARTESIAN_POINT('Ctrl Pts',(-2.71722674145791,-0.0537574658251947,
95.));
#39640=CARTESIAN_POINT('Ctrl Pts',(-2.72416795527845,-0.145963797732815,
95.));
#39641=CARTESIAN_POINT('Ctrl Pts',(-2.72637845709328,-0.238335333551318,
95.));
#39642=CARTESIAN_POINT('Ctrl Pts',(-2.72748334696664,-0.284506014718901,
95.));
#39643=CARTESIAN_POINT('Ctrl Pts',(-2.72740556351808,-0.330718183947068,
95.));
#39644=CARTESIAN_POINT('Ctrl Pts',(-2.72612509839621,-0.376928226489462,
95.));
#39645=CARTESIAN_POINT('Ctrl Pts',(-2.72571336712059,-0.391786983231473,
95.));
#39646=CARTESIAN_POINT('Ctrl Pts',(-2.72517717633184,-0.406647371787764,
95.));
#39647=CARTESIAN_POINT('Ctrl Pts',(-2.72451604953527,-0.421502101712759,
95.));
#39648=CARTESIAN_POINT('Ctrl Pts',(-2.72025658293429,-0.517207231666559,
95.));
#39649=CARTESIAN_POINT('Ctrl Pts',(-2.71083095742351,-0.612346052400123,
95.));
#39650=CARTESIAN_POINT('Ctrl Pts',(-2.69617509433104,-0.706520494550697,
95.));
#39651=CARTESIAN_POINT('Ctrl Pts',(-2.69168471229759,-0.735374422864327,
95.));
#39652=CARTESIAN_POINT('Ctrl Pts',(-2.68670301102806,-0.764137972115757,
95.));
#39653=CARTESIAN_POINT('Ctrl Pts',(-2.6812272256085,-0.792800025397099,
95.));
#39654=CARTESIAN_POINT('Ctrl Pts',(-2.66406428539495,-0.882636472440427,
95.));
#39655=CARTESIAN_POINT('Ctrl Pts',(-2.6420515107896,-0.97147573332325,95.));
#39656=CARTESIAN_POINT('Ctrl Pts',(-2.61549087324854,-1.05908709780632,
95.));
#39657=CARTESIAN_POINT('Ctrl Pts',(-2.58823061274624,-1.14900619764259,
95.));
#39658=CARTESIAN_POINT('Ctrl Pts',(-2.55617956561799,-1.23763257002399,
95.));
#39659=CARTESIAN_POINT('Ctrl Pts',(-2.51960956826968,-1.3247127800465,95.));
#39660=CARTESIAN_POINT('Ctrl Pts',(-2.50475369780857,-1.36008747005534,
95.));
#39661=CARTESIAN_POINT('Ctrl Pts',(-2.48915149373411,-1.39520690037994,
95.));
#39662=CARTESIAN_POINT('Ctrl Pts',(-2.47281882090415,-1.43005347129214,
95.));
#39663=CARTESIAN_POINT('Ctrl Pts',(-2.46389555630005,-1.44909170073766,
95.));
#39664=CARTESIAN_POINT('Ctrl Pts',(-2.4547513259397,-1.46805407731575,94.9999999999999));
#39665=CARTESIAN_POINT('Ctrl Pts',(-2.44540417178415,-1.48690693831173,
94.9999999999999));
#39666=CARTESIAN_POINT('Ctrl Pts',(-2.40260336851074,-1.57323456073041,
94.9999999999999));
#39667=CARTESIAN_POINT('Ctrl Pts',(-2.35550976886648,-1.65736332426466,
94.9999999999999));
#39668=CARTESIAN_POINT('Ctrl Pts',(-2.30446753854991,-1.73904441047229,
94.9999999999999));
#39669=CARTESIAN_POINT('Ctrl Pts',(-2.25252507412462,-1.82216610966616,
94.9999999999999));
#39670=CARTESIAN_POINT('Ctrl Pts',(-2.19649313273819,-1.90275379234213,
94.9999999999999));
#39671=CARTESIAN_POINT('Ctrl Pts',(-2.13667978629767,-1.98053818479137,
94.9999999999999));
#39672=CARTESIAN_POINT('Ctrl Pts',(-2.07625803606746,-2.05911377723128,
94.9999999999999));
#39673=CARTESIAN_POINT('Ctrl Pts',(-2.01197711887089,-2.13482959939233,
94.9999999999999));
#39674=CARTESIAN_POINT('Ctrl Pts',(-1.94410535934088,-2.20738878038354,
94.9999999999999));
#39675=CARTESIAN_POINT('Ctrl Pts',(-1.89472368162325,-2.26018090064055,
94.9999999999999));
#39676=CARTESIAN_POINT('Ctrl Pts',(-1.84344008591747,-2.31130166154995,
94.9999999999999));
#39677=CARTESIAN_POINT('Ctrl Pts',(-1.79034391139651,-2.36062647407542,
94.9999999999999));
#39678=CARTESIAN_POINT('Ctrl Pts',(-1.77873832587776,-2.37140772781214,
94.9999999999999));
#39679=CARTESIAN_POINT('Ctrl Pts',(-1.76705130310331,-2.3820982531773,94.9999999999999));
#39680=CARTESIAN_POINT('Ctrl Pts',(-1.75528982662668,-2.39269177675974,
94.9999999999999));
#39681=CARTESIAN_POINT('Ctrl Pts',(-1.67945270486208,-2.46099802550614,
94.9999999999999));
#39682=CARTESIAN_POINT('Ctrl Pts',(-1.60045108818537,-2.52534093466199,
94.9999999999999));
#39683=CARTESIAN_POINT('Ctrl Pts',(-1.51861308701732,-2.58543865751991,
94.9999999999999));
#39684=CARTESIAN_POINT('Ctrl Pts',(-1.4367014765316,-2.6455904353683,95.));
#39685=CARTESIAN_POINT('Ctrl Pts',(-1.35194779658761,-2.70149022283026,
94.9999999999999));
#39686=CARTESIAN_POINT('Ctrl Pts',(-1.26463604590252,-2.75282922856233,
95.));
#39687=CARTESIAN_POINT('Ctrl Pts',(-1.17912004925445,-2.80311233716627,
95.));
#39688=CARTESIAN_POINT('Ctrl Pts',(-1.09114945513696,-2.84902100918829,
94.9999999999999));
#39689=CARTESIAN_POINT('Ctrl Pts',(-1.00095740892384,-2.89022906672385,
95.));
#39690=CARTESIAN_POINT('Ctrl Pts',(-0.958622435866522,-2.9095715927975,
95.));
#39691=CARTESIAN_POINT('Ctrl Pts',(-0.915797596451656,-2.92787787654872,
95.));
#39692=CARTESIAN_POINT('Ctrl Pts',(-0.872504988190697,-2.94511071874119,
95.));
#39693=CARTESIAN_POINT('Ctrl Pts',(-0.847139851648223,-2.95520743993184,
95.));
#39694=CARTESIAN_POINT('Ctrl Pts',(-0.821614117149488,-2.96493562401012,
94.9999999999999));
#39695=CARTESIAN_POINT('Ctrl Pts',(-0.795934819193142,-2.97429685620567,
94.9999999999999));
#39696=CARTESIAN_POINT('Ctrl Pts',(0.7937992825328,-2.96922295374571,95.));
#39697=CARTESIAN_POINT('Ctrl Pts',(0.889394081720711,-2.93425394918359,
95.));
#39698=CARTESIAN_POINT('Ctrl Pts',(0.982912280288356,-2.89421630604824,
95.));
#39699=CARTESIAN_POINT('Ctrl Pts',(1.07410729213453,-2.84943761375707,95.));
#39700=CARTESIAN_POINT('Ctrl Pts',(1.16513952621937,-2.80473884881213,95.));
#39701=CARTESIAN_POINT('Ctrl Pts',(1.25385743011116,-2.75531514973328,95.));
#39702=CARTESIAN_POINT('Ctrl Pts',(1.33998246484742,-2.70145265972436,95.));
#39703=CARTESIAN_POINT('Ctrl Pts',(1.36671560562667,-2.68473378660531,95.));
#39704=CARTESIAN_POINT('Ctrl Pts',(1.39319836634562,-2.66758719835479,95.));
#39705=CARTESIAN_POINT('Ctrl Pts',(1.41942255413576,-2.65002023451661,95.));
#39706=CARTESIAN_POINT('Ctrl Pts',(1.43652086410149,-2.63856648062858,95.));
#39707=CARTESIAN_POINT('Ctrl Pts',(1.45350887484186,-2.62693412288624,95.));
#39708=CARTESIAN_POINT('Ctrl Pts',(1.4703707131843,-2.61513499781576,95.));
#39709=CARTESIAN_POINT('Ctrl Pts',(1.55302591511012,-2.55729675708287,95.));
#39710=CARTESIAN_POINT('Ctrl Pts',(1.63273013133474,-2.49540305169935,95.));
#39711=CARTESIAN_POINT('Ctrl Pts',(1.70921781353368,-2.42975035881223,95.));
#39712=CARTESIAN_POINT('Ctrl Pts',(1.78531329212295,-2.36443431128283,95.));
#39713=CARTESIAN_POINT('Ctrl Pts',(1.85822565958198,-2.29539692708298,95.));
#39714=CARTESIAN_POINT('Ctrl Pts',(1.9276504475844,-2.22290249111416,95.));
#39715=CARTESIAN_POINT('Ctrl Pts',(1.94134566301126,-2.20860173562885,95.));
#39716=CARTESIAN_POINT('Ctrl Pts',(1.95490501326262,-2.1941663864582,95.));
#39717=CARTESIAN_POINT('Ctrl Pts',(1.96832593513303,-2.17959838567023,95.));
#39718=CARTESIAN_POINT('Ctrl Pts',(1.98260623147684,-2.16409756013845,95.));
#39719=CARTESIAN_POINT('Ctrl Pts',(1.99672372437399,-2.14845301269264,95.));
#39720=CARTESIAN_POINT('Ctrl Pts',(2.01066679948485,-2.13267784635066,95.));
#39721=CARTESIAN_POINT('Ctrl Pts',(2.07578057768892,-2.05900825236527,95.));
#39722=CARTESIAN_POINT('Ctrl Pts',(2.13715676450789,-1.98242441972866,95.));
#39723=CARTESIAN_POINT('Ctrl Pts',(2.194549598969,-1.9032011297646,95.));
#39724=CARTESIAN_POINT('Ctrl Pts',(2.25134918206036,-1.82479674560523,95.));
#39725=CARTESIAN_POINT('Ctrl Pts',(2.30424775307981,-1.7438064127902,94.9999999999999));
#39726=CARTESIAN_POINT('Ctrl Pts',(2.35296126981416,-1.66047518094658,94.9999999999999));
#39727=CARTESIAN_POINT('Ctrl Pts',(2.40036568860705,-1.5793833428355,94.9999999999999));
#39728=CARTESIAN_POINT('Ctrl Pts',(2.4438071815732,-1.49607404530473,95.));
#39729=CARTESIAN_POINT('Ctrl Pts',(2.48297596815033,-1.41076355819206,94.9999999999999));
#39730=CARTESIAN_POINT('Ctrl Pts',(2.50148013223893,-1.37046107782537,94.9999999999999));
#39731=CARTESIAN_POINT('Ctrl Pts',(2.51902998170372,-1.32971189089598,94.9999999999999));
#39732=CARTESIAN_POINT('Ctrl Pts',(2.53558876169176,-1.28853867411852,94.9999999999999));
#39733=CARTESIAN_POINT('Ctrl Pts',(2.54347893045625,-1.26891985985895,94.9999999999999));
#39734=CARTESIAN_POINT('Ctrl Pts',(2.55114403973676,-1.24920477206754,95.));
#39735=CARTESIAN_POINT('Ctrl Pts',(2.55857988947091,-1.22939587775288,95.));
#39736=CARTESIAN_POINT('Ctrl Pts',(2.56375525722037,-1.21560884379528,95.));
#39737=CARTESIAN_POINT('Ctrl Pts',(2.56881605398952,-1.20178568693359,95.));
#39738=CARTESIAN_POINT('Ctrl Pts',(2.57376064275323,-1.18792929888989,95.));
#39739=CARTESIAN_POINT('Ctrl Pts',(2.6049580470237,-1.10050375954049,95.));
#39740=CARTESIAN_POINT('Ctrl Pts',(2.63154314967493,-1.01173042098719,94.9999999999999));
#39741=CARTESIAN_POINT('Ctrl Pts',(2.65326289575206,-0.921831545713812,
94.9999999999999));
#39742=CARTESIAN_POINT('Ctrl Pts',(2.65761145312367,-0.903832697321139,
94.9999999999999));
#39743=CARTESIAN_POINT('Ctrl Pts',(2.66176481894967,-0.885788701871771,
95.));
#39744=CARTESIAN_POINT('Ctrl Pts',(2.66572071053984,-0.867701306572206,
95.));
#39745=CARTESIAN_POINT('Ctrl Pts',(2.68630633473123,-0.773578322220572,
95.));
#39746=CARTESIAN_POINT('Ctrl Pts',(2.70154908258618,-0.678279708787185,
95.));
#39747=CARTESIAN_POINT('Ctrl Pts',(2.71156683220905,-0.582225910335545,
95.));
#39748=CARTESIAN_POINT('Ctrl Pts',(2.72158458183192,-0.486172111883905,
95.));
#39749=CARTESIAN_POINT('Ctrl Pts',(2.72637692884362,-0.389362032339101,
95.));
#39750=CARTESIAN_POINT('Ctrl Pts',(2.72600772437218,-0.292230486803331,
95.));
#39751=CARTESIAN_POINT('Ctrl Pts',(2.72587933530249,-0.258453461515866,
95.));
#39752=CARTESIAN_POINT('Ctrl Pts',(2.725126326345,-0.224637766094994,95.));
#39753=CARTESIAN_POINT('Ctrl Pts',(2.72374998821602,-0.190802465141519,
95.));
#39754=CARTESIAN_POINT('Ctrl Pts',(2.72314858458174,-0.17601781845347,95.));
#39755=CARTESIAN_POINT('Ctrl Pts',(2.72242803550975,-0.161228600798757,
95.));
#39756=CARTESIAN_POINT('Ctrl Pts',(2.72158956888809,-0.146452928724579,
95.));
#39757=CARTESIAN_POINT('Ctrl Pts',(2.71631906770851,-0.0535748163660937,
95.));
#39758=CARTESIAN_POINT('Ctrl Pts',(2.7063884100378,0.0389231339706655,95.));
#39759=CARTESIAN_POINT('Ctrl Pts',(2.69192307739847,0.130668782477267,95.));
#39760=CARTESIAN_POINT('Ctrl Pts',(2.67747069981536,0.222332264187943,95.));
#39761=CARTESIAN_POINT('Ctrl Pts',(2.6584913618998,0.313245746507116,95.0000000000001));
#39762=CARTESIAN_POINT('Ctrl Pts',(2.63506128485434,0.403021048770596,95.0000000000001));
#39763=CARTESIAN_POINT('Ctrl Pts',(2.61213349833566,0.490871761380415,95.0000000000001));
#39764=CARTESIAN_POINT('Ctrl Pts',(2.58494325798982,0.577633328616342,95.0000000000001));
#39765=CARTESIAN_POINT('Ctrl Pts',(2.55352200789815,0.662913185460221,95.0000000000001));
#39766=CARTESIAN_POINT('Ctrl Pts',(2.53742751811359,0.706594954352263,95.0000000000001));
#39767=CARTESIAN_POINT('Ctrl Pts',(2.52022234983568,0.749887433972256,95.0000000000001));
#39768=CARTESIAN_POINT('Ctrl Pts',(2.50190715230985,0.792733884454138,95.0000000000001));
#39769=CARTESIAN_POINT('Ctrl Pts',(2.49657565883769,0.80520634459154,95.0000000000001));
#39770=CARTESIAN_POINT('Ctrl Pts',(2.49115008979521,0.817640989633295,95.0000000000001));
#39771=CARTESIAN_POINT('Ctrl Pts',(2.48563042562688,0.830036369593218,95.0000000000001));
#39772=CARTESIAN_POINT('Ctrl Pts',(2.47997189811484,0.84274359169704,95.0000000000001));
#39773=CARTESIAN_POINT('Ctrl Pts',(2.47421802933406,0.855401541926264,95.0000000000001));
#39774=CARTESIAN_POINT('Ctrl Pts',(2.4683704650422,0.868006079871034,95.0000000000001));
#39775=CARTESIAN_POINT('Ctrl Pts',(2.43080699529853,0.948974865520953,95.0000000000001));
#39776=CARTESIAN_POINT('Ctrl Pts',(2.38936345000638,1.02778052674691,95.0000000000001));
#39777=CARTESIAN_POINT('Ctrl Pts',(2.34411176247456,1.10407309709342,95.0000000000001));
#39778=CARTESIAN_POINT('Ctrl Pts',(2.30016849871569,1.17815971627689,95.0000000000001));
#39779=CARTESIAN_POINT('Ctrl Pts',(2.25263361346913,1.24987705073289,95.0000000000001));
#39780=CARTESIAN_POINT('Ctrl Pts',(2.20153811786332,1.31887168138104,95.0000000000001));
#39781=CARTESIAN_POINT('Ctrl Pts',(2.15104877950881,1.38704781334994,95.0000000000001));
#39782=CARTESIAN_POINT('Ctrl Pts',(2.09708244939439,1.45256603784657,95.0000000000001));
#39783=CARTESIAN_POINT('Ctrl Pts',(2.03964076081768,1.51504411883957,95.0000000000001));
#39784=CARTESIAN_POINT('Ctrl Pts',(2.01565998812739,1.5411274860863,95.0000000000001));
#39785=CARTESIAN_POINT('Ctrl Pts',(1.99107318468021,1.56668043915507,95.0000000000001));
#39786=CARTESIAN_POINT('Ctrl Pts',(1.96587920978157,1.59167263744915,95.0000000000001));
#39787=CARTESIAN_POINT('Ctrl Pts',(1.94985907681406,1.60756446640559,95.0000000000001));
#39788=CARTESIAN_POINT('Ctrl Pts',(1.93359342372445,1.62322952717531,95.0000000000001));
#39789=CARTESIAN_POINT('Ctrl Pts',(1.91708817308061,1.63866486770395,95.0000000000001));
#39790=CARTESIAN_POINT('Ctrl Pts',(1.90919204567957,1.63405297314213,113.997481789454));
#39791=CARTESIAN_POINT('Ctrl Pts',(2.45150048983647,1.00048419650343,113.944664556026));
#39792=CARTESIAN_POINT('Ctrl Pts',(2.84607223516907,-0.837858370588297,
113.839057686671));
#39793=CARTESIAN_POINT('Ctrl Pts',(0.84317678352709,-2.84731406332924,113.680661181388));
#39794=CARTESIAN_POINT('Ctrl Pts',(-1.92777411460126,-2.25549477905844,
113.522292273603));
#39795=CARTESIAN_POINT('Ctrl Pts',(-2.94220166301464,0.387995676951446,
113.363923365819));
#39796=CARTESIAN_POINT('Ctrl Pts',(-1.27606983691641,2.67964581640148,113.205554458035));
#39797=CARTESIAN_POINT('Ctrl Pts',(1.55272161995431,2.5290395279534,113.047185550251));
#39798=CARTESIAN_POINT('Ctrl Pts',(2.96681482889055,0.0746577552526638,
112.888816642467));
#39799=CARTESIAN_POINT('Ctrl Pts',(1.6778616323001,-2.44795918144571,112.730447734683));
#39800=CARTESIAN_POINT('Ctrl Pts',(-1.13979077436967,-2.74013955134929,
112.572078826898));
#39801=CARTESIAN_POINT('Ctrl Pts',(-2.91898098009258,-0.535842258547723,
112.413709919114));
#39802=CARTESIAN_POINT('Ctrl Pts',(-2.0386979343972,2.15668702450009,112.25534101133));
#39803=CARTESIAN_POINT('Ctrl Pts',(0.699037044459727,2.88425144150759,112.096972103546));
#39804=CARTESIAN_POINT('Ctrl Pts',(2.79988124597661,0.983990481949177,111.938603195762));
#39805=CARTESIAN_POINT('Ctrl Pts',(2.34976254180504,-1.81278472818317,111.780234287978));
#39806=CARTESIAN_POINT('Ctrl Pts',(-0.241217557004296,-2.95793561405378,
111.621865380193));
#39807=CARTESIAN_POINT('Ctrl Pts',(-2.6124250528005,-1.40812151641157,111.463496472409));
#39808=CARTESIAN_POINT('Ctrl Pts',(-2.60346025937764,1.42462816365992,111.305127564625));
#39809=CARTESIAN_POINT('Ctrl Pts',(-0.2224909416266,2.9594033363853,111.146758656841));
#39810=CARTESIAN_POINT('Ctrl Pts',(2.36118917324051,1.7978754877943,110.988389749057));
#39811=CARTESIAN_POINT('Ctrl Pts',(2.79359720679656,-1.00169116479646,110.830020841272));
#39812=CARTESIAN_POINT('Ctrl Pts',(0.680767545745605,-2.88862009406214,
110.671651933488));
#39813=CARTESIAN_POINT('Ctrl Pts',(-2.05230730015675,-2.14373628951773,
110.513283025704));
#39814=CARTESIAN_POINT('Ctrl Pts',(-2.91553137268672,0.554298963281664,
110.35491411792));
#39815=CARTESIAN_POINT('Ctrl Pts',(-1.12242391390563,2.74731415726134,110.196545210136));
#39816=CARTESIAN_POINT('Ctrl Pts',(1.69332046845399,2.43726000187965,110.038176302352));
#39817=CARTESIAN_POINT('Ctrl Pts',(2.9662858587266,-0.0933741329074965,
109.879807394567));
#39818=CARTESIAN_POINT('Ctrl Pts',(1.53667746406551,-2.53893538621435,109.721438486783));
#39819=CARTESIAN_POINT('Ctrl Pts',(-1.29299297046839,-2.67128053615198,
109.563069578999));
#39820=CARTESIAN_POINT('Ctrl Pts',(-2.94462154643842,-0.369830329415952,
109.404700671215));
#39821=CARTESIAN_POINT('Ctrl Pts',(-1.9134146247821,2.26857113574608,109.246331763431));
#39822=CARTESIAN_POINT('Ctrl Pts',(0.86109838768306,2.84008452181803,109.087962855647));
#39823=CARTESIAN_POINT('Ctrl Pts',(2.85106734754679,0.824005767008581,108.929593947862));
#39824=CARTESIAN_POINT('Ctrl Pts',(2.24343774831338,-1.94282206950403,108.771225040078));
#39825=CARTESIAN_POINT('Ctrl Pts',(-0.408180979221735,-2.93955078413682,
108.612856132294));
#39826=CARTESIAN_POINT('Ctrl Pts',(-2.68790729096064,-1.25806395684563,
108.45448722451));
#39827=CARTESIAN_POINT('Ctrl Pts',(-2.51868966176006,1.56964101375337,108.296118316726));
#39828=CARTESIAN_POINT('Ctrl Pts',(-0.0547017452741313,2.96725095726307,
108.137749408941));
#39829=CARTESIAN_POINT('Ctrl Pts',(2.45912476054798,1.66140781759745,107.979380501157));
#39830=CARTESIAN_POINT('Ctrl Pts',(2.73245037461282,-1.15813879763718,107.821011593373));
#39831=CARTESIAN_POINT('Ctrl Pts',(0.51624898328965,-2.92250877014367,107.662642685589));
#39832=CARTESIAN_POINT('Ctrl Pts',(-2.1703052449394,-2.02419012647102,107.504273777805));
#39833=CARTESIAN_POINT('Ctrl Pts',(-2.87950114036526,0.718361821750989,
107.345904870021));
#39834=CARTESIAN_POINT('Ctrl Pts',(-0.965192536829941,2.80641655695694,
107.187535962237));
#39835=CARTESIAN_POINT('Ctrl Pts',(1.82849997360527,2.33755392896929,107.029167054452));
#39836=CARTESIAN_POINT('Ctrl Pts',(2.95625186680727,-0.261046785677825,
106.870798146668));
#39837=CARTESIAN_POINT('Ctrl Pts',(1.39057191380851,-2.62180858890217,106.712429238884));
#39838=CARTESIAN_POINT('Ctrl Pts',(-1.44205376838795,-2.59384877226725,
106.5540603311));
#39839=CARTESIAN_POINT('Ctrl Pts',(-2.96082876440973,-0.202641437416436,
106.395691423316));
#39840=CARTESIAN_POINT('Ctrl Pts',(-1.78200191711455,2.37319187840222,106.237322515531));
#39841=CARTESIAN_POINT('Ctrl Pts',(1.02040131331566,2.78681748309749,106.078953607747));
#39842=CARTESIAN_POINT('Ctrl Pts',(2.89312009295593,0.661382379602711,105.920584699963));
#39843=CARTESIAN_POINT('Ctrl Pts',(2.12992618844909,-2.0666361450611,105.762215792179));
#39844=CARTESIAN_POINT('Ctrl Pts',(-0.573836816559167,-2.91174893015787,
105.603846884395));
#39845=CARTESIAN_POINT('Ctrl Pts',(-2.75477888956335,-1.10397635569352,
105.44547797661));
#39846=CARTESIAN_POINT('Ctrl Pts',(-2.42585051691946,1.7096256297435,105.287109068826));
#39847=CARTESIAN_POINT('Ctrl Pts',(0.113262687996535,2.96559304150486,105.128740161042));
#39848=CARTESIAN_POINT('Ctrl Pts',(2.54918261149376,1.51961789196234,104.970371253258));
#39849=CARTESIAN_POINT('Ctrl Pts',(2.66255021640461,-1.31087637458229,104.812002345474));
#39850=CARTESIAN_POINT('Ctrl Pts',(0.350076631837247,-2.94703526890258,
104.65363343769));
#39851=CARTESIAN_POINT('Ctrl Pts',(-2.28135067903068,-1.89815953059813,
104.495264529906));
#39852=CARTESIAN_POINT('Ctrl Pts',(-2.83424650878728,0.880123429833188,
104.336895622121));
#39853=CARTESIAN_POINT('Ctrl Pts',(-0.804869193124953,2.85652868115701,
104.178526714337));
#39854=CARTESIAN_POINT('Ctrl Pts',(1.95782193152955,2.23035956938251,104.020157806553));
#39855=CARTESIAN_POINT('Ctrl Pts',(2.93674760683921,-0.427883182701047,
103.861788898769));
#39856=CARTESIAN_POINT('Ctrl Pts',(1.24001170631118,-2.69628290291013,103.703419990985));
#39857=CARTESIAN_POINT('Ctrl Pts',(-1.58649498842436,-2.50810768828187,
103.5450510832));
#39858=CARTESIAN_POINT('Ctrl Pts',(-2.96755105236673,-0.0348033893664811,
103.386682175416));
#39859=CARTESIAN_POINT('Ctrl Pts',(-1.64488061742202,2.47021016894182,103.228313267632));
#39860=CARTESIAN_POINT('Ctrl Pts',(1.17643541261118,2.72462295451473,103.069944359848));
#39861=CARTESIAN_POINT('Ctrl Pts',(2.92590481113682,0.496640272713199,102.911575452064));
#39862=CARTESIAN_POINT('Ctrl Pts',(2.00959147113718,-2.18382981100793,102.75320654428));
#39863=CARTESIAN_POINT('Ctrl Pts',(-0.737654384115308,-2.87461937200557,
102.594837636495));
#39864=CARTESIAN_POINT('Ctrl Pts',(-2.81282563301446,-0.946352197953286,
102.436468728711));
#39865=CARTESIAN_POINT('Ctrl Pts',(-2.32524022953366,1.84413350906936,102.278099820927));
#39866=CARTESIAN_POINT('Ctrl Pts',(0.280864287495135,2.95443493350659,102.119730913143));
#39867=CARTESIAN_POINT('Ctrl Pts',(2.63107422906718,1.37295991400069,101.961362005359));
#39868=CARTESIAN_POINT('Ctrl Pts',(2.58412065495367,-1.45941459666404,101.802993097575));
#39869=CARTESIAN_POINT('Ctrl Pts',(0.182782819936727,-2.96212102471358,
101.64462418979));
#39870=CARTESIAN_POINT('Ctrl Pts',(-2.38508787166244,-1.76604823511788,
101.486255282006));
#39871=CARTESIAN_POINT('Ctrl Pts',(-2.77991244981906,1.03906558775433,101.327886374222));
#39872=CARTESIAN_POINT('Ctrl Pts',(-0.641967474047549,2.89748999766681,
101.169517466438));
#39873=CARTESIAN_POINT('Ctrl Pts',(2.08087206305652,2.1160203168933,101.011148558654));
#39874=CARTESIAN_POINT('Ctrl Pts',(2.90783556015353,-0.593348868222388,
100.852779650869));
#39875=CARTESIAN_POINT('Ctrl Pts',(1.08547915688257,-2.76211975198173,100.694410743085));
#39876=CARTESIAN_POINT('Ctrl Pts',(-1.72585391727417,-2.41433195326245,
100.536041835301));
#39877=CARTESIAN_POINT('Ctrl Pts',(-2.96476687565186,0.133146150343083,
100.377672927517));
#39878=CARTESIAN_POINT('Ctrl Pts',(-1.50248998985534,2.55931521206319,100.219304019733));
#39879=CARTESIAN_POINT('Ctrl Pts',(1.32870083480892,2.65370017445376,100.060935111949));
#39880=CARTESIAN_POINT('Ctrl Pts',(2.94931647718439,0.330307192955261,99.9025662041639));
#39881=CARTESIAN_POINT('Ctrl Pts',(1.88281908519425,-2.29402764079667,99.7441972963799));
#39882=CARTESIAN_POINT('Ctrl Pts',(-0.899108897014456,-2.82828105315757,
99.5858283885955));
#39883=CARTESIAN_POINT('Ctrl Pts',(-2.86186157023077,-0.785696428085674,
99.4274594808116));
#39884=CARTESIAN_POINT('Ctrl Pts',(-2.21718110178343,1.97273375958331,99.2690905730271));
#39885=CARTESIAN_POINT('Ctrl Pts',(0.447566146327358,2.93381237797627,99.1107216652432));
#39886=CARTESIAN_POINT('Ctrl Pts',(2.70453727577697,1.22190369828033,98.9523527574589));
#39887=CARTESIAN_POINT('Ctrl Pts',(2.49741293719626,-1.60327762583477,98.7939838496747));
#39888=CARTESIAN_POINT('Ctrl Pts',(0.0149034683458423,-2.96771771101614,
98.6356149418906));
#39889=CARTESIAN_POINT('Ctrl Pts',(-2.48118450337799,-1.62827945432984,
98.4772460341062));
#39890=CARTESIAN_POINT('Ctrl Pts',(-2.71667302172388,1.19467912798932,98.3188771263223));
#39891=CARTESIAN_POINT('Ctrl Pts',(-0.477009229269139,2.92916928982671,
98.1605082185381));
#39892=CARTESIAN_POINT('Ctrl Pts',(2.19725617802395,1.99490245057136,98.0021393107537));
#39893=CARTESIAN_POINT('Ctrl Pts',(2.86960835079419,-0.756913770851785,
97.8437704029698));
#39894=CARTESIAN_POINT('Ctrl Pts',(0.927469295965859,-2.81910824312945,
97.6854014951854));
#39895=CARTESIAN_POINT('Ctrl Pts',(-1.85968410254603,-2.31282194845431,
97.5270325874014));
#39896=CARTESIAN_POINT('Ctrl Pts',(-2.9524851929573,0.30066910752466,97.3686636796171));
#39897=CARTESIAN_POINT('Ctrl Pts',(-1.35528610028854,2.64022166642226,97.210294771833));
#39898=CARTESIAN_POINT('Ctrl Pts',(1.47670964695599,2.57427613617538,97.0519258640487));
#39899=CARTESIAN_POINT('Ctrl Pts',(2.96328039903411,0.162916390533464,96.8935569562647));
#39900=CARTESIAN_POINT('Ctrl Pts',(1.7500145362593,-2.39687742344476,96.7351880484805));
#39901=CARTESIAN_POINT('Ctrl Pts',(-1.05768194208838,-2.77288082627902,
96.5768191406962));
#39902=CARTESIAN_POINT('Ctrl Pts',(-2.90173198512928,-0.62252684748547,
96.4184502329122));
#39903=CARTESIAN_POINT('Ctrl Pts',(-2.10201461388728,2.09502063264114,96.2600813251278));
#39904=CARTESIAN_POINT('Ctrl Pts',(0.612824978782371,2.90377914373446,96.1017124173438));
#39905=CARTESIAN_POINT('Ctrl Pts',(2.76935472527221,1.06695745781245,95.9433435095596));
#39906=CARTESIAN_POINT('Ctrl Pts',(2.40266862666488,-1.74205266274717,95.7849746017753));
#39907=CARTESIAN_POINT('Ctrl Pts',(-0.152952049520368,-2.96371237362396,
95.6266056939912));
#39908=CARTESIAN_POINT('Ctrl Pts',(-2.56947425079852,-1.48548241474925,
95.4682367862071));
#39909=CARTESIAN_POINT('Ctrl Pts',(-2.64445097587162,1.34683714954358,95.3098678784228));
#39910=CARTESIAN_POINT('Ctrl Pts',(-0.311076541356304,2.95072891345583,
95.1514989706387));
#39911=CARTESIAN_POINT('Ctrl Pts',(2.30770049687633,1.86886673688316,94.9931300628545));
#39912=CARTESIAN_POINT('Ctrl Pts',(2.81996216194598,-0.921166536179545,
94.8347611550703));
#39913=CARTESIAN_POINT('Ctrl Pts',(1.45428462117612,-2.21245757983627,94.7291818832142));
#39914=CARTESIAN_POINT('Ctrl Pts',(0.649036464259029,-2.42773457963693,
94.6763922472862));
#39915=CARTESIAN_POINT('Ctrl Pts',(2.0520964948903,1.75636305747151,114.106081112791));
#39916=CARTESIAN_POINT('Ctrl Pts',(2.63499713074943,1.07537118514814,114.053263879364));
#39917=CARTESIAN_POINT('Ctrl Pts',(3.0591028656398,-0.900572694815907,113.947657010009));
#39918=CARTESIAN_POINT('Ctrl Pts',(0.906289194931637,-3.06043764556437,
113.789260504724));
#39919=CARTESIAN_POINT('Ctrl Pts',(-2.07206944553626,-2.42432024626506,
113.63089159694));
#39920=CARTESIAN_POINT('Ctrl Pts',(-3.162427652889,0.417037442883985,113.472522689156));
#39921=CARTESIAN_POINT('Ctrl Pts',(-1.37158461638119,2.8802193052442,113.314153781372));
#39922=CARTESIAN_POINT('Ctrl Pts',(1.66894399181015,2.71834002372711,113.155784873588));
#39923=CARTESIAN_POINT('Ctrl Pts',(3.18888313259644,0.0802459439410872,
112.997415965804));
#39924=CARTESIAN_POINT('Ctrl Pts',(1.80345082745639,-2.63119075278318,112.839047058019));
#39925=CARTESIAN_POINT('Ctrl Pts',(-1.22510496431476,-2.94524104139177,
112.680678150235));
#39926=CARTESIAN_POINT('Ctrl Pts',(-3.13746888452353,-0.575950451432188,
112.522309242451));
#39927=CARTESIAN_POINT('Ctrl Pts',(-2.19129599601253,2.31811665755014,112.363940334667));
#39928=CARTESIAN_POINT('Ctrl Pts',(0.751360488841596,3.10013981406113,112.205571426883));
#39929=CARTESIAN_POINT('Ctrl Pts',(3.00945444643971,1.05764290375229,112.047202519098));
#39930=CARTESIAN_POINT('Ctrl Pts',(2.52564402139353,-1.94847301774256,111.888833611314));
#39931=CARTESIAN_POINT('Ctrl Pts',(-0.259272871136612,-3.17933930190371,
111.73046470353));
#39932=CARTESIAN_POINT('Ctrl Pts',(-2.80796701732922,-1.51352046262023,
111.572095795746));
#39933=CARTESIAN_POINT('Ctrl Pts',(-2.79833120242936,1.53126264473197,111.413726887962));
#39934=CARTESIAN_POINT('Ctrl Pts',(-0.239144554624559,3.18091688434692,
111.255357980177));
#39935=CARTESIAN_POINT('Ctrl Pts',(2.5379259447182,1.93244780958568,111.096989072394));
#39936=CARTESIAN_POINT('Ctrl Pts',(3.00270004223804,-1.0766684959185,110.938620164609));
#39937=CARTESIAN_POINT('Ctrl Pts',(0.731723504516477,-3.10483546351917,
110.780251256825));
#39938=CARTESIAN_POINT('Ctrl Pts',(-2.20592403295415,-2.30419655039083,
110.621882349041));
#39939=CARTESIAN_POINT('Ctrl Pts',(-3.13376107142933,0.595788654287395,
110.463513441257));
#39940=CARTESIAN_POINT('Ctrl Pts',(-1.20643818138628,2.95295267190985,110.305144533473));
#39941=CARTESIAN_POINT('Ctrl Pts',(1.82006676903139,2.61969073164313,110.146775625688));
#39942=CARTESIAN_POINT('Ctrl Pts',(3.18831456862103,-0.100363256429076,
109.988406717904));
#39943=CARTESIAN_POINT('Ctrl Pts',(1.65169891888132,-2.72897659436294,109.83003781012));
#39944=CARTESIAN_POINT('Ctrl Pts',(-1.38977445910716,-2.87122787752605,
109.671668902336));
#39945=CARTESIAN_POINT('Ctrl Pts',(-3.1650286663927,-0.397512405530931,
109.513299994552));
#39946=CARTESIAN_POINT('Ctrl Pts',(-2.05663513718945,2.43837537800804,109.354931086767));
#39947=CARTESIAN_POINT('Ctrl Pts',(0.92555224453134,3.05266696747654,109.196562178983));
#39948=CARTESIAN_POINT('Ctrl Pts',(3.06447186590621,0.885683213521782,109.038193271199));
#39949=CARTESIAN_POINT('Ctrl Pts',(2.41136073777209,-2.08824375109192,108.879824363415));
#39950=CARTESIAN_POINT('Ctrl Pts',(-0.438733630090977,-3.15957835374916,
108.721455455631));
#39951=CARTESIAN_POINT('Ctrl Pts',(-2.88909915733862,-1.35223098275157,
108.563086547847));
#39952=CARTESIAN_POINT('Ctrl Pts',(-2.70721546232639,1.6871298148599,108.404717640063));
#39953=CARTESIAN_POINT('Ctrl Pts',(-0.0587962117249828,3.1893519055031,
108.246348732278));
#39954=CARTESIAN_POINT('Ctrl Pts',(2.64319208381275,1.78576543244581,108.087979824494));
#39955=CARTESIAN_POINT('Ctrl Pts',(2.93697632403909,-1.24482635081468,107.92961091671));
#39956=CARTESIAN_POINT('Ctrl Pts',(0.554890604901032,-3.14126073229229,
107.771242008926));
#39957=CARTESIAN_POINT('Ctrl Pts',(-2.33275421195092,-2.17570226783771,
107.612873101142));
#39958=CARTESIAN_POINT('Ctrl Pts',(-3.09503394933374,0.772131740132777,
107.454504193357));
#39959=CARTESIAN_POINT('Ctrl Pts',(-1.03743791841433,3.0164789303234,107.296135285573));
#39960=CARTESIAN_POINT('Ctrl Pts',(1.96536456101083,2.51252158477725,107.137766377789));
#39961=CARTESIAN_POINT('Ctrl Pts',(3.17752952491941,-0.280586332372429,
106.979397470005));
#39962=CARTESIAN_POINT('Ctrl Pts',(1.49465725916726,-2.81805291810986,106.821028562221));
#39963=CARTESIAN_POINT('Ctrl Pts',(-1.54999256897645,-2.7880002883369,106.662659654437));
#39964=CARTESIAN_POINT('Ctrl Pts',(-3.18244900672259,-0.217809300213058,
106.504290746652));
#39965=CARTESIAN_POINT('Ctrl Pts',(-1.91538609029609,2.5508270613174,106.345921838868));
#39966=CARTESIAN_POINT('Ctrl Pts',(1.09677911301541,2.99541285116125,106.187552931084));
#39967=CARTESIAN_POINT('Ctrl Pts',(3.10967229068793,0.710887344223057,106.0291840233));
#39968=CARTESIAN_POINT('Ctrl Pts',(2.28935275295246,-2.22132540259141,105.870815115516));
#39969=CARTESIAN_POINT('Ctrl Pts',(-0.616788930461382,-3.12969551025482,
105.712446207732));
#39970=CARTESIAN_POINT('Ctrl Pts',(-2.96097614499467,-1.18660980967688,
105.554077299947));
#39971=CARTESIAN_POINT('Ctrl Pts',(-2.6074272382202,1.83759238380993,105.395708392163));
#39972=CARTESIAN_POINT('Ctrl Pts',(0.121740484706877,3.18756989351327,105.237339484379));
#39973=CARTESIAN_POINT('Ctrl Pts',(2.73999083210073,1.6333624250768,105.078970576595));
#39974=CARTESIAN_POINT('Ctrl Pts',(2.86184408683125,-1.40899644936311,104.920601668811));
#39975=CARTESIAN_POINT('Ctrl Pts',(0.376280128948743,-3.16762305778437,
104.762232761026));
#39976=CARTESIAN_POINT('Ctrl Pts',(-2.45211147964326,-2.04023818782284,
104.603863853242));
#39977=CARTESIAN_POINT('Ctrl Pts',(-3.04639197481427,0.946001325282417,
104.445494945458));
#39978=CARTESIAN_POINT('Ctrl Pts',(-0.86511425280373,3.07034198441227,104.287126037674));
#39979=CARTESIAN_POINT('Ctrl Pts',(2.10436636398257,2.39730364738964,104.12875712989));
#39980=CARTESIAN_POINT('Ctrl Pts',(3.15656535653917,-0.459910558202012,
103.970388222106));
#39981=CARTESIAN_POINT('Ctrl Pts',(1.33282750779448,-2.8981016900922,103.812019314321));
#39982=CARTESIAN_POINT('Ctrl Pts',(-1.70524532211103,-2.69584142023735,
103.653650406537));
#39983=CARTESIAN_POINT('Ctrl Pts',(-3.18967446294917,-0.037408449029986,
103.495281498753));
#39984=CARTESIAN_POINT('Ctrl Pts',(-1.76800115900506,2.65510724329652,103.336912590969));
#39985=CARTESIAN_POINT('Ctrl Pts',(1.26449248107197,2.92856301570605,103.178543683185));
#39986=CARTESIAN_POINT('Ctrl Pts',(3.14491096948782,0.533814167706403,103.020174775401));
#39987=CARTESIAN_POINT('Ctrl Pts',(2.16001089225898,-2.34729110188136,102.861805867616));
#39988=CARTESIAN_POINT('Ctrl Pts',(-0.792868365185695,-3.08978677696968,
102.703436959832));
#39989=CARTESIAN_POINT('Ctrl Pts',(-3.02336773050613,-1.01718736611457,
102.545068052048));
#39990=CARTESIAN_POINT('Ctrl Pts',(-2.49928619575068,1.98216827826976,102.386699144264));
#39991=CARTESIAN_POINT('Ctrl Pts',(0.301887188988093,3.17557659280544,102.22833023648));
#39992=CARTESIAN_POINT('Ctrl Pts',(2.82801209835501,1.47572698803218,102.069961328695));
#39993=CARTESIAN_POINT('Ctrl Pts',(2.77754401418352,-1.56865286820322,101.911592420911));
#39994=CARTESIAN_POINT('Ctrl Pts',(0.196464250396984,-3.18383799367443,
101.753223513127));
#39995=CARTESIAN_POINT('Ctrl Pts',(-2.56361347854963,-1.89823826329772,
101.594854605343));
#39996=CARTESIAN_POINT('Ctrl Pts',(-2.98799097098955,1.11684042232264,101.436485697559));
#39997=CARTESIAN_POINT('Ctrl Pts',(-0.690019218500169,3.11436928602715,
101.278116789774));
#39998=CARTESIAN_POINT('Ctrl Pts',(2.23662688967128,2.2744060165345,101.119747881991));
#39999=CARTESIAN_POINT('Ctrl Pts',(3.1254892215856,-0.637761473751003,100.961378974206));
#40000=CARTESIAN_POINT('Ctrl Pts',(1.16672808173278,-2.96886647644263,100.803010066422));
#40001=CARTESIAN_POINT('Ctrl Pts',(-1.85503537077141,-2.59504650147861,
100.644641158638));
#40002=CARTESIAN_POINT('Ctrl Pts',(-3.18668188852971,0.143112239046609,
100.486272250854));
#40003=CARTESIAN_POINT('Ctrl Pts',(-1.61495248671667,2.75088186538348,100.327903343069));
#40004=CARTESIAN_POINT('Ctrl Pts',(1.42815508373788,2.8523316126367,100.169534435285));
#40005=CARTESIAN_POINT('Ctrl Pts',(3.17007501620824,0.355030932814977,100.011165527501));
#40006=CARTESIAN_POINT('Ctrl Pts',(2.02374949863382,-2.46573732145668,99.8527966197172));
#40007=CARTESIAN_POINT('Ctrl Pts',(-0.966407868848687,-3.0399800003794,
99.694427711933));
#40008=CARTESIAN_POINT('Ctrl Pts',(-3.07607404421248,-0.844506391995024,
99.5360588041488));
#40009=CARTESIAN_POINT('Ctrl Pts',(-2.38313876165731,2.120394353493,99.3776898963646));
#40010=CARTESIAN_POINT('Ctrl Pts',(0.48106680634269,3.15341042360563,99.2193209885805));
#40011=CARTESIAN_POINT('Ctrl Pts',(2.90697390892733,1.31336410185077,99.0609520807963));
#40012=CARTESIAN_POINT('Ctrl Pts',(2.68434615905282,-1.72328415245439,98.9025831730122));
#40013=CARTESIAN_POINT('Ctrl Pts',(0.0160190040721257,-3.18985359612286,
98.7442142652279));
#40014=CARTESIAN_POINT('Ctrl Pts',(-2.66690301485401,-1.75015738646807,
98.5858453574439));
#40015=CARTESIAN_POINT('Ctrl Pts',(-2.92001802451376,1.28410175215917,98.4274764496595));
#40016=CARTESIAN_POINT('Ctrl Pts',(-0.512713726012357,3.14841979684353,
98.2691075418755));
#40017=CARTESIAN_POINT('Ctrl Pts',(2.36172244248695,2.14422238754322,98.1107386340912));
#40018=CARTESIAN_POINT('Ctrl Pts',(3.08440067708151,-0.813569331390272,
97.9523697263072));
#40019=CARTESIAN_POINT('Ctrl Pts',(0.996891064823428,-3.03012059867614,
97.7940008185227));
#40020=CARTESIAN_POINT('Ctrl Pts',(-1.99888284527162,-2.48593839706633,
97.6356319107388));
#40021=CARTESIAN_POINT('Ctrl Pts',(-3.17348091272117,0.323174414574692,
97.4772630029545));
#40022=CARTESIAN_POINT('Ctrl Pts',(-1.45673027617593,2.83784422822171,97.3188940951704));
#40023=CARTESIAN_POINT('Ctrl Pts',(1.58724246591466,2.76696262582893,97.1605251873862));
#40024=CARTESIAN_POINT('Ctrl Pts',(3.18508414802795,0.175110803929055,97.0021562796021));
#40025=CARTESIAN_POINT('Ctrl Pts',(1.88100443011564,-2.57628548707993,96.8437873718179));
#40026=CARTESIAN_POINT('Ctrl Pts',(-1.13685022466966,-2.9804330251807,96.6854184640336));
#40027=CARTESIAN_POINT('Ctrl Pts',(-3.11892878941644,-0.669123446533811,
96.5270495562496));
#40028=CARTESIAN_POINT('Ctrl Pts',(-2.25935197620778,2.25183449024662,96.3686806484653));
#40029=CARTESIAN_POINT('Ctrl Pts',(0.65869538571899,3.12112917937077,96.2103117406811));
#40030=CARTESIAN_POINT('Ctrl Pts',(2.97664299288246,1.14682001966684,96.0519428328971));
#40031=CARTESIAN_POINT('Ctrl Pts',(2.58251016618233,-1.87244660443017,95.8935739251127));
#40032=CARTESIAN_POINT('Ctrl Pts',(-0.164400624555983,-3.18554845623818,
95.7352050173288));
#40033=CARTESIAN_POINT('Ctrl Pts',(-2.76180131574857,-1.59667188192327,
95.5768361095443));
#40034=CARTESIAN_POINT('Ctrl Pts',(-2.84239010463917,1.44764891516331,95.4184672017605));
#40035=CARTESIAN_POINT('Ctrl Pts',(-0.334360852594403,3.17159317438854,
95.2600982939759));
#40036=CARTESIAN_POINT('Ctrl Pts',(2.48043360101624,2.00875280664075,95.1017293861921));
#40037=CARTESIAN_POINT('Ctrl Pts',(3.03103843395327,-0.990116538764143,
94.9433604784076));
#40038=CARTESIAN_POINT('Ctrl Pts',(1.56313891022217,-2.37806168056784,94.8377812065516));
#40039=CARTESIAN_POINT('Ctrl Pts',(0.697617327903685,-2.60945232443793,
94.7849915706236));
#40040=CARTESIAN_POINT('Ctrl Pts',(2.19500094410104,1.87867314180088,114.214680436129));
#40041=CARTESIAN_POINT('Ctrl Pts',(2.81849377166239,1.15025817379284,114.161863202702));
#40042=CARTESIAN_POINT('Ctrl Pts',(3.27213349611052,-0.963287019043518,
114.056256333345));
#40043=CARTESIAN_POINT('Ctrl Pts',(0.969401606336187,-3.27356122779951,
113.897859828062));
#40044=CARTESIAN_POINT('Ctrl Pts',(-2.21636477647126,-2.5931457134717,113.739490920278));
#40045=CARTESIAN_POINT('Ctrl Pts',(-3.38265364276335,0.446079208816524,
113.581122012494));
#40046=CARTESIAN_POINT('Ctrl Pts',(-1.46709939584595,3.08079279408692,113.42275310471));
#40047=CARTESIAN_POINT('Ctrl Pts',(1.78516636366599,2.90764051950081,113.264384196926));
#40048=CARTESIAN_POINT('Ctrl Pts',(3.41095143630235,0.0858341326295093,
113.106015289141));
#40049=CARTESIAN_POINT('Ctrl Pts',(1.92904002261267,-2.81442232412067,112.947646381357));
#40050=CARTESIAN_POINT('Ctrl Pts',(-1.31041915425987,-3.15034253143425,
112.789277473573));
#40051=CARTESIAN_POINT('Ctrl Pts',(-3.35595678895446,-0.616058644316651,
112.630908565789));
#40052=CARTESIAN_POINT('Ctrl Pts',(-2.34389405762786,2.47954629060019,112.472539658005));
#40053=CARTESIAN_POINT('Ctrl Pts',(0.803683933223465,3.31602818661467,112.31417075022));
#40054=CARTESIAN_POINT('Ctrl Pts',(3.21902764690281,1.13129532555542,112.155801842436));
#40055=CARTESIAN_POINT('Ctrl Pts',(2.701525500982,-2.08416130730195,111.997432934652));
#40056=CARTESIAN_POINT('Ctrl Pts',(-0.277328185268923,-3.40074298975362,
111.839064026868));
#40057=CARTESIAN_POINT('Ctrl Pts',(-3.00350898185795,-1.6189194088289,111.680695119084));
#40058=CARTESIAN_POINT('Ctrl Pts',(-2.99320214548107,1.63789712580403,111.5223262113));
#40059=CARTESIAN_POINT('Ctrl Pts',(-0.255798167622519,3.40243043230853,
111.363957303515));
#40060=CARTESIAN_POINT('Ctrl Pts',(2.71466271619589,2.06702013137707,111.205588395731));
#40061=CARTESIAN_POINT('Ctrl Pts',(3.21180287767952,-1.15164582704055,111.047219487947));
#40062=CARTESIAN_POINT('Ctrl Pts',(0.782679463287348,-3.3210508329762,110.888850580163));
#40063=CARTESIAN_POINT('Ctrl Pts',(-2.35954076575154,-2.46465681126394,
110.730481672379));
#40064=CARTESIAN_POINT('Ctrl Pts',(-3.35199077017193,0.637278345293128,
110.572112764595));
#40065=CARTESIAN_POINT('Ctrl Pts',(-1.29045244886692,3.15859118655836,110.41374385681));
#40066=CARTESIAN_POINT('Ctrl Pts',(1.94681306960879,2.80212146140662,110.255374949026));
#40067=CARTESIAN_POINT('Ctrl Pts',(3.41034327851545,-0.107352379950659,
110.097006041242));
#40068=CARTESIAN_POINT('Ctrl Pts',(1.76672037369713,-2.91901780251153,109.938637133458));
#40069=CARTESIAN_POINT('Ctrl Pts',(-1.48655594774592,-3.07117521890013,
109.780268225674));
#40070=CARTESIAN_POINT('Ctrl Pts',(-3.38543578634698,-0.42519448164591,
109.62189931789));
#40071=CARTESIAN_POINT('Ctrl Pts',(-2.1998556495968,2.60817962027,109.463530410105));
#40072=CARTESIAN_POINT('Ctrl Pts',(0.990006101379621,3.26524941313507,109.305161502321));
#40073=CARTESIAN_POINT('Ctrl Pts',(3.27787638426565,0.947360660034989,109.146792594537));
#40074=CARTESIAN_POINT('Ctrl Pts',(2.57928372723081,-2.2336654326798,108.988423686753));
#40075=CARTESIAN_POINT('Ctrl Pts',(-0.469286280960221,-3.37960592336147,
108.830054778969));
#40076=CARTESIAN_POINT('Ctrl Pts',(-3.0902910237166,-1.4463980086575,108.671685871184));
#40077=CARTESIAN_POINT('Ctrl Pts',(-2.89574126289272,1.80461861596644,108.5133169634));
#40078=CARTESIAN_POINT('Ctrl Pts',(-0.0628906781758312,3.41145285374311,
108.354948055616));
#40079=CARTESIAN_POINT('Ctrl Pts',(2.8272594070775,1.91012304729417,108.196579147832));
#40080=CARTESIAN_POINT('Ctrl Pts',(3.14150227346538,-1.3315139039922,108.038210240048));
#40081=CARTESIAN_POINT('Ctrl Pts',(0.593532226512415,-3.3600126944409,107.879841332264));
#40082=CARTESIAN_POINT('Ctrl Pts',(-2.49520317896243,-2.3272144092044,107.721472424479));
#40083=CARTESIAN_POINT('Ctrl Pts',(-3.31056675830222,0.825901658514566,
107.563103516695));
#40084=CARTESIAN_POINT('Ctrl Pts',(-1.10968329999871,3.22654130368988,107.404734608911));
#40085=CARTESIAN_POINT('Ctrl Pts',(2.10222914841638,2.68748924058522,107.246365701127));
#40086=CARTESIAN_POINT('Ctrl Pts',(3.39880718303156,-0.300125879067034,
107.087996793343));
#40087=CARTESIAN_POINT('Ctrl Pts',(1.59874260452601,-3.01429724731755,106.929627885559));
#40088=CARTESIAN_POINT('Ctrl Pts',(-1.65793136956495,-2.98215180440655,
106.771258977774));
#40089=CARTESIAN_POINT('Ctrl Pts',(-3.40406924903544,-0.232977163009677,
106.61289006999));
#40090=CARTESIAN_POINT('Ctrl Pts',(-2.04877026347763,2.72846224423256,106.454521162206));
#40091=CARTESIAN_POINT('Ctrl Pts',(1.17315691271518,3.20400821922499,106.296152254422));
#40092=CARTESIAN_POINT('Ctrl Pts',(3.32622448841996,0.760392308843405,106.137783346638));
#40093=CARTESIAN_POINT('Ctrl Pts',(2.44877931745582,-2.37601466012173,105.979414438853));
#40094=CARTESIAN_POINT('Ctrl Pts',(-0.659741044363595,-3.34764209035177,
105.821045531069));
#40095=CARTESIAN_POINT('Ctrl Pts',(-3.16717340042598,-1.26924326366024,
105.662676623285));
#40096=CARTESIAN_POINT('Ctrl Pts',(-2.78900395952094,1.96555913787636,105.504307715501));
#40097=CARTESIAN_POINT('Ctrl Pts',(0.130218281417219,3.40954674552168,105.345938807717));
#40098=CARTESIAN_POINT('Ctrl Pts',(2.93079905270771,1.74710695819127,105.187569899933));
#40099=CARTESIAN_POINT('Ctrl Pts',(3.0611379572579,-1.50711652414395,105.029200992148));
#40100=CARTESIAN_POINT('Ctrl Pts',(0.402483626060236,-3.38821084666616,
104.870832084364));
#40101=CARTESIAN_POINT('Ctrl Pts',(-2.62287228025585,-2.18231684504754,
104.71246317658));
#40102=CARTESIAN_POINT('Ctrl Pts',(-3.25853744084126,1.01187922073165,104.554094268796));
#40103=CARTESIAN_POINT('Ctrl Pts',(-0.925359312482507,3.28415528766754,
104.395725361012));
#40104=CARTESIAN_POINT('Ctrl Pts',(2.25091079643559,2.56424772539676,104.237356453228));
#40105=CARTESIAN_POINT('Ctrl Pts',(3.37638310623911,-0.491937933702975,
104.078987545443));
#40106=CARTESIAN_POINT('Ctrl Pts',(1.42564330927776,-3.09992047727427,103.920618637659));
#40107=CARTESIAN_POINT('Ctrl Pts',(-1.8239956557977,-2.88357515219282,103.762249729875));
#40108=CARTESIAN_POINT('Ctrl Pts',(-3.41179787353161,-0.0400135086934916,
103.603880822091));
#40109=CARTESIAN_POINT('Ctrl Pts',(-1.89112170058811,2.84000431765121,103.445511914307));
#40110=CARTESIAN_POINT('Ctrl Pts',(1.35254954953276,3.13250307689736,103.287143006522));
#40111=CARTESIAN_POINT('Ctrl Pts',(3.36391712783881,0.570988062699605,103.128774098738));
#40112=CARTESIAN_POINT('Ctrl Pts',(2.31043031338077,-2.51075239275481,102.970405190954));
#40113=CARTESIAN_POINT('Ctrl Pts',(-0.848082346256082,-3.30495418193377,
102.81203628317));
#40114=CARTESIAN_POINT('Ctrl Pts',(-3.2339098279978,-1.08802253427584,102.653667375386));
#40115=CARTESIAN_POINT('Ctrl Pts',(-2.67333216196771,2.12020304747017,102.495298467602));
#40116=CARTESIAN_POINT('Ctrl Pts',(0.322910090481049,3.39671825210427,102.336929559818));
#40117=CARTESIAN_POINT('Ctrl Pts',(3.02494996764285,1.57849406206368,102.178560652033));
#40118=CARTESIAN_POINT('Ctrl Pts',(2.97096737341337,-1.6778911397424,102.020191744249));
#40119=CARTESIAN_POINT('Ctrl Pts',(0.210145680857242,-3.40555496263529,
101.861822836465));
#40120=CARTESIAN_POINT('Ctrl Pts',(-2.74213908543681,-2.03042829147757,
101.703453928681));
#40121=CARTESIAN_POINT('Ctrl Pts',(-3.19606949216004,1.19461525689096,101.545085020896));
#40122=CARTESIAN_POINT('Ctrl Pts',(-0.738070962952793,3.33124857438748,
101.386716113112));
#40123=CARTESIAN_POINT('Ctrl Pts',(2.39238171628604,2.4327917161757,101.228347205328));
#40124=CARTESIAN_POINT('Ctrl Pts',(3.34314288301767,-0.682174079279619,
101.069978297544));
#40125=CARTESIAN_POINT('Ctrl Pts',(1.247977006583,-3.17561320090353,100.91160938976));
#40126=CARTESIAN_POINT('Ctrl Pts',(-1.98421682426866,-2.77576104969477,
100.753240481976));
#40127=CARTESIAN_POINT('Ctrl Pts',(-3.40859690140757,0.153078327750135,
100.594871574191));
#40128=CARTESIAN_POINT('Ctrl Pts',(-1.72741498357801,2.94244851870377,100.436502666407));
#40129=CARTESIAN_POINT('Ctrl Pts',(1.52760933266685,3.05096305081963,100.278133758623));
#40130=CARTESIAN_POINT('Ctrl Pts',(3.39083355523211,0.379754672674693,100.119764850839));
#40131=CARTESIAN_POINT('Ctrl Pts',(2.16467991207339,-2.63744700211668,99.9613959430545));
#40132=CARTESIAN_POINT('Ctrl Pts',(-1.03370684068292,-3.25167894760123,
99.8030270352703));
#40133=CARTESIAN_POINT('Ctrl Pts',(-3.29028651819418,-0.90331635590437,
99.6446581274863));
#40134=CARTESIAN_POINT('Ctrl Pts',(-2.5490964215312,2.26805494740268,99.4862892197019));
#40135=CARTESIAN_POINT('Ctrl Pts',(0.514567466358019,3.37300846923499,99.3279203119179));
#40136=CARTESIAN_POINT('Ctrl Pts',(3.10941054207769,1.4048245054212,99.1695514041337));
#40137=CARTESIAN_POINT('Ctrl Pts',(2.87127938090939,-1.84329067907401,99.0111824963495));
#40138=CARTESIAN_POINT('Ctrl Pts',(0.0171345397984093,-3.41198948122956,
98.8528135885653));
#40139=CARTESIAN_POINT('Ctrl Pts',(-2.85262152633003,-1.8720353186063,98.6944446807813));
#40140=CARTESIAN_POINT('Ctrl Pts',(-3.12336302730363,1.37352437632903,98.5360757729969));
#40141=CARTESIAN_POINT('Ctrl Pts',(-0.548418222755575,3.36767030386034,
98.3777068652128));
#40142=CARTESIAN_POINT('Ctrl Pts',(2.52618870694997,2.29354232451508,98.2193379574286));
#40143=CARTESIAN_POINT('Ctrl Pts',(3.29919300336885,-0.870224891928761,
98.0609690496445));
#40144=CARTESIAN_POINT('Ctrl Pts',(1.06631283368099,-3.24113295422285,97.9026001418602));
#40145=CARTESIAN_POINT('Ctrl Pts',(-2.13808158799722,-2.65905484567836,
97.7442312340761));
#40146=CARTESIAN_POINT('Ctrl Pts',(-3.39447663248505,0.345679721624724,
97.5858623262918));
#40147=CARTESIAN_POINT('Ctrl Pts',(-1.5581744520633,3.03546679002117,97.4274934185078));
#40148=CARTESIAN_POINT('Ctrl Pts',(1.69777528487333,2.9596491154825,97.2691245107234));
#40149=CARTESIAN_POINT('Ctrl Pts',(3.4068878970218,0.18730521732464,97.1107556029395));
#40150=CARTESIAN_POINT('Ctrl Pts',(2.01199432397197,-2.75569355071509,96.9523866951552));
#40151=CARTESIAN_POINT('Ctrl Pts',(-1.21601850725094,-3.1879852240824,96.7940177873711));
#40152=CARTESIAN_POINT('Ctrl Pts',(-3.33612559370361,-0.715720045582149,
96.6356488795868));
#40153=CARTESIAN_POINT('Ctrl Pts',(-2.41668933852826,2.4086483478521,96.4772799718027));
#40154=CARTESIAN_POINT('Ctrl Pts',(0.70456579265561,3.33847921500707,96.3189110640184));
#40155=CARTESIAN_POINT('Ctrl Pts',(3.18393126049271,1.22668258152122,96.1605421562345));
#40156=CARTESIAN_POINT('Ctrl Pts',(2.76235170569977,-2.00284054611316,96.00217324845));
#40157=CARTESIAN_POINT('Ctrl Pts',(-0.175849199591597,-3.40738453885239,
95.843804340666));
#40158=CARTESIAN_POINT('Ctrl Pts',(-2.95412838069862,-1.7078613490973,95.6854354328817));
#40159=CARTESIAN_POINT('Ctrl Pts',(-3.04032923340671,1.54846068078304,95.5270665250977));
#40160=CARTESIAN_POINT('Ctrl Pts',(-0.357645163832503,3.39245743532123,
95.3686976173134));
#40161=CARTESIAN_POINT('Ctrl Pts',(2.65316670515616,2.14863887639834,95.2103287095293));
#40162=CARTESIAN_POINT('Ctrl Pts',(3.24211470596056,-1.05906654134874,95.0519598017451));
#40163=CARTESIAN_POINT('Ctrl Pts',(1.67199319926822,-2.54366578129941,94.9463805298889));
#40164=CARTESIAN_POINT('Ctrl Pts',(0.746198191548342,-2.79117006923892,
94.8935908939609));
#40165=CARTESIAN_POINT('Ctrl Pts',(2.33790539331178,2.00098322613026,114.323279759466));
#40166=CARTESIAN_POINT('Ctrl Pts',(3.00199041257534,1.22514516243756,114.270462526038));
#40167=CARTESIAN_POINT('Ctrl Pts',(3.48516412658124,-1.02600134327114,114.164855656683));
#40168=CARTESIAN_POINT('Ctrl Pts',(1.03251401774073,-3.48668481003465,114.006459151399));
#40169=CARTESIAN_POINT('Ctrl Pts',(-2.36066010740627,-2.76197118067833,
113.848090243615));
#40170=CARTESIAN_POINT('Ctrl Pts',(-3.60287963263771,0.475120974749064,
113.689721335831));
#40171=CARTESIAN_POINT('Ctrl Pts',(-1.56261417531073,3.28136628292964,113.531352428046));
#40172=CARTESIAN_POINT('Ctrl Pts',(1.90138873552182,3.09694101527453,113.372983520263));
#40173=CARTESIAN_POINT('Ctrl Pts',(3.63301974000825,0.0914223213179323,
113.214614612478));
#40174=CARTESIAN_POINT('Ctrl Pts',(2.05462921776896,-2.99765389545814,113.056245704694));
#40175=CARTESIAN_POINT('Ctrl Pts',(-1.39573334420497,-3.35544402147674,
112.89787679691));
#40176=CARTESIAN_POINT('Ctrl Pts',(-3.57444469338541,-0.656166837201114,
112.739507889126));
#40177=CARTESIAN_POINT('Ctrl Pts',(-2.49649211924318,2.64097592365024,112.581138981341));
#40178=CARTESIAN_POINT('Ctrl Pts',(0.856007377605333,3.53191655916822,112.422770073557));
#40179=CARTESIAN_POINT('Ctrl Pts',(3.42860084736592,1.20494774735854,112.264401165773));
#40180=CARTESIAN_POINT('Ctrl Pts',(2.87740698057048,-2.21984959686134,112.106032257989));
#40181=CARTESIAN_POINT('Ctrl Pts',(-0.295383499401239,-3.62214667760355,
111.947663350205));
#40182=CARTESIAN_POINT('Ctrl Pts',(-3.19905094638667,-1.72431835503756,
111.789294442421));
#40183=CARTESIAN_POINT('Ctrl Pts',(-3.18807308853279,1.74453160687608,111.630925534636));
#40184=CARTESIAN_POINT('Ctrl Pts',(-0.272451780620475,3.62394398027014,
111.472556626852));
#40185=CARTESIAN_POINT('Ctrl Pts',(2.89139948767358,2.20159245316845,111.314187719068));
#40186=CARTESIAN_POINT('Ctrl Pts',(3.42090571312101,-1.2266231581626,111.155818811284));
#40187=CARTESIAN_POINT('Ctrl Pts',(0.833635422058219,-3.53726620243323,
110.9974499035));
#40188=CARTESIAN_POINT('Ctrl Pts',(-2.51315749854894,-2.62511707213705,
110.839080995716));
#40189=CARTESIAN_POINT('Ctrl Pts',(-3.57022046891454,0.678768036298866,
110.680712087931));
#40190=CARTESIAN_POINT('Ctrl Pts',(-1.37446671634757,3.36422970120687,110.522343180147));
#40191=CARTESIAN_POINT('Ctrl Pts',(2.07355937018619,2.98455219117012,110.363974272363));
#40192=CARTESIAN_POINT('Ctrl Pts',(3.63237198840987,-0.114341503472241,
110.205605364579));
#40193=CARTESIAN_POINT('Ctrl Pts',(1.88174182851294,-3.10905901066011,110.047236456795));
#40194=CARTESIAN_POINT('Ctrl Pts',(-1.58333743638467,-3.27112256027421,
109.888867549011));
#40195=CARTESIAN_POINT('Ctrl Pts',(-3.60584290630127,-0.452876557760886,
109.730498641226));
#40196=CARTESIAN_POINT('Ctrl Pts',(-2.34307616200414,2.77798386253196,109.572129733442));
#40197=CARTESIAN_POINT('Ctrl Pts',(1.0544599582279,3.47783185879359,109.413760825658));
#40198=CARTESIAN_POINT('Ctrl Pts',(3.49128090262507,1.00903810654819,109.255391917874));
#40199=CARTESIAN_POINT('Ctrl Pts',(2.74720671668951,-2.3790871142677,109.09702301009));
#40200=CARTESIAN_POINT('Ctrl Pts',(-0.49983893182946,-3.59963349297381,
108.938654102305));
#40201=CARTESIAN_POINT('Ctrl Pts',(-3.29148289009458,-1.54056503456343,
108.780285194521));
#40202=CARTESIAN_POINT('Ctrl Pts',(-3.08426706345904,1.92210741707296,108.621916286737));
#40203=CARTESIAN_POINT('Ctrl Pts',(-0.066985144626685,3.63355380198312,
108.463547378953));
#40204=CARTESIAN_POINT('Ctrl Pts',(3.01132673034226,2.03448066214254,108.305178471169));
#40205=CARTESIAN_POINT('Ctrl Pts',(3.34602822289167,-1.4182014571697,108.146809563385));
#40206=CARTESIAN_POINT('Ctrl Pts',(0.632173848123799,-3.57876465658952,
107.9884406556));
#40207=CARTESIAN_POINT('Ctrl Pts',(-2.65765214597394,-2.47872655057109,
107.830071747816));
#40208=CARTESIAN_POINT('Ctrl Pts',(-3.52609956727071,0.879671576896354,
107.671702840032));
#40209=CARTESIAN_POINT('Ctrl Pts',(-1.18192868158311,3.43660367705634,107.513333932248));
#40210=CARTESIAN_POINT('Ctrl Pts',(2.23909373582195,2.86245689639317,107.354965024464));
#40211=CARTESIAN_POINT('Ctrl Pts',(3.62008484114372,-0.319665425761639,
107.196596116679));
#40212=CARTESIAN_POINT('Ctrl Pts',(1.70282794988475,-3.21054157652525,107.038227208895));
#40213=CARTESIAN_POINT('Ctrl Pts',(-1.76587017015344,-3.17630332047621,
106.879858301111));
#40214=CARTESIAN_POINT('Ctrl Pts',(-3.62568949134831,-0.248145025806301,
106.721489393327));
#40215=CARTESIAN_POINT('Ctrl Pts',(-2.18215443665916,2.90609742714773,106.563120485543));
#40216=CARTESIAN_POINT('Ctrl Pts',(1.24953471241494,3.41260358728873,106.404751577759));
#40217=CARTESIAN_POINT('Ctrl Pts',(3.54277668615197,0.809897273463753,106.246382669975));
#40218=CARTESIAN_POINT('Ctrl Pts',(2.60820588195919,-2.53070391765205,106.08801376219));
#40219=CARTESIAN_POINT('Ctrl Pts',(-0.702693158265811,-3.56558867044873,
105.929644854406));
#40220=CARTESIAN_POINT('Ctrl Pts',(-3.3733706558573,-1.3518767176436,105.771275946622));
#40221=CARTESIAN_POINT('Ctrl Pts',(-2.9705806808217,2.09352589194279,105.612907038838));
#40222=CARTESIAN_POINT('Ctrl Pts',(0.13869607812756,3.6315235975301,105.454538131054));
#40223=CARTESIAN_POINT('Ctrl Pts',(3.12160727331468,1.86085149130572,105.296169223269));
#40224=CARTESIAN_POINT('Ctrl Pts',(3.26043182768453,-1.60523659892479,105.137800315485));
#40225=CARTESIAN_POINT('Ctrl Pts',(0.428687123171732,-3.60879863554794,
104.979431407701));
#40226=CARTESIAN_POINT('Ctrl Pts',(-2.79363308086844,-2.32439550227224,
104.821062499917));
#40227=CARTESIAN_POINT('Ctrl Pts',(-3.47068290686825,1.07775711618088,104.662693592133));
#40228=CARTESIAN_POINT('Ctrl Pts',(-0.985604372161288,3.4979685909228,104.504324684348));
#40229=CARTESIAN_POINT('Ctrl Pts',(2.39745522888862,2.73119180340389,104.345955776564));
#40230=CARTESIAN_POINT('Ctrl Pts',(3.59620085593905,-0.523965309203938,
104.18758686878));
#40231=CARTESIAN_POINT('Ctrl Pts',(1.51845911076105,-3.30173926445634,104.029217960996));
#40232=CARTESIAN_POINT('Ctrl Pts',(-1.94274598948437,-3.07130888414831,
103.870849053212));
#40233=CARTESIAN_POINT('Ctrl Pts',(-3.63392128411406,-0.042618568356995,
103.712480145428));
#40234=CARTESIAN_POINT('Ctrl Pts',(-2.01424224217116,3.0249013920059,103.554111237643));
#40235=CARTESIAN_POINT('Ctrl Pts',(1.44060661799356,3.33644313808868,103.395742329859));
#40236=CARTESIAN_POINT('Ctrl Pts',(3.58292328618981,0.608161957692807,103.237373422075));
#40237=CARTESIAN_POINT('Ctrl Pts',(2.46084973450257,-2.67421368362825,103.079004514291));
#40238=CARTESIAN_POINT('Ctrl Pts',(-0.903296327326473,-3.52012158689788,
102.920635606507));
#40239=CARTESIAN_POINT('Ctrl Pts',(-3.44445192548946,-1.15885770243712,
102.762266698723));
#40240=CARTESIAN_POINT('Ctrl Pts',(-2.84737812818474,2.25823781667056,102.603897790938));
#40241=CARTESIAN_POINT('Ctrl Pts',(0.343932991974009,3.61785991140311,102.445528883154));
#40242=CARTESIAN_POINT('Ctrl Pts',(3.22188783693069,1.68126113609517,102.28715997537));
#40243=CARTESIAN_POINT('Ctrl Pts',(3.16439073264322,-1.78712941128159,102.128791067586));
#40244=CARTESIAN_POINT('Ctrl Pts',(0.223827111317502,-3.62727193159614,
101.970422159802));
#40245=CARTESIAN_POINT('Ctrl Pts',(-2.92066469232399,-2.16261831965741,
101.812053252017));
#40246=CARTESIAN_POINT('Ctrl Pts',(-3.40414801333053,1.27239009145927,101.653684344234));
#40247=CARTESIAN_POINT('Ctrl Pts',(-0.786122707405416,3.54812786274783,
101.495315436449));
#40248=CARTESIAN_POINT('Ctrl Pts',(2.54813654290081,2.5911774158169,101.336946528665));
#40249=CARTESIAN_POINT('Ctrl Pts',(3.56079654444974,-0.726586684808233,
101.178577620881));
#40250=CARTESIAN_POINT('Ctrl Pts',(1.32922593143321,-3.38235992536443,101.020208713097));
#40251=CARTESIAN_POINT('Ctrl Pts',(-2.11339827776591,-2.95647559791092,
100.861839805313));
#40252=CARTESIAN_POINT('Ctrl Pts',(-3.63051191428542,0.16304441645366,100.703470897528));
#40253=CARTESIAN_POINT('Ctrl Pts',(-1.83987748043935,3.13401517202406,100.545101989744));
#40254=CARTESIAN_POINT('Ctrl Pts',(1.62706358159582,3.24959448900257,100.38673308196));
#40255=CARTESIAN_POINT('Ctrl Pts',(3.61159209425597,0.404478412534406,100.228364174176));
#40256=CARTESIAN_POINT('Ctrl Pts',(2.30561032551295,-2.80915668277669,100.069995266392));
#40257=CARTESIAN_POINT('Ctrl Pts',(-1.10100581251714,-3.46337789482306,
99.9116263586078));
#40258=CARTESIAN_POINT('Ctrl Pts',(-3.50449899217589,-0.962126319813717,
99.7532574508236));
#40259=CARTESIAN_POINT('Ctrl Pts',(-2.71505408140509,2.41571554131236,99.5948885430393));
#40260=CARTESIAN_POINT('Ctrl Pts',(0.54806812637335,3.59260651486435,99.4365196352553));
#40261=CARTESIAN_POINT('Ctrl Pts',(3.31184717522804,1.49628490899163,99.278150727471));
#40262=CARTESIAN_POINT('Ctrl Pts',(3.05821260276595,-1.96329720569364,99.1197818196869));
#40263=CARTESIAN_POINT('Ctrl Pts',(0.0182500755246922,-3.63412536633627,
98.9614129119027));
#40264=CARTESIAN_POINT('Ctrl Pts',(-3.03834003780604,-1.99391325074452,
98.8030440041185));
#40265=CARTESIAN_POINT('Ctrl Pts',(-3.32670803009352,1.46294700049888,98.6446750963343));
#40266=CARTESIAN_POINT('Ctrl Pts',(-0.584122719498795,3.58692081087714,
98.4863061885502));
#40267=CARTESIAN_POINT('Ctrl Pts',(2.69065497141298,2.44286226148695,98.3279372807659));
#40268=CARTESIAN_POINT('Ctrl Pts',(3.51398532965618,-0.926880452467247,
98.1695683729819));
#40269=CARTESIAN_POINT('Ctrl Pts',(1.13573460253856,-3.45214530976955,98.0111994651975));
#40270=CARTESIAN_POINT('Ctrl Pts',(-2.27728033072282,-2.83217129429038,
97.8528305574135));
#40271=CARTESIAN_POINT('Ctrl Pts',(-3.61547235224893,0.368185028674753,
97.6944616496293));
#40272=CARTESIAN_POINT('Ctrl Pts',(-1.65961862795068,3.23308935182062,97.536092741845));
#40273=CARTESIAN_POINT('Ctrl Pts',(1.808308103832,3.15233560513605,97.377723834061));
#40274=CARTESIAN_POINT('Ctrl Pts',(3.62869164601564,0.199499630720231,97.2193549262767));
#40275=CARTESIAN_POINT('Ctrl Pts',(2.14298421782831,-2.93510161435026,97.0609860184926));
#40276=CARTESIAN_POINT('Ctrl Pts',(-1.29518678983222,-3.39553742298411,
96.9026171107084));
#40277=CARTESIAN_POINT('Ctrl Pts',(-3.55332239799077,-0.762316644630488,
96.7442482029242));
#40278=CARTESIAN_POINT('Ctrl Pts',(-2.57402670084876,2.5654622054576,96.5858792951401));
#40279=CARTESIAN_POINT('Ctrl Pts',(0.750436199592229,3.55582925064338,96.4275103873558));
#40280=CARTESIAN_POINT('Ctrl Pts',(3.39121952810296,1.30654514337561,96.2691414795717));
#40281=CARTESIAN_POINT('Ctrl Pts',(2.94219324521721,-2.13323448779617,96.1107725717875));
#40282=CARTESIAN_POINT('Ctrl Pts',(-0.187297774627212,-3.62922062146662,
95.9524036640034));
#40283=CARTESIAN_POINT('Ctrl Pts',(-3.14645544564867,-1.81905081627131,
95.7940347562191));
#40284=CARTESIAN_POINT('Ctrl Pts',(-3.23826836217426,1.64927244640277,95.6356658484351));
#40285=CARTESIAN_POINT('Ctrl Pts',(-0.380929475070602,3.61332169625394,
95.4772969406507));
#40286=CARTESIAN_POINT('Ctrl Pts',(2.82589980929608,2.28852494615592,95.3189280328667));
#40287=CARTESIAN_POINT('Ctrl Pts',(3.45319097796785,-1.12801654393334,95.1605591250824));
#40288=CARTESIAN_POINT('Ctrl Pts',(1.78084748831427,-2.70926988203097,95.0549798532264));
#40289=CARTESIAN_POINT('Ctrl Pts',(0.794779055193,-2.97288781403991,95.0021902172983));
#40290=CARTESIAN_POINT('Ctrl Pts',(1.9134659966651,1.63598720337492,114.));
#40291=CARTESIAN_POINT('Ctrl Pts',(1.97550038889691,1.57769010736882,114.));
#40292=CARTESIAN_POINT('Ctrl Pts',(2.0341197291836,1.51620065598168,114.));
#40293=CARTESIAN_POINT('Ctrl Pts',(2.08932641459958,1.45191113897336,114.));
#40294=CARTESIAN_POINT('Ctrl Pts',(2.14568689999563,1.38627799405325,114.));
#40295=CARTESIAN_POINT('Ctrl Pts',(2.19849101332626,1.31772603672195,114.));
#40296=CARTESIAN_POINT('Ctrl Pts',(2.24771556153909,1.24662378886774,114.));
#40297=CARTESIAN_POINT('Ctrl Pts',(2.29816664594502,1.17374987456722,114.));
#40298=CARTESIAN_POINT('Ctrl Pts',(2.34485807578261,1.09819642150282,114.));
#40299=CARTESIAN_POINT('Ctrl Pts',(2.38773087568948,1.02031743916418,114.));
#40300=CARTESIAN_POINT('Ctrl Pts',(2.40643444456904,0.986342170145018,114.));
#40301=CARTESIAN_POINT('Ctrl Pts',(2.42441077356168,0.951923818009723,114.));
#40302=CARTESIAN_POINT('Ctrl Pts',(2.4416526189394,0.917089771608395,114.));
#40303=CARTESIAN_POINT('Ctrl Pts',(2.45250309293484,0.895168341137736,114.));
#40304=CARTESIAN_POINT('Ctrl Pts',(2.46306223222539,0.873083189209911,114.));
#40305=CARTESIAN_POINT('Ctrl Pts',(2.47332929073886,0.850837952133165,114.));
#40306=CARTESIAN_POINT('Ctrl Pts',(2.48084188372401,0.834560708578284,114.));
#40307=CARTESIAN_POINT('Ctrl Pts',(2.48819808553823,0.81819734264052,114.));
#40308=CARTESIAN_POINT('Ctrl Pts',(2.49538774583109,0.801772443778709,114.));
#40309=CARTESIAN_POINT('Ctrl Pts',(2.53205184816493,0.718012690443779,114.));
#40310=CARTESIAN_POINT('Ctrl Pts',(2.56443370917822,0.632561132627693,114.));
#40311=CARTESIAN_POINT('Ctrl Pts',(2.59250806912875,0.545819305993932,114.));
#40312=CARTESIAN_POINT('Ctrl Pts',(2.62096652553687,0.457890730013266,114.));
#40313=CARTESIAN_POINT('Ctrl Pts',(2.64499928611092,0.368635563742515,114.));
#40314=CARTESIAN_POINT('Ctrl Pts',(2.66454092159011,0.27843493656148,114.));
#40315=CARTESIAN_POINT('Ctrl Pts',(2.68410865469452,0.188113847499725,114.));
#40316=CARTESIAN_POINT('Ctrl Pts',(2.69917368039218,0.0968438779961723,
114.));
#40317=CARTESIAN_POINT('Ctrl Pts',(2.7096246951451,0.00498341951435599,
114.));
#40318=CARTESIAN_POINT('Ctrl Pts',(2.71348879003703,-0.0289805099970009,
114.));
#40319=CARTESIAN_POINT('Ctrl Pts',(2.71672165473184,-0.0630253317880274,
114.));
#40320=CARTESIAN_POINT('Ctrl Pts',(2.71931590711735,-0.0971333890683507,
114.));
#40321=CARTESIAN_POINT('Ctrl Pts',(2.72100442149991,-0.119333212647831,
114.));
#40322=CARTESIAN_POINT('Ctrl Pts',(2.72242238171113,-0.141559828395214,
114.));
#40323=CARTESIAN_POINT('Ctrl Pts',(2.7235675220808,-0.163808393204148,114.));
#40324=CARTESIAN_POINT('Ctrl Pts',(2.72420819736649,-0.176255867760832,
114.));
#40325=CARTESIAN_POINT('Ctrl Pts',(2.72476337873092,-0.188709282612654,
114.));
#40326=CARTESIAN_POINT('Ctrl Pts',(2.7252324368028,-0.201157503848221,114.));
#40327=CARTESIAN_POINT('Ctrl Pts',(2.72898278021086,-0.300686980583852,
114.));
#40328=CARTESIAN_POINT('Ctrl Pts',(2.72724148462551,-0.400056709441885,
114.));
#40329=CARTESIAN_POINT('Ctrl Pts',(2.71993962742201,-0.498811550184699,
114.));
#40330=CARTESIAN_POINT('Ctrl Pts',(2.71263777021851,-0.597566390927493,
114.));
#40331=CARTESIAN_POINT('Ctrl Pts',(2.69977584370241,-0.695707537343122,
114.));
#40332=CARTESIAN_POINT('Ctrl Pts',(2.68122651196178,-0.792800808383239,
114.));
#40333=CARTESIAN_POINT('Ctrl Pts',(2.66387227429393,-0.883638566052308,
114.));
#40334=CARTESIAN_POINT('Ctrl Pts',(2.6415397886767,-0.973560147194905,114.));
#40335=CARTESIAN_POINT('Ctrl Pts',(2.61450671787376,-1.06232446094815,114.));
#40336=CARTESIAN_POINT('Ctrl Pts',(2.59875842933366,-1.11403468045077,114.));
#40337=CARTESIAN_POINT('Ctrl Pts',(2.58141387131424,-1.16535211779573,114.));
#40338=CARTESIAN_POINT('Ctrl Pts',(2.56251994638479,-1.21622780801466,114.));
#40339=CARTESIAN_POINT('Ctrl Pts',(2.55761297680077,-1.22944080983416,114.));
#40340=CARTESIAN_POINT('Ctrl Pts',(2.55260194342609,-1.24262256219186,114.));
#40341=CARTESIAN_POINT('Ctrl Pts',(2.54749229902281,-1.25576083529272,114.));
#40342=CARTESIAN_POINT('Ctrl Pts',(2.5132016869521,-1.34393124219844,114.));
#40343=CARTESIAN_POINT('Ctrl Pts',(2.47442287157765,-1.43028360326182,114.));
#40344=CARTESIAN_POINT('Ctrl Pts',(2.43150025930897,-1.51457657732671,114.));
#40345=CARTESIAN_POINT('Ctrl Pts',(2.38773715221989,-1.60052014543408,114.));
#40346=CARTESIAN_POINT('Ctrl Pts',(2.33966609261984,-1.68432359939539,114.));
#40347=CARTESIAN_POINT('Ctrl Pts',(2.28759680182187,-1.76572803828939,114.));
#40348=CARTESIAN_POINT('Ctrl Pts',(2.23465317175456,-1.84849940760502,114.));
#40349=CARTESIAN_POINT('Ctrl Pts',(2.17757554498291,-1.92879134450094,114.));
#40350=CARTESIAN_POINT('Ctrl Pts',(2.11663783812543,-2.00631672329851,114.));
#40351=CARTESIAN_POINT('Ctrl Pts',(2.07420548151236,-2.06029946550106,114.));
#40352=CARTESIAN_POINT('Ctrl Pts',(2.02990040888812,-2.11294049801343,114.));
#40353=CARTESIAN_POINT('Ctrl Pts',(1.98380220585711,-2.16413538567044,114.));
#40354=CARTESIAN_POINT('Ctrl Pts',(1.97305120009932,-2.17607503832023,114.));
#40355=CARTESIAN_POINT('Ctrl Pts',(1.9622027172611,-2.18793578502567,114.));
#40356=CARTESIAN_POINT('Ctrl Pts',(1.95126749026891,-2.19970603226562,114.));
#40357=CARTESIAN_POINT('Ctrl Pts',(1.88257352086365,-2.27364551284258,114.));
#40358=CARTESIAN_POINT('Ctrl Pts',(1.81036676090401,-2.34412026577735,114.));
#40359=CARTESIAN_POINT('Ctrl Pts',(1.73495944557455,-2.4108413165029,114.));
#40360=CARTESIAN_POINT('Ctrl Pts',(1.67111364979667,-2.46733263382534,114.));
#40361=CARTESIAN_POINT('Ctrl Pts',(1.6049724199379,-2.52113307849603,114.));
#40362=CARTESIAN_POINT('Ctrl Pts',(1.53670040710693,-2.57205276284475,114.));
#40363=CARTESIAN_POINT('Ctrl Pts',(1.51106812286496,-2.59117022794673,114.));
#40364=CARTESIAN_POINT('Ctrl Pts',(1.48513572033671,-2.60988115577991,114.));
#40365=CARTESIAN_POINT('Ctrl Pts',(1.45890980106933,-2.62817581421199,114.));
#40366=CARTESIAN_POINT('Ctrl Pts',(1.43763441829496,-2.64301708085742,114.));
#40367=CARTESIAN_POINT('Ctrl Pts',(1.4161671835519,-2.65758318957349,114.));
#40368=CARTESIAN_POINT('Ctrl Pts',(1.3945338103328,-2.67185485201352,114.));
#40369=CARTESIAN_POINT('Ctrl Pts',(1.30939543171884,-2.72802113676084,114.));
#40370=CARTESIAN_POINT('Ctrl Pts',(1.22161013194401,-2.77968415206107,114.));
#40371=CARTESIAN_POINT('Ctrl Pts',(1.13146814684533,-2.82653576956066,114.));
#40372=CARTESIAN_POINT('Ctrl Pts',(1.04714058572959,-2.87036531950615,114.));
#40373=CARTESIAN_POINT('Ctrl Pts',(0.960749769307409,-2.9099844694343,114.));
#40374=CARTESIAN_POINT('Ctrl Pts',(0.872505205252779,-2.94511065658153,
114.));
#40375=CARTESIAN_POINT('Ctrl Pts',(0.847218614713906,-2.95517610957684,
114.));
#40376=CARTESIAN_POINT('Ctrl Pts',(0.82177966221848,-2.96487242144315,114.));
#40377=CARTESIAN_POINT('Ctrl Pts',(0.796195672661137,-2.97420175871636,
114.));
#40378=CARTESIAN_POINT('Ctrl Pts',(-0.794822165015276,-2.97304906723816,
113.997713413532));
#40379=CARTESIAN_POINT('Ctrl Pts',(-1.78094408373656,-2.70941683625881,
113.944923777604));
#40380=CARTESIAN_POINT('Ctrl Pts',(-3.45337864756995,-1.12808000940134,
113.839344505748));
#40381=CARTESIAN_POINT('Ctrl Pts',(-2.82605277153101,2.28865011881991,113.680975597964));
#40382=CARTESIAN_POINT('Ctrl Pts',(0.380950093949879,3.61351685606822,113.522606690179));
#40383=CARTESIAN_POINT('Ctrl Pts',(3.23844382823359,1.64936220470124,113.364237782395));
#40384=CARTESIAN_POINT('Ctrl Pts',(3.14662599275776,-1.81914961314222,113.205868874611));
#40385=CARTESIAN_POINT('Ctrl Pts',(0.187307898924319,-3.62941717620368,
113.047499966827));
#40386=CARTESIAN_POINT('Ctrl Pts',(-2.94235267289263,-2.1333501625449,112.889131059043));
#40387=CARTESIAN_POINT('Ctrl Pts',(-3.3914033194749,1.30661598684926,112.730762151259));
#40388=CARTESIAN_POINT('Ctrl Pts',(-0.750476860684186,3.55602193007364,
112.572393243474));
#40389=CARTESIAN_POINT('Ctrl Pts',(2.5741661903379,2.56560124653058,112.41402433569));
#40390=CARTESIAN_POINT('Ctrl Pts',(3.55351496501208,-0.762357962940957,
112.255655427906));
#40391=CARTESIAN_POINT('Ctrl Pts',(1.29525697823035,-3.3957214333461,112.097286520122));
#40392=CARTESIAN_POINT('Ctrl Pts',(-2.1431003513736,-2.93526067758035,111.938917612338));
#40393=CARTESIAN_POINT('Ctrl Pts',(-3.62888829547523,0.19951044313998,111.780548704554));
#40394=CARTESIAN_POINT('Ctrl Pts',(-1.80840610088971,3.15250643855389,111.622179796769));
#40395=CARTESIAN_POINT('Ctrl Pts',(1.65970856721919,3.23326456230892,111.463810888985));
#40396=CARTESIAN_POINT('Ctrl Pts',(3.61566828494496,0.368204981509806,111.305441981201));
#40397=CARTESIAN_POINT('Ctrl Pts',(2.27740374291247,-2.83232477754531,111.147073073417));
#40398=CARTESIAN_POINT('Ctrl Pts',(-1.13579615117146,-3.4523323912807,110.988704165633));
#40399=CARTESIAN_POINT('Ctrl Pts',(-3.51417576242243,-0.926930682705363,
110.830335257848));
#40400=CARTESIAN_POINT('Ctrl Pts',(-2.69080078557179,2.44299464705653,110.671966350064));
#40401=CARTESIAN_POINT('Ctrl Pts',(0.584154374749769,3.58711519621666,110.51359744228));
#40402=CARTESIAN_POINT('Ctrl Pts',(3.32688831376596,1.4630262817106,110.355228534496));
#40403=CARTESIAN_POINT('Ctrl Pts',(3.03850469400245,-1.9940213065136,110.196859626712));
#40404=CARTESIAN_POINT('Ctrl Pts',(-0.0182510645473885,-3.63432230981833,
110.038490718928));
#40405=CARTESIAN_POINT('Ctrl Pts',(-3.05837833591408,-1.96340360229389,
109.880121811143));
#40406=CARTESIAN_POINT('Ctrl Pts',(-3.31202665354681,1.49636599688186,109.721752903359));
#40407=CARTESIAN_POINT('Ctrl Pts',(-0.548097827727379,3.59280120832229,
109.563383995575));
#40408=CARTESIAN_POINT('Ctrl Pts',(2.71520121782699,2.41584645573589,109.405015087791));
#40409=CARTESIAN_POINT('Ctrl Pts',(3.50468891083895,-0.962178460146911,
109.246646180007));
#40410=CARTESIAN_POINT('Ctrl Pts',(1.1010654791205,-3.46356558501832,109.088277272223));
#40411=CARTESIAN_POINT('Ctrl Pts',(-2.30573527302542,-2.80930891888302,
108.929908364438));
#40412=CARTESIAN_POINT('Ctrl Pts',(-3.61178781659568,0.404500332358161,
108.771539456654));
#40413=CARTESIAN_POINT('Ctrl Pts',(-1.62715175675016,3.24977059367342,108.61317054887));
#40414=CARTESIAN_POINT('Ctrl Pts',(1.83997718857821,3.13418501312623,108.454801641086));
#40415=CARTESIAN_POINT('Ctrl Pts',(3.63070866194348,0.163053252289208,108.296432733302));
#40416=CARTESIAN_POINT('Ctrl Pts',(2.11351280876615,-2.95663581764418,108.138063825517));
#40417=CARTESIAN_POINT('Ctrl Pts',(-1.32929796592752,-3.38254322496773,
107.979694917733));
#40418=CARTESIAN_POINT('Ctrl Pts',(-3.56098951403573,-0.726626060585297,
107.821326009949));
#40419=CARTESIAN_POINT('Ctrl Pts',(-2.54827463359117,2.59131783901361,107.662957102165));
#40420=CARTESIAN_POINT('Ctrl Pts',(0.78616530960755,3.54832014578222,107.504588194381));
#40421=CARTESIAN_POINT('Ctrl Pts',(3.40433249369181,1.27245904585901,107.346219286597));
#40422=CARTESIAN_POINT('Ctrl Pts',(2.92082297136322,-2.16273551803063,107.187850378812));
#40423=CARTESIAN_POINT('Ctrl Pts',(-0.223839241138819,-3.62746850367038,
107.029481471028));
#40424=CARTESIAN_POINT('Ctrl Pts',(-3.16456221988273,-1.78722626085373,
106.871112563244));
#40425=CARTESIAN_POINT('Ctrl Pts',(-3.22206244009988,1.68135224836795,106.71274365546));
#40426=CARTESIAN_POINT('Ctrl Pts',(-0.343951630670548,3.61805597341353,
106.554374747676));
#40427=CARTESIAN_POINT('Ctrl Pts',(2.84753243561908,2.25836019693307,106.396005839891));
#40428=CARTESIAN_POINT('Ctrl Pts',(3.44463859003301,-1.15892050419763,106.237636932107));
#40429=CARTESIAN_POINT('Ctrl Pts',(0.903345279496379,-3.52031235219348,
106.079268024323));
#40430=CARTESIAN_POINT('Ctrl Pts',(-2.46098309487547,-2.67435860679368,
105.920899116539));
#40431=CARTESIAN_POINT('Ctrl Pts',(-3.58311745488613,0.60819491570108,105.762530208755));
#40432=CARTESIAN_POINT('Ctrl Pts',(-1.4406846885203,3.33662394933224,105.604161300971));
#40433=CARTESIAN_POINT('Ctrl Pts',(2.01435139962717,3.02506531992523,105.445792393186));
#40434=CARTESIAN_POINT('Ctrl Pts',(3.63411821653544,-0.0426208779773826,
105.287423485402));
#40435=CARTESIAN_POINT('Ctrl Pts',(1.94285127235686,-3.0714753270205,105.129054577618));
#40436=CARTESIAN_POINT('Ctrl Pts',(-1.51854140033388,-3.30191819499912,
104.970685669834));
#40437=CARTESIAN_POINT('Ctrl Pts',(-3.59639574418431,-0.523993704358454,
104.81231676205));
#40438=CARTESIAN_POINT('Ctrl Pts',(-2.39758515373452,2.73133981437429,104.653947854266));
#40439=CARTESIAN_POINT('Ctrl Pts',(0.985657784836226,3.49815815568509,104.495578946481));
#40440=CARTESIAN_POINT('Ctrl Pts',(3.47087099294263,1.07781552287194,104.337210038697));
#40441=CARTESIAN_POINT('Ctrl Pts',(2.79378447570712,-2.32452146780626,104.178841130913));
#40442=CARTESIAN_POINT('Ctrl Pts',(-0.428710354933595,-3.60899420650229,
104.020472223129));
#40443=CARTESIAN_POINT('Ctrl Pts',(-3.26060851966125,-1.60532359121354,
103.862103315345));
#40444=CARTESIAN_POINT('Ctrl Pts',(-3.12177644199792,1.86095233608523,103.703734407561));
#40445=CARTESIAN_POINT('Ctrl Pts',(-0.138703594458174,3.63172040001413,
103.545365499776));
#40446=CARTESIAN_POINT('Ctrl Pts',(2.97074166494909,2.09363934600253,103.386996591992));
#40447=CARTESIAN_POINT('Ctrl Pts',(3.37355346830678,-1.35194997964774,103.228627684208));
#40448=CARTESIAN_POINT('Ctrl Pts',(0.702731239185455,-3.56578189973352,
103.070258776424));
#40449=CARTESIAN_POINT('Ctrl Pts',(-2.6083472279764,-2.5308410636194,102.91188986864));
#40450=CARTESIAN_POINT('Ctrl Pts',(-3.54296867919103,0.809941164076495,
102.753520960855));
#40451=CARTESIAN_POINT('Ctrl Pts',(-1.24960242821741,3.41278852588135,102.595152053071));
#40452=CARTESIAN_POINT('Ctrl Pts',(2.18227269374953,2.90625491674587,102.436783145287));
#40453=CARTESIAN_POINT('Ctrl Pts',(3.62588597766565,-0.248158473483804,
102.278414237503));
#40454=CARTESIAN_POINT('Ctrl Pts',(1.76596586762753,-3.17647545329235,102.120045329719));
#40455=CARTESIAN_POINT('Ctrl Pts',(-1.70292023092382,-3.21071556480869,
101.961676421935));
#40456=CARTESIAN_POINT('Ctrl Pts',(-3.62028102372934,-0.319682749330519,
101.80330751415));
#40457=CARTESIAN_POINT('Ctrl Pts',(-2.23921507861287,2.86261202098834,101.644938606366));
#40458=CARTESIAN_POINT('Ctrl Pts',(1.18199273362486,3.43678991628124,101.486569698582));
#40459=CARTESIAN_POINT('Ctrl Pts',(3.52629065652986,0.879719248774588,101.328200790798));
#40460=CARTESIAN_POINT('Ctrl Pts',(2.65779617162307,-2.47886087973892,101.169831883014));
#40461=CARTESIAN_POINT('Ctrl Pts',(-0.632208107403957,-3.578958599918,101.01146297523));
#40462=CARTESIAN_POINT('Ctrl Pts',(-3.34620955357793,-1.41827831349775,
100.853094067445));
#40463=CARTESIAN_POINT('Ctrl Pts',(-3.01148992261249,2.03459091637546,100.694725159661));
#40464=CARTESIAN_POINT('Ctrl Pts',(0.0669887747403652,3.63375071448961,
100.536356251877));
#40465=CARTESIAN_POINT('Ctrl Pts',(3.08443420857142,1.92221158148316,100.377987344093));
#40466=CARTESIAN_POINT('Ctrl Pts',(3.29166126481559,-1.54064852211846,100.219618436309));
#40467=CARTESIAN_POINT('Ctrl Pts',(0.499866019507705,-3.59982856724333,
100.061249528525));
#40468=CARTESIAN_POINT('Ctrl Pts',(-2.74735559555312,-2.37921604369379,
99.9028806207401));
#40469=CARTESIAN_POINT('Ctrl Pts',(-3.49147010496271,1.00909278916312,99.7445117129559));
#40470=CARTESIAN_POINT('Ctrl Pts',(-1.05451710238043,3.4780203322898,99.5861428051718));
#40471=CARTESIAN_POINT('Ctrl Pts',(2.34320313989566,2.77813440929543,99.4277738973876));
#40472=CARTESIAN_POINT('Ctrl Pts',(3.60603831707632,-0.452901100416202,
99.2694049896035));
#40473=CARTESIAN_POINT('Ctrl Pts',(1.5834232418962,-3.27129983161196,99.1110360818192));
#40474=CARTESIAN_POINT('Ctrl Pts',(-1.88184380539861,-3.1092274993174,98.9526671740351));
#40475=CARTESIAN_POINT('Ctrl Pts',(-3.63256883687055,-0.11434769996046,
98.794298266251));
#40476=CARTESIAN_POINT('Ctrl Pts',(-2.07367174220406,2.98471393245394,98.6359293584666));
#40477=CARTESIAN_POINT('Ctrl Pts',(1.37454120256743,3.3644120182804,98.4775604506826));
#40478=CARTESIAN_POINT('Ctrl Pts',(3.57041394920919,0.6788048206525,98.3191915428984));
#40479=CARTESIAN_POINT('Ctrl Pts',(2.51329369362716,-2.62525933462612,98.1608226351142));
#40480=CARTESIAN_POINT('Ctrl Pts',(-0.833680599109368,-3.5374578968306,
98.00245372733));
#40481=CARTESIAN_POINT('Ctrl Pts',(-3.42109110162642,-1.2266896323482,97.8440848195459));
#40482=CARTESIAN_POINT('Ctrl Pts',(-2.89155618075458,2.2017117637061,97.6857159117615));
#40483=CARTESIAN_POINT('Ctrl Pts',(0.272466545560592,3.624140371906,97.5273470039775));
#40484=CARTESIAN_POINT('Ctrl Pts',(3.1882458591633,1.74462614811699,97.3689780961933));
#40485=CARTESIAN_POINT('Ctrl Pts',(3.19922431200574,-1.72441180100781,97.2106091884092));
#40486=CARTESIAN_POINT('Ctrl Pts',(0.295399506973262,-3.6223429713569,97.0522402806248));
#40487=CARTESIAN_POINT('Ctrl Pts',(-2.87756291517,-2.21996989781333,96.8938713728408));
#40488=CARTESIAN_POINT('Ctrl Pts',(-3.4287866532623,1.20501304881627,96.7355024650567));
#40489=CARTESIAN_POINT('Ctrl Pts',(-0.856053766316002,3.53210796008794,
96.5771335572723));
#40490=CARTESIAN_POINT('Ctrl Pts',(2.49662740969472,2.64111905210372,96.4187646494883));
#40491=CARTESIAN_POINT('Ctrl Pts',(3.57463840557985,-0.656202408584182,
96.2603957417041));
#40492=CARTESIAN_POINT('Ctrl Pts',(1.39580897694624,-3.35562584110079,96.1020268339198));
#40493=CARTESIAN_POINT('Ctrl Pts',(-2.0547405519129,-2.99781638476409,95.9436579261358));
#40494=CARTESIAN_POINT('Ctrl Pts',(-3.63321664764495,0.0914273426514201,
95.7852890183515));
#40495=CARTESIAN_POINT('Ctrl Pts',(-1.90149172882987,3.09710873123844,95.6269201105673));
#40496=CARTESIAN_POINT('Ctrl Pts',(1.56269876086743,3.28154430658457,95.4685512027832));
#40497=CARTESIAN_POINT('Ctrl Pts',(3.60307507738476,0.475146396019093,95.310182294999));
#40498=CARTESIAN_POINT('Ctrl Pts',(2.36078764608376,-2.76212033287254,95.1518133872148));
#40499=CARTESIAN_POINT('Ctrl Pts',(-1.03256917122443,-3.4868746092295,94.9934444794307));
#40500=CARTESIAN_POINT('Ctrl Pts',(-3.48492740853102,-1.02648407117314,
94.8350755716465));
#40501=CARTESIAN_POINT('Ctrl Pts',(-3.00240564212693,1.22403504121547,94.7294962997903));
#40502=CARTESIAN_POINT('Ctrl Pts',(-2.33907288663243,1.99987526141664,94.6767066638623));
#40503=CARTESIAN_POINT('Ctrl Pts',(-0.746309486510706,-2.79158637039142,
114.106160313476));
#40504=CARTESIAN_POINT('Ctrl Pts',(-1.67224257593793,-2.54404516735251,
114.053370677548));
#40505=CARTESIAN_POINT('Ctrl Pts',(-3.24259860713048,-1.0592266416515,113.947791405692));
#40506=CARTESIAN_POINT('Ctrl Pts',(-2.6535621244696,2.1489603211384,113.789422497907));
#40507=CARTESIAN_POINT('Ctrl Pts',(0.357698465790113,3.39296263749542,113.631053590123));
#40508=CARTESIAN_POINT('Ctrl Pts',(3.04078252585762,1.54869191404229,113.472684682339));
#40509=CARTESIAN_POINT('Ctrl Pts',(2.95456887371925,-1.70811619684037,113.314315774555));
#40510=CARTESIAN_POINT('Ctrl Pts',(0.175875394545547,-3.40789246743471,
113.155946866771));
#40511=CARTESIAN_POINT('Ctrl Pts',(-2.76276355780503,-2.00313923596458,
112.997577958987));
#40512=CARTESIAN_POINT('Ctrl Pts',(-3.1844059983649,1.22686551675796,112.839209051202));
#40513=CARTESIAN_POINT('Ctrl Pts',(-0.704670837311911,3.33897696549902,
112.680840143418));
#40514=CARTESIAN_POINT('Ctrl Pts',(2.4170496650246,2.40900749018828,112.522471235634));
#40515=CARTESIAN_POINT('Ctrl Pts',(3.33662301528205,-0.715826765914207,
112.36410232785));
#40516=CARTESIAN_POINT('Ctrl Pts',(1.2161998153435,-3.18846055231137,112.205733420066));
#40517=CARTESIAN_POINT('Ctrl Pts',(-2.01229431333713,-2.75610442874092,
112.047364512282));
#40518=CARTESIAN_POINT('Ctrl Pts',(-3.4073958674124,0.18733314561058,111.888995604497));
#40519=CARTESIAN_POINT('Ctrl Pts',(-1.69802842442358,2.96009040127061,111.730626696713));
#40520=CARTESIAN_POINT('Ctrl Pts',(1.55840677711217,3.03591938103998,111.572257788929));
#40521=CARTESIAN_POINT('Ctrl Pts',(3.39498275199517,0.345731262635315,111.413888881145));
#40522=CARTESIAN_POINT('Ctrl Pts',(2.13840037779758,-2.65945131301259,111.255519973361));
#40523=CARTESIAN_POINT('Ctrl Pts',(-1.06647182183869,-3.24161621002536,
111.097151065577));
#40524=CARTESIAN_POINT('Ctrl Pts',(-3.29968491594777,-0.870354643201932,
110.938782157792));
#40525=CARTESIAN_POINT('Ctrl Pts',(-2.52656536389381,2.29388429367482,110.780413250008));
#40526=CARTESIAN_POINT('Ctrl Pts',(0.548499992390253,3.36817242645937,110.622044342224));
#40527=CARTESIAN_POINT('Ctrl Pts',(3.12382872346976,1.37372917001392,110.46367543444));
#40528=CARTESIAN_POINT('Ctrl Pts',(2.85304685469831,-1.87231444071136,110.305306526655));
#40529=CARTESIAN_POINT('Ctrl Pts',(-0.0171370945730645,-3.41249821185194,
110.146937618871));
#40530=CARTESIAN_POINT('Ctrl Pts',(-2.87170749118155,-1.84356551532891,
109.988568711087));
#40531=CARTESIAN_POINT('Ctrl Pts',(-3.10987415791403,1.40503396598599,109.830199803303));
#40532=CARTESIAN_POINT('Ctrl Pts',(-0.514644188817999,3.37351138775366,
109.671830895519));
#40533=CARTESIAN_POINT('Ctrl Pts',(2.5494764940416,2.26839311638259,109.513461987735));
#40534=CARTESIAN_POINT('Ctrl Pts',(3.29077710279722,-0.903451041164788,
109.35509307995));
#40535=CARTESIAN_POINT('Ctrl Pts',(1.03386096727849,-3.25216377578184,109.196724172166));
#40536=CARTESIAN_POINT('Ctrl Pts',(-2.16500266774537,-2.63784024777573,
109.038355264382));
#40537=CARTESIAN_POINT('Ctrl Pts',(-3.39133913148654,0.379811294429396,
108.879986356598));
#40538=CARTESIAN_POINT('Ctrl Pts',(-1.52783710055678,3.05141795208415,108.721617448814));
#40539=CARTESIAN_POINT('Ctrl Pts',(1.72767254266597,2.94288724035625,108.56324854103));
#40540=CARTESIAN_POINT('Ctrl Pts',(3.40910512619251,0.153101151862722,108.404879633246));
#40541=CARTESIAN_POINT('Ctrl Pts',(1.98451267273572,-2.7761749180998,108.246510725461));
#40542=CARTESIAN_POINT('Ctrl Pts',(-1.24816308104848,-3.17608668761447,
108.088141817677));
#40543=CARTESIAN_POINT('Ctrl Pts',(-3.34364134855115,-0.682275792032408,
107.929772909893));
#40544=CARTESIAN_POINT('Ctrl Pts',(-2.39273842249622,2.43315444755258,107.771404002109));
#40545=CARTESIAN_POINT('Ctrl Pts',(0.738181009980343,3.33174526646904,107.613035094325));
#40546=CARTESIAN_POINT('Ctrl Pts',(3.1965460289221,1.19479337507238,107.45466618654));
#40547=CARTESIAN_POINT('Ctrl Pts',(2.74254794077725,-2.03073103011525,107.296297278756));
#40548=CARTESIAN_POINT('Ctrl Pts',(-0.210177013762628,-3.40606273386447,
107.137928370972));
#40549=CARTESIAN_POINT('Ctrl Pts',(-2.97141034725229,-1.67814131478147,
106.979559463188));
#40550=CARTESIAN_POINT('Ctrl Pts',(-3.02540099033367,1.57872941691175,106.821190555404));
#40551=CARTESIAN_POINT('Ctrl Pts',(-0.322958236658289,3.3972247057722,106.66282164762));
#40552=CARTESIAN_POINT('Ctrl Pts',(2.67373075813582,2.1205191716023,106.504452739835));
#40553=CARTESIAN_POINT('Ctrl Pts',(3.23439200678694,-1.08818475938934,106.346083832051));
#40554=CARTESIAN_POINT('Ctrl Pts',(0.848208796076863,-3.30544695349847,
106.187714924267));
#40555=CARTESIAN_POINT('Ctrl Pts',(-2.31077480056528,-2.51112674813657,
106.029346016483));
#40556=CARTESIAN_POINT('Ctrl Pts',(-3.36441869083031,0.571073197520321,
105.870977108699));
#40557=CARTESIAN_POINT('Ctrl Pts',(-1.35275121585564,3.13297013585121,105.712608200914));
#40558=CARTESIAN_POINT('Ctrl Pts',(1.89140366849103,2.84042776478352,105.55423929313));
#40559=CARTESIAN_POINT('Ctrl Pts',(3.41230657558429,-0.0400194747429137,
105.395870385346));
#40560=CARTESIAN_POINT('Ctrl Pts',(1.82426761514817,-2.88400509577499,105.237501477562));
#40561=CARTESIAN_POINT('Ctrl Pts',(-1.42585587394465,-3.10038267813378,
105.079132569778));
#40562=CARTESIAN_POINT('Ctrl Pts',(-3.37688652791896,-0.49201128207979,
104.920763661994));
#40563=CARTESIAN_POINT('Ctrl Pts',(-2.25124640920767,2.56463005697977,104.762394754209));
#40564=CARTESIAN_POINT('Ctrl Pts',(0.925497284367084,3.28464495809877,104.604025846425));
#40565=CARTESIAN_POINT('Ctrl Pts',(3.25902329162918,1.01203009280996,104.445656938641));
#40566=CARTESIAN_POINT('Ctrl Pts',(2.62326335281111,-2.18264223040164,104.287288030857));
#40567=CARTESIAN_POINT('Ctrl Pts',(-0.402543636721763,-3.38871603187245,
104.128919123073));
#40568=CARTESIAN_POINT('Ctrl Pts',(-3.06159437560986,-1.50734123653821,
103.970550215289));
#40569=CARTESIAN_POINT('Ctrl Pts',(-2.93123603741461,1.74736745336986,103.812181307504));
#40570=CARTESIAN_POINT('Ctrl Pts',(-0.130237697076901,3.41005511192923,
103.65381239972));
#40571=CARTESIAN_POINT('Ctrl Pts',(2.78941980245543,1.96585220446606,103.495443491936));
#40572=CARTESIAN_POINT('Ctrl Pts',(3.16764562875528,-1.26943250894327,103.337074584152));
#40573=CARTESIAN_POINT('Ctrl Pts',(0.659839412331244,-3.348141226721,103.178705676368));
#40574=CARTESIAN_POINT('Ctrl Pts',(-2.44914443259804,-2.37636892598951,
103.020336768584));
#40575=CARTESIAN_POINT('Ctrl Pts',(-3.32672043140588,0.760505684003158,
102.861967860799));
#40576=CARTESIAN_POINT('Ctrl Pts',(-1.17333183143872,3.2044859396582,102.703598953015));
#40577=CARTESIAN_POINT('Ctrl Pts',(2.04907573691939,2.72886906034401,102.545230045231));
#40578=CARTESIAN_POINT('Ctrl Pts',(3.40457679874342,-0.233011900109024,
102.386861137447));
#40579=CARTESIAN_POINT('Ctrl Pts',(1.65817856858484,-2.98259644585391,102.228492229663));
#40580=CARTESIAN_POINT('Ctrl Pts',(-1.59898097844946,-3.01474668167847,
102.070123321878));
#40581=CARTESIAN_POINT('Ctrl Pts',(-3.39931394816092,-0.300170628098432,
101.911754414094));
#40582=CARTESIAN_POINT('Ctrl Pts',(-2.10254259262445,2.68788994758611,101.75338550631));
#40583=CARTESIAN_POINT('Ctrl Pts',(1.10984875475132,3.22702238382561,101.595016598526));
#40584=CARTESIAN_POINT('Ctrl Pts',(3.31106036670697,0.826024801175402,101.436647690742));
#40585=CARTESIAN_POINT('Ctrl Pts',(2.4955752159428,-2.32756139891226,101.278278782958));
#40586=CARTESIAN_POINT('Ctrl Pts',(-0.593620722687675,-3.36051367527798,
101.119909875173));
#40587=CARTESIAN_POINT('Ctrl Pts',(-3.14197067420732,-1.3317124338819,100.961540967389));
#40588=CARTESIAN_POINT('Ctrl Pts',(-2.8276809539325,1.91040784831451,100.803172059605));
#40589=CARTESIAN_POINT('Ctrl Pts',(0.0629000552312259,3.41196150435303,
100.644803151821));
#40590=CARTESIAN_POINT('Ctrl Pts',(2.89617302045262,1.80488768618331,100.486434244037));
#40591=CARTESIAN_POINT('Ctrl Pts',(3.09075178881617,-1.44661366786822,100.328065336253));
#40592=CARTESIAN_POINT('Ctrl Pts',(0.469356251955776,-3.38010982556621,
100.169696428468));
#40593=CARTESIAN_POINT('Ctrl Pts',(-2.57966830069486,-2.23399847415303,
100.011327520684));
#40594=CARTESIAN_POINT('Ctrl Pts',(-3.27836511850688,0.947501912339738,
99.8529586129002));
#40595=CARTESIAN_POINT('Ctrl Pts',(-0.990153712156691,3.26573626468394,
99.6945897051162));
#40596=CARTESIAN_POINT('Ctrl Pts',(2.20018365000201,2.60856850213676,99.5362207973317));
#40597=CARTESIAN_POINT('Ctrl Pts',(3.38594055778935,-0.425257878515824,
99.3778518895479));
#40598=CARTESIAN_POINT('Ctrl Pts',(1.48677759454023,-3.07163313381674,99.2194829817636));
#40599=CARTESIAN_POINT('Ctrl Pts',(-1.76698379325318,-2.91945303062344,
99.0611140739795));
#40600=CARTESIAN_POINT('Ctrl Pts',(-3.41085176368671,-0.107368386284913,
98.9027451661953));
#40601=CARTESIAN_POINT('Ctrl Pts',(-1.94710334114339,2.80253926017304,98.7443762584111));
#40602=CARTESIAN_POINT('Ctrl Pts',(1.29064485645816,3.15906213527026,98.5860073506268));
#40603=CARTESIAN_POINT('Ctrl Pts',(3.35249055493281,0.637373364056125,98.4276384428428));
#40604=CARTESIAN_POINT('Ctrl Pts',(2.3598925753479,-2.46502429376086,98.2692695350585));
#40605=CARTESIAN_POINT('Ctrl Pts',(-0.782796161482605,-3.32154600455329,
98.1109006272744));
#40606=CARTESIAN_POINT('Ctrl Pts',(-3.21228176030053,-1.15181753846559,
97.9525317194901));
#40607=CARTESIAN_POINT('Ctrl Pts',(-2.71506747479084,2.06732832593376,97.7941628117061));
#40608=CARTESIAN_POINT('Ctrl Pts',(0.255836307364129,3.4029377375855,97.6357939039218));
#40609=CARTESIAN_POINT('Ctrl Pts',(2.99364843452285,1.63814133785425,97.4774249961376));
#40610=CARTESIAN_POINT('Ctrl Pts',(3.00395680772149,-1.61916079141855,97.3190560883535));
#40611=CARTESIAN_POINT('Ctrl Pts',(0.27736953505882,-3.4012500429792,97.1606871805693));
#40612=CARTESIAN_POINT('Ctrl Pts',(-2.70192830062999,-2.08447205856978,
97.0023182727851));
#40613=CARTESIAN_POINT('Ctrl Pts',(-3.21950760709066,1.13146400450909,96.8439493650011));
#40614=CARTESIAN_POINT('Ctrl Pts',(-0.803803762509031,3.31652260596299,
96.6855804572166));
#40615=CARTESIAN_POINT('Ctrl Pts',(2.34424353289394,2.47991599926166,96.5272115494327));
#40616=CARTESIAN_POINT('Ctrl Pts',(3.35645716784768,-0.616150510332253,
96.3688426416484));
#40617=CARTESIAN_POINT('Ctrl Pts',(1.31061453329219,-3.1508122302375,96.2104737338642));
#40618=CARTESIAN_POINT('Ctrl Pts',(-1.92932763290688,-2.81484199264079,
96.0521048260802));
#40619=CARTESIAN_POINT('Ctrl Pts',(-3.41146003475373,0.0858469933911683,
95.8937359182958));
#40620=CARTESIAN_POINT('Ctrl Pts',(-1.78543248818445,2.90807394234403,95.7353670105118));
#40621=CARTESIAN_POINT('Ctrl Pts',(1.4673180506629,3.08125232813832,95.5769981027275));
#40622=CARTESIAN_POINT('Ctrl Pts',(3.38315818207064,0.446145412695689,95.4186291949435));
#40623=CARTESIAN_POINT('Ctrl Pts',(2.2166948701987,-2.59353185912633,95.2602602871591));
#40624=CARTESIAN_POINT('Ctrl Pts',(-0.969545392519947,-3.2740501129473,
95.101891379375));
#40625=CARTESIAN_POINT('Ctrl Pts',(-3.27222176137714,-0.963831701968104,
94.9435224715908));
#40626=CARTESIAN_POINT('Ctrl Pts',(-2.81915114059448,1.14932497266615,94.8379431997347));
#40627=CARTESIAN_POINT('Ctrl Pts',(-2.19630549042403,1.87781109426488,94.7851535638067));
#40628=CARTESIAN_POINT('Ctrl Pts',(-0.697796808006135,-2.61012367354467,
114.214607213421));
#40629=CARTESIAN_POINT('Ctrl Pts',(-1.56354106813931,-2.37867349844622,
114.161817577493));
#40630=CARTESIAN_POINT('Ctrl Pts',(-3.03181856669101,-0.990373273901665,
114.056238305636));
#40631=CARTESIAN_POINT('Ctrl Pts',(-2.4810714774082,2.00927052345691,113.897869397852));
#40632=CARTESIAN_POINT('Ctrl Pts',(0.334446837630344,3.17240841892262,113.739500490068));
#40633=CARTESIAN_POINT('Ctrl Pts',(2.84312122348166,1.44802162338334,113.581131582284));
#40634=CARTESIAN_POINT('Ctrl Pts',(2.76251175468075,-1.59708278053852,113.4227626745));
#40635=CARTESIAN_POINT('Ctrl Pts',(0.164442890166777,-3.18636775866573,
113.264393766716));
#40636=CARTESIAN_POINT('Ctrl Pts',(-2.58317444271743,-1.87292830938426,
113.106024858931));
#40637=CARTESIAN_POINT('Ctrl Pts',(-2.97740867725489,1.14711504666666,112.947655951147));
#40638=CARTESIAN_POINT('Ctrl Pts',(-0.658864813939638,3.12193200092439,
112.789287043363));
#40639=CARTESIAN_POINT('Ctrl Pts',(2.2599331397113,2.25241373384597,112.630918135579));
#40640=CARTESIAN_POINT('Ctrl Pts',(3.11973106555201,-0.669295568887458,
112.472549227795));
#40641=CARTESIAN_POINT('Ctrl Pts',(1.13714265245665,-2.98119967127663,112.314180320011));
#40642=CARTESIAN_POINT('Ctrl Pts',(-1.88148827530065,-2.5769481799015,112.155811412226));
#40643=CARTESIAN_POINT('Ctrl Pts',(-3.18590343934957,0.175155848081176,
111.997442504442));
#40644=CARTESIAN_POINT('Ctrl Pts',(-1.58765074795745,2.76767436398734,111.839073596658));
#40645=CARTESIAN_POINT('Ctrl Pts',(1.45710498700515,2.83857419977103,111.680704688874));
#40646=CARTESIAN_POINT('Ctrl Pts',(3.17429721904537,0.323257543760826,111.52233578109));
#40647=CARTESIAN_POINT('Ctrl Pts',(1.99939701268271,-2.48657784847987,111.363966873305));
#40648=CARTESIAN_POINT('Ctrl Pts',(-0.997147492505912,-3.03090002877003,
111.205597965521));
#40649=CARTESIAN_POINT('Ctrl Pts',(-3.0851940694731,-0.813778603698501,
111.047229057737));
#40650=CARTESIAN_POINT('Ctrl Pts',(-2.36232994221583,2.14477394029311,110.888860149953));
#40651=CARTESIAN_POINT('Ctrl Pts',(0.512845610030737,3.14922965670211,110.730491242169));
#40652=CARTESIAN_POINT('Ctrl Pts',(2.92076913317356,1.28443205831725,110.572122334385));
#40653=CARTESIAN_POINT('Ctrl Pts',(2.66758901539418,-1.75060757490912,110.4137534266));
#40654=CARTESIAN_POINT('Ctrl Pts',(-0.0160231245987433,-3.19067411388555,
110.255384518816));
#40655=CARTESIAN_POINT('Ctrl Pts',(-2.68503664644901,-1.72372742836392,
110.097015611032));
#40656=CARTESIAN_POINT('Ctrl Pts',(-2.90772166228126,1.31370193509011,109.938646703248));
#40657=CARTESIAN_POINT('Ctrl Pts',(-0.48119054990862,3.15422156718503,109.780277795464));
#40658=CARTESIAN_POINT('Ctrl Pts',(2.38375177025621,2.12093977702929,109.62190888768));
#40659=CARTESIAN_POINT('Ctrl Pts',(3.07686529475549,-0.844723622182665,
109.463539979895));
#40660=CARTESIAN_POINT('Ctrl Pts',(0.966656455436494,-3.04076196654535,
109.305171072111));
#40661=CARTESIAN_POINT('Ctrl Pts',(-2.02427006246532,-2.46637157666842,
109.146802164327));
#40662=CARTESIAN_POINT('Ctrl Pts',(-3.17089044637737,0.355122256500635,
108.988433256543));
#40663=CARTESIAN_POINT('Ctrl Pts',(-1.4285224443634,2.85306531049488,108.830064348759));
#40664=CARTESIAN_POINT('Ctrl Pts',(1.61536789675373,2.75158946758626,108.671695440975));
#40665=CARTESIAN_POINT('Ctrl Pts',(3.18750159044155,0.143149051436234,108.51332653319));
#40666=CARTESIAN_POINT('Ctrl Pts',(1.8555125367053,-2.59571401855541,108.354957625406));
#40667=CARTESIAN_POINT('Ctrl Pts',(-1.16702819616944,-2.96963015026121,
108.196588717622));
#40668=CARTESIAN_POINT('Ctrl Pts',(-3.12629318306656,-0.63792552347952,
108.038219809838));
#40669=CARTESIAN_POINT('Ctrl Pts',(-2.23720221140127,2.27499105609152,107.879850902054));
#40670=CARTESIAN_POINT('Ctrl Pts',(0.690196710353136,3.11517038715585,107.72148199427));
#40671=CARTESIAN_POINT('Ctrl Pts',(2.98875956415239,1.11712770428576,107.563113086485));
#40672=CARTESIAN_POINT('Ctrl Pts',(2.56427291019128,-1.89872654219987,107.404744178701));
#40673=CARTESIAN_POINT('Ctrl Pts',(-0.196514786386437,-3.18465696405854,
107.246375270917));
#40674=CARTESIAN_POINT('Ctrl Pts',(-2.77825847462185,-1.56905636870923,
107.088006363133));
#40675=CARTESIAN_POINT('Ctrl Pts',(-2.82873954056747,1.47610658545555,106.929637455349));
#40676=CARTESIAN_POINT('Ctrl Pts',(-0.30196484264603,3.17639343813087,106.771268547564));
#40677=CARTESIAN_POINT('Ctrl Pts',(2.49992908065257,1.98267814627153,106.61289963978));
#40678=CARTESIAN_POINT('Ctrl Pts',(3.02414542354086,-1.01744901458105,106.454530731996));
#40679=CARTESIAN_POINT('Ctrl Pts',(0.793072312657348,-3.09058155480347,
106.296161824212));
#40680=CARTESIAN_POINT('Ctrl Pts',(-2.16056650625509,-2.34789488947946,
106.137792916428));
#40681=CARTESIAN_POINT('Ctrl Pts',(-3.1457199267745,0.533951479339558,105.979424008644));
#40682=CARTESIAN_POINT('Ctrl Pts',(-1.26481774319096,2.92931632237019,105.821055100859));
#40683=CARTESIAN_POINT('Ctrl Pts',(1.76845593735489,2.65579020964182,105.662686193075));
#40684=CARTESIAN_POINT('Ctrl Pts',(3.19049493463312,-0.0374180715084452,
105.504317285291));
#40685=CARTESIAN_POINT('Ctrl Pts',(1.70568395793947,-2.69653486452949,105.345948377507));
#40686=CARTESIAN_POINT('Ctrl Pts',(-1.3331703475554,-2.89884716126845,105.187579469723));
#40687=CARTESIAN_POINT('Ctrl Pts',(-3.15737731165363,-0.460028859801123,
105.029210561938));
#40688=CARTESIAN_POINT('Ctrl Pts',(-2.10490766468081,2.39792029958526,104.870841654154));
#40689=CARTESIAN_POINT('Ctrl Pts',(0.865336783897941,3.07113176051245,104.71247274637));
#40690=CARTESIAN_POINT('Ctrl Pts',(3.04717559031573,0.946244662747985,104.554103838586));
#40691=CARTESIAN_POINT('Ctrl Pts',(2.45274222991511,-2.04076299299701,104.395734930802));
#40692=CARTESIAN_POINT('Ctrl Pts',(-0.376376918509931,-3.16843785724261,
104.237366023018));
#40693=CARTESIAN_POINT('Ctrl Pts',(-2.86258023155845,-1.40935888186287,
104.078997115233));
#40694=CARTESIAN_POINT('Ctrl Pts',(-2.74069563283132,1.6337825706545,103.920628207449));
#40695=CARTESIAN_POINT('Ctrl Pts',(-0.121771799695632,3.18838982384432,
103.762259299665));
#40696=CARTESIAN_POINT('Ctrl Pts',(2.60809793996178,1.83806506292957,103.603890391881));
#40697=CARTESIAN_POINT('Ctrl Pts',(2.96173778920377,-1.1869150382388,103.445521484097));
#40698=CARTESIAN_POINT('Ctrl Pts',(0.616947585477037,-3.13050055370848,
103.287152576312));
#40699=CARTESIAN_POINT('Ctrl Pts',(-2.28994163721969,-2.22189678835962,
103.128783668528));
#40700=CARTESIAN_POINT('Ctrl Pts',(-3.11047218362072,0.711070203929821,
102.970414760744));
#40701=CARTESIAN_POINT('Ctrl Pts',(-1.09706123466004,2.99618335343504,102.81204585296));
#40702=CARTESIAN_POINT('Ctrl Pts',(1.91587878008926,2.55148320394214,102.653676945176));
#40703=CARTESIAN_POINT('Ctrl Pts',(3.18326761982119,-0.217865326734245,
102.495308037392));
#40704=CARTESIAN_POINT('Ctrl Pts',(1.55039126954215,-2.78871743841547,102.336939129607));
#40705=CARTESIAN_POINT('Ctrl Pts',(-1.49504172597511,-2.81877779854825,
102.178570221823));
#40706=CARTESIAN_POINT('Ctrl Pts',(-3.17834687259251,-0.280658506866343,
102.020201314039));
#40707=CARTESIAN_POINT('Ctrl Pts',(-1.96587010663603,2.51316787418387,101.861832406255));
#40708=CARTESIAN_POINT('Ctrl Pts',(1.03770477587778,3.01725485136997,101.703463498471));
#40709=CARTESIAN_POINT('Ctrl Pts',(3.09583007688406,0.772330353576217,101.545094590687));
#40710=CARTESIAN_POINT('Ctrl Pts',(2.33335426026256,-2.1762619180856,101.386725682902));
#40711=CARTESIAN_POINT('Ctrl Pts',(-0.555033337971393,-3.14206875063794,
101.228356775118));
#40712=CARTESIAN_POINT('Ctrl Pts',(-2.9377317948367,-1.24514655426605,101.069987867334));
#40713=CARTESIAN_POINT('Ctrl Pts',(-2.6438719852525,1.78622478025355,100.91161895955));
#40714=CARTESIAN_POINT('Ctrl Pts',(0.058811335722083,3.19017229421644,100.753250051766));
#40715=CARTESIAN_POINT('Ctrl Pts',(2.70791183233384,1.68756379088345,100.594881143982));
#40716=CARTESIAN_POINT('Ctrl Pts',(2.88984231281674,-1.35257881361797,100.436512236197));
#40717=CARTESIAN_POINT('Ctrl Pts',(0.438846484403849,-3.16039108388907,
100.278143328413));
#40718=CARTESIAN_POINT('Ctrl Pts',(-2.41198100583659,-2.08878090461229,
100.119774420629));
#40719=CARTESIAN_POINT('Ctrl Pts',(-3.06526013205104,0.885911035516352,
99.9614055128444));
#40720=CARTESIAN_POINT('Ctrl Pts',(-0.925790321932956,3.05345219707809,
99.8030366050604));
#40721=CARTESIAN_POINT('Ctrl Pts',(2.05716416010835,2.43900259497809,99.6446676972761));
#40722=CARTESIAN_POINT('Ctrl Pts',(3.16584279850237,-0.397614656615443,
99.4862987894921));
#40723=CARTESIAN_POINT('Ctrl Pts',(1.39013194718426,-2.87196643602151,99.3279298817077));
#40724=CARTESIAN_POINT('Ctrl Pts',(-1.65212378110773,-2.72967856192949,
99.1695609739237));
#40725=CARTESIAN_POINT('Ctrl Pts',(-3.18913469050289,-0.100389072609364,
99.0111920661394));
#40726=CARTESIAN_POINT('Ctrl Pts',(-1.82053494008273,2.62036458789214,98.8528231583554));
#40727=CARTESIAN_POINT('Ctrl Pts',(1.2067485103489,2.95371225226013,98.694454250571));
#40728=CARTESIAN_POINT('Ctrl Pts',(3.13456716065645,0.59594190745975,98.536085342787));
#40729=CARTESIAN_POINT('Ctrl Pts',(2.20649145706861,-2.30478925289559,98.3777164350027));
#40730=CARTESIAN_POINT('Ctrl Pts',(-0.731911723855837,-3.10563411227598,
98.2193475272186));
#40731=CARTESIAN_POINT('Ctrl Pts',(-3.00347241897466,-1.07694544458298,
98.0609786194345));
#40732=CARTESIAN_POINT('Ctrl Pts',(-2.53857876882709,1.93294488816143,97.9026097116503));
#40733=CARTESIAN_POINT('Ctrl Pts',(0.239206069167667,3.18173510326499,97.7442408038659));
#40734=CARTESIAN_POINT('Ctrl Pts',(2.79905100988241,1.53165652759152,97.5858718960819));
#40735=CARTESIAN_POINT('Ctrl Pts',(2.80868930343724,-1.51390978182928,97.4275029882977));
#40736=CARTESIAN_POINT('Ctrl Pts',(0.259339563144376,-3.18015711460151,
97.2691340805136));
#40737=CARTESIAN_POINT('Ctrl Pts',(-2.52629368608997,-1.94897421932625,
97.1107651727293));
#40738=CARTESIAN_POINT('Ctrl Pts',(-3.01022856091902,1.05791496020191,96.9523962649453));
#40739=CARTESIAN_POINT('Ctrl Pts',(-0.751553758702059,3.10093725183804,
96.7940273571609));
#40740=CARTESIAN_POINT('Ctrl Pts',(2.19185965609315,2.31871294641959,96.6356584493769));
#40741=CARTESIAN_POINT('Ctrl Pts',(3.13827593011553,-0.576098612080323,
96.4772895415926));
#40742=CARTESIAN_POINT('Ctrl Pts',(1.22542008963813,-2.94599861937422,96.3189206338085));
#40743=CARTESIAN_POINT('Ctrl Pts',(-1.80391471390086,-2.6318676005175,96.1605517260244));
#40744=CARTESIAN_POINT('Ctrl Pts',(-3.18970342186251,0.0802666441309152,
96.0021828182401));
#40745=CARTESIAN_POINT('Ctrl Pts',(-1.66937324753903,2.7190391534496,95.843813910456));
#40746=CARTESIAN_POINT('Ctrl Pts',(1.37193734045838,2.88096034969207,95.6854450026717));
#40747=CARTESIAN_POINT('Ctrl Pts',(3.16324128675654,0.417144429372286,95.5270760948876));
#40748=CARTESIAN_POINT('Ctrl Pts',(2.07260209431364,-2.42494338538013,95.3687071871034));
#40749=CARTESIAN_POINT('Ctrl Pts',(-0.906521613815463,-3.06122561666511,
95.2103382793192));
#40750=CARTESIAN_POINT('Ctrl Pts',(-3.05951611422325,-0.901179332763063,
95.0519693715352));
#40751=CARTESIAN_POINT('Ctrl Pts',(-2.63589663906204,1.07461490411683,94.946390099679));
#40752=CARTESIAN_POINT('Ctrl Pts',(-2.05353809421562,1.75574692711312,94.8936004637509));
#40753=CARTESIAN_POINT('Ctrl Pts',(-0.649284129501564,-2.42866097669793,
114.323054113364));
#40754=CARTESIAN_POINT('Ctrl Pts',(-1.45483956034068,-2.21330182953991,
114.270264477436));
#40755=CARTESIAN_POINT('Ctrl Pts',(-2.82103852625153,-0.921519906151827,
114.16468520558));
#40756=CARTESIAN_POINT('Ctrl Pts',(-2.30858083034679,1.8695807257754,114.006316297796));
#40757=CARTESIAN_POINT('Ctrl Pts',(0.311195209470579,2.95185420034983,113.847947390012));
#40758=CARTESIAN_POINT('Ctrl Pts',(2.64545992110568,1.3473513327244,113.689578482228));
#40759=CARTESIAN_POINT('Ctrl Pts',(2.57045463564224,-1.48604936423666,113.531209574444));
#40760=CARTESIAN_POINT('Ctrl Pts',(0.153010385788004,-2.96484304989676,
113.372840666659));
#40761=CARTESIAN_POINT('Ctrl Pts',(-2.40358532762983,-1.74271738280394,
113.214471758875));
#40762=CARTESIAN_POINT('Ctrl Pts',(-2.77041135614488,1.06736457657537,113.056102851091));
#40763=CARTESIAN_POINT('Ctrl Pts',(-0.613058790567363,2.90488703634978,
112.897733943307));
#40764=CARTESIAN_POINT('Ctrl Pts',(2.10281661439799,2.09581997750367,112.739365035523));
#40765=CARTESIAN_POINT('Ctrl Pts',(2.90283911582197,-0.622764371860707,
112.580996127739));
#40766=CARTESIAN_POINT('Ctrl Pts',(1.0580854895698,-2.7739387902419,112.422627219954));
#40767=CARTESIAN_POINT('Ctrl Pts',(-1.75068223726419,-2.39779193106209,
112.26425831217));
#40768=CARTESIAN_POINT('Ctrl Pts',(-2.96441101128674,0.162978550551776,
112.105889404386));
#40769=CARTESIAN_POINT('Ctrl Pts',(-1.47727307149132,2.57525832670406,111.947520496602));
#40770=CARTESIAN_POINT('Ctrl Pts',(1.35580319689812,2.64122901850209,111.789151588818));
#40771=CARTESIAN_POINT('Ctrl Pts',(2.95361168609557,0.300783824886337,111.630782681033));
#40772=CARTESIAN_POINT('Ctrl Pts',(1.86039364756782,-2.31370438394716,111.472413773249));
#40773=CARTESIAN_POINT('Ctrl Pts',(-0.927823163173134,-2.82018384751469,
111.314044865465));
#40774=CARTESIAN_POINT('Ctrl Pts',(-2.87070322299844,-0.757202564195071,
111.155675957681));
#40775=CARTESIAN_POINT('Ctrl Pts',(-2.19809452053784,1.99566358691141,110.997307049897));
#40776=CARTESIAN_POINT('Ctrl Pts',(0.477191227671217,2.93028688694483,110.838938142113));
#40777=CARTESIAN_POINT('Ctrl Pts',(2.71770954287736,1.19513494662057,110.680569234328));
#40778=CARTESIAN_POINT('Ctrl Pts',(2.48213117609004,-1.62890070910689,110.522200326544));
#40779=CARTESIAN_POINT('Ctrl Pts',(-0.014909154624417,-2.96885001591916,
110.36383141876));
#40780=CARTESIAN_POINT('Ctrl Pts',(-2.49836580171648,-1.60388934139893,
110.205462510976));
#40781=CARTESIAN_POINT('Ctrl Pts',(-2.70556916664848,1.22236990419424,110.047093603192));
#40782=CARTESIAN_POINT('Ctrl Pts',(-0.447736910999243,2.93493174661639,
109.888724695407));
#40783=CARTESIAN_POINT('Ctrl Pts',(2.21802704647083,1.97348643767599,109.730355787623));
#40784=CARTESIAN_POINT('Ctrl Pts',(2.86295348671375,-0.785996203200543,
109.571986879839));
#40785=CARTESIAN_POINT('Ctrl Pts',(0.899451943594493,-2.82936015730887,
109.413617972055));
#40786=CARTESIAN_POINT('Ctrl Pts',(-1.88353745718526,-2.29490290556113,
109.255249064271));
#40787=CARTESIAN_POINT('Ctrl Pts',(-2.95044176126821,0.330433218571872,
109.096880156487));
#40788=CARTESIAN_POINT('Ctrl Pts',(-1.32920778817003,2.6547126689056,108.938511248703));
#40789=CARTESIAN_POINT('Ctrl Pts',(1.5030632508415,2.56029169481628,108.780142340918));
#40790=CARTESIAN_POINT('Ctrl Pts',(2.96589805469058,0.133196951009745,108.621773433134));
#40791=CARTESIAN_POINT('Ctrl Pts',(1.72651240067488,-2.41525311901104,108.46340452535));
#40792=CARTESIAN_POINT('Ctrl Pts',(-1.08589331129042,-2.76317361290795,
108.305035617566));
#40793=CARTESIAN_POINT('Ctrl Pts',(-2.90894501758196,-0.593575254926628,
108.146666709782));
#40794=CARTESIAN_POINT('Ctrl Pts',(-2.08166600030632,2.11682766463048,107.988297801997));
#40795=CARTESIAN_POINT('Ctrl Pts',(0.642212410725931,2.89859550784268,107.829928894213));
#40796=CARTESIAN_POINT('Ctrl Pts',(2.78097309938266,1.03946203349913,107.671559986429));
#40797=CARTESIAN_POINT('Ctrl Pts',(2.38599787960529,-1.76672205428449,107.513191078645));
#40798=CARTESIAN_POINT('Ctrl Pts',(-0.182852559010247,-2.96325119425262,
107.354822170861));
#40799=CARTESIAN_POINT('Ctrl Pts',(-2.58510660199141,-1.45997142263697,
107.196453263076));
#40800=CARTESIAN_POINT('Ctrl Pts',(-2.63207809080127,1.37348375399935,107.038084355292));
#40801=CARTESIAN_POINT('Ctrl Pts',(-0.28097144863377,2.95556217048953,106.879715447508));
#40802=CARTESIAN_POINT('Ctrl Pts',(2.32612740316932,1.84483712094075,106.721346539724));
#40803=CARTESIAN_POINT('Ctrl Pts',(2.81389884029478,-0.946713269772759,
106.56297763194));
#40804=CARTESIAN_POINT('Ctrl Pts',(0.73793582923783,-2.87571615610847,106.404608724156));
#40805=CARTESIAN_POINT('Ctrl Pts',(-2.0103582119449,-2.18466303082235,106.246239816371));
#40806=CARTESIAN_POINT('Ctrl Pts',(-2.92702116271869,0.496829761158795,
106.087870908587));
#40807=CARTESIAN_POINT('Ctrl Pts',(-1.1768842705263,2.72566250888916,105.929502000803));
#40808=CARTESIAN_POINT('Ctrl Pts',(1.64550820621875,2.47115265450012,105.771133093019));
#40809=CARTESIAN_POINT('Ctrl Pts',(2.96868329368197,-0.0348166682739743,
105.612764185235));
#40810=CARTESIAN_POINT('Ctrl Pts',(1.58710030073077,-2.50906463328398,105.454395277451));
#40811=CARTESIAN_POINT('Ctrl Pts',(-1.24048482116616,-2.6973116444031,105.296026369666));
#40812=CARTESIAN_POINT('Ctrl Pts',(-2.9378680953883,-0.42804643752246,105.137657461882));
#40813=CARTESIAN_POINT('Ctrl Pts',(-1.95856892015396,2.23121054219076,104.979288554098));
#40814=CARTESIAN_POINT('Ctrl Pts',(0.805176283428797,2.85761856292613,104.820919646314));
#40815=CARTESIAN_POINT('Ctrl Pts',(2.83532788900229,0.880459232686007,104.66255073853));
#40816=CARTESIAN_POINT('Ctrl Pts',(2.2822211070191,-1.8988837555924,104.504181830746));
#40817=CARTESIAN_POINT('Ctrl Pts',(-0.350210200298097,-2.94815968261277,
104.345812922961));
#40818=CARTESIAN_POINT('Ctrl Pts',(-2.66356608750706,-1.31137652718754,
104.187444015177));
#40819=CARTESIAN_POINT('Ctrl Pts',(-2.55015522824801,1.52019768793913,104.029075107393));
#40820=CARTESIAN_POINT('Ctrl Pts',(-0.113305902314361,2.96672453575942,
103.870706199609));
#40821=CARTESIAN_POINT('Ctrl Pts',(2.42677607746812,1.71027792139309,103.712337291825));
#40822=CARTESIAN_POINT('Ctrl Pts',(2.75582994965227,-1.10439756753432,103.553968384041));
#40823=CARTESIAN_POINT('Ctrl Pts',(0.574055758622828,-2.91285988069597,
103.395599476256));
#40824=CARTESIAN_POINT('Ctrl Pts',(-2.13073884184133,-2.06742465072972,
103.237230568472));
#40825=CARTESIAN_POINT('Ctrl Pts',(-2.89422393583557,0.661634723856482,
103.078861660688));
#40826=CARTESIAN_POINT('Ctrl Pts',(-1.02079063788135,2.78788076721189,102.920492752904));
#40827=CARTESIAN_POINT('Ctrl Pts',(1.78268182325912,2.37409734754027,102.76212384512));
#40828=CARTESIAN_POINT('Ctrl Pts',(2.96195844089894,-0.202718753359468,
102.603754937335));
#40829=CARTESIAN_POINT('Ctrl Pts',(1.44260397049946,-2.59483843097703,102.445386029551));
#40830=CARTESIAN_POINT('Ctrl Pts',(-1.39110247350075,-2.62280891541804,
102.287017121767));
#40831=CARTESIAN_POINT('Ctrl Pts',(-2.9573797970241,-0.261146385634254,
102.128648213983));
#40832=CARTESIAN_POINT('Ctrl Pts',(-1.82919762064763,2.33844580078163,101.970279306199));
#40833=CARTESIAN_POINT('Ctrl Pts',(0.965560797004244,2.80748731891433,101.811910398415));
#40834=CARTESIAN_POINT('Ctrl Pts',(2.88059978706116,0.718635905977031,101.65354149063));
#40835=CARTESIAN_POINT('Ctrl Pts',(2.1711333045823,-2.02496243725894,101.495172582846));
#40836=CARTESIAN_POINT('Ctrl Pts',(-0.516445953255115,-2.92362382599791,
101.336803675062));
#40837=CARTESIAN_POINT('Ctrl Pts',(-2.73349291546608,-1.15858067465021,
101.178434767278));
#40838=CARTESIAN_POINT('Ctrl Pts',(-2.46006301657252,1.66204171219262,101.020065859494));
#40839=CARTESIAN_POINT('Ctrl Pts',(0.0547226162129466,2.96838308407986,
100.861696951709));
#40840=CARTESIAN_POINT('Ctrl Pts',(2.51965064421505,1.57023989558361,100.703328043925));
#40841=CARTESIAN_POINT('Ctrl Pts',(2.68893283681732,-1.25854395936773,100.544959136141));
#40842=CARTESIAN_POINT('Ctrl Pts',(0.408336716851919,-2.94067234221196,
100.386590228357));
#40843=CARTESIAN_POINT('Ctrl Pts',(-2.24429371097833,-1.94356333507155,
100.228221320573));
#40844=CARTESIAN_POINT('Ctrl Pts',(-2.85215514559521,0.82432015869297,100.069852412789));
#40845=CARTESIAN_POINT('Ctrl Pts',(-0.861426931709219,2.84116812947223,
99.9114835050046));
#40846=CARTESIAN_POINT('Ctrl Pts',(1.91414467021469,2.26943668781942,99.7531145972204));
#40847=CARTESIAN_POINT('Ctrl Pts',(2.94574503921539,-0.369971434715065,
99.5947456894364));
#40848=CARTESIAN_POINT('Ctrl Pts',(1.29348629982829,-2.6722997382263,99.4363767816521));
#40849=CARTESIAN_POINT('Ctrl Pts',(-1.53726376896229,-2.53990409323553,
99.2780078738679));
#40850=CARTESIAN_POINT('Ctrl Pts',(-2.96741761731905,-0.0934097589338181,
99.1196389660839));
#40851=CARTESIAN_POINT('Ctrl Pts',(-1.69396653902206,2.43818991561124,98.9612700582995));
#40852=CARTESIAN_POINT('Ctrl Pts',(1.12285216423963,2.74836236925,98.8029011505155));
#40853=CARTESIAN_POINT('Ctrl Pts',(2.91664376638008,0.554510450863373,98.6445322427313));
#40854=CARTESIAN_POINT('Ctrl Pts',(2.05309033878933,-2.14455421203033,98.4861633349471));
#40855=CARTESIAN_POINT('Ctrl Pts',(-0.681027286229073,-2.88972221999867,
98.3277944271628));
#40856=CARTESIAN_POINT('Ctrl Pts',(-2.79466307764877,-1.00207335070038,
98.1694255193788));
#40857=CARTESIAN_POINT('Ctrl Pts',(-2.36209006286334,1.79856145038909,98.0110566115945));
#40858=CARTESIAN_POINT('Ctrl Pts',(0.222575830971204,2.96053246894448,97.8526877038105));
#40859=CARTESIAN_POINT('Ctrl Pts',(2.60445358524196,1.42517171732879,97.694318796026));
#40860=CARTESIAN_POINT('Ctrl Pts',(2.61342179915298,-1.40865877224002,97.5359498882422));
#40861=CARTESIAN_POINT('Ctrl Pts',(0.241309591229933,-2.95906418622381,
97.3775809804578));
#40862=CARTESIAN_POINT('Ctrl Pts',(-2.35065907154996,-1.81347638008271,
97.2192120726736));
#40863=CARTESIAN_POINT('Ctrl Pts',(-2.80094951474737,0.984365915894731,
97.0608431648896));
#40864=CARTESIAN_POINT('Ctrl Pts',(-0.699303754895083,2.88535189771308,
96.9024742571053));
#40865=CARTESIAN_POINT('Ctrl Pts',(2.03947577929237,2.15750989357752,96.7441053493211));
#40866=CARTESIAN_POINT('Ctrl Pts',(2.92009469238337,-0.536046713828397,
96.5857364415371));
#40867=CARTESIAN_POINT('Ctrl Pts',(1.14022564598408,-2.74118500851093,96.4273675337527));
#40868=CARTESIAN_POINT('Ctrl Pts',(-1.67850179489484,-2.4488932083942,96.2689986259687));
#40869=CARTESIAN_POINT('Ctrl Pts',(-2.96794680897129,0.0746862948706615,
96.1106297181844));
#40870=CARTESIAN_POINT('Ctrl Pts',(-1.55331400689361,2.53000436455518,95.9522608104003));
#40871=CARTESIAN_POINT('Ctrl Pts',(1.27655663025386,2.68066837124582,95.7938919026161));
#40872=CARTESIAN_POINT('Ctrl Pts',(2.94332439144243,0.388143446048883,95.6355229948319));
#40873=CARTESIAN_POINT('Ctrl Pts',(1.92850931842858,-2.25635491163392,95.4771540870476));
#40874=CARTESIAN_POINT('Ctrl Pts',(-0.84349783511098,-2.84840112038291,
95.3187851792635));
#40875=CARTESIAN_POINT('Ctrl Pts',(-2.84681046706935,-0.838526963558023,
95.1604162714794));
#40876=CARTESIAN_POINT('Ctrl Pts',(-2.4526421375296,0.999904835567503,95.0548369996233));
#40877=CARTESIAN_POINT('Ctrl Pts',(-1.91077069800722,1.63368275996136,95.0020473636952));
#40878=CARTESIAN_POINT('Ctrl Pts',(-0.793799282533084,-2.96922295374563,
114.));
#40879=CARTESIAN_POINT('Ctrl Pts',(-0.887756405416284,-2.93485301849123,
114.));
#40880=CARTESIAN_POINT('Ctrl Pts',(-0.979607394515572,-2.89562354334601,
114.));
#40881=CARTESIAN_POINT('Ctrl Pts',(-1.06913777784631,-2.8518719612289,114.));
#40882=CARTESIAN_POINT('Ctrl Pts',(-1.15999321053621,-2.80747285584995,
114.));
#40883=CARTESIAN_POINT('Ctrl Pts',(-1.24845948656086,-2.7584161121202,114.));
#40884=CARTESIAN_POINT('Ctrl Pts',(-1.33428309468856,-2.70500832173497,
114.));
#40885=CARTESIAN_POINT('Ctrl Pts',(-1.4201843897322,-2.65155218700005,114.));
#40886=CARTESIAN_POINT('Ctrl Pts',(-1.50343881675033,-2.59373634276815,
114.));
#40887=CARTESIAN_POINT('Ctrl Pts',(-1.58375375152654,-2.53183366530801,
114.));
#40888=CARTESIAN_POINT('Ctrl Pts',(-1.64735338850338,-2.48281429144772,
114.));
#40889=CARTESIAN_POINT('Ctrl Pts',(-1.70910910828567,-2.43123137544921,
114.));
#40890=CARTESIAN_POINT('Ctrl Pts',(-1.76885487784217,-2.37720991548722,
114.));
#40891=CARTESIAN_POINT('Ctrl Pts',(-1.78256802692274,-2.36481063869311,
114.));
#40892=CARTESIAN_POINT('Ctrl Pts',(-1.79617749974221,-2.3522805878216,114.));
#40893=CARTESIAN_POINT('Ctrl Pts',(-1.80966297662315,-2.33963863235335,
114.));
#40894=CARTESIAN_POINT('Ctrl Pts',(-1.88210098192872,-2.2717316502446,114.));
#40895=CARTESIAN_POINT('Ctrl Pts',(-1.95107281091722,-2.20050300321149,
114.));
#40896=CARTESIAN_POINT('Ctrl Pts',(-2.01633867799913,-2.12624319266344,
114.));
#40897=CARTESIAN_POINT('Ctrl Pts',(-2.08124950129726,-2.05238735260256,
114.));
#40898=CARTESIAN_POINT('Ctrl Pts',(-2.14249506046558,-1.97553244140376,
114.));
#40899=CARTESIAN_POINT('Ctrl Pts',(-2.19979582352635,-1.89593746805701,
114.));
#40900=CARTESIAN_POINT('Ctrl Pts',(-2.25579080895265,-1.81815631586134,
114.));
#40901=CARTESIAN_POINT('Ctrl Pts',(-2.30801903030654,-1.73775782070226,
114.));
#40902=CARTESIAN_POINT('Ctrl Pts',(-2.35617234908628,-1.6549694155717,114.));
#40903=CARTESIAN_POINT('Ctrl Pts',(-2.37613161281103,-1.620654114919,114.));
#40904=CARTESIAN_POINT('Ctrl Pts',(-2.39539019249454,-1.58592810520914,
114.));
#40905=CARTESIAN_POINT('Ctrl Pts',(-2.41392350328627,-1.55080728403562,
114.));
#40906=CARTESIAN_POINT('Ctrl Pts',(-2.42930717614674,-1.52165506025888,
114.));
#40907=CARTESIAN_POINT('Ctrl Pts',(-2.44419111793619,-1.49223081023459,
114.));
#40908=CARTESIAN_POINT('Ctrl Pts',(-2.45856039815702,-1.46254361992092,
114.));
#40909=CARTESIAN_POINT('Ctrl Pts',(-2.46495040099425,-1.44934175960374,
114.));
#40910=CARTESIAN_POINT('Ctrl Pts',(-2.47123463557079,-1.4360960866698,114.));
#40911=CARTESIAN_POINT('Ctrl Pts',(-2.47741091898805,-1.42281028747023,
114.));
#40912=CARTESIAN_POINT('Ctrl Pts',(-2.51759768923482,-1.33636455240484,
114.));
#40913=CARTESIAN_POINT('Ctrl Pts',(-2.55323686315738,-1.24818320074038,
114.));
#40914=CARTESIAN_POINT('Ctrl Pts',(-2.58406781887899,-1.15850854008231,
114.));
#40915=CARTESIAN_POINT('Ctrl Pts',(-2.6148987746006,-1.06883387942424,114.));
#40916=CARTESIAN_POINT('Ctrl Pts',(-2.64092196711114,-0.977665187699464,
114.));
#40917=CARTESIAN_POINT('Ctrl Pts',(-2.66182132438789,-0.885235488973918,
114.));
#40918=CARTESIAN_POINT('Ctrl Pts',(-2.66314166753101,-0.879396126675976,
114.));
#40919=CARTESIAN_POINT('Ctrl Pts',(-2.66444154050489,-0.873551730452811,
114.));
#40920=CARTESIAN_POINT('Ctrl Pts',(-2.66572085552459,-0.867702358851152,
114.));
#40921=CARTESIAN_POINT('Ctrl Pts',(-2.68608266907363,-0.774602682775677,
114.));
#40922=CARTESIAN_POINT('Ctrl Pts',(-2.7012408677073,-0.680241604070945,
114.));
#40923=CARTESIAN_POINT('Ctrl Pts',(-2.71127329807981,-0.58502826549681,
114.));
#40924=CARTESIAN_POINT('Ctrl Pts',(-2.71432415693148,-0.556073919839703,
114.));
#40925=CARTESIAN_POINT('Ctrl Pts',(-2.71690065119253,-0.527040860992301,
114.));
#40926=CARTESIAN_POINT('Ctrl Pts',(-2.71900407437446,-0.497940927530195,
114.));
#40927=CARTESIAN_POINT('Ctrl Pts',(-2.72063483457608,-0.475380078259617,
114.));
#40928=CARTESIAN_POINT('Ctrl Pts',(-2.72198123645291,-0.452779035766268,
114.));
#40929=CARTESIAN_POINT('Ctrl Pts',(-2.72304371940055,-0.430143407437012,
114.));
#40930=CARTESIAN_POINT('Ctrl Pts',(-2.72369452838722,-0.41627827165448,
114.));
#40931=CARTESIAN_POINT('Ctrl Pts',(-2.72423869350137,-0.402401224478398,
114.));
#40932=CARTESIAN_POINT('Ctrl Pts',(-2.72467613491267,-0.388526209993681,
114.));
#40933=CARTESIAN_POINT('Ctrl Pts',(-2.72760970254779,-0.29547764993958,
114.));
#40934=CARTESIAN_POINT('Ctrl Pts',(-2.72575570446157,-0.202367859072132,
114.));
#40935=CARTESIAN_POINT('Ctrl Pts',(-2.71925034893427,-0.109570485685123,
114.));
#40936=CARTESIAN_POINT('Ctrl Pts',(-2.71271344795737,-0.0163231238456995,
114.));
#40937=CARTESIAN_POINT('Ctrl Pts',(-2.70147961390672,0.0766097727305058,
114.));
#40938=CARTESIAN_POINT('Ctrl Pts',(-2.68563588787195,0.168836959232147,
114.));
#40939=CARTESIAN_POINT('Ctrl Pts',(-2.67002467875455,0.259710652177,114.));
#40940=CARTESIAN_POINT('Ctrl Pts',(-2.6499374210433,0.349900044984494,114.));
#40941=CARTESIAN_POINT('Ctrl Pts',(-2.62541421207747,0.439005547405842,
114.));
#40942=CARTESIAN_POINT('Ctrl Pts',(-2.61599341629587,0.473236171240522,
114.));
#40943=CARTESIAN_POINT('Ctrl Pts',(-2.60591755234073,0.507306502518509,
114.));
#40944=CARTESIAN_POINT('Ctrl Pts',(-2.59518738165598,0.541192473955113,
114.));
#40945=CARTESIAN_POINT('Ctrl Pts',(-2.5893302318919,0.559689403355105,114.));
#40946=CARTESIAN_POINT('Ctrl Pts',(-2.58327811024553,0.578131385467199,
114.));
#40947=CARTESIAN_POINT('Ctrl Pts',(-2.57703104241714,0.596514388648216,
114.));
#40948=CARTESIAN_POINT('Ctrl Pts',(-2.57101572615014,0.614215425536017,
114.));
#40949=CARTESIAN_POINT('Ctrl Pts',(-2.56481956583144,0.63186163539755,114.));
#40950=CARTESIAN_POINT('Ctrl Pts',(-2.55844967245198,0.649430828571657,
114.));
#40951=CARTESIAN_POINT('Ctrl Pts',(-2.52769580588534,0.73425495204952,114.));
#40952=CARTESIAN_POINT('Ctrl Pts',(-2.49285847495252,0.817397602756055,
114.));
#40953=CARTESIAN_POINT('Ctrl Pts',(-2.45399738165239,0.898485836372846,
114.));
#40954=CARTESIAN_POINT('Ctrl Pts',(-2.4224968286348,0.964215438533597,114.));
#40955=CARTESIAN_POINT('Ctrl Pts',(-2.38835153732701,1.02859487584379,114.));
#40956=CARTESIAN_POINT('Ctrl Pts',(-2.35157529000334,1.09140786163922,114.));
#40957=CARTESIAN_POINT('Ctrl Pts',(-2.33607146419489,1.1178880400465,114.));
#40958=CARTESIAN_POINT('Ctrl Pts',(-2.32009987385018,1.14408960317399,114.));
#40959=CARTESIAN_POINT('Ctrl Pts',(-2.30366078197046,1.16999529935414,114.));
#40960=CARTESIAN_POINT('Ctrl Pts',(-2.28749242428528,1.19547435653008,114.));
#40961=CARTESIAN_POINT('Ctrl Pts',(-2.27088535181155,1.22064570837715,114.));
#40962=CARTESIAN_POINT('Ctrl Pts',(-2.25384672324409,1.24548702198906,114.));
#40963=CARTESIAN_POINT('Ctrl Pts',(-2.2054204117729,1.31608972252691,114.));
#40964=CARTESIAN_POINT('Ctrl Pts',(-2.15349724301452,1.38404994787183,114.));
#40965=CARTESIAN_POINT('Ctrl Pts',(-2.09810553423573,1.4490110003995,114.));
#40966=CARTESIAN_POINT('Ctrl Pts',(-2.05603144768597,1.49835370902269,114.));
#40967=CARTESIAN_POINT('Ctrl Pts',(-2.01195547754715,1.54596540514302,114.));
#40968=CARTESIAN_POINT('Ctrl Pts',(-1.96587909147006,1.59167278088311,114.));
#40969=CARTESIAN_POINT('Ctrl Pts',(-1.94985536550434,1.60756817819673,114.));
#40970=CARTESIAN_POINT('Ctrl Pts',(-1.93358962678968,1.62323311874396,114.));
#40971=CARTESIAN_POINT('Ctrl Pts',(-1.91708805188416,1.63866502517338,114.));
#40972=CARTESIAN_POINT('Origin',(0.,0.,94.));
#40973=CARTESIAN_POINT('Origin',(0.,0.,0.));
#40974=CARTESIAN_POINT('',(-8.,-9.79717439317883E-16,114.));
#40975=CARTESIAN_POINT('Origin',(0.,0.,114.));
#40976=CARTESIAN_POINT('',(-8.,-9.79717439317883E-16,0.));
#40977=CARTESIAN_POINT('',(-8.,-9.79717439317883E-16,0.));
#40978=CARTESIAN_POINT('Origin',(0.,0.,0.));
#40979=CARTESIAN_POINT('Origin',(0.,0.,114.));
#40980=CARTESIAN_POINT('Origin',(0.,0.,0.));
#94383=UNCERTAINTY_MEASURE_WITH_UNIT(LENGTH_MEASURE(0.01),#94413,
'DISTANCE_ACCURACY_VALUE',
'Maximum model space distance between geometric entities at asserted c
onnectivities');
#94394=UNCERTAINTY_MEASURE_WITH_UNIT(LENGTH_MEASURE(0.01),#94413,
'DISTANCE_ACCURACY_VALUE',
'Maximum model space distance between geometric entities at asserted c
onnectivities');
#94401=(
GEOMETRIC_REPRESENTATION_CONTEXT(3)
GLOBAL_UNCERTAINTY_ASSIGNED_CONTEXT((#94383))
GLOBAL_UNIT_ASSIGNED_CONTEXT((#94413,#94415,#94416))
REPRESENTATION_CONTEXT('','3D')
);
#94412=(
GEOMETRIC_REPRESENTATION_CONTEXT(3)
GLOBAL_UNCERTAINTY_ASSIGNED_CONTEXT((#94394))
GLOBAL_UNIT_ASSIGNED_CONTEXT((#94413,#94415,#94416))
REPRESENTATION_CONTEXT('','3D')
);
#94413=(
LENGTH_UNIT()
NAMED_UNIT(*)
SI_UNIT(.MILLI.,.METRE.)
);
#94415=(
NAMED_UNIT(*)
PLANE_ANGLE_UNIT()
SI_UNIT($,.RADIAN.)
);
#94416=(
NAMED_UNIT(*)
SI_UNIT($,.STERADIAN.)
SOLID_ANGLE_UNIT()
);
#94423=SHAPE_DEFINITION_REPRESENTATION(#94440,#94492);
#94440=PRODUCT_DEFINITION_SHAPE('',$,#94510);
#94492=SHAPE_REPRESENTATION('',(#8512),#94401);
#94503=PRODUCT_DEFINITION_CONTEXT('part definition',#94556,'design');
#94510=PRODUCT_DEFINITION('Corner pillar','Corner pillar',#94527,#94503);
#94527=PRODUCT_DEFINITION_FORMATION('',$,#94564);
#94556=APPLICATION_CONTEXT(
'Core Data for Automotive Mechanical Design Process');
#94557=PRODUCT_CONTEXT('part definition',#94556,'mechanical');
#94564=PRODUCT('Corner pillar','Corner pillar',$,(#94557));
#94577=PRESENTATION_STYLE_ASSIGNMENT((#94584));
#94584=SURFACE_STYLE_USAGE(.BOTH.,#94591);
#94591=SURFACE_SIDE_STYLE('',(#94598));
#94598=SURFACE_STYLE_FILL_AREA(#94605);
#94605=FILL_AREA_STYLE('Opaque(104,114,127)',(#94612));
#94612=FILL_AREA_STYLE_COLOUR('Opaque(104,114,127)',#94619);
#94619=COLOUR_RGB('Opaque(104,114,127)',0.407843137254902,0.447058823529412,
0.498039215686275);
ENDSEC;
END-ISO-10303-21;
